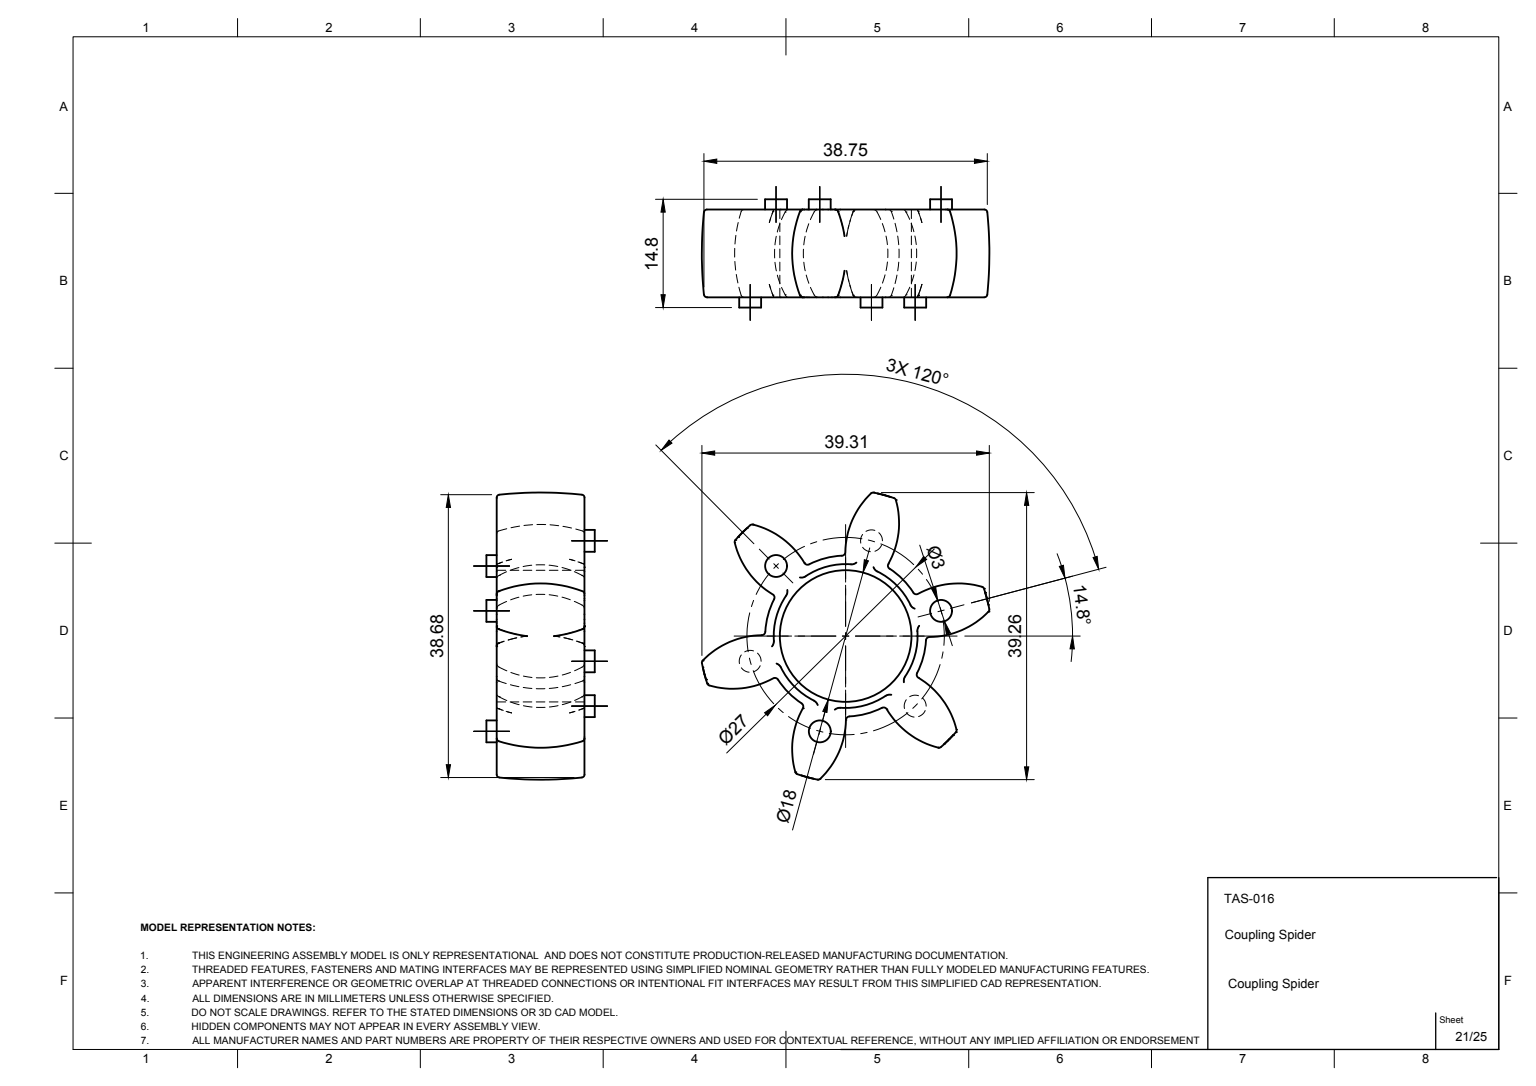
ISO-10303-21;
HEADER;
/* Generated by software containing ST-Developer
 * from STEP Tools, Inc. (www.steptools.com) 
 */

FILE_DESCRIPTION(
/* description */ ('STEP AP214'),
/* implementation_level */ '2;1');

FILE_NAME(
/* name */ 'Coupling Spider.step',
/* time_stamp */ '2026-11-15T14:55:55-08:00',
/* author */ (''),
/* organization */ (''),
/* preprocessor_version */ 'ST-DEVELOPER v20.2',
/* originating_system */ 'Autodesk Translation Framework v15.17.0.0',
/* authorisation */ '');

FILE_SCHEMA (('AUTOMOTIVE_DESIGN { 1 0 10303 214 3 1 1 }'));
ENDSEC;

DATA;
#10=MECHANICAL_DESIGN_GEOMETRIC_PRESENTATION_REPRESENTATION('',(#939),#57079);
#36=B_SPLINE_SURFACE_WITH_KNOTS('',3,3,((#37392,#37393,#37394,#37395,#37396),
(#37397,#37398,#37399,#37400,#37401),(#37402,#37403,#37404,#37405,#37406),
(#37407,#37408,#37409,#37410,#37411),(#37412,#37413,#37414,#37415,#37416),
(#37417,#37418,#37419,#37420,#37421),(#37422,#37423,#37424,#37425,#37426)),
 .UNSPECIFIED.,.F.,.F.,.F.,(4,1,1,1,4),(4,1,4),(0.002628442342492,0.25,
0.5,0.75,0.9693574094799),(0.1621510896547,6.217857289747,12.27407139219),
 .UNSPECIFIED.);
#37=B_SPLINE_SURFACE_WITH_KNOTS('',3,3,((#38122,#38123,#38124,#38125,#38126),
(#38127,#38128,#38129,#38130,#38131),(#38132,#38133,#38134,#38135,#38136),
(#38137,#38138,#38139,#38140,#38141)),.UNSPECIFIED.,.F.,.F.,.F.,(4,4),(4,
1,4),(-0.024990257354348,0.982485330053312),(0.334063910607008,6.217857289747,
12.1016506682418),.UNSPECIFIED.);
#38=B_SPLINE_SURFACE_WITH_KNOTS('',3,3,((#38952,#38953,#38954,#38955,#38956),
(#38957,#38958,#38959,#38960,#38961),(#38962,#38963,#38964,#38965,#38966),
(#38967,#38968,#38969,#38970,#38971),(#38972,#38973,#38974,#38975,#38976),
(#38977,#38978,#38979,#38980,#38981),(#38982,#38983,#38984,#38985,#38986)),
 .UNSPECIFIED.,.F.,.F.,.F.,(4,1,1,1,4),(4,1,4),(0.0306420330999,0.25,0.5,
0.75,0.9973715693979),(0.1621509986241,6.217857289747,12.27408153313),
 .UNSPECIFIED.);
#39=B_SPLINE_SURFACE_WITH_KNOTS('',3,3,((#39922,#39923,#39924,#39925,#39926),
(#39927,#39928,#39929,#39930,#39931),(#39932,#39933,#39934,#39935,#39936),
(#39937,#39938,#39939,#39940,#39941),(#39942,#39943,#39944,#39945,#39946),
(#39947,#39948,#39949,#39950,#39951),(#39952,#39953,#39954,#39955,#39956)),
 .UNSPECIFIED.,.F.,.F.,.F.,(4,1,1,1,4),(4,1,4),(0.002628433572892,0.25,
0.5,0.75,0.9693578567347),(0.1621510896604,6.217857289747,12.27407139218),
 .UNSPECIFIED.);
#40=B_SPLINE_SURFACE_WITH_KNOTS('',3,3,((#40661,#40662,#40663,#40664,#40665),
(#40666,#40667,#40668,#40669,#40670),(#40671,#40672,#40673,#40674,#40675),
(#40676,#40677,#40678,#40679,#40680)),.UNSPECIFIED.,.F.,.F.,.F.,(4,4),(4,
1,4),(-0.0250566951233491,0.98252386483041),(0.33399816619982,6.217857289747,
12.1017164126489),.UNSPECIFIED.);
#41=B_SPLINE_SURFACE_WITH_KNOTS('',3,3,((#41491,#41492,#41493,#41494,#41495),
(#41496,#41497,#41498,#41499,#41500),(#41501,#41502,#41503,#41504,#41505),
(#41506,#41507,#41508,#41509,#41510),(#41511,#41512,#41513,#41514,#41515),
(#41516,#41517,#41518,#41519,#41520),(#41521,#41522,#41523,#41524,#41525)),
 .UNSPECIFIED.,.F.,.F.,.F.,(4,1,1,1,4),(4,1,4),(0.03064262133498,0.25,0.5,
0.75,0.9973715578641),(0.1621509986155,6.217857289747,12.27408153314),
 .UNSPECIFIED.);
#42=B_SPLINE_SURFACE_WITH_KNOTS('',3,3,((#42483,#42484,#42485,#42486,#42487),
(#42488,#42489,#42490,#42491,#42492),(#42493,#42494,#42495,#42496,#42497),
(#42498,#42499,#42500,#42501,#42502),(#42503,#42504,#42505,#42506,#42507),
(#42508,#42509,#42510,#42511,#42512),(#42513,#42514,#42515,#42516,#42517)),
 .UNSPECIFIED.,.F.,.F.,.F.,(4,1,1,1,4),(4,1,4),(0.002628427667201,0.25,
0.5,0.75,0.9693581579284),(0.1621510896466,6.217857289747,12.2740713922),
 .UNSPECIFIED.);
#43=B_SPLINE_SURFACE_WITH_KNOTS('',3,3,((#43199,#43200,#43201,#43202,#43203),
(#43204,#43205,#43206,#43207,#43208),(#43209,#43210,#43211,#43212,#43213),
(#43214,#43215,#43216,#43217,#43218)),.UNSPECIFIED.,.F.,.F.,.F.,(4,4),(4,
1,4),(-0.025111513161759,0.982555658087823),(0.333943919417255,6.217857289747,
12.1017706594305),.UNSPECIFIED.);
#44=B_SPLINE_SURFACE_WITH_KNOTS('',3,3,((#44029,#44030,#44031,#44032,#44033),
(#44034,#44035,#44036,#44037,#44038),(#44039,#44040,#44041,#44042,#44043),
(#44044,#44045,#44046,#44047,#44048),(#44049,#44050,#44051,#44052,#44053),
(#44054,#44055,#44056,#44057,#44058),(#44059,#44060,#44061,#44062,#44063)),
 .UNSPECIFIED.,.F.,.F.,.F.,(4,1,1,1,4),(4,1,4),(0.0306416740573,0.25,0.5,
0.75,0.9973715764379),(0.1621509986173,6.217857289747,12.27408153313),
 .UNSPECIFIED.);
#45=B_SPLINE_SURFACE_WITH_KNOTS('',3,3,((#45013,#45014,#45015,#45016,#45017),
(#45018,#45019,#45020,#45021,#45022),(#45023,#45024,#45025,#45026,#45027),
(#45028,#45029,#45030,#45031,#45032),(#45033,#45034,#45035,#45036,#45037),
(#45038,#45039,#45040,#45041,#45042),(#45043,#45044,#45045,#45046,#45047)),
 .UNSPECIFIED.,.F.,.F.,.F.,(4,1,1,1,4),(4,1,4),(0.002628398063673,0.25,
0.5,0.75,0.9693596677257),(0.1621510897017,6.217857289747,12.27407139231),
 .UNSPECIFIED.);
#46=B_SPLINE_SURFACE_WITH_KNOTS('',3,3,((#45733,#45734,#45735,#45736,#45737),
(#45738,#45739,#45740,#45741,#45742),(#45743,#45744,#45745,#45746,#45747),
(#45748,#45749,#45750,#45751,#45752)),.UNSPECIFIED.,.F.,.F.,.F.,(4,4),(4,
1,4),(-0.0251115131966662,0.982555658077179),(0.3339439193833,6.217857289747,
12.1017706594645),.UNSPECIFIED.);
#47=B_SPLINE_SURFACE_WITH_KNOTS('',3,3,((#46556,#46557,#46558,#46559,#46560),
(#46561,#46562,#46563,#46564,#46565),(#46566,#46567,#46568,#46569,#46570),
(#46571,#46572,#46573,#46574,#46575),(#46576,#46577,#46578,#46579,#46580),
(#46581,#46582,#46583,#46584,#46585),(#46586,#46587,#46588,#46589,#46590)),
 .UNSPECIFIED.,.F.,.F.,.F.,(4,1,1,1,4),(4,1,4),(0.03064220512297,0.25,0.5,
0.75,0.997371566025),(0.1621509986341,6.217857289747,12.27408153327),
 .UNSPECIFIED.);
#48=B_SPLINE_SURFACE_WITH_KNOTS('',3,3,((#47286,#47287,#47288,#47289,#47290),
(#47291,#47292,#47293,#47294,#47295),(#47296,#47297,#47298,#47299,#47300),
(#47301,#47302,#47303,#47304,#47305),(#47306,#47307,#47308,#47309,#47310),
(#47311,#47312,#47313,#47314,#47315),(#47316,#47317,#47318,#47319,#47320)),
 .UNSPECIFIED.,.F.,.F.,.F.,(4,1,1,1,4),(4,1,4),(0.002628430752027,0.25,
0.5,0.75,0.9693580006005),(0.1621510896555,6.217857289747,12.27407139218),
 .UNSPECIFIED.);
#49=B_SPLINE_SURFACE_WITH_KNOTS('',3,3,((#48651,#48652,#48653,#48654,#48655),
(#48656,#48657,#48658,#48659,#48660),(#48661,#48662,#48663,#48664,#48665),
(#48666,#48667,#48668,#48669,#48670),(#48671,#48672,#48673,#48674,#48675),
(#48676,#48677,#48678,#48679,#48680),(#48681,#48682,#48683,#48684,#48685)),
 .UNSPECIFIED.,.F.,.F.,.F.,(4,1,1,1,4),(4,1,4),(0.002629007110398,0.25,
0.5,0.75,0.9693286059854),(0.162151089685,6.217857289747,12.27407139234),
 .UNSPECIFIED.);
#50=B_SPLINE_SURFACE_WITH_KNOTS('',3,3,((#49402,#49403,#49404,#49405,#49406),
(#49407,#49408,#49409,#49410,#49411),(#49412,#49413,#49414,#49415,#49416),
(#49417,#49418,#49419,#49420,#49421)),.UNSPECIFIED.,.F.,.F.,.F.,(4,4),(4,
1,4),(-0.025177674866951,0.982594028216162),(0.333878446168046,6.217857289747,
12.1018361326796),.UNSPECIFIED.);
#51=B_SPLINE_SURFACE_WITH_KNOTS('',3,3,((#50226,#50227,#50228,#50229,#50230),
(#50231,#50232,#50233,#50234,#50235),(#50236,#50237,#50238,#50239,#50240),
(#50241,#50242,#50243,#50244,#50245),(#50246,#50247,#50248,#50249,#50250),
(#50251,#50252,#50253,#50254,#50255),(#50256,#50257,#50258,#50259,#50260)),
 .UNSPECIFIED.,.F.,.F.,.F.,(4,1,1,1,4),(4,1,4),(0.03067153885244,0.25,0.5,
0.75,0.9973709908605),(0.1621509986464,6.217857289747,12.27408153326),
 .UNSPECIFIED.);
#52=B_SPLINE_SURFACE_WITH_KNOTS('',3,3,((#50705,#50706,#50707,#50708,#50709),
(#50710,#50711,#50712,#50713,#50714),(#50715,#50716,#50717,#50718,#50719),
(#50720,#50721,#50722,#50723,#50724)),.UNSPECIFIED.,.F.,.F.,.F.,(4,4),(4,
1,4),(-0.0249902573400751,0.982485330102956),(0.334063910620545,6.217857289747,
12.1016506682281),.UNSPECIFIED.);
#53=B_SPLINE_SURFACE_WITH_KNOTS('',3,3,((#51211,#51212,#51213,#51214,#51215),
(#51216,#51217,#51218,#51219,#51220),(#51221,#51222,#51223,#51224,#51225),
(#51226,#51227,#51228,#51229,#51230),(#51231,#51232,#51233,#51234,#51235),
(#51236,#51237,#51238,#51239,#51240),(#51241,#51242,#51243,#51244,#51245)),
 .UNSPECIFIED.,.F.,.F.,.F.,(4,1,1,1,4),(4,1,4),(0.03064179013217,0.25,0.5,
0.75,0.997371574162),(0.1621509986021,6.217857289747,12.27408153315),
 .UNSPECIFIED.);
#54=ELLIPSE('',#25490,14.1459545202442,4.90175276915756);
#55=ELLIPSE('',#25504,38.974702057433,37.2141854840257);
#56=ELLIPSE('',#25512,14.1454026092901,4.90137019917901);
#57=ELLIPSE('',#25526,38.9778279365771,37.2201555784017);
#58=ELLIPSE('',#25534,14.1449420010391,4.90105113596068);
#59=ELLIPSE('',#25548,38.975599782719,37.215899615947);
#60=ELLIPSE('',#25556,14.1449570638359,4.90106151145033);
#61=ELLIPSE('',#25570,38.9740482939914,37.2129370257381);
#62=ELLIPSE('',#25579,14.14611930392,4.90186695347628);
#63=ELLIPSE('',#25593,14.1445653378396,4.90078996091196);
#64=ELLIPSE('',#25607,38.9767662731696,37.2181280215083);
#65=ELLIPSE('',#25633,38.97568443858,37.2160612851944);
#162=(
BOUNDED_SURFACE()
B_SPLINE_SURFACE(3,3,((#36423,#36424,#36425,#36426,#36427,#36428,#36429,
#36430,#36431,#36432),(#36433,#36434,#36435,#36436,#36437,#36438,#36439,
#36440,#36441,#36442),(#36443,#36444,#36445,#36446,#36447,#36448,#36449,
#36450,#36451,#36452),(#36453,#36454,#36455,#36456,#36457,#36458,#36459,
#36460,#36461,#36462)),.UNSPECIFIED.,.F.,.F.,.F.)
B_SPLINE_SURFACE_WITH_KNOTS((4,4),(4,1,1,1,1,1,1,4),(0.0902477597713112,
0.904395368827396),(0.02358777781772,0.1427066556452,0.2856868894759,0.4285070295258,
0.571316470583,0.7141880571253,0.8571205016359,0.9886565450754),
 .UNSPECIFIED.)
GEOMETRIC_REPRESENTATION_ITEM()
RATIONAL_B_SPLINE_SURFACE(((1.11546174586943,1.11546174586943,1.11546174586943,
1.11546174586943,1.11546174586943,1.11546174586943,1.11546174586943,1.11546174586943,
1.11546174586943,1.11546174586943),(0.962519072862034,0.962519072862034,
0.962519072862034,0.962519072862034,0.962519072862034,0.962519072862034,
0.962519072862034,0.962519072862034,0.962519072862034,0.962519072862034),
(0.96151932941876,0.96151932941876,0.96151932941876,0.96151932941876,0.96151932941876,
0.96151932941876,0.96151932941876,0.96151932941876,0.96151932941876,0.96151932941876),
(1.1124625155396,1.1124625155396,1.1124625155396,1.1124625155396,1.1124625155396,
1.1124625155396,1.1124625155396,1.1124625155396,1.1124625155396,1.1124625155396)))
REPRESENTATION_ITEM('')
SURFACE()
);
#163=(
BOUNDED_SURFACE()
B_SPLINE_SURFACE(3,3,((#36555,#36556,#36557,#36558,#36559,#36560,#36561,
#36562,#36563),(#36564,#36565,#36566,#36567,#36568,#36569,#36570,#36571,
#36572),(#36573,#36574,#36575,#36576,#36577,#36578,#36579,#36580,#36581),
(#36582,#36583,#36584,#36585,#36586,#36587,#36588,#36589,#36590)),
 .UNSPECIFIED.,.F.,.F.,.F.)
B_SPLINE_SURFACE_WITH_KNOTS((4,4),(4,1,1,1,1,1,4),(0.0546212561079652,0.945380228523745),
(0.228750194394892,0.3042889925712,0.4133392424319,0.5264696341084,0.6424947869233,
0.7601009691825,0.774320140471063),.UNSPECIFIED.)
GEOMETRIC_REPRESENTATION_ITEM()
RATIONAL_B_SPLINE_SURFACE(((1.19596662858113,1.19596662858113,1.19596662858113,
1.19596662858113,1.19596662858113,1.19596662858113,1.19596662858113,1.19596662858113,
1.19596662858113),(0.934677354980995,0.934677354980995,0.934677354980995,
0.934677354980995,0.934677354980995,0.934677354980995,0.934677354980995,
0.934677354980995,0.934677354980995),(0.934677790473648,0.934677790473648,
0.934677790473648,0.934677790473648,0.934677790473648,0.934677790473648,
0.934677790473648,0.934677790473648,0.934677790473648),(1.19596793505909,
1.19596793505909,1.19596793505909,1.19596793505909,1.19596793505909,1.19596793505909,
1.19596793505909,1.19596793505909,1.19596793505909)))
REPRESENTATION_ITEM('')
SURFACE()
);
#164=(
BOUNDED_SURFACE()
B_SPLINE_SURFACE(3,3,((#36641,#36642,#36643,#36644,#36645,#36646,#36647,
#36648,#36649),(#36650,#36651,#36652,#36653,#36654,#36655,#36656,#36657,
#36658),(#36659,#36660,#36661,#36662,#36663,#36664,#36665,#36666,#36667),
(#36668,#36669,#36670,#36671,#36672,#36673,#36674,#36675,#36676)),
 .UNSPECIFIED.,.F.,.F.,.F.)
B_SPLINE_SURFACE_WITH_KNOTS((4,4),(4,1,1,1,1,1,4),(0.0545959214790058,0.945405071292651),
(0.226579922118566,0.3006458185639,0.4098657082077,0.5233967602133,0.640305105005,
0.7591301880899,0.772969164981535),.UNSPECIFIED.)
GEOMETRIC_REPRESENTATION_ITEM()
RATIONAL_B_SPLINE_SURFACE(((1.19598782351354,1.19598782351354,1.19598782351354,
1.19598782351354,1.19598782351354,1.19598782351354,1.19598782351354,1.19598782351354,
1.19598782351354),(0.934670434267463,0.934670434267463,0.934670434267463,
0.934670434267463,0.934670434267463,0.934670434267463,0.934670434267463,
0.934670434267463,0.934670434267463),(0.93467072549571,0.93467072549571,
0.93467072549571,0.93467072549571,0.93467072549571,0.93467072549571,0.93467072549571,
0.93467072549571,0.93467072549571),(1.19598869719828,1.19598869719828,1.19598869719828,
1.19598869719828,1.19598869719828,1.19598869719828,1.19598869719828,1.19598869719828,
1.19598869719828)))
REPRESENTATION_ITEM('')
SURFACE()
);
#165=(
BOUNDED_SURFACE()
B_SPLINE_SURFACE(3,3,((#36787,#36788,#36789,#36790,#36791,#36792,#36793,
#36794,#36795,#36796,#36797),(#36798,#36799,#36800,#36801,#36802,#36803,
#36804,#36805,#36806,#36807,#36808),(#36809,#36810,#36811,#36812,#36813,
#36814,#36815,#36816,#36817,#36818,#36819),(#36820,#36821,#36822,#36823,
#36824,#36825,#36826,#36827,#36828,#36829,#36830)),.UNSPECIFIED.,.F.,.F.,
 .F.)
B_SPLINE_SURFACE_WITH_KNOTS((4,4),(4,1,1,1,1,1,1,1,4),(0.0753633924341077,
0.903558847349357),(-0.009670337421386,0.,0.1430991485311,0.2858285059199,
0.4284781713031,0.5715215149008,0.7145472299923,0.8573672624017,0.9759160460961),
 .UNSPECIFIED.)
GEOMETRIC_REPRESENTATION_ITEM()
RATIONAL_B_SPLINE_SURFACE(((1.12354604895393,1.12354604895393,1.12354604895393,
1.12354604895393,1.12354604895393,1.12354604895393,1.12354604895393,1.12354604895393,
1.12354604895393,1.12354604895393,1.12354604895393),(0.962906301315212,
0.962906301315212,0.962906301315212,0.962906301315212,0.962906301315212,
0.962906301315212,0.962906301315212,0.962906301315212,0.962906301315212,
0.962906301315212,0.962906301315212),(0.958919449944363,0.958919449944363,
0.958919449944363,0.958919449944363,0.958919449944363,0.958919449944363,
0.958919449944363,0.958919449944363,0.958919449944363,0.958919449944363,
0.958919449944363),(1.11158549484138,1.11158549484138,1.11158549484138,
1.11158549484138,1.11158549484138,1.11158549484138,1.11158549484138,1.11158549484138,
1.11158549484138,1.11158549484138,1.11158549484138)))
REPRESENTATION_ITEM('')
SURFACE()
);
#166=(
BOUNDED_SURFACE()
B_SPLINE_SURFACE(3,3,((#36947,#36948,#36949,#36950),(#36951,#36952,#36953,
#36954),(#36955,#36956,#36957,#36958),(#36959,#36960,#36961,#36962)),
 .UNSPECIFIED.,.F.,.F.,.F.)
B_SPLINE_SURFACE_WITH_KNOTS((4,4),(4,4),(0.0986320320063612,0.901362552769513),
(-0.975145040413366,-0.0991746183846591),.UNSPECIFIED.)
GEOMETRIC_REPRESENTATION_ITEM()
RATIONAL_B_SPLINE_SURFACE(((1.17563600435392,1.17563600435392,1.17563600435392,
1.17563600435392),(0.941456244993259,0.941456244993259,0.941456244993259,
0.941456244993259),(0.941454665226083,0.941454665226083,0.941454665226083,
0.941454665226083),(1.17563126505239,1.17563126505239,1.17563126505239,
1.17563126505239)))
REPRESENTATION_ITEM('')
SURFACE()
);
#167=(
BOUNDED_SURFACE()
B_SPLINE_SURFACE(3,3,((#36981,#36982,#36983,#36984,#36985,#36986,#36987,
#36988,#36989,#36990,#36991,#36992,#36993,#36994,#36995,#36996,#36997,#36998,
#36999,#37000,#37001,#37002,#37003,#37004,#37005,#37006,#37007,#37008,#37009,
#37010,#37011,#37012,#37013),(#37014,#37015,#37016,#37017,#37018,#37019,
#37020,#37021,#37022,#37023,#37024,#37025,#37026,#37027,#37028,#37029,#37030,
#37031,#37032,#37033,#37034,#37035,#37036,#37037,#37038,#37039,#37040,#37041,
#37042,#37043,#37044,#37045,#37046),(#37047,#37048,#37049,#37050,#37051,
#37052,#37053,#37054,#37055,#37056,#37057,#37058,#37059,#37060,#37061,#37062,
#37063,#37064,#37065,#37066,#37067,#37068,#37069,#37070,#37071,#37072,#37073,
#37074,#37075,#37076,#37077,#37078,#37079),(#37080,#37081,#37082,#37083,
#37084,#37085,#37086,#37087,#37088,#37089,#37090,#37091,#37092,#37093,#37094,
#37095,#37096,#37097,#37098,#37099,#37100,#37101,#37102,#37103,#37104,#37105,
#37106,#37107,#37108,#37109,#37110,#37111,#37112)),.UNSPECIFIED.,.F.,.F.,
 .F.)
B_SPLINE_SURFACE_WITH_KNOTS((4,4),(4,1,1,1,1,1,1,1,1,1,1,1,1,1,1,1,1,1,
1,1,1,1,1,1,1,1,1,1,1,1,4),(0.10838765227344,0.903585982727356),(-0.009736901738826,
0.,0.02218340749156,0.04656850383685,0.07320121634793,0.1023238311649,0.1343066238742,
0.1695984990871,0.2086121558937,0.2515303853623,0.2985746389689,0.3503366286804,
0.4076785718738,0.4682255700465,0.5282360307704,0.5849839255388,0.6367806003914,
0.6825368401892,0.7235074075059,0.7605068126506,0.7940285468273,0.8241776680761,
0.851065051828,0.8750212083666,0.8964625051056,0.9157946807006,0.9333731860455,
0.9493575699015,0.9638584550806,0.977054470158,0.9857155005173),
 .UNSPECIFIED.)
GEOMETRIC_REPRESENTATION_ITEM()
RATIONAL_B_SPLINE_SURFACE(((1.07414161106601,1.07414161106601,1.07414161106601,
1.07414161106601,1.07414161106601,1.07414161106601,1.07414161106601,1.07414161106601,
1.07414161106601,1.07414161106601,1.07414161106601,1.07414161106601,1.07414161106601,
1.07414161106601,1.07414161106601,1.07414161106601,1.07414161106601,1.07414161106601,
1.07414161106601,1.07414161106601,1.07414161106601,1.07414161106601,1.07414161106601,
1.07414161106601,1.07414161106601,1.07414161106601,1.07414161106601,1.07414161106601,
1.07414161106601,1.07414161106601,1.07414161106601,1.07414161106601,1.07414161106601),
(0.973774865432272,0.973774865432272,0.973774865432272,0.973774865432272,
0.973774865432272,0.973774865432272,0.973774865432272,0.973774865432272,
0.973774865432272,0.973774865432272,0.973774865432272,0.973774865432272,
0.973774865432272,0.973774865432272,0.973774865432272,0.973774865432272,
0.973774865432272,0.973774865432272,0.973774865432272,0.973774865432272,
0.973774865432272,0.973774865432272,0.973774865432272,0.973774865432272,
0.973774865432272,0.973774865432272,0.973774865432272,0.973774865432272,
0.973774865432272,0.973774865432272,0.973774865432272,0.973774865432272,
0.973774865432272),(0.975309233264917,0.975309233264917,0.975309233264917,
0.975309233264917,0.975309233264917,0.975309233264917,0.975309233264917,
0.975309233264917,0.975309233264917,0.975309233264917,0.975309233264917,
0.975309233264917,0.975309233264917,0.975309233264917,0.975309233264917,
0.975309233264917,0.975309233264917,0.975309233264917,0.975309233264917,
0.975309233264917,0.975309233264917,0.975309233264917,0.975309233264917,
0.975309233264917,0.975309233264917,0.975309233264917,0.975309233264917,
0.975309233264917,0.975309233264917,0.975309233264917,0.975309233264917,
0.975309233264917,0.975309233264917),(1.07874471456394,1.07874471456394,
1.07874471456394,1.07874471456394,1.07874471456394,1.07874471456394,1.07874471456394,
1.07874471456394,1.07874471456394,1.07874471456394,1.07874471456394,1.07874471456394,
1.07874471456394,1.07874471456394,1.07874471456394,1.07874471456394,1.07874471456394,
1.07874471456394,1.07874471456394,1.07874471456394,1.07874471456394,1.07874471456394,
1.07874471456394,1.07874471456394,1.07874471456394,1.07874471456394,1.07874471456394,
1.07874471456394,1.07874471456394,1.07874471456394,1.07874471456394,1.07874471456394,
1.07874471456394)))
REPRESENTATION_ITEM('')
SURFACE()
);
#168=(
BOUNDED_SURFACE()
B_SPLINE_SURFACE(3,3,((#37499,#37500,#37501,#37502,#37503,#37504,#37505,
#37506,#37507,#37508),(#37509,#37510,#37511,#37512,#37513,#37514,#37515,
#37516,#37517,#37518),(#37519,#37520,#37521,#37522,#37523,#37524,#37525,
#37526,#37527,#37528),(#37529,#37530,#37531,#37532,#37533,#37534,#37535,
#37536,#37537,#37538)),.UNSPECIFIED.,.F.,.F.,.F.)
B_SPLINE_SURFACE_WITH_KNOTS((4,4),(4,1,1,1,1,1,1,4),(0.0573940888734465,
0.942594572239928),(0.2949017622243,0.3477745082592,0.410039088065,0.4702670303195,
0.5296668592001,0.589892029113,0.6521532381952,0.7051388515263),
 .UNSPECIFIED.)
GEOMETRIC_REPRESENTATION_ITEM()
RATIONAL_B_SPLINE_SURFACE(((1.19352947582456,1.19352947582456,1.19352947582456,
1.19352947582456,1.19352947582456,1.19352947582456,1.19352947582456,1.19352947582456,
1.19352947582456,1.19352947582456),(0.935493480011236,0.935493480011236,
0.935493480011236,0.935493480011236,0.935493480011236,0.935493480011236,
0.935493480011236,0.935493480011236,0.935493480011236,0.935493480011236),
(0.935490174767419,0.935490174767419,0.935490174767419,0.935490174767419,
0.935490174767419,0.935490174767419,0.935490174767419,0.935490174767419,
0.935490174767419,0.935490174767419),(1.19351956009311,1.19351956009311,
1.19351956009311,1.19351956009311,1.19351956009311,1.19351956009311,1.19351956009311,
1.19351956009311,1.19351956009311,1.19351956009311)))
REPRESENTATION_ITEM('')
SURFACE()
);
#169=(
BOUNDED_SURFACE()
B_SPLINE_SURFACE(3,3,((#37638,#37639,#37640,#37641,#37642,#37643,#37644,
#37645,#37646),(#37647,#37648,#37649,#37650,#37651,#37652,#37653,#37654,
#37655),(#37656,#37657,#37658,#37659,#37660,#37661,#37662,#37663,#37664),
(#37665,#37666,#37667,#37668,#37669,#37670,#37671,#37672,#37673)),
 .UNSPECIFIED.,.F.,.F.,.F.)
B_SPLINE_SURFACE_WITH_KNOTS((4,4),(4,1,1,1,1,1,4),(0.0546805339304302,0.945320968231971),
(0.225741042054691,0.2411747389776,0.3599582619163,0.4768206617319,0.5903023688695,
0.6994747309877,0.773101800008629),.UNSPECIFIED.)
GEOMETRIC_REPRESENTATION_ITEM()
RATIONAL_B_SPLINE_SURFACE(((1.19591424064832,1.19591424064832,1.19591424064832,
1.19591424064832,1.19591424064832,1.19591424064832,1.19591424064832,1.19591424064832,
1.19591424064832),(0.934694812542253,0.934694812542253,0.934694812542253,
0.934694812542253,0.934694812542253,0.934694812542253,0.934694812542253,
0.934694812542253,0.934694812542253),(0.934695253118102,0.934695253118102,
0.934695253118102,0.934695253118102,0.934695253118102,0.934695253118102,
0.934695253118102,0.934695253118102,0.934695253118102),(1.19591556237587,
1.19591556237587,1.19591556237587,1.19591556237587,1.19591556237587,1.19591556237587,
1.19591556237587,1.19591556237587,1.19591556237587)))
REPRESENTATION_ITEM('')
SURFACE()
);
#170=(
BOUNDED_SURFACE()
B_SPLINE_SURFACE(3,3,((#37790,#37791,#37792,#37793,#37794,#37795,#37796,
#37797,#37798,#37799),(#37800,#37801,#37802,#37803,#37804,#37805,#37806,
#37807,#37808,#37809),(#37810,#37811,#37812,#37813,#37814,#37815,#37816,
#37817,#37818,#37819),(#37820,#37821,#37822,#37823,#37824,#37825,#37826,
#37827,#37828,#37829)),.UNSPECIFIED.,.F.,.F.,.F.)
B_SPLINE_SURFACE_WITH_KNOTS((4,4),(4,1,1,1,1,1,1,4),(0.0902148383069544,
0.903852967096121),(0.01134228752749,0.1428795013597,0.2858119516079,0.4286835332756,
0.5714929665995,0.7143131101565,0.8572933444563,0.9764111906646),
 .UNSPECIFIED.)
GEOMETRIC_REPRESENTATION_ITEM()
RATIONAL_B_SPLINE_SURFACE(((1.11548029903383,1.11548029903383,1.11548029903383,
1.11548029903383,1.11548029903383,1.11548029903383,1.11548029903383,1.11548029903383,
1.11548029903383,1.11548029903383),(0.962621056026685,0.962621056026685,
0.962621056026685,0.962621056026685,0.962621056026685,0.962621056026685,
0.962621056026685,0.962621056026685,0.962621056026685,0.962621056026685),
(0.961514633856943,0.961514633856943,0.961514633856943,0.961514633856943,
0.961514633856943,0.961514633856943,0.961514633856943,0.961514633856943,
0.961514633856943,0.961514633856943),(1.1121610325246,1.1121610325246,1.1121610325246,
1.1121610325246,1.1121610325246,1.1121610325246,1.1121610325246,1.1121610325246,
1.1121610325246,1.1121610325246)))
REPRESENTATION_ITEM('')
SURFACE()
);
#171=(
BOUNDED_SURFACE()
B_SPLINE_SURFACE(3,3,((#37856,#37857,#37858,#37859,#37860,#37861,#37862,
#37863,#37864),(#37865,#37866,#37867,#37868,#37869,#37870,#37871,#37872,
#37873),(#37874,#37875,#37876,#37877,#37878,#37879,#37880,#37881,#37882),
(#37883,#37884,#37885,#37886,#37887,#37888,#37889,#37890,#37891)),
 .UNSPECIFIED.,.F.,.F.,.F.)
B_SPLINE_SURFACE_WITH_KNOTS((4,4),(4,1,1,1,1,1,4),(0.0546950340476835,0.945306466434247),
(0.226871363787984,0.3005222549961,0.4096933649143,0.5231718563143,0.6400288266084,
0.7588043312261,0.774243594722914),.UNSPECIFIED.)
GEOMETRIC_REPRESENTATION_ITEM()
RATIONAL_B_SPLINE_SURFACE(((1.19590147953157,1.19590147953157,1.19590147953157,
1.19590147953157,1.19590147953157,1.19590147953157,1.19590147953157,1.19590147953157,
1.19590147953157),(0.934699066754979,0.934699066754979,0.934699066754979,
0.934699066754979,0.934699066754979,0.934699066754979,0.934699066754979,
0.934699066754979,0.934699066754979),(0.934699506823618,0.934699506823618,
0.934699506823618,0.934699506823618,0.934699506823618,0.934699506823618,
0.934699506823618,0.934699506823618,0.934699506823618),(1.19590279973749,
1.19590279973749,1.19590279973749,1.19590279973749,1.19590279973749,1.19590279973749,
1.19590279973749,1.19590279973749,1.19590279973749)))
REPRESENTATION_ITEM('')
SURFACE()
);
#172=(
BOUNDED_SURFACE()
B_SPLINE_SURFACE(3,3,((#38005,#38006,#38007,#38008,#38009,#38010,#38011,
#38012,#38013,#38014),(#38015,#38016,#38017,#38018,#38019,#38020,#38021,
#38022,#38023,#38024),(#38025,#38026,#38027,#38028,#38029,#38030,#38031,
#38032,#38033,#38034),(#38035,#38036,#38037,#38038,#38039,#38040,#38041,
#38042,#38043,#38044)),.UNSPECIFIED.,.F.,.F.,.F.)
B_SPLINE_SURFACE_WITH_KNOTS((4,4),(4,1,1,1,1,1,1,4),(0.0902464241409013,
0.90385943340213),(0.02358777781733,0.1427066555246,0.2856868899129,0.4285070341315,
0.5713164659964,0.7141880467444,0.8571204980751,0.9886565450756),
 .UNSPECIFIED.)
GEOMETRIC_REPRESENTATION_ITEM()
RATIONAL_B_SPLINE_SURFACE(((1.115462498594,1.115462498594,1.115462498594,
1.115462498594,1.115462498594,1.115462498594,1.115462498594,1.115462498594,
1.115462498594,1.115462498594),(0.962619755259846,0.962619755259846,0.962619755259846,
0.962619755259846,0.962619755259846,0.962619755259846,0.962619755259846,
0.962619755259846,0.962619755259846,0.962619755259846),(0.961520464178815,
0.961520464178815,0.961520464178815,0.961520464178815,0.961520464178815,
0.961520464178815,0.961520464178815,0.961520464178815,0.961520464178815,
0.961520464178815),(1.11216462535091,1.11216462535091,1.11216462535091,
1.11216462535091,1.11216462535091,1.11216462535091,1.11216462535091,1.11216462535091,
1.11216462535091,1.11216462535091)))
REPRESENTATION_ITEM('')
SURFACE()
);
#173=(
BOUNDED_SURFACE()
B_SPLINE_SURFACE(3,3,((#38084,#38085,#38086,#38087,#38088,#38089),(#38090,
#38091,#38092,#38093,#38094,#38095),(#38096,#38097,#38098,#38099,#38100,
#38101),(#38102,#38103,#38104,#38105,#38106,#38107)),.UNSPECIFIED.,.F.,
 .F.,.F.)
B_SPLINE_SURFACE_WITH_KNOTS((4,4),(4,1,1,4),(0.098634219138839,0.901369959992847),
(0.317543733196422,0.3333147448851,0.6666852551146,0.682456266811579),
 .UNSPECIFIED.)
GEOMETRIC_REPRESENTATION_ITEM()
RATIONAL_B_SPLINE_SURFACE(((1.17563408853202,1.17563408853202,1.17563408853202,
1.17563408853202,1.17563408853202,1.17563408853202),(0.941454084655573,
0.941454084655573,0.941454084655573,0.941454084655573,0.941454084655573,
0.941454084655573),(0.941455303829106,0.941455303829106,0.941455303829106,
0.941455303829106,0.941455303829106,0.941455303829106),(1.17563774605262,
1.17563774605262,1.17563774605262,1.17563774605262,1.17563774605262,1.17563774605262)))
REPRESENTATION_ITEM('')
SURFACE()
);
#174=(
BOUNDED_SURFACE()
B_SPLINE_SURFACE(3,3,((#38347,#38348,#38349,#38350,#38351,#38352,#38353,
#38354,#38355,#38356,#38357,#38358,#38359,#38360,#38361,#38362,#38363,#38364,
#38365,#38366,#38367,#38368,#38369,#38370,#38371,#38372,#38373,#38374,#38375,
#38376,#38377,#38378,#38379,#38380,#38381,#38382,#38383,#38384,#38385,#38386),
(#38387,#38388,#38389,#38390,#38391,#38392,#38393,#38394,#38395,#38396,
#38397,#38398,#38399,#38400,#38401,#38402,#38403,#38404,#38405,#38406,#38407,
#38408,#38409,#38410,#38411,#38412,#38413,#38414,#38415,#38416,#38417,#38418,
#38419,#38420,#38421,#38422,#38423,#38424,#38425,#38426),(#38427,#38428,
#38429,#38430,#38431,#38432,#38433,#38434,#38435,#38436,#38437,#38438,#38439,
#38440,#38441,#38442,#38443,#38444,#38445,#38446,#38447,#38448,#38449,#38450,
#38451,#38452,#38453,#38454,#38455,#38456,#38457,#38458,#38459,#38460,#38461,
#38462,#38463,#38464,#38465,#38466),(#38467,#38468,#38469,#38470,#38471,
#38472,#38473,#38474,#38475,#38476,#38477,#38478,#38479,#38480,#38481,#38482,
#38483,#38484,#38485,#38486,#38487,#38488,#38489,#38490,#38491,#38492,#38493,
#38494,#38495,#38496,#38497,#38498,#38499,#38500,#38501,#38502,#38503,#38504,
#38505,#38506)),.UNSPECIFIED.,.F.,.F.,.F.)
B_SPLINE_SURFACE_WITH_KNOTS((4,4),(4,1,1,1,1,1,1,1,1,1,1,1,1,1,1,1,1,1,
1,1,1,1,1,1,1,1,1,1,1,1,1,1,1,1,1,1,1,4),(0.109557825387019,0.885251264327289),
(-0.009601789265351,0.,0.02232759876063,0.04690438428766,0.07379256313496,
0.1032821525101,0.1358145488914,0.1719130282251,0.2120212567552,0.2562571680377,
0.3048298949267,0.3584023231075,0.4161460884584,0.4734208057337,0.5265860543835,
0.5739192804757,0.6155188222739,0.652989783064,0.6871354795262,0.7180181889022,
0.7460302867732,0.7715243416789,0.7947371788944,0.8158355553748,0.8349846338442,
0.8523571535156,0.8681359777146,0.8825006466305,0.8956281837459,0.9076945427556,
0.918845104806,0.9291452127897,0.9386434680723,0.9473863882152,0.9554261628486,
0.9628162067307,0.9696068473728,0.972066289545),.UNSPECIFIED.)
GEOMETRIC_REPRESENTATION_ITEM()
RATIONAL_B_SPLINE_SURFACE(((1.07369782396742,1.07369782396742,1.07369782396742,
1.07369782396742,1.07369782396742,1.07369782396742,1.07369782396742,1.07369782396742,
1.07369782396742,1.07369782396742,1.07369782396742,1.07369782396742,1.07369782396742,
1.07369782396742,1.07369782396742,1.07369782396742,1.07369782396742,1.07369782396742,
1.07369782396742,1.07369782396742,1.07369782396742,1.07369782396742,1.07369782396742,
1.07369782396742,1.07369782396742,1.07369782396742,1.07369782396742,1.07369782396742,
1.07369782396742,1.07369782396742,1.07369782396742,1.07369782396742,1.07369782396742,
1.07369782396742,1.07369782396742,1.07369782396742,1.07369782396742,1.07369782396742,
1.07369782396742,1.07369782396742),(0.976087264738623,0.976087264738623,
0.976087264738623,0.976087264738623,0.976087264738623,0.976087264738623,
0.976087264738623,0.976087264738623,0.976087264738623,0.976087264738623,
0.976087264738623,0.976087264738623,0.976087264738623,0.976087264738623,
0.976087264738623,0.976087264738623,0.976087264738623,0.976087264738623,
0.976087264738623,0.976087264738623,0.976087264738623,0.976087264738623,
0.976087264738623,0.976087264738623,0.976087264738623,0.976087264738623,
0.976087264738623,0.976087264738623,0.976087264738623,0.976087264738623,
0.976087264738623,0.976087264738623,0.976087264738623,0.976087264738623,
0.976087264738623,0.976087264738623,0.976087264738623,0.976087264738623,
0.976087264738623,0.976087264738623),(0.975438400849373,0.975438400849373,
0.975438400849373,0.975438400849373,0.975438400849373,0.975438400849373,
0.975438400849373,0.975438400849373,0.975438400849373,0.975438400849373,
0.975438400849373,0.975438400849373,0.975438400849373,0.975438400849373,
0.975438400849373,0.975438400849373,0.975438400849373,0.975438400849373,
0.975438400849373,0.975438400849373,0.975438400849373,0.975438400849373,
0.975438400849373,0.975438400849373,0.975438400849373,0.975438400849373,
0.975438400849373,0.975438400849373,0.975438400849373,0.975438400849373,
0.975438400849373,0.975438400849373,0.975438400849373,0.975438400849373,
0.975438400849373,0.975438400849373,0.975438400849373,0.975438400849373,
0.975438400849373,0.975438400849373),(1.07175123229967,1.07175123229967,
1.07175123229967,1.07175123229967,1.07175123229967,1.07175123229967,1.07175123229967,
1.07175123229967,1.07175123229967,1.07175123229967,1.07175123229967,1.07175123229967,
1.07175123229967,1.07175123229967,1.07175123229967,1.07175123229967,1.07175123229967,
1.07175123229967,1.07175123229967,1.07175123229967,1.07175123229967,1.07175123229967,
1.07175123229967,1.07175123229967,1.07175123229967,1.07175123229967,1.07175123229967,
1.07175123229967,1.07175123229967,1.07175123229967,1.07175123229967,1.07175123229967,
1.07175123229967,1.07175123229967,1.07175123229967,1.07175123229967,1.07175123229967,
1.07175123229967,1.07175123229967,1.07175123229967)))
REPRESENTATION_ITEM('')
SURFACE()
);
#175=(
BOUNDED_SURFACE()
B_SPLINE_SURFACE(3,3,((#38632,#38633,#38634,#38635,#38636,#38637,#38638,
#38639,#38640),(#38641,#38642,#38643,#38644,#38645,#38646,#38647,#38648,
#38649),(#38650,#38651,#38652,#38653,#38654,#38655,#38656,#38657,#38658),
(#38659,#38660,#38661,#38662,#38663,#38664,#38665,#38666,#38667)),
 .UNSPECIFIED.,.F.,.F.,.F.)
B_SPLINE_SURFACE_WITH_KNOTS((4,4),(4,1,1,1,1,1,4),(0.0545575351232763,0.945444284135705),
(0.226990618484223,0.2408830109944,0.3597029788422,0.4766081773209,0.5901375306023,
0.6993568121791,0.773423227451189),.UNSPECIFIED.)
GEOMETRIC_REPRESENTATION_ITEM()
RATIONAL_B_SPLINE_SURFACE(((1.1960229215533,1.1960229215533,1.1960229215533,
1.1960229215533,1.1960229215533,1.1960229215533,1.1960229215533,1.1960229215533,
1.1960229215533),(0.934658492422782,0.934658492422782,0.934658492422782,
0.934658492422782,0.934658492422782,0.934658492422782,0.934658492422782,
0.934658492422782,0.934658492422782),(0.934659026150056,0.934659026150056,
0.934659026150056,0.934659026150056,0.934659026150056,0.934659026150056,
0.934659026150056,0.934659026150056,0.934659026150056),(1.19602452273512,
1.19602452273512,1.19602452273512,1.19602452273512,1.19602452273512,1.19602452273512,
1.19602452273512,1.19602452273512,1.19602452273512)))
REPRESENTATION_ITEM('')
SURFACE()
);
#176=(
BOUNDED_SURFACE()
B_SPLINE_SURFACE(3,3,((#38790,#38791,#38792,#38793,#38794,#38795,#38796,
#38797,#38798,#38799),(#38800,#38801,#38802,#38803,#38804,#38805,#38806,
#38807,#38808,#38809),(#38810,#38811,#38812,#38813,#38814,#38815,#38816,
#38817,#38818,#38819),(#38820,#38821,#38822,#38823,#38824,#38825,#38826,
#38827,#38828,#38829)),.UNSPECIFIED.,.F.,.F.,.F.)
B_SPLINE_SURFACE_WITH_KNOTS((4,4),(4,1,1,1,1,1,1,4),(0.089702696705292,
0.903562227825136),(0.02295305876099,0.1427319370604,0.2857219203474,0.4285792797614,
0.5713515650105,0.7142098207389,0.8572808214069,0.9622634165798),
 .UNSPECIFIED.)
GEOMETRIC_REPRESENTATION_ITEM()
RATIONAL_B_SPLINE_SURFACE(((1.11534309462385,1.11534309462385,1.11534309462385,
1.11534309462385,1.11534309462385,1.11534309462385,1.11534309462385,1.11534309462385,
1.11534309462385,1.11534309462385),(0.96281454820187,0.96281454820187,0.96281454820187,
0.96281454820187,0.96281454820187,0.96281454820187,0.96281454820187,0.96281454820187,
0.96281454820187,0.96281454820187),(0.961562661748843,0.961562661748843,
0.961562661748843,0.961562661748843,0.961562661748843,0.961562661748843,
0.961562661748843,0.961562661748843,0.961562661748843,0.961562661748843),
(1.11158743526477,1.11158743526477,1.11158743526477,1.11158743526477,1.11158743526477,
1.11158743526477,1.11158743526477,1.11158743526477,1.11158743526477,1.11158743526477)))
REPRESENTATION_ITEM('')
SURFACE()
);
#177=(
BOUNDED_SURFACE()
B_SPLINE_SURFACE(3,3,((#39048,#39049,#39050,#39051,#39052,#39053,#39054,
#39055,#39056,#39057),(#39058,#39059,#39060,#39061,#39062,#39063,#39064,
#39065,#39066,#39067),(#39068,#39069,#39070,#39071,#39072,#39073,#39074,
#39075,#39076,#39077),(#39078,#39079,#39080,#39081,#39082,#39083,#39084,
#39085,#39086,#39087)),.UNSPECIFIED.,.F.,.F.,.F.)
B_SPLINE_SURFACE_WITH_KNOTS((4,4),(4,1,1,1,1,1,1,4),(0.057320173478123,
0.942665361817278),(0.2948675792044,0.3465037559324,0.4092144664244,0.4700480650883,
0.529946403199,0.5907794942564,0.6534941325732,0.7051005237738),
 .UNSPECIFIED.)
GEOMETRIC_REPRESENTATION_ITEM()
RATIONAL_B_SPLINE_SURFACE(((1.19359440570704,1.19359440570704,1.19359440570704,
1.19359440570704,1.19359440570704,1.19359440570704,1.19359440570704,1.19359440570704,
1.19359440570704,1.19359440570704),(0.935472748603642,0.935472748603642,
0.935472748603642,0.935472748603642,0.935472748603642,0.935472748603642,
0.935472748603642,0.935472748603642,0.935472748603642,0.935472748603642),
(0.935468531499884,0.935468531499884,0.935468531499884,0.935468531499884,
0.935468531499884,0.935468531499884,0.935468531499884,0.935468531499884,
0.935468531499884,0.935468531499884),(1.19358175439577,1.19358175439577,
1.19358175439577,1.19358175439577,1.19358175439577,1.19358175439577,1.19358175439577,
1.19358175439577,1.19358175439577,1.19358175439577)))
REPRESENTATION_ITEM('')
SURFACE()
);
#178=(
BOUNDED_SURFACE()
B_SPLINE_SURFACE(3,3,((#39173,#39174,#39175,#39176,#39177,#39178,#39179,
#39180,#39181),(#39182,#39183,#39184,#39185,#39186,#39187,#39188,#39189,
#39190),(#39191,#39192,#39193,#39194,#39195,#39196,#39197,#39198,#39199),
(#39200,#39201,#39202,#39203,#39204,#39205,#39206,#39207,#39208)),
 .UNSPECIFIED.,.F.,.F.,.F.)
B_SPLINE_SURFACE_WITH_KNOTS((4,4),(4,1,1,1,1,1,4),(0.0545718989489667,0.945429093825032),
(0.226579922118891,0.300645818564,0.4098657082078,0.5233967602134,0.6403051050052,
0.7591301880902,0.77299234439195),.UNSPECIFIED.)
GEOMETRIC_REPRESENTATION_ITEM()
RATIONAL_B_SPLINE_SURFACE(((1.19600896499511,1.19600896499511,1.19600896499511,
1.19600896499511,1.19600896499511,1.19600896499511,1.19600896499511,1.19600896499511,
1.19600896499511),(0.934663387090781,0.934663387090781,0.934663387090781,
0.934663387090781,0.934663387090781,0.934663387090781,0.934663387090781,
0.934663387090781,0.934663387090781),(0.934663678335422,0.934663678335422,
0.934663678335422,0.934663678335422,0.934663678335422,0.934663678335422,
0.934663678335422,0.934663678335422,0.934663678335422),(1.19600983872903,
1.19600983872903,1.19600983872903,1.19600983872903,1.19600983872903,1.19600983872903,
1.19600983872903,1.19600983872903,1.19600983872903)))
REPRESENTATION_ITEM('')
SURFACE()
);
#179=(
BOUNDED_SURFACE()
B_SPLINE_SURFACE(3,3,((#39319,#39320,#39321,#39322,#39323,#39324,#39325,
#39326,#39327,#39328,#39329),(#39330,#39331,#39332,#39333,#39334,#39335,
#39336,#39337,#39338,#39339,#39340),(#39341,#39342,#39343,#39344,#39345,
#39346,#39347,#39348,#39349,#39350,#39351),(#39352,#39353,#39354,#39355,
#39356,#39357,#39358,#39359,#39360,#39361,#39362)),.UNSPECIFIED.,.F.,.F.,
 .F.)
B_SPLINE_SURFACE_WITH_KNOTS((4,4),(4,1,1,1,1,1,1,1,4),(0.0753633923116561,
0.903558734772718),(-0.009670337421385,0.,0.1430991485311,0.2858285059199,
0.4284781713031,0.5715215149008,0.7145472299923,0.8573672624017,0.9759160460961),
 .UNSPECIFIED.)
GEOMETRIC_REPRESENTATION_ITEM()
RATIONAL_B_SPLINE_SURFACE(((1.12354604900567,1.12354604900567,1.12354604900567,
1.12354604900567,1.12354604900567,1.12354604900567,1.12354604900567,1.12354604900567,
1.12354604900567,1.12354604900567,1.12354604900567),(0.962906323157822,
0.962906323157822,0.962906323157822,0.962906323157822,0.962906323157822,
0.962906323157822,0.962906323157822,0.962906323157822,0.962906323157822,
0.962906323157822,0.962906323157822),(0.958919451011949,0.958919451011949,
0.958919451011949,0.958919451011949,0.958919451011949,0.958919451011949,
0.958919451011949,0.958919451011949,0.958919451011949,0.958919451011949,
0.958919451011949),(1.11158543256805,1.11158543256805,1.11158543256805,
1.11158543256805,1.11158543256805,1.11158543256805,1.11158543256805,1.11158543256805,
1.11158543256805,1.11158543256805,1.11158543256805)))
REPRESENTATION_ITEM('')
SURFACE()
);
#180=(
BOUNDED_SURFACE()
B_SPLINE_SURFACE(3,3,((#39479,#39480,#39481,#39482),(#39483,#39484,#39485,
#39486),(#39487,#39488,#39489,#39490),(#39491,#39492,#39493,#39494)),
 .UNSPECIFIED.,.F.,.F.,.F.)
B_SPLINE_SURFACE_WITH_KNOTS((4,4),(4,4),(0.0986320319987802,0.901362552767005),
(-0.975145040400083,-0.0991746183717141),.UNSPECIFIED.)
GEOMETRIC_REPRESENTATION_ITEM()
RATIONAL_B_SPLINE_SURFACE(((1.17563600436181,1.17563600436181,1.17563600436181,
1.17563600436181),(0.94145624499344,0.94145624499344,0.94145624499344,0.94145624499344),
(0.94145466522332,0.941454665223321,0.941454665223321,0.941454665223321),
(1.17563126505145,1.17563126505145,1.17563126505145,1.17563126505145)))
REPRESENTATION_ITEM('')
SURFACE()
);
#181=(
BOUNDED_SURFACE()
B_SPLINE_SURFACE(3,3,((#39513,#39514,#39515,#39516,#39517,#39518,#39519,
#39520,#39521,#39522,#39523,#39524,#39525,#39526,#39527,#39528,#39529,#39530,
#39531,#39532,#39533,#39534,#39535,#39536,#39537,#39538,#39539,#39540,#39541,
#39542,#39543,#39544,#39545),(#39546,#39547,#39548,#39549,#39550,#39551,
#39552,#39553,#39554,#39555,#39556,#39557,#39558,#39559,#39560,#39561,#39562,
#39563,#39564,#39565,#39566,#39567,#39568,#39569,#39570,#39571,#39572,#39573,
#39574,#39575,#39576,#39577,#39578),(#39579,#39580,#39581,#39582,#39583,
#39584,#39585,#39586,#39587,#39588,#39589,#39590,#39591,#39592,#39593,#39594,
#39595,#39596,#39597,#39598,#39599,#39600,#39601,#39602,#39603,#39604,#39605,
#39606,#39607,#39608,#39609,#39610,#39611),(#39612,#39613,#39614,#39615,
#39616,#39617,#39618,#39619,#39620,#39621,#39622,#39623,#39624,#39625,#39626,
#39627,#39628,#39629,#39630,#39631,#39632,#39633,#39634,#39635,#39636,#39637,
#39638,#39639,#39640,#39641,#39642,#39643,#39644)),.UNSPECIFIED.,.F.,.F.,
 .F.)
B_SPLINE_SURFACE_WITH_KNOTS((4,4),(4,1,1,1,1,1,1,1,1,1,1,1,1,1,1,1,1,1,
1,1,1,1,1,1,1,1,1,1,1,1,4),(0.108382715709703,0.903586121555296),(-0.009736901741271,
0.,0.02218380445754,0.04656911069387,0.07320179425856,0.1023242565949,0.134306834044,
0.1695984355629,0.2086117112192,0.2515292087379,0.2985721062314,0.3503319196398,
0.4076720811719,0.4682188084844,0.5282303398,0.5849800412443,0.6367784970474,
0.6825358730223,0.7235071660675,0.760507022248,0.7940289957981,0.8241782115926,
0.8510656102853,0.8750217369476,0.8964629740695,0.915795075343,0.9333734980491,
0.949357773524,0.9638585157197,0.9770543997027,0.9857155005215),
 .UNSPECIFIED.)
GEOMETRIC_REPRESENTATION_ITEM()
RATIONAL_B_SPLINE_SURFACE(((1.07414347861564,1.07414347861564,1.07414347861564,
1.07414347861564,1.07414347861564,1.07414347861564,1.07414347861564,1.07414347861564,
1.07414347861564,1.07414347861564,1.07414347861564,1.07414347861564,1.07414347861564,
1.07414347861564,1.07414347861564,1.07414347861564,1.07414347861564,1.07414347861564,
1.07414347861564,1.07414347861564,1.07414347861564,1.07414347861564,1.07414347861564,
1.07414347861564,1.07414347861564,1.07414347861564,1.07414347861564,1.07414347861564,
1.07414347861564,1.07414347861564,1.07414347861564,1.07414347861564,1.07414347861564),
(0.973774829458314,0.973774829458314,0.973774829458314,0.973774829458314,
0.973774829458314,0.973774829458314,0.973774829458314,0.973774829458314,
0.973774829458314,0.973774829458314,0.973774829458314,0.973774829458314,
0.973774829458314,0.973774829458314,0.973774829458314,0.973774829458314,
0.973774829458314,0.973774829458314,0.973774829458314,0.973774829458314,
0.973774829458314,0.973774829458314,0.973774829458314,0.973774829458314,
0.973774829458314,0.973774829458314,0.973774829458314,0.973774829458314,
0.973774829458314,0.973774829458314,0.973774829458314,0.973774829458314,
0.973774829458314),(0.975308592237003,0.975308592237003,0.975308592237003,
0.975308592237003,0.975308592237003,0.975308592237003,0.975308592237003,
0.975308592237003,0.975308592237003,0.975308592237003,0.975308592237003,
0.975308592237003,0.975308592237003,0.975308592237003,0.975308592237003,
0.975308592237003,0.975308592237003,0.975308592237003,0.975308592237003,
0.975308592237003,0.975308592237003,0.975308592237003,0.975308592237003,
0.975308592237003,0.975308592237003,0.975308592237003,0.975308592237003,
0.975308592237003,0.975308592237003,0.975308592237003,0.975308592237003,
0.975308592237003,0.975308592237003),(1.07874476695171,1.07874476695171,
1.07874476695171,1.07874476695171,1.07874476695171,1.07874476695171,1.07874476695171,
1.07874476695171,1.07874476695171,1.07874476695171,1.07874476695171,1.07874476695171,
1.07874476695171,1.07874476695171,1.07874476695171,1.07874476695171,1.07874476695171,
1.07874476695171,1.07874476695171,1.07874476695171,1.07874476695171,1.07874476695171,
1.07874476695171,1.07874476695171,1.07874476695171,1.07874476695171,1.07874476695171,
1.07874476695171,1.07874476695171,1.07874476695171,1.07874476695171,1.07874476695171,
1.07874476695171)))
REPRESENTATION_ITEM('')
SURFACE()
);
#182=(
BOUNDED_SURFACE()
B_SPLINE_SURFACE(3,3,((#40029,#40030,#40031,#40032,#40033,#40034,#40035,
#40036,#40037,#40038),(#40039,#40040,#40041,#40042,#40043,#40044,#40045,
#40046,#40047,#40048),(#40049,#40050,#40051,#40052,#40053,#40054,#40055,
#40056,#40057,#40058),(#40059,#40060,#40061,#40062,#40063,#40064,#40065,
#40066,#40067,#40068)),.UNSPECIFIED.,.F.,.F.,.F.)
B_SPLINE_SURFACE_WITH_KNOTS((4,4),(4,1,1,1,1,1,1,4),(0.0573683470670303,
0.942619239203189),(0.2949033483364,0.3467756743286,0.4093838918203,0.4700724725555,
0.5298509963668,0.5905363232075,0.6531416885286,0.7051372589503),
 .UNSPECIFIED.)
GEOMETRIC_REPRESENTATION_ITEM()
RATIONAL_B_SPLINE_SURFACE(((1.19355202165888,1.19355202165888,1.19355202165888,
1.19355202165888,1.19355202165888,1.19355202165888,1.19355202165888,1.19355202165888,
1.19355202165888,1.19355202165888),(0.935486278261233,0.935486278261233,
0.935486278261233,0.935486278261233,0.935486278261233,0.935486278261233,
0.935486278261233,0.935486278261233,0.935486278261233,0.935486278261233),
(0.935482659497885,0.935482659497885,0.935482659497885,0.935482659497885,
0.935482659497885,0.935482659497885,0.935482659497885,0.935482659497885,
0.935482659497885,0.935482659497885),(1.19354116536884,1.19354116536884,
1.19354116536884,1.19354116536884,1.19354116536884,1.19354116536884,1.19354116536884,
1.19354116536884,1.19354116536884,1.19354116536884)))
REPRESENTATION_ITEM('')
SURFACE()
);
#183=(
BOUNDED_SURFACE()
B_SPLINE_SURFACE(3,3,((#40177,#40178,#40179,#40180,#40181,#40182,#40183,
#40184,#40185),(#40186,#40187,#40188,#40189,#40190,#40191,#40192,#40193,
#40194),(#40195,#40196,#40197,#40198,#40199,#40200,#40201,#40202,#40203),
(#40204,#40205,#40206,#40207,#40208,#40209,#40210,#40211,#40212)),
 .UNSPECIFIED.,.F.,.F.,.F.)
B_SPLINE_SURFACE_WITH_KNOTS((4,4),(4,1,1,1,1,1,4),(0.054657385317252,0.945344116841943),
(0.225718740397496,0.2411747389778,0.3599582619165,0.4768206617321,0.5903023688696,
0.6994747309877,0.773103852050118),.UNSPECIFIED.)
GEOMETRIC_REPRESENTATION_ITEM()
RATIONAL_B_SPLINE_SURFACE(((1.19593460922364,1.19593460922364,1.19593460922364,
1.19593460922364,1.19593460922364,1.19593460922364,1.19593460922364,1.19593460922364,
1.19593460922364),(0.934688022994918,0.934688022994918,0.934688022994918,
0.934688022994918,0.934688022994918,0.934688022994918,0.934688022994918,
0.934688022994918,0.934688022994918),(0.934688463592728,0.934688463592728,
0.934688463592728,0.934688463592728,0.934688463592728,0.934688463592728,
0.934688463592728,0.934688463592728,0.934688463592728),(1.19593593101708,
1.19593593101708,1.19593593101708,1.19593593101708,1.19593593101708,1.19593593101708,
1.19593593101708,1.19593593101708,1.19593593101708)))
REPRESENTATION_ITEM('')
SURFACE()
);
#184=(
BOUNDED_SURFACE()
B_SPLINE_SURFACE(3,3,((#40329,#40330,#40331,#40332,#40333,#40334,#40335,
#40336,#40337,#40338),(#40339,#40340,#40341,#40342,#40343,#40344,#40345,
#40346,#40347,#40348),(#40349,#40350,#40351,#40352,#40353,#40354,#40355,
#40356,#40357,#40358),(#40359,#40360,#40361,#40362,#40363,#40364,#40365,
#40366,#40367,#40368)),.UNSPECIFIED.,.F.,.F.,.F.)
B_SPLINE_SURFACE_WITH_KNOTS((4,4),(4,1,1,1,1,1,1,4),(0.090214820579119,
0.903852852741469),(0.0113422875274,0.1428795028973,0.2858119560905,0.4286835352561,
0.5714929646109,0.7143131099677,0.8572933445083,0.9764111906646),
 .UNSPECIFIED.)
GEOMETRIC_REPRESENTATION_ITEM()
RATIONAL_B_SPLINE_SURFACE(((1.11548030902687,1.11548030902687,1.11548030902687,
1.11548030902687,1.11548030902687,1.11548030902687,1.11548030902687,1.11548030902687,
1.11548030902687,1.11548030902687),(0.962621077558573,0.962621077558573,
0.962621077558573,0.962621077558573,0.962621077558573,0.962621077558573,
0.962621077558573,0.962621077558573,0.962621077558573,0.962621077558573),
(0.961514630885325,0.961514630885325,0.961514630885325,0.961514630885325,
0.961514630885325,0.961514630885325,0.961514630885325,0.961514630885325,
0.961514630885325,0.961514630885325),(1.11216096900712,1.11216096900712,
1.11216096900712,1.11216096900712,1.11216096900712,1.11216096900712,1.11216096900712,
1.11216096900712,1.11216096900712,1.11216096900712)))
REPRESENTATION_ITEM('')
SURFACE()
);
#185=(
BOUNDED_SURFACE()
B_SPLINE_SURFACE(3,3,((#40395,#40396,#40397,#40398,#40399,#40400,#40401,
#40402,#40403),(#40404,#40405,#40406,#40407,#40408,#40409,#40410,#40411,
#40412),(#40413,#40414,#40415,#40416,#40417,#40418,#40419,#40420,#40421),
(#40422,#40423,#40424,#40425,#40426,#40427,#40428,#40429,#40430)),
 .UNSPECIFIED.,.F.,.F.,.F.)
B_SPLINE_SURFACE_WITH_KNOTS((4,4),(4,1,1,1,1,1,4),(0.054728297573913,0.945273202908356),
(0.226874247895751,0.300522254996,0.4096933649142,0.5231718563142,0.6400288266082,
0.7588043312258,0.774211492154076),.UNSPECIFIED.)
GEOMETRIC_REPRESENTATION_ITEM()
RATIONAL_B_SPLINE_SURFACE(((1.19587221360212,1.19587221360212,1.19587221360212,
1.19587221360212,1.19587221360212,1.19587221360212,1.19587221360212,1.19587221360212,
1.19587221360212),(0.934708822097536,0.934708822097536,0.934708822097536,
0.934708822097536,0.934708822097536,0.934708822097536,0.934708822097536,
0.934708822097536,0.934708822097536),(0.934709262133402,0.934709262133402,
0.934709262133402,0.934709262133402,0.934709262133402,0.934709262133402,
0.934709262133402,0.934709262133402,0.934709262133402),(1.19587353370972,
1.19587353370972,1.19587353370972,1.19587353370972,1.19587353370972,1.19587353370972,
1.19587353370972,1.19587353370972,1.19587353370972)))
REPRESENTATION_ITEM('')
SURFACE()
);
#186=(
BOUNDED_SURFACE()
B_SPLINE_SURFACE(3,3,((#40544,#40545,#40546,#40547,#40548,#40549,#40550,
#40551,#40552,#40553),(#40554,#40555,#40556,#40557,#40558,#40559,#40560,
#40561,#40562,#40563),(#40564,#40565,#40566,#40567,#40568,#40569,#40570,
#40571,#40572,#40573),(#40574,#40575,#40576,#40577,#40578,#40579,#40580,
#40581,#40582,#40583)),.UNSPECIFIED.,.F.,.F.,.F.)
B_SPLINE_SURFACE_WITH_KNOTS((4,4),(4,1,1,1,1,1,1,4),(0.0902463740384735,
0.903859594390682),(0.02358777781734,0.1427066554906,0.2856868900361,0.4285070354297,
0.5713164647035,0.7141880438182,0.8571204970713,0.9886565450757),
 .UNSPECIFIED.)
GEOMETRIC_REPRESENTATION_ITEM()
RATIONAL_B_SPLINE_SURFACE(((1.11546252682894,1.11546252682894,1.11546252682894,
1.11546252682894,1.11546252682894,1.11546252682894,1.11546252682894,1.11546252682894,
1.11546252682894,1.11546252682894),(0.962619725152993,0.962619725152993,
0.962619725152993,0.962619725152993,0.962619725152993,0.962619725152993,
0.962619725152993,0.962619725152993,0.962619725152993,0.962619725152993),
(0.961520454467663,0.961520454467663,0.961520454467663,0.961520454467663,
0.961520454467663,0.961520454467663,0.961520454467663,0.961520454467663,
0.961520454467663,0.961520454467663),(1.11216471477295,1.11216471477295,
1.11216471477295,1.11216471477295,1.11216471477295,1.11216471477295,1.11216471477295,
1.11216471477295,1.11216471477295,1.11216471477295)))
REPRESENTATION_ITEM('')
SURFACE()
);
#187=(
BOUNDED_SURFACE()
B_SPLINE_SURFACE(3,3,((#40623,#40624,#40625,#40626,#40627,#40628),(#40629,
#40630,#40631,#40632,#40633,#40634),(#40635,#40636,#40637,#40638,#40639,
#40640),(#40641,#40642,#40643,#40644,#40645,#40646)),.UNSPECIFIED.,.F.,
 .F.,.F.)
B_SPLINE_SURFACE_WITH_KNOTS((4,4),(4,1,1,4),(0.0986342191388958,0.901369959996773),
(0.317543733191685,0.3333147448852,0.6666852551147,0.682456266808859),
 .UNSPECIFIED.)
GEOMETRIC_REPRESENTATION_ITEM()
RATIONAL_B_SPLINE_SURFACE(((1.17563408853197,1.17563408853197,1.17563408853197,
1.17563408853197,1.17563408853197,1.17563408853197),(0.941454084654427,
0.941454084654427,0.941454084654428,0.941454084654428,0.941454084654428,
0.941454084654428),(0.941455303829123,0.941455303829123,0.941455303829123,
0.941455303829123,0.941455303829123,0.941455303829123),(1.17563774605606,
1.17563774605606,1.17563774605606,1.17563774605606,1.17563774605606,1.17563774605606)))
REPRESENTATION_ITEM('')
SURFACE()
);
#188=(
BOUNDED_SURFACE()
B_SPLINE_SURFACE(3,3,((#40886,#40887,#40888,#40889,#40890,#40891,#40892,
#40893,#40894,#40895,#40896,#40897,#40898,#40899,#40900,#40901,#40902,#40903,
#40904,#40905,#40906,#40907,#40908,#40909,#40910,#40911,#40912,#40913,#40914,
#40915,#40916,#40917,#40918,#40919,#40920,#40921,#40922,#40923,#40924,#40925),
(#40926,#40927,#40928,#40929,#40930,#40931,#40932,#40933,#40934,#40935,
#40936,#40937,#40938,#40939,#40940,#40941,#40942,#40943,#40944,#40945,#40946,
#40947,#40948,#40949,#40950,#40951,#40952,#40953,#40954,#40955,#40956,#40957,
#40958,#40959,#40960,#40961,#40962,#40963,#40964,#40965),(#40966,#40967,
#40968,#40969,#40970,#40971,#40972,#40973,#40974,#40975,#40976,#40977,#40978,
#40979,#40980,#40981,#40982,#40983,#40984,#40985,#40986,#40987,#40988,#40989,
#40990,#40991,#40992,#40993,#40994,#40995,#40996,#40997,#40998,#40999,#41000,
#41001,#41002,#41003,#41004,#41005),(#41006,#41007,#41008,#41009,#41010,
#41011,#41012,#41013,#41014,#41015,#41016,#41017,#41018,#41019,#41020,#41021,
#41022,#41023,#41024,#41025,#41026,#41027,#41028,#41029,#41030,#41031,#41032,
#41033,#41034,#41035,#41036,#41037,#41038,#41039,#41040,#41041,#41042,#41043,
#41044,#41045)),.UNSPECIFIED.,.F.,.F.,.F.)
B_SPLINE_SURFACE_WITH_KNOTS((4,4),(4,1,1,1,1,1,1,1,1,1,1,1,1,1,1,1,1,1,
1,1,1,1,1,1,1,1,1,1,1,1,1,1,1,1,1,1,1,4),(0.109557713609705,0.885247213323687),
(-0.009601789269793,0.,0.02232800254047,0.04690499692097,0.07379314494475,
0.1032825879248,0.1358147775015,0.1719129911135,0.2120208291974,0.2562559556703,
0.3048272129563,0.3583973876345,0.4161404010308,0.4734162974592,0.526583520073,
0.5739184110835,0.6155189332402,0.6529905554197,0.6871367384821,0.7180197388927,
0.7460319790749,0.7715260585384,0.7947388244259,0.8158370649057,0.8349859745155,
0.852358315218,0.8681369543747,0.882501434184,0.895628780335,0.9076949488169,
0.9188453219145,0.9291452487614,0.9386433394322,0.9473861202751,0.9554257888082,
0.9628157674929,0.9696063892784,0.9720662895839),.UNSPECIFIED.)
GEOMETRIC_REPRESENTATION_ITEM()
RATIONAL_B_SPLINE_SURFACE(((1.07369786616139,1.07369786616139,1.07369786616139,
1.07369786616139,1.07369786616139,1.07369786616139,1.07369786616139,1.07369786616139,
1.07369786616139,1.07369786616139,1.07369786616139,1.07369786616139,1.07369786616139,
1.07369786616139,1.07369786616139,1.07369786616139,1.07369786616139,1.07369786616139,
1.07369786616139,1.07369786616139,1.07369786616139,1.07369786616139,1.07369786616139,
1.07369786616139,1.07369786616139,1.07369786616139,1.07369786616139,1.07369786616139,
1.07369786616139,1.07369786616139,1.07369786616139,1.07369786616139,1.07369786616139,
1.07369786616139,1.07369786616139,1.07369786616139,1.07369786616139,1.07369786616139,
1.07369786616139,1.07369786616139),(0.976087774690969,0.976087774690969,
0.976087774690969,0.976087774690969,0.976087774690969,0.976087774690969,
0.976087774690969,0.976087774690969,0.976087774690969,0.976087774690969,
0.976087774690969,0.976087774690969,0.976087774690969,0.976087774690969,
0.976087774690969,0.976087774690969,0.976087774690969,0.976087774690969,
0.976087774690969,0.976087774690969,0.976087774690969,0.976087774690969,
0.976087774690969,0.976087774690969,0.976087774690969,0.976087774690969,
0.976087774690969,0.976087774690969,0.976087774690969,0.976087774690969,
0.976087774690969,0.976087774690969,0.976087774690969,0.976087774690969,
0.976087774690969,0.976087774690969,0.976087774690969,0.976087774690969,
0.976087774690969,0.976087774690969),(0.975438393751835,0.975438393751835,
0.975438393751835,0.975438393751835,0.975438393751835,0.975438393751835,
0.975438393751835,0.975438393751835,0.975438393751835,0.975438393751835,
0.975438393751835,0.975438393751835,0.975438393751835,0.975438393751835,
0.975438393751835,0.975438393751835,0.975438393751835,0.975438393751835,
0.975438393751835,0.975438393751835,0.975438393751835,0.975438393751835,
0.975438393751835,0.975438393751835,0.975438393751835,0.975438393751835,
0.975438393751835,0.975438393751835,0.975438393751835,0.975438393751835,
0.975438393751835,0.975438393751835,0.975438393751835,0.975438393751835,
0.975438393751835,0.975438393751835,0.975438393751835,0.975438393751835,
0.975438393751835,0.975438393751835),(1.07174972334399,1.07174972334399,
1.07174972334399,1.07174972334399,1.07174972334399,1.07174972334399,1.07174972334399,
1.07174972334399,1.07174972334399,1.07174972334399,1.07174972334399,1.07174972334399,
1.07174972334399,1.07174972334399,1.07174972334399,1.07174972334399,1.07174972334399,
1.07174972334399,1.07174972334399,1.07174972334399,1.07174972334399,1.07174972334399,
1.07174972334399,1.07174972334399,1.07174972334399,1.07174972334399,1.07174972334399,
1.07174972334399,1.07174972334399,1.07174972334399,1.07174972334399,1.07174972334399,
1.07174972334399,1.07174972334399,1.07174972334399,1.07174972334399,1.07174972334399,
1.07174972334399,1.07174972334399,1.07174972334399)))
REPRESENTATION_ITEM('')
SURFACE()
);
#189=(
BOUNDED_SURFACE()
B_SPLINE_SURFACE(3,3,((#41171,#41172,#41173,#41174,#41175,#41176,#41177,
#41178,#41179),(#41180,#41181,#41182,#41183,#41184,#41185,#41186,#41187,
#41188),(#41189,#41190,#41191,#41192,#41193,#41194,#41195,#41196,#41197),
(#41198,#41199,#41200,#41201,#41202,#41203,#41204,#41205,#41206)),
 .UNSPECIFIED.,.F.,.F.,.F.)
B_SPLINE_SURFACE_WITH_KNOTS((4,4),(4,1,1,1,1,1,4),(0.0545876560709944,0.945414163178399),
(0.227019637278718,0.2408830109945,0.3597029788423,0.4766081773209,0.5901375306023,
0.6993568121791,0.77342322572),.UNSPECIFIED.)
GEOMETRIC_REPRESENTATION_ITEM()
RATIONAL_B_SPLINE_SURFACE(((1.19599641219284,1.19599641219284,1.19599641219284,
1.19599641219284,1.19599641219284,1.19599641219284,1.19599641219284,1.19599641219284,
1.19599641219284),(0.934667328915005,0.934667328915005,0.934667328915005,
0.934667328915005,0.934667328915005,0.934667328915005,0.934667328915005,
0.934667328915005,0.934667328915006),(0.934667862603376,0.934667862603376,
0.934667862603376,0.934667862603376,0.934667862603376,0.934667862603376,
0.934667862603376,0.934667862603376,0.934667862603376),(1.19599801325795,
1.19599801325795,1.19599801325795,1.19599801325795,1.19599801325795,1.19599801325795,
1.19599801325795,1.19599801325795,1.19599801325795)))
REPRESENTATION_ITEM('')
SURFACE()
);
#190=(
BOUNDED_SURFACE()
B_SPLINE_SURFACE(3,3,((#41329,#41330,#41331,#41332,#41333,#41334,#41335,
#41336,#41337,#41338),(#41339,#41340,#41341,#41342,#41343,#41344,#41345,
#41346,#41347,#41348),(#41349,#41350,#41351,#41352,#41353,#41354,#41355,
#41356,#41357,#41358),(#41359,#41360,#41361,#41362,#41363,#41364,#41365,
#41366,#41367,#41368)),.UNSPECIFIED.,.F.,.F.,.F.)
B_SPLINE_SURFACE_WITH_KNOTS((4,4),(4,1,1,1,1,1,1,4),(0.0897026986543284,
0.903562378195111),(0.02295305876099,0.1427319370604,0.2857219203474,0.4285792797614,
0.5713515650105,0.7142098207389,0.8572808214069,0.9622634165798),
 .UNSPECIFIED.)
GEOMETRIC_REPRESENTATION_ITEM()
RATIONAL_B_SPLINE_SURFACE(((1.11534309355231,1.11534309355231,1.11534309355231,
1.11534309355231,1.11534309355231,1.11534309355231,1.11534309355231,1.11534309355231,
1.11534309355231,1.11534309355231),(0.962814520006825,0.962814520006825,
0.962814520006825,0.962814520006825,0.962814520006825,0.962814520006825,
0.962814520006825,0.962814520006825,0.962814520006825,0.962814520006825),
(0.961562661637633,0.961562661637633,0.961562661637633,0.961562661637633,
0.961562661637633,0.961562661637633,0.961562661637633,0.961562661637633,
0.961562661637633,0.961562661637633),(1.11158751844473,1.11158751844473,
1.11158751844473,1.11158751844473,1.11158751844473,1.11158751844473,1.11158751844473,
1.11158751844473,1.11158751844473,1.11158751844473)))
REPRESENTATION_ITEM('')
SURFACE()
);
#191=(
BOUNDED_SURFACE()
B_SPLINE_SURFACE(3,3,((#41587,#41588,#41589,#41590,#41591,#41592,#41593,
#41594,#41595,#41596),(#41597,#41598,#41599,#41600,#41601,#41602,#41603,
#41604,#41605,#41606),(#41607,#41608,#41609,#41610,#41611,#41612,#41613,
#41614,#41615,#41616),(#41617,#41618,#41619,#41620,#41621,#41622,#41623,
#41624,#41625,#41626)),.UNSPECIFIED.,.F.,.F.,.F.)
B_SPLINE_SURFACE_WITH_KNOTS((4,4),(4,1,1,1,1,1,1,4),(0.0573528854689029,
0.942634096168851),(0.2948654053633,0.3479036645395,0.4101463286025,0.4703448613228,
0.5297234926217,0.5899248652657,0.6521709850243,0.7051026564205),
 .UNSPECIFIED.)
GEOMETRIC_REPRESENTATION_ITEM()
RATIONAL_B_SPLINE_SURFACE(((1.19356575363168,1.19356575363168,1.19356575363168,
1.19356575363168,1.19356575363168,1.19356575363168,1.19356575363168,1.19356575363168,
1.19356575363168,1.19356575363168),(0.935481877334427,0.935481877334427,
0.935481877334427,0.935481877334427,0.935481877334427,0.935481877334427,
0.935481877334427,0.935481877334427,0.935481877334427,0.935481877334427),
(0.935478082178781,0.935478082178781,0.935478082178781,0.935478082178781,
0.935478082178781,0.935478082178781,0.935478082178781,0.935478082178781,
0.935478082178781,0.935478082178781),(1.19355436816475,1.19355436816475,
1.19355436816475,1.19355436816475,1.19355436816475,1.19355436816475,1.19355436816475,
1.19355436816475,1.19355436816475,1.19355436816475)))
REPRESENTATION_ITEM('')
SURFACE()
);
#192=(
BOUNDED_SURFACE()
B_SPLINE_SURFACE(3,3,((#41733,#41734,#41735,#41736,#41737,#41738,#41739,
#41740,#41741),(#41742,#41743,#41744,#41745,#41746,#41747,#41748,#41749,
#41750),(#41751,#41752,#41753,#41754,#41755,#41756,#41757,#41758,#41759),
(#41760,#41761,#41762,#41763,#41764,#41765,#41766,#41767,#41768)),
 .UNSPECIFIED.,.F.,.F.,.F.)
B_SPLINE_SURFACE_WITH_KNOTS((4,4),(4,1,1,1,1,1,4),(0.0545525345384962,0.945448460040463),
(0.226579630138955,0.3004022999601,0.4096207676398,0.5231927024745,0.6401765809238,
0.7590171413674,0.773021471035039),.UNSPECIFIED.)
GEOMETRIC_REPRESENTATION_ITEM()
RATIONAL_B_SPLINE_SURFACE(((1.19602600408056,1.19602600408056,1.19602600408056,
1.19602600408056,1.19602600408056,1.19602600408056,1.19602600408056,1.19602600408056,
1.19602600408056),(0.934657706853242,0.934657706853242,0.934657706853242,
0.934657706853242,0.934657706853242,0.934657706853242,0.934657706853242,
0.934657706853242,0.934657706853242),(0.934657998640073,0.934657998640073,
0.934657998640073,0.934657998640073,0.934657998640073,0.934657998640073,
0.934657998640073,0.934657998640073,0.934657998640073),(1.19602687944105,
1.19602687944105,1.19602687944105,1.19602687944105,1.19602687944105,1.19602687944105,
1.19602687944105,1.19602687944105,1.19602687944105)))
REPRESENTATION_ITEM('')
SURFACE()
);
#193=(
BOUNDED_SURFACE()
B_SPLINE_SURFACE(3,3,((#41879,#41880,#41881,#41882,#41883,#41884,#41885,
#41886,#41887,#41888,#41889),(#41890,#41891,#41892,#41893,#41894,#41895,
#41896,#41897,#41898,#41899,#41900),(#41901,#41902,#41903,#41904,#41905,
#41906,#41907,#41908,#41909,#41910,#41911),(#41912,#41913,#41914,#41915,
#41916,#41917,#41918,#41919,#41920,#41921,#41922)),.UNSPECIFIED.,.F.,.F.,
 .F.)
B_SPLINE_SURFACE_WITH_KNOTS((4,4),(4,1,1,1,1,1,1,1,4),(0.0753633925526522,
0.903551965100841),(-0.009670337421388,0.,0.1430991485311,0.2858285059199,
0.4284781713031,0.5715215149008,0.7145472299923,0.8573672624017,0.9759160460961),
 .UNSPECIFIED.)
GEOMETRIC_REPRESENTATION_ITEM()
RATIONAL_B_SPLINE_SURFACE(((1.12354604891087,1.12354604891087,1.12354604891087,
1.12354604891087,1.12354604891087,1.12354604891087,1.12354604891087,1.12354604891087,
1.12354604891087,1.12354604891087,1.12354604891087),(0.962907636211588,
0.962907636211588,0.962907636211588,0.962907636211588,0.962907636211588,
0.962907636211588,0.962907636211588,0.962907636211588,0.962907636211588,
0.962907636211588,0.962907636211588),(0.958919516229146,0.958919516229146,
0.958919516229146,0.958919516229146,0.958919516229146,0.958919516229146,
0.958919516229146,0.958919516229146,0.958919516229146,0.958919516229146,
0.958919516229146),(1.11158168896355,1.11158168896355,1.11158168896355,
1.11158168896355,1.11158168896355,1.11158168896355,1.11158168896355,1.11158168896355,
1.11158168896355,1.11158168896355,1.11158168896355)))
REPRESENTATION_ITEM('')
SURFACE()
);
#194=(
BOUNDED_SURFACE()
B_SPLINE_SURFACE(3,3,((#42039,#42040,#42041,#42042),(#42043,#42044,#42045,
#42046),(#42047,#42048,#42049,#42050),(#42051,#42052,#42053,#42054)),
 .UNSPECIFIED.,.F.,.F.,.F.)
B_SPLINE_SURFACE_WITH_KNOTS((4,4),(4,4),(0.0986320320018917,0.901362552765544),
(-0.975145040392605,-0.0991746183702489),.UNSPECIFIED.)
GEOMETRIC_REPRESENTATION_ITEM()
RATIONAL_B_SPLINE_SURFACE(((1.17563600436037,1.17563600436037,1.17563600436037,
1.17563600436037),(0.941456244993406,0.941456244993406,0.941456244993406,
0.941456244993406),(0.941454665223768,0.941454665223768,0.941454665223768,
0.941454665223768),(1.17563126505145,1.17563126505145,1.17563126505145,
1.17563126505145)))
REPRESENTATION_ITEM('')
SURFACE()
);
#195=(
BOUNDED_SURFACE()
B_SPLINE_SURFACE(3,3,((#42073,#42074,#42075,#42076,#42077,#42078,#42079,
#42080,#42081,#42082,#42083,#42084,#42085,#42086,#42087,#42088,#42089,#42090,
#42091,#42092,#42093,#42094,#42095,#42096,#42097,#42098,#42099,#42100,#42101,
#42102,#42103,#42104,#42105),(#42106,#42107,#42108,#42109,#42110,#42111,
#42112,#42113,#42114,#42115,#42116,#42117,#42118,#42119,#42120,#42121,#42122,
#42123,#42124,#42125,#42126,#42127,#42128,#42129,#42130,#42131,#42132,#42133,
#42134,#42135,#42136,#42137,#42138),(#42139,#42140,#42141,#42142,#42143,
#42144,#42145,#42146,#42147,#42148,#42149,#42150,#42151,#42152,#42153,#42154,
#42155,#42156,#42157,#42158,#42159,#42160,#42161,#42162,#42163,#42164,#42165,
#42166,#42167,#42168,#42169,#42170,#42171),(#42172,#42173,#42174,#42175,
#42176,#42177,#42178,#42179,#42180,#42181,#42182,#42183,#42184,#42185,#42186,
#42187,#42188,#42189,#42190,#42191,#42192,#42193,#42194,#42195,#42196,#42197,
#42198,#42199,#42200,#42201,#42202,#42203,#42204)),.UNSPECIFIED.,.F.,.F.,
 .F.)
B_SPLINE_SURFACE_WITH_KNOTS((4,4),(4,1,1,1,1,1,1,1,1,1,1,1,1,1,1,1,1,1,
1,1,1,1,1,1,1,1,1,1,1,1,4),(0.108378650171574,0.903586235863032),(-0.009736901743296,
0.,0.02218413179576,0.04656961109638,0.07320227077888,0.1023246073713,0.1343070073107,
0.1695983831343,0.2086113444874,0.2515282384527,0.2985700177486,0.350328036692,
0.4076667288658,0.4682132326039,0.528225646619,0.5849768379219,0.6367767624475,
0.6825350754174,0.7235069669497,0.7605071950811,0.7940293660298,0.8241786597893,
0.8510660708028,0.8750221728291,0.8964633607905,0.9157954007781,0.9333737553394,
0.9493579414419,0.963858565732,0.9770543416123,0.985715500525),
 .UNSPECIFIED.)
GEOMETRIC_REPRESENTATION_ITEM()
RATIONAL_B_SPLINE_SURFACE(((1.07414501665385,1.07414501665385,1.07414501665385,
1.07414501665385,1.07414501665385,1.07414501665385,1.07414501665385,1.07414501665385,
1.07414501665385,1.07414501665385,1.07414501665385,1.07414501665385,1.07414501665385,
1.07414501665385,1.07414501665385,1.07414501665385,1.07414501665385,1.07414501665385,
1.07414501665385,1.07414501665385,1.07414501665385,1.07414501665385,1.07414501665385,
1.07414501665385,1.07414501665385,1.07414501665385,1.07414501665385,1.07414501665385,
1.07414501665385,1.07414501665385,1.07414501665385,1.07414501665385,1.07414501665385),
(0.973774799844115,0.973774799844115,0.973774799844115,0.973774799844115,
0.973774799844115,0.973774799844115,0.973774799844115,0.973774799844115,
0.973774799844115,0.973774799844115,0.973774799844115,0.973774799844115,
0.973774799844115,0.973774799844115,0.973774799844115,0.973774799844115,
0.973774799844115,0.973774799844115,0.973774799844115,0.973774799844115,
0.973774799844115,0.973774799844115,0.973774799844115,0.973774799844115,
0.973774799844115,0.973774799844115,0.973774799844115,0.973774799844115,
0.973774799844115,0.973774799844115,0.973774799844115,0.973774799844115,
0.973774799844115),(0.975308064317468,0.975308064317468,0.975308064317468,
0.975308064317468,0.975308064317468,0.975308064317468,0.975308064317468,
0.975308064317468,0.975308064317468,0.975308064317468,0.975308064317468,
0.975308064317468,0.975308064317468,0.975308064317468,0.975308064317468,
0.975308064317468,0.975308064317468,0.975308064317468,0.975308064317468,
0.975308064317468,0.975308064317468,0.975308064317468,0.975308064317468,
0.975308064317468,0.975308064317468,0.975308064317468,0.975308064317468,
0.975308064317468,0.975308064317468,0.975308064317468,0.975308064317468,
0.975308064317468,0.975308064317468),(1.07874481007391,1.07874481007391,
1.07874481007391,1.07874481007391,1.07874481007391,1.07874481007391,1.07874481007391,
1.07874481007391,1.07874481007391,1.07874481007391,1.07874481007391,1.07874481007391,
1.07874481007391,1.07874481007391,1.07874481007391,1.07874481007391,1.07874481007391,
1.07874481007391,1.07874481007391,1.07874481007391,1.07874481007391,1.07874481007391,
1.07874481007391,1.07874481007391,1.07874481007391,1.07874481007391,1.07874481007391,
1.07874481007391,1.07874481007391,1.07874481007391,1.07874481007391,1.07874481007391,
1.07874481007391)))
REPRESENTATION_ITEM('')
SURFACE()
);
#196=(
BOUNDED_SURFACE()
B_SPLINE_SURFACE(3,3,((#42590,#42591,#42592,#42593,#42594,#42595,#42596,
#42597,#42598,#42599,#42600),(#42601,#42602,#42603,#42604,#42605,#42606,
#42607,#42608,#42609,#42610,#42611),(#42612,#42613,#42614,#42615,#42616,
#42617,#42618,#42619,#42620,#42621,#42622),(#42623,#42624,#42625,#42626,
#42627,#42628,#42629,#42630,#42631,#42632,#42633)),.UNSPECIFIED.,.F.,.F.,
 .F.)
B_SPLINE_SURFACE_WITH_KNOTS((4,4),(4,1,1,1,1,1,1,1,4),(0.0573248939826349,
0.942652782085426),(0.294899609167,0.3228689298849,0.3831046509521,0.4422669195799,
0.4999589566113,0.5576491953134,0.6168076022616,0.6770470459264,0.7051410016013),
 .UNSPECIFIED.)
GEOMETRIC_REPRESENTATION_ITEM()
RATIONAL_B_SPLINE_SURFACE(((1.19358809665843,1.19358809665843,1.19358809665843,
1.19358809665843,1.19358809665843,1.19358809665843,1.19358809665843,1.19358809665843,
1.19358809665843,1.19358809665843,1.19358809665843),(0.935477142828405,
0.935477142828405,0.935477142828405,0.935477142828405,0.935477142828405,
0.935477142828405,0.935477142828405,0.935477142828405,0.935477142828405,
0.935477142828405,0.935477142828405),(0.935470634611331,0.935470634611331,
0.935470634611331,0.935470634611331,0.935470634611331,0.935470634611331,
0.935470634611331,0.935470634611331,0.935470634611331,0.935470634611331,
0.935470634611331),(1.19356857200721,1.19356857200721,1.19356857200721,
1.19356857200721,1.19356857200721,1.19356857200721,1.19356857200721,1.19356857200721,
1.19356857200721,1.19356857200721,1.19356857200721)))
REPRESENTATION_ITEM('')
SURFACE()
);
#197=(
BOUNDED_SURFACE()
B_SPLINE_SURFACE(3,3,((#42718,#42719,#42720,#42721,#42722,#42723,#42724,
#42725,#42726),(#42727,#42728,#42729,#42730,#42731,#42732,#42733,#42734,
#42735),(#42736,#42737,#42738,#42739,#42740,#42741,#42742,#42743,#42744),
(#42745,#42746,#42747,#42748,#42749,#42750,#42751,#42752,#42753)),
 .UNSPECIFIED.,.F.,.F.,.F.)
B_SPLINE_SURFACE_WITH_KNOTS((4,4),(4,1,1,1,1,1,4),(0.0546312169533823,0.945370286804514),
(0.225683109986944,0.2412765766488,0.3600743765287,0.4770048853175,0.5905230256156,
0.6996938806735,0.773232633815288),.UNSPECIFIED.)
GEOMETRIC_REPRESENTATION_ITEM()
RATIONAL_B_SPLINE_SURFACE(((1.19595763086821,1.19595763086821,1.19595763086821,
1.19595763086821,1.19595763086821,1.19595763086821,1.19595763086821,1.19595763086821,
1.19595763086821),(0.934680348618612,0.934680348618612,0.934680348618612,
0.934680348618612,0.934680348618612,0.934680348618612,0.934680348618612,
0.934680348618612,0.934680348618612),(0.934680789711243,0.934680789711243,
0.934680789711243,0.934680789711243,0.934680789711243,0.934680789711243,
0.934680789711243,0.934680789711243,0.934680789711243),(1.1959589541461,
1.1959589541461,1.1959589541461,1.1959589541461,1.1959589541461,1.1959589541461,
1.1959589541461,1.1959589541461,1.1959589541461)))
REPRESENTATION_ITEM('')
SURFACE()
);
#198=(
BOUNDED_SURFACE()
B_SPLINE_SURFACE(3,3,((#42867,#42868,#42869,#42870,#42871,#42872,#42873,
#42874,#42875,#42876),(#42877,#42878,#42879,#42880,#42881,#42882,#42883,
#42884,#42885,#42886),(#42887,#42888,#42889,#42890,#42891,#42892,#42893,
#42894,#42895,#42896),(#42897,#42898,#42899,#42900,#42901,#42902,#42903,
#42904,#42905,#42906)),.UNSPECIFIED.,.F.,.F.,.F.)
B_SPLINE_SURFACE_WITH_KNOTS((4,4),(4,1,1,1,1,1,1,4),(0.0902162146474901,
0.90384766932744),(0.01134228752741,0.1428795028254,0.2858119558808,0.4286835351635,
0.5714929647039,0.7143131099766,0.8572933445059,0.9764111906646),
 .UNSPECIFIED.)
GEOMETRIC_REPRESENTATION_ITEM()
RATIONAL_B_SPLINE_SURFACE(((1.11547952330921,1.11547952330921,1.11547952330921,
1.11547952330921,1.11547952330921,1.11547952330921,1.11547952330921,1.11547952330921,
1.11547952330921,1.11547952330921),(0.962622047579736,0.962622047579736,
0.962622047579736,0.962622047579736,0.962622047579736,0.962622047579736,
0.962622047579736,0.962622047579736,0.962622047579736,0.962622047579736),
(0.961514903100546,0.961514903100546,0.961514903100546,0.961514903100546,
0.961514903100546,0.961514903100546,0.961514903100546,0.961514903100546,
0.961514903100546,0.961514903100546),(1.11215808987164,1.11215808987164,
1.11215808987164,1.11215808987164,1.11215808987164,1.11215808987164,1.11215808987164,
1.11215808987164,1.11215808987164,1.11215808987164)))
REPRESENTATION_ITEM('')
SURFACE()
);
#199=(
BOUNDED_SURFACE()
B_SPLINE_SURFACE(3,3,((#42933,#42934,#42935,#42936,#42937,#42938,#42939,
#42940,#42941),(#42942,#42943,#42944,#42945,#42946,#42947,#42948,#42949,
#42950),(#42951,#42952,#42953,#42954,#42955,#42956,#42957,#42958,#42959),
(#42960,#42961,#42962,#42963,#42964,#42965,#42966,#42967,#42968)),
 .UNSPECIFIED.,.F.,.F.,.F.)
B_SPLINE_SURFACE_WITH_KNOTS((4,4),(4,1,1,1,1,1,4),(0.0547193706907307,0.94528212979141),
(0.226873519265384,0.300522254996,0.4096933649141,0.5231718563141,0.6400288266082,
0.7588043312258,0.774220135722599),.UNSPECIFIED.)
GEOMETRIC_REPRESENTATION_ITEM()
RATIONAL_B_SPLINE_SURFACE(((1.19588006744166,1.19588006744166,1.19588006744166,
1.19588006744166,1.19588006744166,1.19588006744166,1.19588006744166,1.19588006744166,
1.19588006744166),(0.934706204142303,0.934706204142303,0.934706204142303,
0.934706204142303,0.934706204142303,0.934706204142303,0.934706204142303,
0.934706204142303,0.934706204142303),(0.934706644186953,0.934706644186953,
0.934706644186953,0.934706644186953,0.934706644186953,0.934706644186953,
0.934706644186953,0.934706644186953,0.934706644186953),(1.19588138757561,
1.19588138757561,1.19588138757561,1.19588138757561,1.19588138757561,1.19588138757561,
1.19588138757561,1.19588138757561,1.19588138757561)))
REPRESENTATION_ITEM('')
SURFACE()
);
#200=(
BOUNDED_SURFACE()
B_SPLINE_SURFACE(3,3,((#43082,#43083,#43084,#43085,#43086,#43087,#43088,
#43089,#43090,#43091),(#43092,#43093,#43094,#43095,#43096,#43097,#43098,
#43099,#43100,#43101),(#43102,#43103,#43104,#43105,#43106,#43107,#43108,
#43109,#43110,#43111),(#43112,#43113,#43114,#43115,#43116,#43117,#43118,
#43119,#43120,#43121)),.UNSPECIFIED.,.F.,.F.,.F.)
B_SPLINE_SURFACE_WITH_KNOTS((4,4),(4,1,1,1,1,1,1,4),(0.0902477372797298,
0.903859553668012),(0.02358777781735,0.1427066554932,0.2856868900266,0.4285070353299,
0.5713164648028,0.714188044043,0.8571204971484,0.9886565450757),
 .UNSPECIFIED.)
GEOMETRIC_REPRESENTATION_ITEM()
RATIONAL_B_SPLINE_SURFACE(((1.11546175854762,1.11546175854762,1.11546175854762,
1.11546175854762,1.11546175854762,1.11546175854762,1.11546175854762,1.11546175854762,
1.11546175854762,1.11546175854762),(0.962619729119499,0.962619729119499,
0.962619729119499,0.962619729119499,0.962619729119499,0.962619729119499,
0.962619729119499,0.962619729119499,0.962619729119499,0.962619729119499),
(0.961520706987935,0.961520706987935,0.961520706987935,0.961520706987935,
0.961520706987935,0.961520706987935,0.961520706987935,0.961520706987935,
0.961520706987935,0.961520706987935),(1.11216469215293,1.11216469215293,
1.11216469215293,1.11216469215293,1.11216469215293,1.11216469215293,1.11216469215293,
1.11216469215293,1.11216469215293,1.11216469215293)))
REPRESENTATION_ITEM('')
SURFACE()
);
#201=(
BOUNDED_SURFACE()
B_SPLINE_SURFACE(3,3,((#43161,#43162,#43163,#43164,#43165,#43166),(#43167,
#43168,#43169,#43170,#43171,#43172),(#43173,#43174,#43175,#43176,#43177,
#43178),(#43179,#43180,#43181,#43182,#43183,#43184)),.UNSPECIFIED.,.F.,
 .F.,.F.)
B_SPLINE_SURFACE_WITH_KNOTS((4,4),(4,1,1,4),(0.0986342191388437,0.901369960096874),
(0.317543733191054,0.3333147448853,0.6666852551148,0.682456266810123),
 .UNSPECIFIED.)
GEOMETRIC_REPRESENTATION_ITEM()
RATIONAL_B_SPLINE_SURFACE(((1.17563408853202,1.17563408853202,1.17563408853202,
1.17563408853202,1.17563408853202,1.17563408853202),(0.941454084625226,
0.941454084625226,0.941454084625226,0.941454084625226,0.941454084625226,
0.941454084625226),(0.941455303829108,0.941455303829108,0.941455303829108,
0.941455303829108,0.941455303829108,0.941455303829108),(1.17563774614367,
1.17563774614367,1.17563774614367,1.17563774614367,1.17563774614367,1.17563774614367)))
REPRESENTATION_ITEM('')
SURFACE()
);
#202=(
BOUNDED_SURFACE()
B_SPLINE_SURFACE(3,3,((#43424,#43425,#43426,#43427,#43428,#43429,#43430,
#43431,#43432,#43433,#43434,#43435,#43436,#43437,#43438,#43439,#43440,#43441,
#43442,#43443,#43444,#43445,#43446,#43447,#43448,#43449,#43450,#43451,#43452,
#43453,#43454,#43455,#43456,#43457,#43458,#43459,#43460,#43461,#43462,#43463),
(#43464,#43465,#43466,#43467,#43468,#43469,#43470,#43471,#43472,#43473,
#43474,#43475,#43476,#43477,#43478,#43479,#43480,#43481,#43482,#43483,#43484,
#43485,#43486,#43487,#43488,#43489,#43490,#43491,#43492,#43493,#43494,#43495,
#43496,#43497,#43498,#43499,#43500,#43501,#43502,#43503),(#43504,#43505,
#43506,#43507,#43508,#43509,#43510,#43511,#43512,#43513,#43514,#43515,#43516,
#43517,#43518,#43519,#43520,#43521,#43522,#43523,#43524,#43525,#43526,#43527,
#43528,#43529,#43530,#43531,#43532,#43533,#43534,#43535,#43536,#43537,#43538,
#43539,#43540,#43541,#43542,#43543),(#43544,#43545,#43546,#43547,#43548,
#43549,#43550,#43551,#43552,#43553,#43554,#43555,#43556,#43557,#43558,#43559,
#43560,#43561,#43562,#43563,#43564,#43565,#43566,#43567,#43568,#43569,#43570,
#43571,#43572,#43573,#43574,#43575,#43576,#43577,#43578,#43579,#43580,#43581,
#43582,#43583)),.UNSPECIFIED.,.F.,.F.,.F.)
B_SPLINE_SURFACE_WITH_KNOTS((4,4),(4,1,1,1,1,1,1,1,1,1,1,1,1,1,1,1,1,1,
1,1,1,1,1,1,1,1,1,1,1,1,1,1,1,1,1,1,1,4),(0.109557623003378,0.885243870225913),
(-0.009601789273473,0.,0.02232833549656,0.04690550208439,0.07379362467687,
0.1032829469298,0.1358149659673,0.1719129604547,0.2120204765667,0.2562549558966,
0.3048250014041,0.3583933178769,0.4161357109095,0.4734125795377,0.5265814299997,
0.5739176940639,0.6155190247053,0.6529911923141,0.6871377766586,0.7180210170724,
0.7460333746103,0.7715274743231,0.7947401813888,0.8158383097167,0.8349870800806,
0.8523592732021,0.86813775977,0.8825020836395,0.8956292723195,0.9076952836912,
0.9188455009779,0.9291452784589,0.9386432333899,0.9473858993638,0.9554254804025,
0.9628154053197,0.9696060115487,0.972066289616),.UNSPECIFIED.)
GEOMETRIC_REPRESENTATION_ITEM()
RATIONAL_B_SPLINE_SURFACE(((1.07369790036373,1.07369790036373,1.07369790036373,
1.07369790036373,1.07369790036373,1.07369790036373,1.07369790036373,1.07369790036373,
1.07369790036373,1.07369790036373,1.07369790036373,1.07369790036373,1.07369790036373,
1.07369790036373,1.07369790036373,1.07369790036373,1.07369790036373,1.07369790036373,
1.07369790036373,1.07369790036373,1.07369790036373,1.07369790036373,1.07369790036373,
1.07369790036373,1.07369790036373,1.07369790036373,1.07369790036373,1.07369790036373,
1.07369790036373,1.07369790036373,1.07369790036373,1.07369790036373,1.07369790036373,
1.07369790036373,1.07369790036373,1.07369790036373,1.07369790036373,1.07369790036373,
1.07369790036373,1.07369790036373),(0.976088195527518,0.976088195527518,
0.976088195527518,0.976088195527518,0.976088195527518,0.976088195527518,
0.976088195527518,0.976088195527518,0.976088195527518,0.976088195527518,
0.976088195527518,0.976088195527518,0.976088195527518,0.976088195527518,
0.976088195527518,0.976088195527518,0.976088195527518,0.976088195527518,
0.976088195527518,0.976088195527518,0.976088195527518,0.976088195527518,
0.976088195527518,0.976088195527518,0.976088195527518,0.976088195527518,
0.976088195527518,0.976088195527518,0.976088195527518,0.976088195527518,
0.976088195527518,0.976088195527518,0.976088195527518,0.976088195527518,
0.976088195527518,0.976088195527518,0.976088195527518,0.976088195527518,
0.976088195527518,0.976088195527518),(0.97543838810218,0.97543838810218,
0.97543838810218,0.97543838810218,0.97543838810218,0.97543838810218,0.97543838810218,
0.97543838810218,0.97543838810218,0.97543838810218,0.97543838810218,0.97543838810218,
0.97543838810218,0.97543838810218,0.97543838810218,0.97543838810218,0.97543838810218,
0.97543838810218,0.97543838810218,0.97543838810218,0.97543838810218,0.97543838810218,
0.97543838810218,0.97543838810218,0.97543838810218,0.97543838810218,0.97543838810218,
0.97543838810218,0.97543838810218,0.97543838810218,0.97543838810218,0.97543838810218,
0.97543838810218,0.97543838810218,0.97543838810218,0.97543838810218,0.97543838810218,
0.97543838810218,0.97543838810218,0.97543838810218),(1.07174847808772,1.07174847808772,
1.07174847808772,1.07174847808772,1.07174847808772,1.07174847808772,1.07174847808772,
1.07174847808772,1.07174847808772,1.07174847808772,1.07174847808772,1.07174847808772,
1.07174847808772,1.07174847808772,1.07174847808772,1.07174847808772,1.07174847808772,
1.07174847808772,1.07174847808772,1.07174847808772,1.07174847808772,1.07174847808772,
1.07174847808772,1.07174847808772,1.07174847808772,1.07174847808772,1.07174847808772,
1.07174847808772,1.07174847808772,1.07174847808772,1.07174847808772,1.07174847808772,
1.07174847808772,1.07174847808772,1.07174847808772,1.07174847808772,1.07174847808772,
1.07174847808772,1.07174847808772,1.07174847808772)))
REPRESENTATION_ITEM('')
SURFACE()
);
#203=(
BOUNDED_SURFACE()
B_SPLINE_SURFACE(3,3,((#43709,#43710,#43711,#43712,#43713,#43714,#43715,
#43716,#43717),(#43718,#43719,#43720,#43721,#43722,#43723,#43724,#43725,
#43726),(#43727,#43728,#43729,#43730,#43731,#43732,#43733,#43734,#43735),
(#43736,#43737,#43738,#43739,#43740,#43741,#43742,#43743,#43744)),
 .UNSPECIFIED.,.F.,.F.,.F.)
B_SPLINE_SURFACE_WITH_KNOTS((4,4),(4,1,1,1,1,1,4),(0.0545793311456824,0.945422488105894),
(0.227011587403803,0.2408830109939,0.3597029788418,0.4766081773206,0.5901375306021,
0.6993568121789,0.773423223303175),.UNSPECIFIED.)
GEOMETRIC_REPRESENTATION_ITEM()
RATIONAL_B_SPLINE_SURFACE(((1.19600373875636,1.19600373875636,1.19600373875636,
1.19600373875636,1.19600373875636,1.19600373875636,1.19600373875636,1.19600373875636,
1.19600373875636),(0.934664886716483,0.934664886716483,0.934664886716483,
0.934664886716483,0.934664886716483,0.934664886716483,0.934664886716483,
0.934664886716483,0.934664886716483),(0.934665420415469,0.934665420415469,
0.934665420415469,0.934665420415469,0.934665420415469,0.934665420415469,
0.934665420415469,0.934665420415469,0.934665420415469),(1.19600533985332,
1.19600533985332,1.19600533985332,1.19600533985332,1.19600533985332,1.19600533985332,
1.19600533985332,1.19600533985332,1.19600533985332)))
REPRESENTATION_ITEM('')
SURFACE()
);
#204=(
BOUNDED_SURFACE()
B_SPLINE_SURFACE(3,3,((#43867,#43868,#43869,#43870,#43871,#43872,#43873,
#43874,#43875,#43876),(#43877,#43878,#43879,#43880,#43881,#43882,#43883,
#43884,#43885,#43886),(#43887,#43888,#43889,#43890,#43891,#43892,#43893,
#43894,#43895,#43896),(#43897,#43898,#43899,#43900,#43901,#43902,#43903,
#43904,#43905,#43906)),.UNSPECIFIED.,.F.,.F.,.F.)
B_SPLINE_SURFACE_WITH_KNOTS((4,4),(4,1,1,1,1,1,1,4),(0.0897026965389358,
0.903562338706292),(0.02295305876098,0.1427319370604,0.2857219203474,0.4285792797614,
0.5713515650105,0.7142098207389,0.8572808214069,0.9622634165798),
 .UNSPECIFIED.)
GEOMETRIC_REPRESENTATION_ITEM()
RATIONAL_B_SPLINE_SURFACE(((1.11534309473627,1.11534309473627,1.11534309473627,
1.11534309473627,1.11534309473627,1.11534309473627,1.11534309473627,1.11534309473627,
1.11534309473627,1.11534309473627),(0.962814527415761,0.962814527415761,
0.962814527415761,0.962814527415761,0.962814527415761,0.962814527415761,
0.962814527415761,0.962814527415761,0.962814527415761,0.962814527415761),
(0.961562661370903,0.961562661370903,0.961562661370903,0.961562661370903,
0.961562661370903,0.961562661370903,0.961562661370903,0.961562661370903,
0.961562661370903,0.961562661370903),(1.11158749660169,1.11158749660169,
1.11158749660169,1.11158749660169,1.11158749660169,1.11158749660169,1.11158749660169,
1.11158749660169,1.11158749660169,1.11158749660169)))
REPRESENTATION_ITEM('')
SURFACE()
);
#205=(
BOUNDED_SURFACE()
B_SPLINE_SURFACE(3,3,((#44125,#44126,#44127,#44128,#44129,#44130,#44131,
#44132,#44133,#44134),(#44135,#44136,#44137,#44138,#44139,#44140,#44141,
#44142,#44143,#44144),(#44145,#44146,#44147,#44148,#44149,#44150,#44151,
#44152,#44153,#44154),(#44155,#44156,#44157,#44158,#44159,#44160,#44161,
#44162,#44163,#44164)),.UNSPECIFIED.,.F.,.F.,.F.)
B_SPLINE_SURFACE_WITH_KNOTS((4,4),(4,1,1,1,1,1,1,4),(0.0573437802388626,
0.942642820662885),(0.2948660946595,0.3474071011045,0.4097589840936,0.4702619662571,
0.529805073191,0.590310974462,0.6526656534762,0.705101945972),
 .UNSPECIFIED.)
GEOMETRIC_REPRESENTATION_ITEM()
RATIONAL_B_SPLINE_SURFACE(((1.19357372994919,1.19357372994919,1.19357372994919,
1.19357372994919,1.19357372994919,1.19357372994919,1.19357372994919,1.19357372994919,
1.19357372994919,1.19357372994919),(0.935479329637411,0.935479329637411,
0.935479329637411,0.935479329637411,0.935479329637411,0.935479329637411,
0.935479329637411,0.935479329637411,0.935479329637411,0.935479329637411),
(0.935475423409424,0.935475423409424,0.935475423409424,0.935475423409424,
0.935475423409424,0.935475423409424,0.935475423409424,0.935475423409424,
0.935475423409424,0.935475423409424),(1.19356201126523,1.19356201126523,
1.19356201126523,1.19356201126523,1.19356201126523,1.19356201126523,1.19356201126523,
1.19356201126523,1.19356201126523,1.19356201126523)))
REPRESENTATION_ITEM('')
SURFACE()
);
#206=(
BOUNDED_SURFACE()
B_SPLINE_SURFACE(3,3,((#44259,#44260,#44261,#44262,#44263,#44264,#44265,
#44266,#44267),(#44268,#44269,#44270,#44271,#44272,#44273,#44274,#44275,
#44276),(#44277,#44278,#44279,#44280,#44281,#44282,#44283,#44284,#44285),
(#44286,#44287,#44288,#44289,#44290,#44291,#44292,#44293,#44294)),
 .UNSPECIFIED.,.F.,.F.,.F.)
B_SPLINE_SURFACE_WITH_KNOTS((4,4),(4,1,1,1,1,1,4),(0.0548579677244621,0.945143053644028),
(0.226589591927513,0.2992910874271,0.4098062007976,0.5242045106109,0.6406468664689,
0.7577450573157,0.772721238525241),.UNSPECIFIED.)
GEOMETRIC_REPRESENTATION_ITEM()
RATIONAL_B_SPLINE_SURFACE(((1.19575728709686,1.19575728709686,1.19575728709686,
1.19575728709686,1.19575728709686,1.19575728709686,1.19575728709686,1.19575728709686,
1.19575728709686),(0.934747271527121,0.934747271527121,0.934747271527121,
0.934747271527121,0.934747271527121,0.934747271527121,0.934747271527121,
0.934747271527121,0.934747271527121),(0.934747570967958,0.934747570967958,
0.934747570967958,0.934747570967958,0.934747570967958,0.934747570967958,
0.934747570967958,0.934747570967958,0.934747570967958),(1.19575818541937,
1.19575818541937,1.19575818541937,1.19575818541937,1.19575818541937,1.19575818541937,
1.19575818541937,1.19575818541937,1.19575818541937)))
REPRESENTATION_ITEM('')
SURFACE()
);
#207=(
BOUNDED_SURFACE()
B_SPLINE_SURFACE(3,3,((#44408,#44409,#44410,#44411,#44412,#44413,#44414,
#44415,#44416,#44417,#44418),(#44419,#44420,#44421,#44422,#44423,#44424,
#44425,#44426,#44427,#44428,#44429),(#44430,#44431,#44432,#44433,#44434,
#44435,#44436,#44437,#44438,#44439,#44440),(#44441,#44442,#44443,#44444,
#44445,#44446,#44447,#44448,#44449,#44450,#44451)),.UNSPECIFIED.,.F.,.F.,
 .F.)
B_SPLINE_SURFACE_WITH_KNOTS((4,4),(4,1,1,1,1,1,1,1,4),(0.075363327412368,
0.90576708085259),(-0.009670337409301,0.,0.1430996309434,0.2858291680282,
0.4284783625449,0.5715211775605,0.714546629698,0.8573667380228,0.9759160461734),
 .UNSPECIFIED.)
GEOMETRIC_REPRESENTATION_ITEM()
RATIONAL_B_SPLINE_SURFACE(((1.12354608676129,1.12354608676129,1.12354608676129,
1.12354608676129,1.12354608676129,1.12354608676129,1.12354608676129,1.12354608676129,
1.12354608676129,1.12354608676129,1.12354608676129),(0.962477985028778,
0.962477985028778,0.962477985028778,0.962477985028778,0.962477985028778,
0.962477985028778,0.962477985028778,0.962477985028778,0.962477985028778,
0.962477985028778,0.962477985028778),(0.958899291150656,0.958899291150656,
0.958899291150656,0.958899291150656,0.958899291150656,0.958899291150656,
0.958899291150656,0.958899291150656,0.958899291150656,0.958899291150656,
0.958899291150656),(1.11281000512692,1.11281000512692,1.11281000512692,
1.11281000512692,1.11281000512692,1.11281000512692,1.11281000512692,1.11281000512692,
1.11281000512692,1.11281000512692,1.11281000512692)))
REPRESENTATION_ITEM('')
SURFACE()
);
#208=(
BOUNDED_SURFACE()
B_SPLINE_SURFACE(3,3,((#44568,#44569,#44570,#44571),(#44572,#44573,#44574,
#44575),(#44576,#44577,#44578,#44579),(#44580,#44581,#44582,#44583)),
 .UNSPECIFIED.,.F.,.F.,.F.)
B_SPLINE_SURFACE_WITH_KNOTS((4,4),(4,4),(0.0986320319756791,0.901362552764652),
(-0.975145040412961,-0.0991746183684475),.UNSPECIFIED.)
GEOMETRIC_REPRESENTATION_ITEM()
RATIONAL_B_SPLINE_SURFACE(((1.17563600438331,1.17563600438331,1.17563600438331,
1.17563600438331),(0.941456244993666,0.941456244993666,0.941456244993666,
0.941456244993666),(0.941454665216122,0.941454665216122,0.941454665216122,
0.941454665216122),(1.17563126505067,1.17563126505067,1.17563126505067,
1.17563126505067)))
REPRESENTATION_ITEM('')
SURFACE()
);
#209=(
BOUNDED_SURFACE()
B_SPLINE_SURFACE(3,3,((#44602,#44603,#44604,#44605,#44606,#44607,#44608,
#44609,#44610,#44611,#44612,#44613,#44614,#44615,#44616,#44617,#44618,#44619,
#44620,#44621,#44622,#44623,#44624,#44625,#44626,#44627,#44628,#44629,#44630,
#44631,#44632,#44633,#44634),(#44635,#44636,#44637,#44638,#44639,#44640,
#44641,#44642,#44643,#44644,#44645,#44646,#44647,#44648,#44649,#44650,#44651,
#44652,#44653,#44654,#44655,#44656,#44657,#44658,#44659,#44660,#44661,#44662,
#44663,#44664,#44665,#44666,#44667),(#44668,#44669,#44670,#44671,#44672,
#44673,#44674,#44675,#44676,#44677,#44678,#44679,#44680,#44681,#44682,#44683,
#44684,#44685,#44686,#44687,#44688,#44689,#44690,#44691,#44692,#44693,#44694,
#44695,#44696,#44697,#44698,#44699,#44700),(#44701,#44702,#44703,#44704,
#44705,#44706,#44707,#44708,#44709,#44710,#44711,#44712,#44713,#44714,#44715,
#44716,#44717,#44718,#44719,#44720,#44721,#44722,#44723,#44724,#44725,#44726,
#44727,#44728,#44729,#44730,#44731,#44732,#44733)),.UNSPECIFIED.,.F.,.F.,
 .F.)
B_SPLINE_SURFACE_WITH_KNOTS((4,4),(4,1,1,1,1,1,1,1,1,1,1,1,1,1,1,1,1,1,
1,1,1,1,1,1,1,1,1,1,1,1,4),(0.108378650282158,0.90358623629129),(-0.009736901743293,
0.,0.02218413179616,0.04656961109721,0.07320227078019,0.1023246073732,0.1343070073132,
0.1695983831374,0.2086113444912,0.2515282384572,0.298570017754,0.3503280366984,
0.407666728873,0.4682132326112,0.5282256466259,0.5849768379281,0.6367767624527,
0.6825350754217,0.7235069669533,0.7605071950843,0.7940293660324,0.8241786597915,
0.8510660708046,0.8750221728306,0.8964633607917,0.915795400779,0.9333737553402,
0.9493579414425,0.9638585657324,0.9770543416126,0.985715500525),
 .UNSPECIFIED.)
GEOMETRIC_REPRESENTATION_ITEM()
RATIONAL_B_SPLINE_SURFACE(((1.07414501661197,1.07414501661197,1.07414501661197,
1.07414501661197,1.07414501661197,1.07414501661197,1.07414501661197,1.07414501661197,
1.07414501661197,1.07414501661197,1.07414501661197,1.07414501661197,1.07414501661197,
1.07414501661197,1.07414501661197,1.07414501661197,1.07414501661197,1.07414501661197,
1.07414501661197,1.07414501661197,1.07414501661197,1.07414501661197,1.07414501661197,
1.07414501661197,1.07414501661197,1.07414501661197,1.07414501661197,1.07414501661197,
1.07414501661197,1.07414501661197,1.07414501661197,1.07414501661197,1.07414501661197),
(0.973774799790487,0.973774799790487,0.973774799790487,0.973774799790487,
0.973774799790487,0.973774799790487,0.973774799790487,0.973774799790487,
0.973774799790487,0.973774799790487,0.973774799790487,0.973774799790487,
0.973774799790487,0.973774799790487,0.973774799790487,0.973774799790487,
0.973774799790487,0.973774799790487,0.973774799790487,0.973774799790487,
0.973774799790487,0.973774799790487,0.973774799790487,0.973774799790487,
0.973774799790487,0.973774799790487,0.973774799790487,0.973774799790487,
0.973774799790487,0.973774799790487,0.973774799790487,0.973774799790487,
0.973774799790487),(0.975308064333504,0.975308064333504,0.975308064333504,
0.975308064333504,0.975308064333504,0.975308064333504,0.975308064333504,
0.975308064333504,0.975308064333504,0.975308064333504,0.975308064333504,
0.975308064333504,0.975308064333504,0.975308064333504,0.975308064333504,
0.975308064333504,0.975308064333504,0.975308064333504,0.975308064333504,
0.975308064333504,0.975308064333504,0.975308064333504,0.975308064333504,
0.975308064333504,0.975308064333504,0.975308064333504,0.975308064333504,
0.975308064333504,0.975308064333504,0.975308064333504,0.975308064333504,
0.975308064333504,0.975308064333504),(1.07874481024102,1.07874481024102,
1.07874481024102,1.07874481024102,1.07874481024102,1.07874481024102,1.07874481024102,
1.07874481024102,1.07874481024102,1.07874481024102,1.07874481024102,1.07874481024102,
1.07874481024102,1.07874481024102,1.07874481024102,1.07874481024102,1.07874481024102,
1.07874481024102,1.07874481024102,1.07874481024102,1.07874481024102,1.07874481024102,
1.07874481024102,1.07874481024102,1.07874481024102,1.07874481024102,1.07874481024102,
1.07874481024102,1.07874481024102,1.07874481024102,1.07874481024102,1.07874481024102,
1.07874481024102)))
REPRESENTATION_ITEM('')
SURFACE()
);
#210=(
BOUNDED_SURFACE()
B_SPLINE_SURFACE(3,3,((#45120,#45121,#45122,#45123,#45124,#45125,#45126,
#45127,#45128,#45129),(#45130,#45131,#45132,#45133,#45134,#45135,#45136,
#45137,#45138,#45139),(#45140,#45141,#45142,#45143,#45144,#45145,#45146,
#45147,#45148,#45149),(#45150,#45151,#45152,#45153,#45154,#45155,#45156,
#45157,#45158,#45159)),.UNSPECIFIED.,.F.,.F.,.F.)
B_SPLINE_SURFACE_WITH_KNOTS((4,4),(4,1,1,1,1,1,1,4),(0.0576542468391072,
0.942338471723155),(0.2949063013325,0.3507658351833,0.4113946127403,0.470739629438,
0.5289312325493,0.5882633205163,0.6488928044224,0.7051344531532),
 .UNSPECIFIED.)
GEOMETRIC_REPRESENTATION_ITEM()
RATIONAL_B_SPLINE_SURFACE(((1.19330101599729,1.19330101599729,1.19330101599729,
1.19330101599729,1.19330101599729,1.19330101599729,1.19330101599729,1.19330101599729,
1.19330101599729,1.19330101599729),(0.935568449281609,0.935568449281609,
0.935568449281609,0.935568449281609,0.935568449281609,0.935568449281609,
0.935568449281609,0.935568449281609,0.935568449281609,0.935568449281609),
(0.935566328018295,0.935566328018295,0.935566328018295,0.935566328018295,
0.935566328018295,0.935566328018295,0.935566328018295,0.935566328018295,
0.935566328018295,0.935566328018295),(1.19329465220735,1.19329465220735,
1.19329465220735,1.19329465220735,1.19329465220735,1.19329465220735,1.19329465220735,
1.19329465220735,1.19329465220735,1.19329465220735)))
REPRESENTATION_ITEM('')
SURFACE()
);
#211=(
BOUNDED_SURFACE()
B_SPLINE_SURFACE(3,3,((#45250,#45251,#45252,#45253,#45254,#45255,#45256,
#45257,#45258),(#45259,#45260,#45261,#45262,#45263,#45264,#45265,#45266,
#45267),(#45268,#45269,#45270,#45271,#45272,#45273,#45274,#45275,#45276),
(#45277,#45278,#45279,#45280,#45281,#45282,#45283,#45284,#45285)),
 .UNSPECIFIED.,.F.,.F.,.F.)
B_SPLINE_SURFACE_WITH_KNOTS((4,4),(4,1,1,1,1,1,4),(0.0549539789496563,0.945047550786385),
(0.225999549185134,0.2426046586147,0.359632647929,0.4760208069216,0.5903747960474,
0.7008431878989,0.773895646058005),.UNSPECIFIED.)
GEOMETRIC_REPRESENTATION_ITEM()
RATIONAL_B_SPLINE_SURFACE(((1.19567368239687,1.19567368239687,1.19567368239687,
1.19567368239687,1.19567368239687,1.19567368239687,1.19567368239687,1.19567368239687,
1.19567368239687),(0.934774990814295,0.934774990814295,0.934774990814295,
0.934774990814295,0.934774990814295,0.934774990814295,0.934774990814295,
0.934774990814295,0.934774990814295),(0.93477543920178,0.93477543920178,
0.93477543920178,0.93477543920178,0.93477543920178,0.93477543920178,0.93477543920178,
0.93477543920178,0.93477543920178),(1.19567502755933,1.19567502755933,1.19567502755933,
1.19567502755933,1.19567502755933,1.19567502755933,1.19567502755933,1.19567502755933,
1.19567502755933)))
REPRESENTATION_ITEM('')
SURFACE()
);
#212=(
BOUNDED_SURFACE()
B_SPLINE_SURFACE(3,3,((#45402,#45403,#45404,#45405,#45406,#45407,#45408,
#45409,#45410,#45411),(#45412,#45413,#45414,#45415,#45416,#45417,#45418,
#45419,#45420,#45421),(#45422,#45423,#45424,#45425,#45426,#45427,#45428,
#45429,#45430,#45431),(#45432,#45433,#45434,#45435,#45436,#45437,#45438,
#45439,#45440,#45441)),.UNSPECIFIED.,.F.,.F.,.F.)
B_SPLINE_SURFACE_WITH_KNOTS((4,4),(4,1,1,1,1,1,1,4),(0.0902151502653892,
0.906139739364474),(0.0113422875341,0.1428793791643,0.2858116106518,0.4286834137584,
0.5714931631331,0.7143130817917,0.857293314129,0.9764111906614),
 .UNSPECIFIED.)
GEOMETRIC_REPRESENTATION_ITEM()
RATIONAL_B_SPLINE_SURFACE(((1.11548012320919,1.11548012320919,1.11548012320919,
1.11548012320919,1.11548012320919,1.11548012320919,1.11548012320919,1.11548012320919,
1.11548012320919,1.11548012320919),(0.962191436654982,0.962191436654982,
0.962191436654982,0.962191436654982,0.962191436654982,0.962191436654982,
0.962191436654982,0.962191436654982,0.962191436654982,0.962191436654982),
(0.961509671356259,0.961509671356259,0.961509671356259,0.961509671356259,
0.961509671356259,0.961509671356259,0.961509671356259,0.961509671356259,
0.961509671356259,0.961509671356259),(1.11343482731302,1.11343482731302,
1.11343482731302,1.11343482731302,1.11343482731302,1.11343482731302,1.11343482731302,
1.11343482731302,1.11343482731302,1.11343482731302)))
REPRESENTATION_ITEM('')
SURFACE()
);
#213=(
BOUNDED_SURFACE()
B_SPLINE_SURFACE(3,3,((#45468,#45469,#45470,#45471,#45472,#45473,#45474,
#45475),(#45476,#45477,#45478,#45479,#45480,#45481,#45482,#45483),(#45484,
#45485,#45486,#45487,#45488,#45489,#45490,#45491),(#45492,#45493,#45494,
#45495,#45496,#45497,#45498,#45499)),.UNSPECIFIED.,.F.,.F.,.F.)
B_SPLINE_SURFACE_WITH_KNOTS((4,4),(4,1,1,1,1,4),(0.0538108527545732,0.94619037239879),
(0.229096267158528,0.3087140271309,0.421124754351,0.5382875231502,0.659432849143,
0.77499777021192),.UNSPECIFIED.)
GEOMETRIC_REPRESENTATION_ITEM()
RATIONAL_B_SPLINE_SURFACE(((1.19668201979503,1.19668201979503,1.19668201979503,
1.19668201979503,1.19668201979503,1.19668201979503,1.19668201979503,1.19668201979503),
(0.934438966699946,0.934438966699946,0.934438966699946,0.934438966699946,
0.934438966699946,0.934438966699946,0.934438966699946,0.934438966699946),
(0.93443932673555,0.93443932673555,0.93443932673555,0.93443932673555,0.93443932673555,
0.93443932673555,0.93443932673555,0.93443932673555),(1.19668309990185,1.19668309990185,
1.19668309990185,1.19668309990185,1.19668309990185,1.19668309990185,1.19668309990185,
1.19668309990185)))
REPRESENTATION_ITEM('')
SURFACE()
);
#214=(
BOUNDED_SURFACE()
B_SPLINE_SURFACE(3,3,((#45616,#45617,#45618,#45619,#45620,#45621,#45622,
#45623,#45624,#45625),(#45626,#45627,#45628,#45629,#45630,#45631,#45632,
#45633,#45634,#45635),(#45636,#45637,#45638,#45639,#45640,#45641,#45642,
#45643,#45644,#45645),(#45646,#45647,#45648,#45649,#45650,#45651,#45652,
#45653,#45654,#45655)),.UNSPECIFIED.,.F.,.F.,.F.)
B_SPLINE_SURFACE_WITH_KNOTS((4,4),(4,1,1,1,1,1,1,4),(0.0902467380234992,
0.903452489290608),(0.02358777780153,0.1427066858466,0.2856869182934,0.4285068377462,
0.5713165853686,0.7141883873726,0.8571206201588,0.9886565450661),
 .UNSPECIFIED.)
GEOMETRIC_REPRESENTATION_ITEM()
RATIONAL_B_SPLINE_SURFACE(((1.11546232169106,1.11546232169106,1.11546232169106,
1.11546232169106,1.11546232169106,1.11546232169106,1.11546232169106,1.11546232169106,
1.11546232169106,1.11546232169106),(0.962696201577782,0.962696201577782,
0.962696201577782,0.962696201577782,0.962696201577782,0.962696201577782,
0.962696201577782,0.962696201577782,0.962696201577782,0.962696201577782),
(0.961521659864195,0.961521659864195,0.961521659864195,0.961521659864195,
0.961521659864195,0.961521659864195,0.961521659864195,0.961521659864195,
0.961521659864195,0.961521659864195),(1.1119386965503,1.1119386965503,1.1119386965503,
1.1119386965503,1.1119386965503,1.1119386965503,1.1119386965503,1.1119386965503,
1.1119386965503,1.1119386965503)))
REPRESENTATION_ITEM('')
SURFACE()
);
#215=(
BOUNDED_SURFACE()
B_SPLINE_SURFACE(3,3,((#45695,#45696,#45697,#45698,#45699,#45700),(#45701,
#45702,#45703,#45704,#45705,#45706),(#45707,#45708,#45709,#45710,#45711,
#45712),(#45713,#45714,#45715,#45716,#45717,#45718)),.UNSPECIFIED.,.F.,
 .F.,.F.)
B_SPLINE_SURFACE_WITH_KNOTS((4,4),(4,1,1,4),(0.0986342191388391,0.901369959991362),
(0.317543733196465,0.3333147448852,0.6666852551147,0.682456266811625),
 .UNSPECIFIED.)
GEOMETRIC_REPRESENTATION_ITEM()
RATIONAL_B_SPLINE_SURFACE(((1.17563408853202,1.17563408853202,1.17563408853202,
1.17563408853202,1.17563408853202,1.17563408853202),(0.941454084656006,
0.941454084656006,0.941454084656006,0.941454084656006,0.941454084656006,
0.941454084656006),(0.941455303829106,0.941455303829106,0.941455303829106,
0.941455303829106,0.941455303829106,0.941455303829106),(1.17563774605132,
1.17563774605132,1.17563774605132,1.17563774605132,1.17563774605132,1.17563774605132)))
REPRESENTATION_ITEM('')
SURFACE()
);
#216=(
BOUNDED_SURFACE()
B_SPLINE_SURFACE(3,3,((#45958,#45959,#45960,#45961,#45962,#45963,#45964,
#45965,#45966,#45967,#45968,#45969,#45970,#45971,#45972,#45973,#45974,#45975,
#45976,#45977,#45978,#45979,#45980,#45981,#45982,#45983,#45984,#45985,#45986,
#45987,#45988,#45989,#45990,#45991,#45992,#45993,#45994,#45995,#45996,#45997),
(#45998,#45999,#46000,#46001,#46002,#46003,#46004,#46005,#46006,#46007,
#46008,#46009,#46010,#46011,#46012,#46013,#46014,#46015,#46016,#46017,#46018,
#46019,#46020,#46021,#46022,#46023,#46024,#46025,#46026,#46027,#46028,#46029,
#46030,#46031,#46032,#46033,#46034,#46035,#46036,#46037),(#46038,#46039,
#46040,#46041,#46042,#46043,#46044,#46045,#46046,#46047,#46048,#46049,#46050,
#46051,#46052,#46053,#46054,#46055,#46056,#46057,#46058,#46059,#46060,#46061,
#46062,#46063,#46064,#46065,#46066,#46067,#46068,#46069,#46070,#46071,#46072,
#46073,#46074,#46075,#46076,#46077),(#46078,#46079,#46080,#46081,#46082,
#46083,#46084,#46085,#46086,#46087,#46088,#46089,#46090,#46091,#46092,#46093,
#46094,#46095,#46096,#46097,#46098,#46099,#46100,#46101,#46102,#46103,#46104,
#46105,#46106,#46107,#46108,#46109,#46110,#46111,#46112,#46113,#46114,#46115,
#46116,#46117)),.UNSPECIFIED.,.F.,.F.,.F.)
B_SPLINE_SURFACE_WITH_KNOTS((4,4),(4,1,1,1,1,1,1,1,1,1,1,1,1,1,1,1,1,1,
1,1,1,1,1,1,1,1,1,1,1,1,1,1,1,1,1,1,1,4),(0.109557621894297,0.885243870276793),
(-0.009601789273476,0.,0.02232833549642,0.04690550208409,0.0737936246764,
0.1032829469292,0.1358149659664,0.1719129604536,0.2120204765653,0.256254955895,
0.3048250014022,0.3583933178747,0.4161357109072,0.4734125795356,0.5265814299979,
0.5739176940624,0.615519024704,0.652991192313,0.6871377766576,0.7180210170715,
0.7460333746096,0.7715274743224,0.7947401813882,0.8158383097162,0.8349870800801,
0.8523592732018,0.8681377597697,0.8825020836392,0.8956292723193,0.907695283691,
0.9188455009777,0.9291452784588,0.9386432333898,0.9473858993637,0.9554254804025,
0.9628154053196,0.9696060115487,0.972066289616),.UNSPECIFIED.)
GEOMETRIC_REPRESENTATION_ITEM()
RATIONAL_B_SPLINE_SURFACE(((1.07369790078242,1.07369790078242,1.07369790078242,
1.07369790078242,1.07369790078242,1.07369790078242,1.07369790078242,1.07369790078242,
1.07369790078242,1.07369790078242,1.07369790078242,1.07369790078242,1.07369790078242,
1.07369790078242,1.07369790078242,1.07369790078242,1.07369790078242,1.07369790078242,
1.07369790078242,1.07369790078242,1.07369790078242,1.07369790078242,1.07369790078242,
1.07369790078242,1.07369790078242,1.07369790078242,1.07369790078242,1.07369790078242,
1.07369790078242,1.07369790078242,1.07369790078242,1.07369790078242,1.07369790078242,
1.07369790078242,1.07369790078242,1.07369790078242,1.07369790078242,1.07369790078242,
1.07369790078242,1.07369790078242),(0.976088195522974,0.976088195522974,
0.976088195522974,0.976088195522974,0.976088195522974,0.976088195522974,
0.976088195522974,0.976088195522974,0.976088195522974,0.976088195522974,
0.976088195522974,0.976088195522974,0.976088195522974,0.976088195522974,
0.976088195522974,0.976088195522974,0.976088195522974,0.976088195522974,
0.976088195522974,0.976088195522974,0.976088195522974,0.976088195522974,
0.976088195522974,0.976088195522974,0.976088195522974,0.976088195522974,
0.976088195522974,0.976088195522974,0.976088195522974,0.976088195522974,
0.976088195522974,0.976088195522974,0.976088195522974,0.976088195522974,
0.976088195522974,0.976088195522974,0.976088195522974,0.976088195522974,
0.976088195522974,0.976088195522974),(0.97543838796439,0.97543838796439,
0.97543838796439,0.97543838796439,0.97543838796439,0.97543838796439,0.97543838796439,
0.97543838796439,0.97543838796439,0.97543838796439,0.97543838796439,0.97543838796439,
0.97543838796439,0.97543838796439,0.97543838796439,0.97543838796439,0.97543838796439,
0.97543838796439,0.97543838796439,0.97543838796439,0.97543838796439,0.97543838796439,
0.97543838796439,0.97543838796439,0.97543838796439,0.97543838796439,0.97543838796439,
0.97543838796439,0.97543838796439,0.97543838796439,0.97543838796439,0.97543838796439,
0.97543838796439,0.97543838796439,0.97543838796439,0.97543838796439,0.97543838796439,
0.97543838796439,0.97543838796439,0.97543838796439),(1.07174847810667,1.07174847810667,
1.07174847810667,1.07174847810667,1.07174847810667,1.07174847810667,1.07174847810667,
1.07174847810667,1.07174847810667,1.07174847810667,1.07174847810667,1.07174847810667,
1.07174847810667,1.07174847810667,1.07174847810667,1.07174847810667,1.07174847810667,
1.07174847810667,1.07174847810667,1.07174847810667,1.07174847810667,1.07174847810667,
1.07174847810667,1.07174847810667,1.07174847810667,1.07174847810667,1.07174847810667,
1.07174847810667,1.07174847810667,1.07174847810667,1.07174847810667,1.07174847810667,
1.07174847810667,1.07174847810667,1.07174847810667,1.07174847810667,1.07174847810667,
1.07174847810667,1.07174847810667,1.07174847810667)))
REPRESENTATION_ITEM('')
SURFACE()
);
#217=(
BOUNDED_SURFACE()
B_SPLINE_SURFACE(3,3,((#46243,#46244,#46245,#46246,#46247,#46248,#46249,
#46250),(#46251,#46252,#46253,#46254,#46255,#46256,#46257,#46258),(#46259,
#46260,#46261,#46262,#46263,#46264,#46265,#46266),(#46267,#46268,#46269,
#46270,#46271,#46272,#46273,#46274)),.UNSPECIFIED.,.F.,.F.,.F.)
B_SPLINE_SURFACE_WITH_KNOTS((4,4),(4,1,1,1,1,4),(0.0538140162332302,0.946187598359706),
(0.226399629870169,0.3386790291836,0.4601779185567,0.5776891459497,0.6904350358172,
0.773432296606802),.UNSPECIFIED.)
GEOMETRIC_REPRESENTATION_ITEM()
RATIONAL_B_SPLINE_SURFACE(((1.19667979358655,1.19667979358655,1.19667979358655,
1.19667979358655,1.19667979358655,1.19667979358655,1.19667979358655,1.19667979358655),
(0.934439594326999,0.934439594326999,0.934439594326999,0.934439594326999,
0.934439594326999,0.934439594326999,0.934439594326999,0.934439594326999),
(0.934440068805344,0.934440068805343,0.934440068805343,0.934440068805343,
0.934440068805343,0.934440068805343,0.934440068805343,0.934440068805343),
(1.19668121702158,1.19668121702158,1.19668121702158,1.19668121702158,1.19668121702158,
1.19668121702158,1.19668121702158,1.19668121702158)))
REPRESENTATION_ITEM('')
SURFACE()
);
#218=(
BOUNDED_SURFACE()
B_SPLINE_SURFACE(3,3,((#46394,#46395,#46396,#46397,#46398,#46399,#46400,
#46401,#46402,#46403),(#46404,#46405,#46406,#46407,#46408,#46409,#46410,
#46411,#46412,#46413),(#46414,#46415,#46416,#46417,#46418,#46419,#46420,
#46421,#46422,#46423),(#46424,#46425,#46426,#46427,#46428,#46429,#46430,
#46431,#46432,#46433)),.UNSPECIFIED.,.F.,.F.,.F.)
B_SPLINE_SURFACE_WITH_KNOTS((4,4),(4,1,1,1,1,1,1,4),(0.0889032005159359,
0.902793520014641),(0.02295305876274,0.1427319133548,0.2857218418975,0.4285793286892,
0.5713517372348,0.7142096687795,0.8572807309771,0.9622634166072),
 .UNSPECIFIED.)
GEOMETRIC_REPRESENTATION_ITEM()
RATIONAL_B_SPLINE_SURFACE(((1.11579304262805,1.11579304262805,1.11579304262805,
1.11579304262805,1.11579304262805,1.11579304262805,1.11579304262805,1.11579304262805,
1.11579304262805,1.11579304262805),(0.962961500959473,0.962961500959473,
0.962961500959473,0.962961500959473,0.962961500959473,0.962961500959473,
0.962961500959473,0.962961500959473,0.962961500959473,0.962961500959473),
(0.961418065199563,0.961418065199563,0.961418065199563,0.961418065199563,
0.961418065199563,0.961418065199563,0.961418065199563,0.961418065199563,
0.961418065199563,0.961418065199563),(1.11116273534832,1.11116273534832,
1.11116273534832,1.11116273534832,1.11116273534832,1.11116273534832,1.11116273534832,
1.11116273534832,1.11116273534832,1.11116273534832)))
REPRESENTATION_ITEM('')
SURFACE()
);
#219=(
BOUNDED_SURFACE()
B_SPLINE_SURFACE(3,3,((#46652,#46653,#46654,#46655,#46656,#46657,#46658,
#46659,#46660,#46661),(#46662,#46663,#46664,#46665,#46666,#46667,#46668,
#46669,#46670,#46671),(#46672,#46673,#46674,#46675,#46676,#46677,#46678,
#46679,#46680,#46681),(#46682,#46683,#46684,#46685,#46686,#46687,#46688,
#46689,#46690,#46691)),.UNSPECIFIED.,.F.,.F.,.F.)
B_SPLINE_SURFACE_WITH_KNOTS((4,4),(4,1,1,1,1,1,1,4),(0.0566082084903071,
0.943377877952831),(0.294866436509,0.3476249436887,0.4099876923829,0.4703085802384,
0.5297603546224,0.5900842016518,0.6524504076229,0.7051016030693),
 .UNSPECIFIED.)
GEOMETRIC_REPRESENTATION_ITEM()
RATIONAL_B_SPLINE_SURFACE(((1.19421794191571,1.19421794191571,1.19421794191571,
1.19421794191571,1.19421794191571,1.19421794191571,1.19421794191571,1.19421794191571,
1.19421794191571,1.19421794191571),(0.935264749044728,0.935264749044728,
0.935264749044728,0.935264749044728,0.935264749044728,0.935264749044728,
0.935264749044728,0.935264749044728,0.935264749044728,0.935264749044728),
(0.935260686091779,0.935260686091779,0.935260686091779,0.935260686091779,
0.935260686091779,0.935260686091779,0.935260686091779,0.935260686091779,
0.935260686091779,0.935260686091779),(1.19420575305686,1.19420575305686,
1.19420575305686,1.19420575305686,1.19420575305686,1.19420575305686,1.19420575305686,
1.19420575305686,1.19420575305686,1.19420575305686)))
REPRESENTATION_ITEM('')
SURFACE()
);
#220=(
BOUNDED_SURFACE()
B_SPLINE_SURFACE(3,3,((#46787,#46788,#46789,#46790),(#46791,#46792,#46793,
#46794),(#46795,#46796,#46797,#46798),(#46799,#46800,#46801,#46802)),
 .UNSPECIFIED.,.F.,.F.,.F.)
B_SPLINE_SURFACE_WITH_KNOTS((4,4),(4,4),(0.0986320320012492,0.901362552769613),
(-0.975145040391543,-0.0991746183696281),.UNSPECIFIED.)
GEOMETRIC_REPRESENTATION_ITEM()
RATIONAL_B_SPLINE_SURFACE(((1.1756360043584,1.1756360043584,1.1756360043584,
1.1756360043584),(0.94145624499323,0.94145624499323,0.94145624499323,0.94145624499323),
(0.941454665224592,0.941454665224592,0.941454665224592,0.941454665224592),
(1.17563126505248,1.17563126505248,1.17563126505248,1.17563126505248)))
REPRESENTATION_ITEM('')
SURFACE()
);
#221=(
BOUNDED_SURFACE()
B_SPLINE_SURFACE(3,3,((#46821,#46822,#46823,#46824,#46825,#46826,#46827,
#46828,#46829,#46830,#46831),(#46832,#46833,#46834,#46835,#46836,#46837,
#46838,#46839,#46840,#46841,#46842),(#46843,#46844,#46845,#46846,#46847,
#46848,#46849,#46850,#46851,#46852,#46853),(#46854,#46855,#46856,#46857,
#46858,#46859,#46860,#46861,#46862,#46863,#46864)),.UNSPECIFIED.,.F.,.F.,
 .F.)
B_SPLINE_SURFACE_WITH_KNOTS((4,4),(4,1,1,1,1,1,1,1,4),(0.0753633925353489,
0.90355881590316),(-0.009670337421385,0.,0.1430991485311,0.2858285059199,
0.4284781713031,0.5715215149008,0.7145472299923,0.8573672624017,0.9759160460961),
 .UNSPECIFIED.)
GEOMETRIC_REPRESENTATION_ITEM()
RATIONAL_B_SPLINE_SURFACE(((1.12354604889356,1.12354604889356,1.12354604889356,
1.12354604889356,1.12354604889356,1.12354604889356,1.12354604889356,1.12354604889356,
1.12354604889356,1.12354604889356,1.12354604889356),(0.962906307414026,
0.962906307414026,0.962906307414026,0.962906307414026,0.962906307414026,
0.962906307414026,0.962906307414026,0.962906307414026,0.962906307414026,
0.962906307414026,0.962906307414026),(0.958919450266201,0.958919450266201,
0.958919450266201,0.958919450266201,0.958919450266201,0.958919450266201,
0.958919450266201,0.958919450266201,0.958919450266201,0.958919450266201,
0.958919450266201),(1.11158547745009,1.11158547745009,1.11158547745009,
1.11158547745009,1.11158547745009,1.11158547745009,1.11158547745009,1.11158547745009,
1.11158547745009,1.11158547745009,1.11158547745009)))
REPRESENTATION_ITEM('')
SURFACE()
);
#222=(
BOUNDED_SURFACE()
B_SPLINE_SURFACE(3,3,((#47032,#47033,#47034,#47035,#47036,#47037,#47038,
#47039,#47040),(#47041,#47042,#47043,#47044,#47045,#47046,#47047,#47048,
#47049),(#47050,#47051,#47052,#47053,#47054,#47055,#47056,#47057,#47058),
(#47059,#47060,#47061,#47062,#47063,#47064,#47065,#47066,#47067)),
 .UNSPECIFIED.,.F.,.F.,.F.)
B_SPLINE_SURFACE_WITH_KNOTS((4,4),(4,1,1,1,1,1,4),(0.0545899833427553,0.945411009430165),
(0.226573738413812,0.3006458185641,0.409865708208,0.5233967602136,0.6403051050053,
0.7591301880906,0.77297490226788),.UNSPECIFIED.)
GEOMETRIC_REPRESENTATION_ITEM()
RATIONAL_B_SPLINE_SURFACE(((1.19599304937649,1.19599304937649,1.19599304937649,
1.19599304937649,1.19599304937649,1.19599304937649,1.19599304937649,1.19599304937649,
1.19599304937649),(0.934668692308928,0.934668692308928,0.934668692308928,
0.934668692308928,0.934668692308928,0.934668692308928,0.934668692308928,
0.934668692308928,0.934668692308928),(0.934668983541427,0.934668983541427,
0.934668983541427,0.934668983541427,0.934668983541427,0.934668983541427,
0.934668983541427,0.934668983541427,0.934668983541427),(1.19599392307399,
1.19599392307399,1.19599392307399,1.19599392307399,1.19599392307399,1.19599392307399,
1.19599392307399,1.19599392307399,1.19599392307399)))
REPRESENTATION_ITEM('')
SURFACE()
);
#223=(
BOUNDED_SURFACE()
B_SPLINE_SURFACE(3,3,((#47118,#47119,#47120,#47121,#47122,#47123,#47124,
#47125,#47126,#47127),(#47128,#47129,#47130,#47131,#47132,#47133,#47134,
#47135,#47136,#47137),(#47138,#47139,#47140,#47141,#47142,#47143,#47144,
#47145,#47146,#47147),(#47148,#47149,#47150,#47151,#47152,#47153,#47154,
#47155,#47156,#47157)),.UNSPECIFIED.,.F.,.F.,.F.)
B_SPLINE_SURFACE_WITH_KNOTS((4,4),(4,1,1,1,1,1,1,4),(0.0573875678003812,
0.942600786703194),(0.2949023604086,0.3473747858184,0.4097087132847,0.4701865626765,
0.5297465130048,0.5902215650413,0.6525525187134,0.7051382449586),
 .UNSPECIFIED.)
GEOMETRIC_REPRESENTATION_ITEM()
RATIONAL_B_SPLINE_SURFACE(((1.19353520188251,1.19353520188251,1.19353520188251,
1.19353520188251,1.19353520188251,1.19353520188251,1.19353520188251,1.19353520188251,
1.19353520188251,1.19353520188251),(0.935491660752717,0.935491660752717,
0.935491660752717,0.935491660752717,0.935491660752717,0.935491660752717,
0.935491660752717,0.935491660752717,0.935491660752717,0.935491660752717),
(0.935488266084021,0.935488266084021,0.935488266084021,0.935488266084021,
0.935488266084021,0.935488266084021,0.935488266084021,0.935488266084021,
0.935488266084021,0.935488266084021),(1.19352501787643,1.19352501787643,
1.19352501787643,1.19352501787643,1.19352501787643,1.19352501787643,1.19352501787643,
1.19352501787643,1.19352501787643,1.19352501787643)))
REPRESENTATION_ITEM('')
SURFACE()
);
#224=(
BOUNDED_SURFACE()
B_SPLINE_SURFACE(3,3,((#47465,#47466,#47467,#47468,#47469,#47470,#47471,
#47472,#47473,#47474,#47475,#47476,#47477,#47478,#47479,#47480,#47481,#47482,
#47483,#47484,#47485,#47486,#47487,#47488,#47489,#47490,#47491,#47492,#47493,
#47494,#47495,#47496,#47497),(#47498,#47499,#47500,#47501,#47502,#47503,
#47504,#47505,#47506,#47507,#47508,#47509,#47510,#47511,#47512,#47513,#47514,
#47515,#47516,#47517,#47518,#47519,#47520,#47521,#47522,#47523,#47524,#47525,
#47526,#47527,#47528,#47529,#47530),(#47531,#47532,#47533,#47534,#47535,
#47536,#47537,#47538,#47539,#47540,#47541,#47542,#47543,#47544,#47545,#47546,
#47547,#47548,#47549,#47550,#47551,#47552,#47553,#47554,#47555,#47556,#47557,
#47558,#47559,#47560,#47561,#47562,#47563),(#47564,#47565,#47566,#47567,
#47568,#47569,#47570,#47571,#47572,#47573,#47574,#47575,#47576,#47577,#47578,
#47579,#47580,#47581,#47582,#47583,#47584,#47585,#47586,#47587,#47588,#47589,
#47590,#47591,#47592,#47593,#47594,#47595,#47596)),.UNSPECIFIED.,.F.,.F.,
 .F.)
B_SPLINE_SURFACE_WITH_KNOTS((4,4),(4,1,1,1,1,1,1,1,1,1,1,1,1,1,1,1,1,1,
1,1,1,1,1,1,1,1,1,1,1,1,4),(0.108387652276654,0.903585982346435),(-0.00973690173883,
0.,0.02218340749114,0.04656850383599,0.0732012163466,0.102323831163,0.1343066238718,
0.1695984990841,0.2086121558901,0.2515303853581,0.298574638964,0.3503366286747,
0.4076785718675,0.4682255700403,0.5282360307647,0.5849839255341,0.6367806003876,
0.6825368401862,0.7235074075035,0.7605068126486,0.7940285468258,0.8241776680749,
0.8510650518271,0.8750212083659,0.8964625051051,0.9157946807002,0.9333731860453,
0.9493575699013,0.9638584550805,0.9770544701579,0.9857155005173),
 .UNSPECIFIED.)
GEOMETRIC_REPRESENTATION_ITEM()
RATIONAL_B_SPLINE_SURFACE(((1.07414161106479,1.07414161106479,1.07414161106479,
1.07414161106479,1.07414161106479,1.07414161106479,1.07414161106479,1.07414161106479,
1.07414161106479,1.07414161106479,1.07414161106479,1.07414161106479,1.07414161106479,
1.07414161106479,1.07414161106479,1.07414161106479,1.07414161106479,1.07414161106479,
1.07414161106479,1.07414161106479,1.07414161106479,1.07414161106479,1.07414161106479,
1.07414161106479,1.07414161106479,1.07414161106479,1.07414161106479,1.07414161106479,
1.07414161106479,1.07414161106479,1.07414161106479,1.07414161106479,1.07414161106479),
(0.973774865480363,0.973774865480363,0.973774865480363,0.973774865480363,
0.973774865480363,0.973774865480363,0.973774865480363,0.973774865480363,
0.973774865480363,0.973774865480363,0.973774865480363,0.973774865480363,
0.973774865480363,0.973774865480363,0.973774865480363,0.973774865480363,
0.973774865480363,0.973774865480363,0.973774865480363,0.973774865480363,
0.973774865480363,0.973774865480363,0.973774865480363,0.973774865480363,
0.973774865480363,0.973774865480363,0.973774865480363,0.973774865480363,
0.973774865480363,0.973774865480363,0.973774865480363,0.973774865480363,
0.973774865480363),(0.975309233263865,0.975309233263865,0.975309233263865,
0.975309233263865,0.975309233263865,0.975309233263865,0.975309233263865,
0.975309233263865,0.975309233263865,0.975309233263865,0.975309233263865,
0.975309233263865,0.975309233263865,0.975309233263865,0.975309233263865,
0.975309233263865,0.975309233263865,0.975309233263865,0.975309233263865,
0.975309233263865,0.975309233263865,0.975309233263865,0.975309233263865,
0.975309233263865,0.975309233263865,0.975309233263865,0.975309233263865,
0.975309233263865,0.975309233263865,0.975309233263865,0.975309233263865,
0.975309233263865,0.975309233263865),(1.0787447144153,1.0787447144153,1.0787447144153,
1.0787447144153,1.0787447144153,1.0787447144153,1.0787447144153,1.0787447144153,
1.0787447144153,1.0787447144153,1.0787447144153,1.0787447144153,1.0787447144153,
1.0787447144153,1.0787447144153,1.0787447144153,1.0787447144153,1.0787447144153,
1.0787447144153,1.0787447144153,1.0787447144153,1.0787447144153,1.0787447144153,
1.0787447144153,1.0787447144153,1.0787447144153,1.0787447144153,1.0787447144153,
1.0787447144153,1.0787447144153,1.0787447144153,1.0787447144153,1.0787447144153)))
REPRESENTATION_ITEM('')
SURFACE()
);
#225=(
BOUNDED_SURFACE()
B_SPLINE_SURFACE(3,3,((#47691,#47692,#47693,#47694,#47695,#47696,#47697,
#47698,#47699,#47700),(#47701,#47702,#47703,#47704,#47705,#47706,#47707,
#47708,#47709,#47710),(#47711,#47712,#47713,#47714,#47715,#47716,#47717,
#47718,#47719,#47720),(#47721,#47722,#47723,#47724,#47725,#47726,#47727,
#47728,#47729,#47730)),.UNSPECIFIED.,.F.,.F.,.F.)
B_SPLINE_SURFACE_WITH_KNOTS((4,4),(4,1,1,1,1,1,1,4),(0.0902161588351993,
0.903852934841359),(0.01134228752764,0.1428794983947,0.2858119429636,0.4286835294563,
0.5714929704347,0.7143131105204,0.8572933443558,0.9764111906647),
 .UNSPECIFIED.)
GEOMETRIC_REPRESENTATION_ITEM()
RATIONAL_B_SPLINE_SURFACE(((1.115479554767,1.115479554767,1.115479554767,
1.115479554767,1.115479554767,1.115479554767,1.115479554767,1.115479554767,
1.115479554767,1.115479554767),(0.96262105849538,0.96262105849538,0.96262105849538,
0.96262105849538,0.96262105849538,0.96262105849538,0.96262105849538,0.96262105849538,
0.96262105849538,0.96262105849538),(0.96151487844256,0.96151487844256,0.96151487844256,
0.96151487844256,0.96151487844256,0.96151487844256,0.96151487844256,0.96151487844256,
0.96151487844256,0.96151487844256),(1.11216101460854,1.11216101460854,1.11216101460854,
1.11216101460854,1.11216101460854,1.11216101460854,1.11216101460854,1.11216101460854,
1.11216101460854,1.11216101460854)))
REPRESENTATION_ITEM('')
SURFACE()
);
#226=(
BOUNDED_SURFACE()
B_SPLINE_SURFACE(3,3,((#47806,#47807,#47808,#47809,#47810,#47811,#47812,
#47813,#47814),(#47815,#47816,#47817,#47818,#47819,#47820,#47821,#47822,
#47823),(#47824,#47825,#47826,#47827,#47828,#47829,#47830,#47831,#47832),
(#47833,#47834,#47835,#47836,#47837,#47838,#47839,#47840,#47841)),
 .UNSPECIFIED.,.F.,.F.,.F.)
B_SPLINE_SURFACE_WITH_KNOTS((4,4),(4,1,1,1,1,1,4),(0.0546747561307775,0.945326746030744),
(0.22573546897307,0.241174738978,0.3599582619168,0.4768206617324,0.5903023688699,
0.699474730988,0.773102378452142),.UNSPECIFIED.)
GEOMETRIC_REPRESENTATION_ITEM()
RATIONAL_B_SPLINE_SURFACE(((1.19591932446267,1.19591932446267,1.19591932446267,
1.19591932446267,1.19591932446267,1.19591932446267,1.19591932446267,1.19591932446267,
1.19591932446267),(0.934693117931845,0.934693117931846,0.934693117931845,
0.934693117931845,0.934693117931845,0.934693117931845,0.934693117931845,
0.934693117931845,0.934693117931845),(0.934693558513152,0.934693558513152,
0.934693558513152,0.934693558513152,0.934693558513152,0.934693558513152,
0.934693558513152,0.934693558513152,0.934693558513152),(1.19592064620659,
1.19592064620659,1.19592064620659,1.19592064620659,1.19592064620659,1.19592064620659,
1.19592064620659,1.19592064620659,1.19592064620659)))
REPRESENTATION_ITEM('')
SURFACE()
);
#227=(
BOUNDED_SURFACE()
B_SPLINE_SURFACE(3,3,((#47899,#47900,#47901,#47902,#47903,#47904,#47905,
#47906,#47907),(#47908,#47909,#47910,#47911,#47912,#47913,#47914,#47915,
#47916),(#47917,#47918,#47919,#47920,#47921,#47922,#47923,#47924,#47925),
(#47926,#47927,#47928,#47929,#47930,#47931,#47932,#47933,#47934)),
 .UNSPECIFIED.,.F.,.F.,.F.)
B_SPLINE_SURFACE_WITH_KNOTS((4,4),(4,1,1,1,1,1,4),(0.0546340546499548,0.945366954784258),
(0.0404198562176404,0.1289115432366,0.2650470428868,0.4067050538029,0.552064790134,
0.7002092373436,0.711879622175772),.UNSPECIFIED.)
GEOMETRIC_REPRESENTATION_ITEM()
RATIONAL_B_SPLINE_SURFACE(((1.19595478336993,1.19595478336993,1.19595478336993,
1.19595478336993,1.19595478336993,1.19595478336993,1.19595478336993,1.19595478336993,
1.19595478336993),(0.934681442785239,0.934681442785239,0.934681442785239,
0.934681442785239,0.934681442785239,0.934681442785239,0.934681442785239,
0.934681442785239,0.934681442785239),(0.934681738876859,0.934681738876859,
0.93468173887686,0.934681738876859,0.934681738876859,0.934681738876859,
0.934681738876859,0.934681738876859,0.934681738876859),(1.19595567164479,
1.19595567164479,1.19595567164479,1.19595567164479,1.19595567164479,1.19595567164479,
1.19595567164479,1.19595567164479,1.19595567164479)))
REPRESENTATION_ITEM('')
SURFACE()
);
#228=(
BOUNDED_SURFACE()
B_SPLINE_SURFACE(3,3,((#48048,#48049,#48050,#48051,#48052,#48053,#48054,
#48055,#48056,#48057,#48058),(#48059,#48060,#48061,#48062,#48063,#48064,
#48065,#48066,#48067,#48068,#48069),(#48070,#48071,#48072,#48073,#48074,
#48075,#48076,#48077,#48078,#48079,#48080),(#48081,#48082,#48083,#48084,
#48085,#48086,#48087,#48088,#48089,#48090,#48091)),.UNSPECIFIED.,.F.,.F.,
 .F.)
B_SPLINE_SURFACE_WITH_KNOTS((4,4),(4,1,1,1,1,1,1,1,4),(0.075363327330941,
0.903974066580243),(-0.009670337409304,0.,0.1430996309434,0.2858291680282,
0.4284783625449,0.5715211775606,0.714546629698,0.8573667380228,0.9759160461734),
 .UNSPECIFIED.)
GEOMETRIC_REPRESENTATION_ITEM()
RATIONAL_B_SPLINE_SURFACE(((1.12354608686857,1.12354608686857,1.12354608686857,
1.12354608686857,1.12354608686857,1.12354608686857,1.12354608686857,1.12354608686857,
1.12354608686857,1.12354608686857,1.12354608686857),(0.962825764515366,
0.962825764515366,0.962825764515366,0.962825764515366,0.962825764515366,
0.962825764515366,0.962825764515366,0.962825764515366,0.962825764515366,
0.962825764515366,0.962825764515366),(0.958915479647154,0.958915479647154,
0.958915479647154,0.958915479647154,0.958915479647154,0.958915479647154,
0.958915479647154,0.958915479647154,0.958915479647154,0.958915479647154,
0.958915479647154),(1.11181523226393,1.11181523226393,1.11181523226393,
1.11181523226393,1.11181523226393,1.11181523226393,1.11181523226393,1.11181523226393,
1.11181523226393,1.11181523226393,1.11181523226393)))
REPRESENTATION_ITEM('')
SURFACE()
);
#229=(
BOUNDED_SURFACE()
B_SPLINE_SURFACE(3,3,((#48208,#48209,#48210,#48211),(#48212,#48213,#48214,
#48215),(#48216,#48217,#48218,#48219),(#48220,#48221,#48222,#48223)),
 .UNSPECIFIED.,.F.,.F.,.F.)
B_SPLINE_SURFACE_WITH_KNOTS((4,4),(4,4),(0.0986320319978618,0.901362552762759),
(-0.975145040400047,-0.0991746183719311),.UNSPECIFIED.)
GEOMETRIC_REPRESENTATION_ITEM()
RATIONAL_B_SPLINE_SURFACE(((1.17563600436588,1.17563600436588,1.17563600436588,
1.17563600436588),(0.941456244993756,0.941456244993756,0.941456244993756,
0.941456244993756),(0.941454665222131,0.941454665222131,0.941454665222131,
0.941454665222131),(1.175631265051,1.175631265051,1.175631265051,1.175631265051)))
REPRESENTATION_ITEM('')
SURFACE()
);
#230=(
BOUNDED_SURFACE()
B_SPLINE_SURFACE(3,3,((#48242,#48243,#48244,#48245,#48246,#48247,#48248,
#48249,#48250,#48251,#48252,#48253,#48254,#48255,#48256,#48257,#48258,#48259,
#48260,#48261,#48262,#48263,#48264,#48265,#48266,#48267,#48268,#48269,#48270,
#48271,#48272,#48273,#48274),(#48275,#48276,#48277,#48278,#48279,#48280,
#48281,#48282,#48283,#48284,#48285,#48286,#48287,#48288,#48289,#48290,#48291,
#48292,#48293,#48294,#48295,#48296,#48297,#48298,#48299,#48300,#48301,#48302,
#48303,#48304,#48305,#48306,#48307),(#48308,#48309,#48310,#48311,#48312,
#48313,#48314,#48315,#48316,#48317,#48318,#48319,#48320,#48321,#48322,#48323,
#48324,#48325,#48326,#48327,#48328,#48329,#48330,#48331,#48332,#48333,#48334,
#48335,#48336,#48337,#48338,#48339,#48340),(#48341,#48342,#48343,#48344,
#48345,#48346,#48347,#48348,#48349,#48350,#48351,#48352,#48353,#48354,#48355,
#48356,#48357,#48358,#48359,#48360,#48361,#48362,#48363,#48364,#48365,#48366,
#48367,#48368,#48369,#48370,#48371,#48372,#48373)),.UNSPECIFIED.,.F.,.F.,
 .F.)
B_SPLINE_SURFACE_WITH_KNOTS((4,4),(4,1,1,1,1,1,1,1,1,1,1,1,1,1,1,1,1,1,
1,1,1,1,1,1,1,1,1,1,1,1,4),(0.108373753360322,0.903586374444769),(-0.00973690174573,
0.,0.02218452663189,0.04657021466942,0.07320284553102,0.1023250304429,0.1343072162648,
0.1695983198482,0.2086109020835,0.2515270680609,0.2985674986552,0.3503233532582,
0.4076602728557,0.4682065066511,0.528219985243,0.5849729736978,0.6367746699729,
0.6825341132663,0.7235067267525,0.7605074035617,0.7940298126239,0.8241792004265,
0.851066626301,0.8750226986103,0.896463827273,0.9157957933363,0.9333740656998,
0.949358143999,0.9638586260694,0.9770542715531,0.9857155005292),
 .UNSPECIFIED.)
GEOMETRIC_REPRESENTATION_ITEM()
RATIONAL_B_SPLINE_SURFACE(((1.07414686918065,1.07414686918065,1.07414686918065,
1.07414686918065,1.07414686918065,1.07414686918065,1.07414686918065,1.07414686918065,
1.07414686918065,1.07414686918065,1.07414686918065,1.07414686918065,1.07414686918065,
1.07414686918065,1.07414686918065,1.07414686918065,1.07414686918065,1.07414686918065,
1.07414686918065,1.07414686918065,1.07414686918065,1.07414686918065,1.07414686918065,
1.07414686918065,1.07414686918065,1.07414686918065,1.07414686918065,1.07414686918065,
1.07414686918065,1.07414686918065,1.07414686918065,1.07414686918065,1.07414686918065),
(0.973774764072452,0.973774764072452,0.973774764072452,0.973774764072452,
0.973774764072452,0.973774764072452,0.973774764072452,0.973774764072452,
0.973774764072452,0.973774764072452,0.973774764072452,0.973774764072452,
0.973774764072452,0.973774764072452,0.973774764072452,0.973774764072452,
0.973774764072452,0.973774764072452,0.973774764072452,0.973774764072452,
0.973774764072452,0.973774764072452,0.973774764072452,0.973774764072452,
0.973774764072452,0.973774764072452,0.973774764072452,0.973774764072452,
0.973774764072452,0.973774764072452,0.973774764072452,0.973774764072452,
0.973774764072452),(0.975307428462876,0.975307428462876,0.975307428462876,
0.975307428462876,0.975307428462876,0.975307428462876,0.975307428462876,
0.975307428462876,0.975307428462876,0.975307428462876,0.975307428462876,
0.975307428462876,0.975307428462876,0.975307428462876,0.975307428462876,
0.975307428462876,0.975307428462876,0.975307428462876,0.975307428462876,
0.975307428462876,0.975307428462876,0.975307428462876,0.975307428462876,
0.975307428462876,0.975307428462876,0.975307428462876,0.975307428462876,
0.975307428462876,0.975307428462876,0.975307428462876,0.975307428462876,
0.975307428462876,0.975307428462876),(1.07874486235192,1.07874486235192,
1.07874486235192,1.07874486235192,1.07874486235192,1.07874486235192,1.07874486235192,
1.07874486235192,1.07874486235192,1.07874486235192,1.07874486235192,1.07874486235192,
1.07874486235192,1.07874486235192,1.07874486235192,1.07874486235192,1.07874486235192,
1.07874486235192,1.07874486235192,1.07874486235192,1.07874486235192,1.07874486235192,
1.07874486235192,1.07874486235192,1.07874486235192,1.07874486235192,1.07874486235192,
1.07874486235192,1.07874486235192,1.07874486235192,1.07874486235192,1.07874486235192,
1.07874486235192)))
REPRESENTATION_ITEM('')
SURFACE()
);
#231=(
BOUNDED_SURFACE()
B_SPLINE_SURFACE(3,3,((#48758,#48759,#48760,#48761,#48762,#48763,#48764,
#48765,#48766,#48767,#48768,#48769,#48770),(#48771,#48772,#48773,#48774,
#48775,#48776,#48777,#48778,#48779,#48780,#48781,#48782,#48783),(#48784,
#48785,#48786,#48787,#48788,#48789,#48790,#48791,#48792,#48793,#48794,#48795,
#48796),(#48797,#48798,#48799,#48800,#48801,#48802,#48803,#48804,#48805,
#48806,#48807,#48808,#48809)),.UNSPECIFIED.,.F.,.F.,.F.)
B_SPLINE_SURFACE_WITH_KNOTS((4,4),(4,1,1,1,1,1,1,1,1,1,4),(0.0574231646653068,
0.945306788892276),(0.1309905936005,0.1664977910666,0.2356164564824,0.3128428890291,
0.4007505433904,0.5000361747357,0.5993121726045,0.6872040763411,0.7644181606731,
0.8335262268397,0.8690088218608),.UNSPECIFIED.)
GEOMETRIC_REPRESENTATION_ITEM()
RATIONAL_B_SPLINE_SURFACE(((1.19350274020032,1.19350274020032,1.19350274020032,
1.19350274020032,1.19350274020032,1.19350274020032,1.19350274020032,1.19350274020032,
1.19350274020032,1.19350274020032,1.19350274020032,1.19350274020032,1.19350274020032),
(0.934703362630941,0.934703362630941,0.934703362630941,0.934703362630941,
0.934703362630941,0.934703362630941,0.934703362630941,0.934703362630941,
0.934703362630941,0.934703362630941,0.934703362630941,0.934703362630941,
0.934703362630941),(0.935501540738208,0.935501540738208,0.935501540738208,
0.935501540738208,0.935501540738208,0.935501540738208,0.935501540738208,
0.935501540738208,0.935501540738208,0.935501540738208,0.935501540738208,
0.935501540738208,0.935501540738208),(1.19589727452213,1.19589727452213,
1.19589727452213,1.19589727452213,1.19589727452213,1.19589727452213,1.19589727452213,
1.19589727452213,1.19589727452213,1.19589727452213,1.19589727452213,1.19589727452213,
1.19589727452213)))
REPRESENTATION_ITEM('')
SURFACE()
);
#232=(
BOUNDED_SURFACE()
B_SPLINE_SURFACE(3,3,((#48921,#48922,#48923,#48924,#48925,#48926,#48927,
#48928,#48929),(#48930,#48931,#48932,#48933,#48934,#48935,#48936,#48937,
#48938),(#48939,#48940,#48941,#48942,#48943,#48944,#48945,#48946,#48947),
(#48948,#48949,#48950,#48951,#48952,#48953,#48954,#48955,#48956)),
 .UNSPECIFIED.,.F.,.F.,.F.)
B_SPLINE_SURFACE_WITH_KNOTS((4,4),(4,1,1,1,1,1,4),(0.0546972932257005,0.945304219631693),
(0.286889171703242,0.3000858921602,0.4481462942066,0.5934294748234,0.7350160218511,
0.8711055251025,0.961148082229091),.UNSPECIFIED.)
GEOMETRIC_REPRESENTATION_ITEM()
RATIONAL_B_SPLINE_SURFACE(((1.19590004288633,1.19590004288633,1.19590004288633,
1.19590004288633,1.19590004288633,1.19590004288633,1.19590004288633,1.19590004288633,
1.19590004288633),(0.934699542008166,0.934699542008166,0.934699542008166,
0.934699542008166,0.934699542008166,0.934699542008166,0.934699542008166,
0.934699542008166,0.934699542008166),(0.934699985705345,0.934699985705345,
0.934699985705345,0.934699985705345,0.934699985705345,0.934699985705345,
0.934699985705345,0.934699985705345,0.934699985705345),(1.19590137397786,
1.19590137397786,1.19590137397786,1.19590137397786,1.19590137397786,1.19590137397786,
1.19590137397786,1.19590137397786,1.19590137397786)))
REPRESENTATION_ITEM('')
SURFACE()
);
#233=(
BOUNDED_SURFACE()
B_SPLINE_SURFACE(3,3,((#49070,#49071,#49072,#49073,#49074,#49075,#49076,
#49077,#49078,#49079),(#49080,#49081,#49082,#49083,#49084,#49085,#49086,
#49087,#49088,#49089),(#49090,#49091,#49092,#49093,#49094,#49095,#49096,
#49097,#49098,#49099),(#49100,#49101,#49102,#49103,#49104,#49105,#49106,
#49107,#49108,#49109)),.UNSPECIFIED.,.F.,.F.,.F.)
B_SPLINE_SURFACE_WITH_KNOTS((4,4),(4,1,1,1,1,1,1,4),(0.0902165725701947,
0.904252559393621),(0.0113422875341,0.1428793759885,0.285811601384,0.4286834096628,
0.5714931672581,0.7143130821911,0.8572933140146,0.9764111906785),
 .UNSPECIFIED.)
GEOMETRIC_REPRESENTATION_ITEM()
RATIONAL_B_SPLINE_SURFACE(((1.11547932157709,1.11547932157709,1.11547932157709,
1.11547932157709,1.11547932157709,1.11547932157709,1.11547932157709,1.11547932157709,
1.11547932157709,1.11547932157709),(0.962545979710326,0.962545979710326,
0.962545979710326,0.962545979710326,0.962545979710326,0.962545979710326,
0.962545979710326,0.962545979710326,0.962545979710326,0.962545979710326),
(0.961513905112406,0.961513905112406,0.961513905112406,0.961513905112406,
0.961513905112406,0.961513905112406,0.961513905112406,0.961513905112406,
0.961513905112406,0.961513905112406),(1.11238309778333,1.11238309778333,
1.11238309778333,1.11238309778333,1.11238309778333,1.11238309778333,1.11238309778333,
1.11238309778333,1.11238309778333,1.11238309778333)))
REPRESENTATION_ITEM('')
SURFACE()
);
#234=(
BOUNDED_SURFACE()
B_SPLINE_SURFACE(3,3,((#49136,#49137,#49138,#49139,#49140,#49141,#49142,
#49143,#49144),(#49145,#49146,#49147,#49148,#49149,#49150,#49151,#49152,
#49153),(#49154,#49155,#49156,#49157,#49158,#49159,#49160,#49161,#49162),
(#49163,#49164,#49165,#49166,#49167,#49168,#49169,#49170,#49171)),
 .UNSPECIFIED.,.F.,.F.,.F.)
B_SPLINE_SURFACE_WITH_KNOTS((4,4),(4,1,1,1,1,1,4),(0.0547421202676084,0.945259392236121),
(0.038975628375885,0.1288834130457,0.26496497341,0.4065466125696,0.5518231987718,
0.6998761197252,0.71318036205432),.UNSPECIFIED.)
GEOMETRIC_REPRESENTATION_ITEM()
RATIONAL_B_SPLINE_SURFACE(((1.19586062030508,1.19586062030508,1.19586062030508,
1.19586062030508,1.19586062030508,1.19586062030508,1.19586062030508,1.19586062030508,
1.19586062030508),(0.934712683016858,0.934712683016858,0.934712683016858,
0.934712683016858,0.934712683016858,0.934712683016858,0.934712683016858,
0.934712683016858,0.934712683016858),(0.934713126565695,0.934713126565695,
0.934713126565695,0.934713126565695,0.934713126565695,0.934713126565695,
0.934713126565695,0.934713126565695,0.934713126565695),(1.19586195095159,
1.19586195095159,1.19586195095159,1.19586195095159,1.19586195095159,1.19586195095159,
1.19586195095159,1.19586195095159,1.19586195095159)))
REPRESENTATION_ITEM('')
SURFACE()
);
#235=(
BOUNDED_SURFACE()
B_SPLINE_SURFACE(3,3,((#49285,#49286,#49287,#49288,#49289,#49290,#49291,
#49292,#49293,#49294),(#49295,#49296,#49297,#49298,#49299,#49300,#49301,
#49302,#49303,#49304),(#49305,#49306,#49307,#49308,#49309,#49310,#49311,
#49312,#49313,#49314),(#49315,#49316,#49317,#49318,#49319,#49320,#49321,
#49322,#49323,#49324)),.UNSPECIFIED.,.F.,.F.,.F.)
B_SPLINE_SURFACE_WITH_KNOTS((4,4),(4,1,1,1,1,1,1,4),(0.0902480906385812,
0.904266113670097),(0.02358777780563,0.1427066860199,0.2856869176887,0.4285068315006,
0.5713165915697,0.7141884014049,0.8571206249672,0.9886565450657),
 .UNSPECIFIED.)
GEOMETRIC_REPRESENTATION_ITEM()
RATIONAL_B_SPLINE_SURFACE(((1.11546155940106,1.11546155940106,1.11546155940106,
1.11546155940106,1.11546155940106,1.11546155940106,1.11546155940106,1.11546155940106,
1.11546155940106,1.11546155940106),(0.962543353412622,0.962543353412622,
0.962543353412622,0.962543353412622,0.962543353412622,0.962543353412622,
0.962543353412622,0.962543353412622,0.962543353412622,0.962543353412622),
(0.961519712013558,0.961519712013558,0.961519712013558,0.961519712013558,
0.961519712013558,0.961519712013558,0.961519712013558,0.961519712013558,
0.961519712013558,0.961519712013558),(1.11239063520387,1.11239063520387,
1.11239063520387,1.11239063520387,1.11239063520387,1.11239063520387,1.11239063520387,
1.11239063520387,1.11239063520387,1.11239063520387)))
REPRESENTATION_ITEM('')
SURFACE()
);
#236=(
BOUNDED_SURFACE()
B_SPLINE_SURFACE(3,3,((#49364,#49365,#49366,#49367,#49368,#49369),(#49370,
#49371,#49372,#49373,#49374,#49375),(#49376,#49377,#49378,#49379,#49380,
#49381),(#49382,#49383,#49384,#49385,#49386,#49387)),.UNSPECIFIED.,.F.,
 .F.,.F.)
B_SPLINE_SURFACE_WITH_KNOTS((4,4),(4,1,1,4),(0.0986342191388939,0.901369960074243),
(0.317543733191689,0.3333147448852,0.6666852551147,0.682456266808865),
 .UNSPECIFIED.)
GEOMETRIC_REPRESENTATION_ITEM()
RATIONAL_B_SPLINE_SURFACE(((1.17563408853197,1.17563408853197,1.17563408853197,
1.17563408853197,1.17563408853197,1.17563408853197),(0.941454084631828,
0.941454084631828,0.941454084631828,0.941454084631828,0.941454084631828,
0.941454084631828),(0.941455303829123,0.941455303829123,0.941455303829123,
0.941455303829123,0.941455303829123,0.941455303829123),(1.17563774612386,
1.17563774612386,1.17563774612386,1.17563774612386,1.17563774612386,1.17563774612386)))
REPRESENTATION_ITEM('')
SURFACE()
);
#237=(
BOUNDED_SURFACE()
B_SPLINE_SURFACE(3,3,((#49627,#49628,#49629,#49630,#49631,#49632,#49633,
#49634,#49635,#49636,#49637,#49638,#49639,#49640,#49641,#49642,#49643,#49644,
#49645,#49646,#49647,#49648,#49649,#49650,#49651,#49652,#49653,#49654,#49655,
#49656,#49657,#49658,#49659,#49660,#49661,#49662,#49663,#49664,#49665,#49666),
(#49667,#49668,#49669,#49670,#49671,#49672,#49673,#49674,#49675,#49676,
#49677,#49678,#49679,#49680,#49681,#49682,#49683,#49684,#49685,#49686,#49687,
#49688,#49689,#49690,#49691,#49692,#49693,#49694,#49695,#49696,#49697,#49698,
#49699,#49700,#49701,#49702,#49703,#49704,#49705,#49706),(#49707,#49708,
#49709,#49710,#49711,#49712,#49713,#49714,#49715,#49716,#49717,#49718,#49719,
#49720,#49721,#49722,#49723,#49724,#49725,#49726,#49727,#49728,#49729,#49730,
#49731,#49732,#49733,#49734,#49735,#49736,#49737,#49738,#49739,#49740,#49741,
#49742,#49743,#49744,#49745,#49746),(#49747,#49748,#49749,#49750,#49751,
#49752,#49753,#49754,#49755,#49756,#49757,#49758,#49759,#49760,#49761,#49762,
#49763,#49764,#49765,#49766,#49767,#49768,#49769,#49770,#49771,#49772,#49773,
#49774,#49775,#49776,#49777,#49778,#49779,#49780,#49781,#49782,#49783,#49784,
#49785,#49786)),.UNSPECIFIED.,.F.,.F.,.F.)
B_SPLINE_SURFACE_WITH_KNOTS((4,4),(4,1,1,1,1,1,1,1,1,1,1,1,1,1,1,1,1,1,
1,1,1,1,1,1,1,1,1,1,1,1,1,1,1,1,1,1,1,4),(0.109557513697332,0.88523983460631),
(-0.009601789277903,0.,0.02232873710628,0.04690611139379,0.07379420329328,
0.1032833799132,0.1358151932356,0.1719129234016,0.2120200511384,0.2562537498977,
0.3048223338256,0.3583884089718,0.4161300533589,0.4734080944977,0.5265789086099,
0.5739168290462,0.615519134979,0.652991960542,0.6871390289507,0.7180225588761,
0.7460350579758,0.7715291821123,0.7947418182217,0.8158398112656,0.8349884136664,
0.8523604287723,0.8681387312846,0.8825028670571,0.8956298657939,0.9076956876584,
0.9188457170059,0.9291453143216,0.9386431055222,0.9473856329388,0.9554251084374,
0.9628149684932,0.9696055559494,0.9720662896547),.UNSPECIFIED.)
GEOMETRIC_REPRESENTATION_ITEM()
RATIONAL_B_SPLINE_SURFACE(((1.0736979416248,1.0736979416248,1.0736979416248,
1.0736979416248,1.0736979416248,1.0736979416248,1.0736979416248,1.0736979416248,
1.0736979416248,1.0736979416248,1.0736979416248,1.0736979416248,1.0736979416248,
1.0736979416248,1.0736979416248,1.0736979416248,1.0736979416248,1.0736979416248,
1.0736979416248,1.0736979416248,1.0736979416248,1.0736979416248,1.0736979416248,
1.0736979416248,1.0736979416248,1.0736979416248,1.0736979416248,1.0736979416248,
1.0736979416248,1.0736979416248,1.0736979416248,1.0736979416248,1.0736979416248,
1.0736979416248,1.0736979416248,1.0736979416248,1.0736979416248,1.0736979416248,
1.0736979416248,1.0736979416248),(0.976088703540388,0.976088703540388,0.976088703540388,
0.976088703540388,0.976088703540388,0.976088703540388,0.976088703540388,
0.976088703540388,0.976088703540388,0.976088703540388,0.976088703540388,
0.976088703540388,0.976088703540388,0.976088703540388,0.976088703540388,
0.976088703540388,0.976088703540388,0.976088703540388,0.976088703540388,
0.976088703540388,0.976088703540388,0.976088703540388,0.976088703540388,
0.976088703540388,0.976088703540388,0.976088703540388,0.976088703540388,
0.976088703540388,0.976088703540388,0.976088703540388,0.976088703540388,
0.976088703540388,0.976088703540388,0.976088703540388,0.976088703540388,
0.976088703540388,0.976088703540388,0.976088703540388,0.976088703540388,
0.976088703540388),(0.975438381295863,0.975438381295863,0.975438381295863,
0.975438381295863,0.975438381295863,0.975438381295863,0.975438381295863,
0.975438381295863,0.975438381295863,0.975438381295863,0.975438381295863,
0.975438381295863,0.975438381295863,0.975438381295863,0.975438381295863,
0.975438381295863,0.975438381295863,0.975438381295863,0.975438381295863,
0.975438381295863,0.975438381295863,0.975438381295863,0.975438381295863,
0.975438381295863,0.975438381295863,0.975438381295863,0.975438381295863,
0.975438381295863,0.975438381295863,0.975438381295863,0.975438381295863,
0.975438381295863,0.975438381295863,0.975438381295863,0.975438381295863,
0.975438381295863,0.975438381295863,0.975438381295863,0.975438381295863,
0.975438381295863),(1.07174697489122,1.07174697489122,1.07174697489122,
1.07174697489122,1.07174697489122,1.07174697489122,1.07174697489122,1.07174697489122,
1.07174697489122,1.07174697489122,1.07174697489122,1.07174697489122,1.07174697489122,
1.07174697489122,1.07174697489122,1.07174697489122,1.07174697489122,1.07174697489122,
1.07174697489122,1.07174697489122,1.07174697489122,1.07174697489122,1.07174697489122,
1.07174697489122,1.07174697489122,1.07174697489122,1.07174697489122,1.07174697489122,
1.07174697489122,1.07174697489122,1.07174697489122,1.07174697489122,1.07174697489122,
1.07174697489122,1.07174697489122,1.07174697489122,1.07174697489122,1.07174697489122,
1.07174697489122,1.07174697489122)))
REPRESENTATION_ITEM('')
SURFACE()
);
#238=(
BOUNDED_SURFACE()
B_SPLINE_SURFACE(3,3,((#49912,#49913,#49914,#49915,#49916,#49917,#49918,
#49919,#49920),(#49921,#49922,#49923,#49924,#49925,#49926,#49927,#49928,
#49929),(#49930,#49931,#49932,#49933,#49934,#49935,#49936,#49937,#49938),
(#49939,#49940,#49941,#49942,#49943,#49944,#49945,#49946,#49947)),
 .UNSPECIFIED.,.F.,.F.,.F.)
B_SPLINE_SURFACE_WITH_KNOTS((4,4),(4,1,1,1,1,1,4),(0.0546349420399352,0.945366895174421),
(0.288003830103446,0.2998193985502,0.4479601517394,0.5933162069375,0.7349712858318,
0.871099664451,0.959211435602542),.UNSPECIFIED.)
GEOMETRIC_REPRESENTATION_ITEM()
RATIONAL_B_SPLINE_SURFACE(((1.19595529172475,1.19595529172475,1.19595529172475,
1.19595529172475,1.19595529172475,1.19595529172475,1.19595529172475,1.19595529172475,
1.19595529172475),(0.93468103052344,0.93468103052344,0.93468103052344,0.93468103052344,
0.93468103052344,0.93468103052344,0.93468103052344,0.93468103052344,0.93468103052344),
(0.934681569426094,0.934681569426094,0.934681569426094,0.934681569426094,
0.934681569426094,0.934681569426094,0.934681569426094,0.934681569426094,
0.934681569426094),(1.19595690843272,1.19595690843272,1.19595690843272,
1.19595690843272,1.19595690843272,1.19595690843272,1.19595690843272,1.19595690843272,
1.19595690843272)))
REPRESENTATION_ITEM('')
SURFACE()
);
#239=(
BOUNDED_SURFACE()
B_SPLINE_SURFACE(3,3,((#50064,#50065,#50066,#50067,#50068,#50069,#50070,
#50071,#50072,#50073),(#50074,#50075,#50076,#50077,#50078,#50079,#50080,
#50081,#50082,#50083),(#50084,#50085,#50086,#50087,#50088,#50089,#50090,
#50091,#50092,#50093),(#50094,#50095,#50096,#50097,#50098,#50099,#50100,
#50101,#50102,#50103)),.UNSPECIFIED.,.F.,.F.,.F.)
B_SPLINE_SURFACE_WITH_KNOTS((4,4),(4,1,1,1,1,1,1,4),(0.0897027042850842,
0.903974528617832),(0.02295305876273,0.1427319133548,0.2857218418975,0.4285793286892,
0.5713517372348,0.7142096687795,0.8572807309771,0.9622634166072),
 .UNSPECIFIED.)
GEOMETRIC_REPRESENTATION_ITEM()
RATIONAL_B_SPLINE_SURFACE(((1.11534309040735,1.11534309040735,1.11534309040735,
1.11534309040735,1.11534309040735,1.11534309040735,1.11534309040735,1.11534309040735,
1.11534309040735,1.11534309040735),(0.962737277287542,0.962737277287542,
0.962737277287542,0.962737277287542,0.962737277287542,0.962737277287542,
0.962737277287542,0.962737277287542,0.962737277287542,0.962737277287542),
(0.961561433546803,0.961561433546803,0.961561433546803,0.961561433546803,
0.961561433546803,0.961561433546803,0.961561433546803,0.961561433546803,
0.961561433546803,0.961561433546803),(1.11181555918513,1.11181555918513,
1.11181555918513,1.11181555918513,1.11181555918513,1.11181555918513,1.11181555918513,
1.11181555918513,1.11181555918513,1.11181555918513)))
REPRESENTATION_ITEM('')
SURFACE()
);
#240=(
BOUNDED_SURFACE()
B_SPLINE_SURFACE(3,3,((#50322,#50323,#50324,#50325,#50326,#50327,#50328,
#50329,#50330,#50331,#50332,#50333,#50334),(#50335,#50336,#50337,#50338,
#50339,#50340,#50341,#50342,#50343,#50344,#50345,#50346,#50347),(#50348,
#50349,#50350,#50351,#50352,#50353,#50354,#50355,#50356,#50357,#50358,#50359,
#50360),(#50361,#50362,#50363,#50364,#50365,#50366,#50367,#50368,#50369,
#50370,#50371,#50372,#50373)),.UNSPECIFIED.,.F.,.F.,.F.)
B_SPLINE_SURFACE_WITH_KNOTS((4,4),(4,1,1,1,1,1,1,1,1,1,4),(0.0573922460373052,
0.945244139733566),(0.1310483619551,0.1664290842009,0.2355281267714,0.3127253439453,
0.4006209236964,0.4999619679894,0.5993131607486,0.6872253246198,0.7644355181441,
0.8335456904892,0.8689506588994),.UNSPECIFIED.)
GEOMETRIC_REPRESENTATION_ITEM()
RATIONAL_B_SPLINE_SURFACE(((1.19353001815818,1.19353001815818,1.19353001815818,
1.19353001815818,1.19353001815818,1.19353001815818,1.19353001815818,1.19353001815818,
1.19353001815818,1.19353001815818,1.19353001815818,1.19353001815818,1.19353001815818),
(0.934721488377597,0.934721488377597,0.934721488377597,0.934721488377597,
0.934721488377597,0.934721488377597,0.934721488377597,0.934721488377597,
0.934721488377597,0.934721488377597,0.934721488377597,0.934721488377597,
0.934721488377597),(0.935492282742568,0.935492282742568,0.935492282742568,
0.935492282742568,0.935492282742568,0.935492282742568,0.935492282742568,
0.935492282742568,0.935492282742568,0.935492282742568,0.935492282742568,
0.935492282742568,0.935492282742568),(1.19584240125309,1.19584240125309,
1.19584240125309,1.19584240125309,1.19584240125309,1.19584240125309,1.19584240125309,
1.19584240125309,1.19584240125309,1.19584240125309,1.19584240125309,1.19584240125309,
1.19584240125309)))
REPRESENTATION_ITEM('')
SURFACE()
);
#241=(
BOUNDED_SURFACE()
B_SPLINE_SURFACE(2,2,((#50483,#50484,#50485),(#50486,#50487,#50488),(#50489,
#50490,#50491)),.UNSPECIFIED.,.F.,.F.,.F.)
B_SPLINE_SURFACE_WITH_KNOTS((3,3),(3,3),(-0.384396778003823,0.384396780054855),
(0.714171252135544,1.38022246560866),.UNSPECIFIED.)
GEOMETRIC_REPRESENTATION_ITEM()
RATIONAL_B_SPLINE_SURFACE(((1.,0.945057588082017,1.),(0.92702480918682,
0.876091830262289,0.92702480918682),(1.,0.945057588082017,1.)))
REPRESENTATION_ITEM('')
SURFACE()
);
#242=(
BOUNDED_SURFACE()
B_SPLINE_SURFACE(2,2,((#50597,#50598,#50599),(#50600,#50601,#50602),(#50603,
#50604,#50605)),.UNSPECIFIED.,.F.,.F.,.F.)
B_SPLINE_SURFACE_WITH_KNOTS((3,3),(3,3),(-0.384396778088211,0.384396780096543),
(1.76137009171851,2.42742001680813),.UNSPECIFIED.)
GEOMETRIC_REPRESENTATION_ITEM()
RATIONAL_B_SPLINE_SURFACE(((1.,0.945057798670611,1.),(0.927024809163182,
0.8760920254608,0.927024809163182),(1.,0.945057798670611,1.)))
REPRESENTATION_ITEM('')
SURFACE()
);
#243=(
BOUNDED_SURFACE()
B_SPLINE_SURFACE(2,2,((#50608,#50609,#50610),(#50611,#50612,#50613),(#50614,
#50615,#50616)),.UNSPECIFIED.,.F.,.F.,.F.)
B_SPLINE_SURFACE_WITH_KNOTS((3,3),(3,3),(-0.384396778254674,0.384396780219765),
(-0.333024963743409,0.33302496374341),.UNSPECIFIED.)
GEOMETRIC_REPRESENTATION_ITEM()
RATIONAL_B_SPLINE_SURFACE(((1.,0.945057798278785,1.),(0.927024809108865,
0.876092025046235,0.927024809108865),(1.,0.945057798278785,1.)))
REPRESENTATION_ITEM('')
SURFACE()
);
#244=(
BOUNDED_SURFACE()
B_SPLINE_SURFACE(2,2,((#50619,#50620,#50621),(#50622,#50623,#50624),(#50625,
#50626,#50627)),.UNSPECIFIED.,.F.,.F.,.F.)
B_SPLINE_SURFACE_WITH_KNOTS((3,3),(3,3),(-0.384396778076674,0.384396780107987),
(-2.42742011306213,-1.76137023584075),.UNSPECIFIED.)
GEOMETRIC_REPRESENTATION_ITEM()
RATIONAL_B_SPLINE_SURFACE(((1.,0.945057806494753,1.),(0.927024809163199,
0.87609203271399,0.927024809163199),(1.,0.945057806494753,1.)))
REPRESENTATION_ITEM('')
SURFACE()
);
#245=(
BOUNDED_SURFACE()
B_SPLINE_SURFACE(2,2,((#50630,#50631,#50632),(#50633,#50634,#50635),(#50636,
#50637,#50638)),.UNSPECIFIED.,.F.,.F.,.F.)
B_SPLINE_SURFACE_WITH_KNOTS((3,3),(3,3),(-0.384396775432716,0.384396776804917),
(-1.38022383251571,-0.714172862049472),.UNSPECIFIED.)
GEOMETRIC_REPRESENTATION_ITEM()
RATIONAL_B_SPLINE_SURFACE(((1.,0.945057627801957,1.),(0.927024810278266,
0.876091868115137,0.927024810278266),(1.,0.945057627801957,1.)))
REPRESENTATION_ITEM('')
SURFACE()
);
#246=(
BOUNDED_SURFACE()
B_SPLINE_SURFACE(2,2,((#50641,#50642,#50643),(#50644,#50645,#50646),(#50647,
#50648,#50649)),.UNSPECIFIED.,.F.,.F.,.F.)
B_SPLINE_SURFACE_WITH_KNOTS((3,3),(3,3),(-0.384396777981939,0.384396780078218),
(-0.333024791636522,0.333024914411102),.UNSPECIFIED.)
GEOMETRIC_REPRESENTATION_ITEM()
RATIONAL_B_SPLINE_SURFACE(((1.,0.945057834473379,1.),(0.927024809186542,
0.876092058672931,0.927024809186542),(1.,0.945057834473379,1.)))
REPRESENTATION_ITEM('')
SURFACE()
);
#247=(
BOUNDED_SURFACE()
B_SPLINE_SURFACE(3,3,((#50680,#50681,#50682,#50683,#50684,#50685),(#50686,
#50687,#50688,#50689,#50690,#50691),(#50692,#50693,#50694,#50695,#50696,
#50697),(#50698,#50699,#50700,#50701,#50702,#50703)),.UNSPECIFIED.,.F.,
 .F.,.F.)
B_SPLINE_SURFACE_WITH_KNOTS((4,4),(4,1,1,4),(0.0986342191388488,0.901369960096482),
(0.317543733191041,0.3333147448853,0.6666852551147,0.682456266810084),
 .UNSPECIFIED.)
GEOMETRIC_REPRESENTATION_ITEM()
RATIONAL_B_SPLINE_SURFACE(((1.17563408853201,1.17563408853201,1.17563408853201,
1.17563408853201,1.17563408853201,1.17563408853201),(0.94145408462534,0.94145408462534,
0.94145408462534,0.94145408462534,0.94145408462534,0.94145408462534),(0.941455303829109,
0.941455303829109,0.941455303829109,0.941455303829109,0.941455303829109,
0.941455303829109),(1.17563774614332,1.17563774614332,1.17563774614332,
1.17563774614332,1.17563774614332,1.17563774614332)))
REPRESENTATION_ITEM('')
SURFACE()
);
#248=(
BOUNDED_SURFACE()
B_SPLINE_SURFACE(3,3,((#50930,#50931,#50932,#50933,#50934,#50935,#50936,
#50937,#50938,#50939,#50940,#50941,#50942,#50943,#50944,#50945,#50946,#50947,
#50948,#50949,#50950,#50951,#50952,#50953,#50954,#50955,#50956,#50957,#50958,
#50959,#50960,#50961,#50962,#50963,#50964,#50965,#50966,#50967,#50968,#50969),
(#50970,#50971,#50972,#50973,#50974,#50975,#50976,#50977,#50978,#50979,
#50980,#50981,#50982,#50983,#50984,#50985,#50986,#50987,#50988,#50989,#50990,
#50991,#50992,#50993,#50994,#50995,#50996,#50997,#50998,#50999,#51000,#51001,
#51002,#51003,#51004,#51005,#51006,#51007,#51008,#51009),(#51010,#51011,
#51012,#51013,#51014,#51015,#51016,#51017,#51018,#51019,#51020,#51021,#51022,
#51023,#51024,#51025,#51026,#51027,#51028,#51029,#51030,#51031,#51032,#51033,
#51034,#51035,#51036,#51037,#51038,#51039,#51040,#51041,#51042,#51043,#51044,
#51045,#51046,#51047,#51048,#51049),(#51050,#51051,#51052,#51053,#51054,
#51055,#51056,#51057,#51058,#51059,#51060,#51061,#51062,#51063,#51064,#51065,
#51066,#51067,#51068,#51069,#51070,#51071,#51072,#51073,#51074,#51075,#51076,
#51077,#51078,#51079,#51080,#51081,#51082,#51083,#51084,#51085,#51086,#51087,
#51088,#51089)),.UNSPECIFIED.,.F.,.F.,.F.)
B_SPLINE_SURFACE_WITH_KNOTS((4,4),(4,1,1,1,1,1,1,1,1,1,1,1,1,1,1,1,1,1,
1,1,1,1,1,1,1,1,1,1,1,1,1,1,1,1,1,1,1,4),(0.109557826006967,0.885251264281302),
(-0.009601789265348,0.,0.02232759876008,0.04690438428648,0.07379256313311,
0.1032821525075,0.1358145488879,0.1719130282207,0.2120212567498,0.2562571680312,
0.304829894919,0.3584023230986,0.416146088449,0.4734208057249,0.5265860543759,
0.5739192804694,0.6155188222685,0.6529897830592,0.6871354795221,0.7180181888986,
0.7460302867701,0.7715243416762,0.7947371788921,0.8158355553727,0.8349846338425,
0.8523571535141,0.8681359777133,0.8825006466294,0.8956281837449,0.9076945427548,
0.9188451048053,0.9291452127891,0.9386434680718,0.9473863882147,0.9554261628483,
0.9628162067304,0.9696068473725,0.972066289545),.UNSPECIFIED.)
GEOMETRIC_REPRESENTATION_ITEM()
RATIONAL_B_SPLINE_SURFACE(((1.07369782373338,1.07369782373338,1.07369782373338,
1.07369782373338,1.07369782373338,1.07369782373338,1.07369782373338,1.07369782373338,
1.07369782373338,1.07369782373338,1.07369782373338,1.07369782373338,1.07369782373338,
1.07369782373338,1.07369782373338,1.07369782373338,1.07369782373338,1.07369782373338,
1.07369782373338,1.07369782373338,1.07369782373338,1.07369782373338,1.07369782373338,
1.07369782373338,1.07369782373338,1.07369782373338,1.07369782373338,1.07369782373338,
1.07369782373338,1.07369782373338,1.07369782373338,1.07369782373338,1.07369782373338,
1.07369782373338,1.07369782373338,1.07369782373338,1.07369782373338,1.07369782373338,
1.07369782373338,1.07369782373338),(0.976087264743372,0.976087264743372,
0.976087264743372,0.976087264743372,0.976087264743372,0.976087264743372,
0.976087264743372,0.976087264743372,0.976087264743372,0.976087264743372,
0.976087264743372,0.976087264743372,0.976087264743372,0.976087264743372,
0.976087264743372,0.976087264743372,0.976087264743372,0.976087264743372,
0.976087264743372,0.976087264743372,0.976087264743372,0.976087264743372,
0.976087264743372,0.976087264743372,0.976087264743372,0.976087264743372,
0.976087264743372,0.976087264743372,0.976087264743372,0.976087264743372,
0.976087264743372,0.976087264743372,0.976087264743372,0.976087264743372,
0.976087264743372,0.976087264743372,0.976087264743372,0.976087264743372,
0.976087264743372,0.976087264743372),(0.975438400926425,0.975438400926425,
0.975438400926425,0.975438400926425,0.975438400926425,0.975438400926425,
0.975438400926425,0.975438400926425,0.975438400926425,0.975438400926425,
0.975438400926425,0.975438400926425,0.975438400926425,0.975438400926425,
0.975438400926425,0.975438400926425,0.975438400926425,0.975438400926425,
0.975438400926425,0.975438400926425,0.975438400926425,0.975438400926425,
0.975438400926425,0.975438400926425,0.975438400926425,0.975438400926425,
0.975438400926425,0.975438400926425,0.975438400926425,0.975438400926425,
0.975438400926425,0.975438400926425,0.975438400926425,0.975438400926425,
0.975438400926425,0.975438400926425,0.975438400926425,0.975438400926425,
0.975438400926425,0.975438400926425),(1.07175123228254,1.07175123228254,
1.07175123228254,1.07175123228254,1.07175123228254,1.07175123228254,1.07175123228254,
1.07175123228254,1.07175123228254,1.07175123228254,1.07175123228254,1.07175123228254,
1.07175123228254,1.07175123228254,1.07175123228254,1.07175123228254,1.07175123228254,
1.07175123228254,1.07175123228254,1.07175123228254,1.07175123228254,1.07175123228254,
1.07175123228254,1.07175123228254,1.07175123228254,1.07175123228254,1.07175123228254,
1.07175123228254,1.07175123228254,1.07175123228254,1.07175123228254,1.07175123228254,
1.07175123228254,1.07175123228254,1.07175123228254,1.07175123228254,1.07175123228254,
1.07175123228254,1.07175123228254,1.07175123228254)))
REPRESENTATION_ITEM('')
SURFACE()
);
#249=(
BOUNDED_SURFACE()
B_SPLINE_SURFACE(3,3,((#51342,#51343,#51344,#51345,#51346,#51347,#51348,
#51349,#51350,#51351,#51352),(#51353,#51354,#51355,#51356,#51357,#51358,
#51359,#51360,#51361,#51362,#51363),(#51364,#51365,#51366,#51367,#51368,
#51369,#51370,#51371,#51372,#51373,#51374),(#51375,#51376,#51377,#51378,
#51379,#51380,#51381,#51382,#51383,#51384,#51385)),.UNSPECIFIED.,.F.,.F.,
 .F.)
B_SPLINE_SURFACE_WITH_KNOTS((4,4),(4,1,1,1,1,1,1,1,4),(0.0572583228212178,
0.942717312100056),(0.294864893273,0.3218289753162,0.3824545414156,0.4420617671716,
0.5001624934407,0.5582690238001,0.6178889113001,0.678495276987,0.7051030418064),
 .UNSPECIFIED.)
GEOMETRIC_REPRESENTATION_ITEM()
RATIONAL_B_SPLINE_SURFACE(((1.19364643609647,1.19364643609647,1.19364643609647,
1.19364643609647,1.19364643609647,1.19364643609647,1.19364643609647,1.19364643609647,
1.19364643609647,1.19364643609647,1.19364643609647),(0.93545829250305,0.93545829250305,
0.93545829250305,0.93545829250305,0.93545829250305,0.93545829250305,0.93545829250305,
0.93545829250305,0.93545829250305,0.93545829250305,0.93545829250305),(0.935451188163467,
0.935451188163467,0.935451188163467,0.935451188163467,0.935451188163467,
0.935451188163467,0.935451188163467,0.935451188163467,0.935451188163467,
0.935451188163467,0.935451188163467),(1.19362512307772,1.19362512307772,
1.19362512307772,1.19362512307772,1.19362512307772,1.19362512307772,1.19362512307772,
1.19362512307772,1.19362512307772,1.19362512307772,1.19362512307772)))
REPRESENTATION_ITEM('')
SURFACE()
);
#250=(
BOUNDED_SURFACE()
B_SPLINE_SURFACE(3,3,((#51387,#51388,#51389,#51390,#51391,#51392,#51393,
#51394,#51395),(#51396,#51397,#51398,#51399,#51400,#51401,#51402,#51403,
#51404),(#51405,#51406,#51407,#51408,#51409,#51410,#51411,#51412,#51413),
(#51414,#51415,#51416,#51417,#51418,#51419,#51420,#51421,#51422)),
 .UNSPECIFIED.,.F.,.F.,.F.)
B_SPLINE_SURFACE_WITH_KNOTS((4,4),(4,1,1,1,1,1,4),(0.0529020528542322,0.947099750452704),
(0.225333279461291,0.239572547302,0.3572550155842,0.4733386917216,0.5865153077446,
0.6955949780245,0.773470390427119),.UNSPECIFIED.)
GEOMETRIC_REPRESENTATION_ITEM()
RATIONAL_B_SPLINE_SURFACE(((1.19748288514912,1.19748288514912,1.19748288514912,
1.19748288514912,1.19748288514912,1.19748288514912,1.19748288514912,1.19748288514912,
1.19748288514912),(0.934171840603826,0.934171840603826,0.934171840603826,
0.934171840603826,0.934171840603826,0.934171840603826,0.934171840603826,
0.934171840603826,0.934171840603826),(0.934172371617932,0.934172371617932,
0.934172371617932,0.934172371617932,0.934172371617932,0.934172371617932,
0.934172371617932,0.934172371617932,0.934172371617932),(1.19748447819143,
1.19748447819143,1.19748447819143,1.19748447819143,1.19748447819143,1.19748447819143,
1.19748447819143,1.19748447819143,1.19748447819143)))
REPRESENTATION_ITEM('')
SURFACE()
);
#251=(
BOUNDED_SURFACE()
B_SPLINE_SURFACE(3,3,((#51525,#51526,#51527,#51528,#51529,#51530,#51531,
#51532,#51533,#51534),(#51535,#51536,#51537,#51538,#51539,#51540,#51541,
#51542,#51543,#51544),(#51545,#51546,#51547,#51548,#51549,#51550,#51551,
#51552,#51553,#51554),(#51555,#51556,#51557,#51558,#51559,#51560,#51561,
#51562,#51563,#51564)),.UNSPECIFIED.,.F.,.F.,.F.)
B_SPLINE_SURFACE_WITH_KNOTS((4,4),(4,1,1,1,1,1,1,4),(0.0889268305855224,
0.904017315502728),(0.02295305876099,0.1427319370604,0.2857219203474,0.4285792797614,
0.5713515650105,0.7142098207389,0.8572808214069,0.9622634165798),
 .UNSPECIFIED.)
GEOMETRIC_REPRESENTATION_ITEM()
RATIONAL_B_SPLINE_SURFACE(((1.11577973130528,1.11577973130528,1.11577973130528,
1.11577973130528,1.11577973130528,1.11577973130528,1.11577973130528,1.11577973130528,
1.11577973130528,1.11577973130528),(0.962731621536822,0.962731621536822,
0.962731621536822,0.962731621536822,0.962731621536822,0.962731621536822,
0.962731621536822,0.962731621536822,0.962731621536822,0.962731621536822),
(0.961418126538433,0.961418126538433,0.961418126538433,0.961418126538433,
0.961418126538433,0.961418126538433,0.961418126538433,0.961418126538433,
0.961418126538433,0.961418126538433),(1.11183924631011,1.11183924631011,
1.11183924631011,1.11183924631011,1.11183924631011,1.11183924631011,1.11183924631011,
1.11183924631011,1.11183924631011,1.11183924631011)))
REPRESENTATION_ITEM('')
SURFACE()
);
#254=SPHERICAL_SURFACE('',#25482,0.4000000000033);
#255=SPHERICAL_SURFACE('',#25492,0.4);
#256=SPHERICAL_SURFACE('',#25497,0.4000000000033);
#257=SPHERICAL_SURFACE('',#25501,0.4000000000033);
#258=SPHERICAL_SURFACE('',#25506,0.4000000000004);
#259=SPHERICAL_SURFACE('',#25514,0.4);
#260=SPHERICAL_SURFACE('',#25519,0.4000000000033);
#261=SPHERICAL_SURFACE('',#25523,0.4000000000033);
#262=SPHERICAL_SURFACE('',#25528,0.4000000000004);
#263=SPHERICAL_SURFACE('',#25536,0.4);
#264=SPHERICAL_SURFACE('',#25541,0.4000000000033);
#265=SPHERICAL_SURFACE('',#25545,0.4000000000033);
#266=SPHERICAL_SURFACE('',#25550,0.4000000000004);
#267=SPHERICAL_SURFACE('',#25558,0.4);
#268=SPHERICAL_SURFACE('',#25563,0.4000000000033);
#269=SPHERICAL_SURFACE('',#25567,0.4000000000033);
#270=SPHERICAL_SURFACE('',#25572,0.4000000000004);
#271=SPHERICAL_SURFACE('',#25575,0.4000000000003);
#272=SPHERICAL_SURFACE('',#25581,0.4);
#273=SPHERICAL_SURFACE('',#25587,0.4000000000033);
#274=SPHERICAL_SURFACE('',#25595,0.4);
#275=SPHERICAL_SURFACE('',#25600,0.4000000000033);
#276=SPHERICAL_SURFACE('',#25604,0.4000000000033);
#277=SPHERICAL_SURFACE('',#25609,0.4000000000004);
#664=B_SPLINE_CURVE_WITH_KNOTS('',3,(#36464,#36465,#36466,#36467,#36468,
#36469,#36470,#36471,#36472,#36473,#36474,#36475,#36476,#36477,#36478,#36479,
#36480,#36481,#36482,#36483,#36484,#36485),.UNSPECIFIED.,.F.,.F.,(4,3,3,
3,3,3,3,4),(0.,0.1428571428571,0.2857142857143,0.4285714285714,0.5714285714286,
0.7142857142857,0.8571428571429,0.999999898934281),.UNSPECIFIED.);
#665=B_SPLINE_CURVE_WITH_KNOTS('',3,(#36487,#36488,#36489,#36490,#36491,
#36492,#36493,#36494,#36495,#36496),.UNSPECIFIED.,.F.,.F.,(4,2,2,2,4),(0.,
0.25,0.5,0.75,0.999999977827856),.UNSPECIFIED.);
#666=B_SPLINE_CURVE_WITH_KNOTS('',3,(#36497,#36498,#36499,#36500,#36501,
#36502,#36503,#36504,#36505,#36506,#36507,#36508,#36509,#36510,#36511,#36512,
#36513,#36514,#36515,#36516,#36517,#36518,#36519,#36520,#36521,#36522,#36523,
#36524,#36525,#36526,#36527,#36528,#36529,#36530,#36531,#36532,#36533,#36534,
#36535,#36536,#36537,#36538,#36539,#36540,#36541,#36542,#36543,#36544,#36545,
#36546,#36547,#36548,#36549,#36550,#36551,#36552,#36553,#36554),
 .UNSPECIFIED.,.F.,.F.,(4,3,3,3,3,3,3,3,3,3,3,3,3,3,3,3,3,3,3,4),(0.,0.105002988004599,
0.155917176333588,0.250000000000014,0.344903197011831,0.374883793981179,
0.375000000000021,0.437500000000025,0.468750000000026,0.484375000000028,
0.49475363720318,0.50000000000003,0.589831227578696,0.605819254748115,0.693556036024795,
0.774340158848298,0.83459764802956,0.912184758108774,0.984866536115133,
1.),.UNSPECIFIED.);
#667=B_SPLINE_CURVE_WITH_KNOTS('',3,(#36594,#36595,#36596,#36597,#36598,
#36599,#36600),.UNSPECIFIED.,.F.,.F.,(4,3,4),(0.,0.5,1.),.UNSPECIFIED.);
#668=B_SPLINE_CURVE_WITH_KNOTS('',3,(#36601,#36602,#36603,#36604,#36605,
#36606,#36607,#36608,#36609,#36610,#36611,#36612,#36613,#36614,#36615,#36616,
#36617,#36618,#36619,#36620,#36621,#36622,#36623,#36624,#36625,#36626,#36627,
#36628,#36629,#36630,#36631,#36632,#36633,#36634,#36635,#36636,#36637,#36638,
#36639,#36640),.UNSPECIFIED.,.F.,.F.,(4,3,3,3,3,3,3,3,3,3,3,3,3,4),(0.,
0.0909082481788675,0.123952457010317,0.249999999999991,0.369498550498918,
0.437499999999988,0.466123466012437,0.495112348455061,0.499999999999986,
0.615780953250484,0.725499099793163,0.834738856311408,0.940690774028189,
0.999999999999981),.UNSPECIFIED.);
#669=B_SPLINE_CURVE_WITH_KNOTS('',3,(#36681,#36682,#36683,#36684,#36685,
#36686,#36687),.UNSPECIFIED.,.F.,.F.,(4,3,4),(0.,0.5,1.),.UNSPECIFIED.);
#670=B_SPLINE_CURVE_WITH_KNOTS('',3,(#36689,#36690,#36691,#36692,#36693,
#36694,#36695,#36696,#36697,#36698,#36699,#36700,#36701,#36702,#36703,#36704,
#36705,#36706,#36707,#36708,#36709,#36710,#36711,#36712,#36713,#36714,#36715,
#36716,#36717,#36718,#36719,#36720,#36721,#36722,#36723,#36724,#36725,#36726,
#36727,#36728),.UNSPECIFIED.,.F.,.F.,(4,3,3,3,3,3,3,3,3,3,3,3,3,4),(0.,
0.0902944655636358,0.118857317207941,0.249999999999996,0.363581344800914,
0.437499999999993,0.46615258320005,0.495170166317412,0.499999999999992,
0.615785321959331,0.718419711826768,0.827854048218974,0.933927706995318,
1.),.UNSPECIFIED.);
#671=B_SPLINE_CURVE_WITH_KNOTS('',3,(#36729,#36730,#36731,#36732,#36733,
#36734,#36735,#36736,#36737,#36738,#36739,#36740,#36741,#36742,#36743,#36744,
#36745,#36746,#36747,#36748,#36749,#36750,#36751,#36752,#36753,#36754,#36755,
#36756,#36757,#36758,#36759,#36760,#36761,#36762,#36763,#36764,#36765,#36766,
#36767,#36768,#36769,#36770,#36771,#36772,#36773,#36774,#36775,#36776,#36777,
#36778,#36779,#36780,#36781,#36782,#36783,#36784,#36785,#36786),
 .UNSPECIFIED.,.F.,.F.,(4,3,3,3,3,3,3,3,3,3,3,3,3,3,3,3,3,3,3,4),(0.,0.105552995127946,
0.150464219760517,0.249999999999963,0.345315720540772,0.371222911163473,
0.374999999999944,0.437499999999933,0.468749999999929,0.484374999999928,
0.494785177746841,0.499999999999927,0.589592294372024,0.602891943836453,
0.690489241102981,0.771089083019577,0.833649950322395,0.911000884560973,
0.983433730186261,1.),.UNSPECIFIED.);
#672=B_SPLINE_CURVE_WITH_KNOTS('',3,(#36832,#36833,#36834,#36835,#36836,
#36837,#36838,#36839,#36840,#36841,#36842,#36843,#36844,#36845,#36846,#36847,
#36848,#36849,#36850,#36851,#36852,#36853,#36854,#36855,#36856,#36857,#36858,
#36859,#36860,#36861,#36862,#36863,#36864,#36865,#36866,#36867,#36868,#36869,
#36870,#36871,#36872,#36873,#36874,#36875,#36876,#36877,#36878,#36879,#36880,
#36881,#36882,#36883,#36884,#36885,#36886,#36887,#36888,#36889,#36890,#36891,
#36892,#36893,#36894,#36895,#36896,#36897,#36898,#36899,#36900,#36901,#36902,
#36903,#36904),.UNSPECIFIED.,.F.,.F.,(4,3,3,3,3,3,3,3,3,3,3,3,3,3,3,3,3,
3,3,3,3,3,3,3,4),(0.,0.0458328892065342,0.0918178601818331,0.137727870818893,
0.1428571428571,0.14853659813261,0.203804992710247,0.259124754660749,0.2857142857143,
0.296137570174206,0.362354499372803,0.4285714285714,0.443717909280085,0.511006798168795,
0.5714285714286,0.591516277431312,0.658633939603418,0.7142857142857,0.739436741598557,
0.798289799370729,0.8571428571429,0.887213042156971,0.933524276500352,0.979590782779799,
1.),.UNSPECIFIED.);
#673=B_SPLINE_CURVE_WITH_KNOTS('',3,(#36907,#36908,#36909,#36910,#36911,
#36912,#36913,#36914,#36915,#36916,#36917,#36918,#36919,#36920,#36921,#36922,
#36923,#36924,#36925,#36926,#36927,#36928,#36929,#36930,#36931,#36932,#36933,
#36934,#36935,#36936,#36937,#36938,#36939,#36940,#36941,#36942,#36943,#36944,
#36945,#36946),.UNSPECIFIED.,.F.,.F.,(4,3,3,3,3,3,3,3,3,3,3,3,3,4),(0.,
0.13299060193257,0.15336958276858,0.288984804521056,0.306719318925449,0.443622689339626,
0.460361902078992,0.597256089920579,0.614811263003171,0.75,0.769627679195988,
0.90936404691236,0.924609578280667,0.999999999980555),.UNSPECIFIED.);
#674=B_SPLINE_CURVE_WITH_KNOTS('',3,(#36969,#36970,#36971,#36972,#36973,
#36974,#36975,#36976,#36977,#36978),.UNSPECIFIED.,.F.,.F.,(4,3,3,4),(0.,
0.3333333333333,0.6666666666667,1.),.UNSPECIFIED.);
#675=B_SPLINE_CURVE_WITH_KNOTS('',3,(#37114,#37115,#37116,#37117,#37118,
#37119,#37120,#37121,#37122,#37123,#37124,#37125,#37126,#37127,#37128,#37129,
#37130,#37131,#37132,#37133,#37134,#37135,#37136,#37137,#37138,#37139,#37140,
#37141,#37142,#37143,#37144,#37145,#37146,#37147,#37148,#37149,#37150,#37151,
#37152,#37153,#37154,#37155,#37156,#37157,#37158,#37159,#37160,#37161,#37162,
#37163,#37164,#37165,#37166,#37167,#37168,#37169,#37170,#37171,#37172,#37173,
#37174,#37175,#37176,#37177,#37178,#37179,#37180,#37181,#37182,#37183,#37184,
#37185,#37186,#37187,#37188,#37189,#37190,#37191,#37192,#37193,#37194,#37195,
#37196,#37197,#37198,#37199,#37200,#37201,#37202),.UNSPECIFIED.,.F.,.F.,
(4,2,2,1,2,2,2,2,1,1,2,2,2,2,1,1,1,2,2,2,2,2,2,2,2,2,1,2,2,2,1,1,2,2,2,
2,1,1,2,2,2,2,1,1,2,2,2,1,1,2,2,4),(0.,0.031249999999999,0.0468749999999985,
0.0546874999999983,0.0585937499999983,0.0624999999999984,0.0937499999999984,
0.109374999999998,0.117187499999999,0.121093749999999,0.123046874999999,
0.124999999999999,0.1875,0.21875,0.234375,0.2421875,0.24609375,0.248046875,
0.25,0.312500000000001,0.343750000000002,0.359375000000002,0.375000000000002,
0.437500000000003,0.468750000000003,0.484375000000004,0.492187500000004,
0.496093750000004,0.500000000000004,0.562500000000005,0.593750000000005,
0.609375000000006,0.617187500000006,0.625000000000006,0.687500000000006,
0.718750000000006,0.734375000000007,0.742187500000007,0.746093750000007,
0.750000000000007,0.812500000000008,0.843750000000008,0.859375000000009,
0.867187500000009,0.871093750000009,0.875000000000009,0.906250000000007,
0.921875000000006,0.929687500000006,0.933593750000006,0.937500000000006,
1.),.UNSPECIFIED.);
#676=B_SPLINE_CURVE_WITH_KNOTS('',3,(#37205,#37206,#37207,#37208,#37209,
#37210,#37211,#37212,#37213,#37214,#37215,#37216,#37217,#37218,#37219,#37220,
#37221,#37222,#37223,#37224,#37225,#37226,#37227,#37228,#37229,#37230,#37231,
#37232,#37233,#37234,#37235,#37236,#37237,#37238,#37239,#37240,#37241,#37242,
#37243,#37244,#37245,#37246,#37247,#37248,#37249,#37250,#37251,#37252,#37253,
#37254,#37255,#37256,#37257,#37258,#37259,#37260,#37261,#37262,#37263,#37264,
#37265,#37266,#37267,#37268,#37269,#37270,#37271,#37272,#37273,#37274,#37275,
#37276,#37277,#37278,#37279,#37280,#37281,#37282,#37283,#37284,#37285,#37286,
#37287,#37288,#37289,#37290,#37291,#37292,#37293,#37294,#37295,#37296,#37297,
#37298,#37299,#37300,#37301,#37302,#37303,#37304,#37305,#37306,#37307,#37308,
#37309,#37310,#37311,#37312,#37313,#37314,#37315,#37316,#37317,#37318,#37319,
#37320,#37321,#37322,#37323,#37324,#37325,#37326,#37327,#37328,#37329,#37330,
#37331,#37332,#37333,#37334,#37335,#37336,#37337,#37338,#37339,#37340,#37341,
#37342,#37343,#37344,#37345,#37346,#37347,#37348,#37349,#37350,#37351,#37352,
#37353,#37354,#37355,#37356,#37357,#37358,#37359,#37360,#37361,#37362,#37363,
#37364,#37365,#37366,#37367,#37368,#37369,#37370,#37371,#37372,#37373,#37374,
#37375,#37376,#37377,#37378,#37379,#37380,#37381,#37382,#37383,#37384,#37385,
#37386,#37387,#37388,#37389,#37390,#37391),.UNSPECIFIED.,.F.,.F.,(4,3,3,
3,3,3,3,3,3,3,3,3,3,3,3,3,3,3,3,3,3,3,3,3,3,3,3,3,3,3,3,3,3,3,3,3,3,3,3,
3,3,3,3,3,3,3,3,3,3,3,3,3,3,3,3,3,3,3,3,3,3,3,4),(7.50077097463719E-8,2.18347029427447E-7,
0.0229487856938132,0.0291139710122845,0.0509738189930032,0.0551840493051654,
0.0624999999999677,0.0795327477259671,0.100117077611303,0.102945273631019,
0.109374999999943,0.11718749999994,0.121093749999938,0.123046874999937,
0.124511718749936,0.124999999999936,0.126823302088405,0.154172312025519,
0.168540298053765,0.195094832668279,0.207814194056933,0.234374999999943,
0.243586029297769,0.245604724495927,0.249999999999944,0.286467474258032,
0.32318429611145,0.33538678826966,0.372228071632762,0.396071565286844,0.433033005791837,
0.468749999999958,0.471330308172129,0.484374999999959,0.49218749999996,
0.499325175973332,0.49999999999996,0.539362014881174,0.553208179067863,
0.592489117635982,0.619376295226936,0.658509964129895,0.6731316840546,0.711996821297296,
0.71672755379256,0.718749999999974,0.734374999999975,0.742187499999975,
0.746093749999976,0.749489018450129,0.749999999999976,0.753696520049675,
0.789783434716073,0.822480899844826,0.851890674726284,0.878120292282693,
0.901491656587809,0.922410562386568,0.941272552181438,0.958424197689089,
0.97402098939019,0.988170714014038,1.),.UNSPECIFIED.);
#677=B_SPLINE_CURVE_WITH_KNOTS('',3,(#37428,#37429,#37430,#37431,#37432,
#37433,#37434,#37435,#37436,#37437),.UNSPECIFIED.,.F.,.F.,(4,2,2,2,4),(2.21660088532052E-8,
0.25,0.5,0.75,1.),.UNSPECIFIED.);
#678=B_SPLINE_CURVE_WITH_KNOTS('',3,(#37438,#37439,#37440,#37441,#37442,
#37443,#37444,#37445,#37446,#37447,#37448,#37449,#37450,#37451,#37452,#37453,
#37454,#37455,#37456,#37457,#37458,#37459,#37460,#37461,#37462,#37463,#37464,
#37465,#37466,#37467,#37468,#37469,#37470,#37471,#37472,#37473,#37474,#37475,
#37476,#37477,#37478,#37479,#37480,#37481,#37482,#37483,#37484,#37485,#37486,
#37487,#37488,#37489,#37490,#37491,#37492,#37493,#37494,#37495,#37496,#37497,
#37498),.UNSPECIFIED.,.F.,.F.,(4,3,3,3,3,3,3,3,3,3,3,3,3,3,3,3,3,3,3,3,
4),(4.17868136098958E-11,0.100717583252596,0.175358791626298,0.238666052088337,
0.25,0.301434359568119,0.35111583137364,0.400012448249277,0.450006224124639,
0.497458126672331,0.5,0.500002161178376,0.547542422094837,0.598156816571128,
0.647554640521333,0.698777320260667,0.75,0.812847074588508,0.88799364390341,
0.987406860642747,0.999999999945156),.UNSPECIFIED.);
#679=B_SPLINE_CURVE_WITH_KNOTS('',3,(#37541,#37542,#37543,#37544,#37545,
#37546,#37547,#37548,#37549,#37550,#37551,#37552,#37553,#37554,#37555,#37556,
#37557,#37558,#37559,#37560,#37561,#37562,#37563,#37564,#37565,#37566,#37567,
#37568,#37569,#37570,#37571,#37572,#37573,#37574,#37575,#37576,#37577,#37578,
#37579,#37580,#37581,#37582,#37583,#37584,#37585,#37586,#37587,#37588,#37589,
#37590,#37591,#37592,#37593,#37594,#37595,#37596,#37597,#37598,#37599,#37600,
#37601,#37602,#37603,#37604,#37605,#37606,#37607,#37608,#37609,#37610,#37611,
#37612,#37613,#37614,#37615,#37616,#37617,#37618,#37619,#37620,#37621,#37622,
#37623,#37624,#37625,#37626,#37627,#37628,#37629,#37630,#37631,#37632,#37633,
#37634,#37635,#37636,#37637),.UNSPECIFIED.,.F.,.F.,(4,3,3,3,3,3,3,3,3,3,
3,3,3,3,3,3,3,3,3,3,3,3,3,3,3,3,3,3,3,3,3,3,4),(0.,0.0611399008016612,0.118912943243393,
0.122279801603322,0.125000000000001,0.18183766361929,0.187500000000002,
0.218750000000002,0.234375000000002,0.242187500000002,0.247821297884802,
0.250000000000002,0.273770686693072,0.341484900394223,0.40789775146333,
0.425473607482879,0.492297059906689,0.500000000000002,0.565514473352424,
0.574275766966002,0.625000000000002,0.687500000000002,0.718750000000001,
0.725971908159189,0.734375000000002,0.742187500000001,0.747865905418132,
0.750000000000001,0.805738424564014,0.862859242738749,0.877451482579203,
0.938725741289602,1.),.UNSPECIFIED.);
#680=B_SPLINE_CURVE_WITH_KNOTS('',3,(#37676,#37677,#37678,#37679,#37680,
#37681,#37682,#37683,#37684,#37685,#37686,#37687,#37688,#37689,#37690,#37691,
#37692,#37693,#37694,#37695,#37696,#37697,#37698,#37699,#37700,#37701,#37702,
#37703,#37704,#37705,#37706,#37707,#37708,#37709,#37710,#37711,#37712,#37713,
#37714,#37715,#37716,#37717,#37718,#37719,#37720,#37721,#37722,#37723,#37724),
 .UNSPECIFIED.,.F.,.F.,(4,3,3,3,3,3,3,3,3,3,3,3,3,3,3,3,4),(0.,0.0770829581399577,
0.115833104604136,0.19702880740101,0.250000000000003,0.333153117311277,
0.356333767066429,0.375000000000002,0.422947860378306,0.471329030291448,
0.500000000000002,0.606855024395177,0.708280894793895,0.713710048790352,
0.815228553321396,0.918005904150946,1.),.UNSPECIFIED.);
#681=B_SPLINE_CURVE_WITH_KNOTS('',3,(#37725,#37726,#37727,#37728,#37729,
#37730,#37731),.UNSPECIFIED.,.F.,.F.,(4,3,4),(0.,0.5,0.999999979800132),
 .UNSPECIFIED.);
#682=B_SPLINE_CURVE_WITH_KNOTS('',3,(#37732,#37733,#37734,#37735,#37736,
#37737,#37738,#37739,#37740,#37741,#37742,#37743,#37744,#37745,#37746,#37747,
#37748,#37749,#37750,#37751,#37752,#37753,#37754,#37755,#37756,#37757,#37758,
#37759,#37760,#37761,#37762,#37763,#37764,#37765,#37766,#37767,#37768,#37769,
#37770,#37771,#37772,#37773,#37774,#37775,#37776,#37777,#37778,#37779,#37780,
#37781,#37782,#37783,#37784,#37785,#37786,#37787,#37788,#37789),
 .UNSPECIFIED.,.F.,.F.,(4,3,3,3,3,3,3,3,3,3,3,3,3,3,3,3,3,3,3,4),(0.,0.0715674218076948,
0.147880597762145,0.168248115152606,0.25000000000001,0.335016575408999,
0.375000000000014,0.399721731097707,0.437500000000018,0.468750000000019,
0.48437500000002,0.49533836253787,0.50000000000002,0.59336847865171,0.631329959825261,
0.726440396785077,0.827653169575289,0.852289991333602,0.957929681900358,
1.),.UNSPECIFIED.);
#683=B_SPLINE_CURVE_WITH_KNOTS('',3,(#37832,#37833,#37834,#37835,#37836,
#37837,#37838,#37839,#37840,#37841,#37842,#37843,#37844,#37845,#37846,#37847,
#37848,#37849,#37850,#37851,#37852,#37853),.UNSPECIFIED.,.F.,.F.,(4,3,3,
3,3,3,3,4),(1.01036473954356E-7,0.1428571428571,0.2857142857143,0.4285714285714,
0.5714285714286,0.7142857142857,0.8571428571429,1.),.UNSPECIFIED.);
#684=B_SPLINE_CURVE_WITH_KNOTS('',3,(#37896,#37897,#37898,#37899,#37900,
#37901,#37902),.UNSPECIFIED.,.F.,.F.,(4,3,4),(2.15057445811703E-8,0.5,1.),
 .UNSPECIFIED.);
#685=B_SPLINE_CURVE_WITH_KNOTS('',3,(#37904,#37905,#37906,#37907,#37908,
#37909,#37910,#37911,#37912,#37913,#37914,#37915,#37916,#37917,#37918,#37919,
#37920,#37921,#37922,#37923,#37924,#37925,#37926,#37927,#37928,#37929,#37930,
#37931,#37932,#37933,#37934,#37935,#37936,#37937,#37938,#37939,#37940,#37941,
#37942,#37943,#37944,#37945,#37946),.UNSPECIFIED.,.F.,.F.,(4,3,3,3,3,3,
3,3,3,3,3,3,3,3,4),(0.,0.0900134680643692,0.1164031392641,0.243030188030943,
0.249999999999983,0.360148491907499,0.437499999999976,0.466161731423018,
0.495188458339603,0.499999999999975,0.615787821036494,0.712805741778485,
0.822400103490752,0.928574215008832,1.),.UNSPECIFIED.);
#686=B_SPLINE_CURVE_WITH_KNOTS('',3,(#37947,#37948,#37949,#37950,#37951,
#37952,#37953,#37954,#37955,#37956,#37957,#37958,#37959,#37960,#37961,#37962,
#37963,#37964,#37965,#37966,#37967,#37968,#37969,#37970,#37971,#37972,#37973,
#37974,#37975,#37976,#37977,#37978,#37979,#37980,#37981,#37982,#37983,#37984,
#37985,#37986,#37987,#37988,#37989,#37990,#37991,#37992,#37993,#37994,#37995,
#37996,#37997,#37998,#37999,#38000,#38001,#38002,#38003,#38004),
 .UNSPECIFIED.,.F.,.F.,(4,3,3,3,3,3,3,3,3,3,3,3,3,3,3,3,3,3,3,4),(0.,0.105620931649772,
0.147712761945928,0.249999999999997,0.345332751509973,0.368665278781871,
0.374999999999996,0.437499999999994,0.468749999999995,0.484374999999994,
0.494735172857366,0.499999999999994,0.589017276416335,0.600284492062021,
0.686110218149057,0.749999999999997,0.831760917477541,0.908457546686943,
0.980209191163759,1.),.UNSPECIFIED.);
#687=B_SPLINE_CURVE_WITH_KNOTS('',3,(#38046,#38047,#38048,#38049,#38050,
#38051,#38052,#38053,#38054,#38055,#38056,#38057,#38058,#38059,#38060,#38061,
#38062,#38063,#38064,#38065,#38066,#38067),.UNSPECIFIED.,.F.,.F.,(4,3,3,
3,3,3,3,4),(0.,0.1428571428571,0.2857142857143,0.4285714285714,0.5714285714286,
0.7142857142857,0.8571428571429,0.99999989893635),.UNSPECIFIED.);
#688=B_SPLINE_CURVE_WITH_KNOTS('',3,(#38070,#38071,#38072,#38073,#38074,
#38075,#38076,#38077,#38078,#38079),.UNSPECIFIED.,.F.,.F.,(4,2,2,2,4),(0.,
0.25,0.499999999999999,0.749999999999999,0.999999977827809),
 .UNSPECIFIED.);
#689=B_SPLINE_CURVE_WITH_KNOTS('',3,(#38109,#38110,#38111,#38112,#38113,
#38114,#38115,#38116,#38117,#38118,#38119,#38120,#38121),.UNSPECIFIED.,
 .F.,.F.,(4,3,3,3,4),(0.,0.0431918509065784,0.5,0.956806409099894,1.),
 .UNSPECIFIED.);
#690=B_SPLINE_CURVE_WITH_KNOTS('',3,(#38142,#38143,#38144,#38145,#38146,
#38147,#38148,#38149,#38150,#38151,#38152,#38153,#38154,#38155,#38156,#38157,
#38158,#38159,#38160,#38161,#38162,#38163,#38164,#38165,#38166,#38167,#38168,
#38169,#38170,#38171,#38172,#38173,#38174,#38175,#38176,#38177,#38178,#38179,
#38180,#38181,#38182,#38183,#38184,#38185,#38186,#38187,#38188,#38189,#38190,
#38191,#38192,#38193,#38194,#38195,#38196,#38197,#38198,#38199,#38200,#38201,
#38202,#38203,#38204,#38205,#38206,#38207,#38208,#38209,#38210,#38211,#38212,
#38213,#38214,#38215,#38216,#38217,#38218,#38219,#38220,#38221,#38222,#38223,
#38224,#38225,#38226,#38227,#38228,#38229,#38230,#38231,#38232,#38233,#38234,
#38235,#38236,#38237,#38238,#38239,#38240,#38241,#38242,#38243,#38244,#38245,
#38246,#38247,#38248,#38249,#38250,#38251,#38252,#38253,#38254,#38255,#38256,
#38257,#38258,#38259,#38260,#38261,#38262,#38263,#38264,#38265,#38266,#38267,
#38268,#38269,#38270,#38271,#38272,#38273,#38274,#38275,#38276,#38277,#38278,
#38279,#38280,#38281,#38282,#38283,#38284,#38285,#38286,#38287,#38288,#38289,
#38290,#38291,#38292,#38293,#38294,#38295,#38296,#38297,#38298,#38299,#38300,
#38301,#38302,#38303,#38304,#38305,#38306,#38307,#38308,#38309,#38310,#38311,
#38312,#38313,#38314,#38315,#38316,#38317,#38318,#38319,#38320,#38321,#38322,
#38323,#38324,#38325,#38326,#38327,#38328,#38329,#38330,#38331,#38332,#38333,
#38334,#38335,#38336,#38337,#38338,#38339,#38340,#38341,#38342,#38343,#38344,
#38345,#38346),.UNSPECIFIED.,.F.,.F.,(4,3,3,3,3,3,3,3,3,3,3,3,3,3,3,3,3,
3,3,3,3,3,3,3,3,3,3,3,3,3,3,3,3,3,3,3,3,3,3,3,3,3,3,3,3,3,3,3,3,3,3,3,3,
3,3,3,3,3,3,3,3,3,3,3,3,3,3,3,4),(0.,0.0249952040648666,0.0499029976050593,
0.0680454790691359,0.0924338447088906,0.107880913519564,0.131553995034703,
0.140984707740201,0.16395680048273,0.171035558612113,0.193345860441903,
0.199615480235769,0.218750000000002,0.227604280455894,0.234375000000003,
0.242187500000003,0.246093750000003,0.248046875000003,0.249023437500003,
0.250000000000003,0.254582622012608,0.280004563056784,0.307433325464391,
0.30946109206094,0.337151591946959,0.344194252878218,0.372025449866619,
0.384942334286463,0.412589612654437,0.429868562571756,0.457864931018828,
0.468749999999994,0.477270445734503,0.484374999999993,0.492187499999993,
0.496093749999992,0.498046874999992,0.499999999999992,0.531323458090248,
0.565671952103585,0.578524990186005,0.613136937556426,0.61640423603698,
0.648095328683626,0.674911251899195,0.697968240955163,0.718048375778514,
0.718749999999977,0.734374999999976,0.735668182771794,0.742187499999975,
0.746093749999975,0.748046874999975,0.749023437499975,0.749999999999975,
0.751820094958488,0.773837782688054,0.795119290834591,0.815755174137061,
0.835862819339601,0.855595765790536,0.874999999999987,0.875158502104443,
0.894772749621587,0.914585430706598,0.934770786003287,0.955587723025151,
0.977474708625959,0.999999988569583),.UNSPECIFIED.);
#691=B_SPLINE_CURVE_WITH_KNOTS('',3,(#38509,#38510,#38511,#38512,#38513,
#38514,#38515,#38516,#38517,#38518,#38519,#38520,#38521,#38522,#38523,#38524,
#38525,#38526,#38527,#38528,#38529,#38530,#38531,#38532,#38533,#38534,#38535,
#38536,#38537,#38538,#38539,#38540,#38541,#38542,#38543,#38544,#38545,#38546,
#38547,#38548,#38549,#38550,#38551,#38552,#38553,#38554,#38555,#38556,#38557,
#38558,#38559,#38560,#38561,#38562,#38563,#38564,#38565,#38566,#38567,#38568,
#38569,#38570,#38571,#38572,#38573,#38574,#38575,#38576,#38577,#38578,#38579,
#38580,#38581,#38582,#38583,#38584,#38585,#38586,#38587,#38588,#38589,#38590,
#38591,#38592,#38593,#38594,#38595,#38596,#38597,#38598,#38599,#38600,#38601,
#38602,#38603,#38604,#38605,#38606,#38607,#38608,#38609,#38610,#38611,#38612,
#38613,#38614,#38615,#38616,#38617,#38618,#38619,#38620,#38621,#38622,#38623,
#38624,#38625,#38626,#38627,#38628,#38629),.UNSPECIFIED.,.F.,.F.,(4,3,3,
3,3,3,3,3,3,3,3,3,3,3,3,3,3,3,3,3,3,3,3,3,3,3,3,3,3,3,3,3,3,3,3,3,3,3,3,
3,4),(7.98332897105801E-8,0.0312500598749729,0.0618422405072992,0.0934211202536609,
0.125000000000023,0.155569265149762,0.187159632574901,0.218750000000039,
0.234375000000042,0.242187500000044,0.246093750000044,0.248046875000045,
0.249023437500045,0.250000000000045,0.450377467746167,0.499981371599102,
0.500000000000075,0.625000000000089,0.687500000000097,0.718750000000101,
0.734375000000103,0.742187500000103,0.749511718750104,0.750000000000104,
0.765918986862788,0.781838152049637,0.79775750567844,0.813677171231473,
0.829597016624591,0.845517165313362,0.859375000000058,0.867187500000055,
0.871093750000053,0.873046875000052,0.874023437500052,0.875000000000052,
0.899836670682714,0.924877489292667,0.949727576111283,0.974863760616905,
0.999999945122527),.UNSPECIFIED.);
#692=B_SPLINE_CURVE_WITH_KNOTS('',3,(#38670,#38671,#38672,#38673,#38674,
#38675,#38676,#38677,#38678,#38679,#38680,#38681,#38682,#38683,#38684,#38685,
#38686,#38687,#38688,#38689,#38690,#38691,#38692,#38693,#38694,#38695,#38696,
#38697,#38698,#38699,#38700,#38701,#38702,#38703,#38704,#38705,#38706,#38707,
#38708,#38709,#38710,#38711,#38712,#38713,#38714,#38715,#38716,#38717,#38718),
 .UNSPECIFIED.,.F.,.F.,(4,3,3,3,3,3,3,3,3,3,3,3,3,3,3,3,4),(0.,0.0771288858376249,
0.118224466833141,0.199428832370291,0.25,0.333192391283466,0.35971949877537,
0.375000000000001,0.422997119033468,0.471428608082327,0.500000000000001,
0.602026122232166,0.703467968575276,0.719208889717013,0.820752755140426,
0.923561571449876,1.),.UNSPECIFIED.);
#693=B_SPLINE_CURVE_WITH_KNOTS('',3,(#38720,#38721,#38722,#38723,#38724,
#38725,#38726),.UNSPECIFIED.,.F.,.F.,(4,3,4),(0.,0.5,1.),.UNSPECIFIED.);
#694=B_SPLINE_CURVE_WITH_KNOTS('',3,(#38729,#38730,#38731,#38732,#38733,
#38734,#38735,#38736,#38737,#38738,#38739,#38740,#38741,#38742,#38743,#38744,
#38745,#38746,#38747,#38748,#38749,#38750,#38751,#38752,#38753,#38754,#38755,
#38756,#38757,#38758,#38759,#38760,#38761,#38762,#38763,#38764,#38765,#38766,
#38767,#38768,#38769,#38770,#38771,#38772,#38773,#38774,#38775,#38776,#38777,
#38778,#38779,#38780,#38781,#38782,#38783,#38784,#38785,#38786,#38787,#38788,
#38789),.UNSPECIFIED.,.F.,.F.,(4,3,3,3,3,3,3,3,3,3,3,3,3,3,3,3,3,3,3,3,
4),(0.,0.0723228733734608,0.149373740660938,0.166421151448187,0.245216396826458,
0.249999999999982,0.335716238671773,0.374999999999972,0.397180419852709,
0.437499999999968,0.468749999999969,0.48437499999997,0.495375830345444,
0.499999999999971,0.593362814881258,0.628795106216759,0.723805214627839,
0.824915510586949,0.849552874144399,0.955120141692627,1.),.UNSPECIFIED.);
#695=B_SPLINE_CURVE_WITH_KNOTS('',3,(#38830,#38831,#38832,#38833,#38834,
#38835,#38836,#38837,#38838,#38839,#38840,#38841,#38842,#38843,#38844,#38845,
#38846,#38847,#38848,#38849,#38850,#38851,#38852,#38853,#38854,#38855,#38856,
#38857,#38858,#38859,#38860,#38861,#38862,#38863,#38864,#38865,#38866,#38867,
#38868,#38869,#38870,#38871,#38872),.UNSPECIFIED.,.F.,.F.,(4,3,3,3,3,3,
3,3,3,3,3,3,3,3,4),(2.99705957294E-11,0.0832138091825946,0.218578168494638,
0.246109287965936,0.25,0.383459477745923,0.408370300217607,0.541180649747327,
0.570056216707183,0.702294204129991,0.731364949826117,0.75,0.881938317493617,
0.892442289989345,0.999999987394246),.UNSPECIFIED.);
#696=B_SPLINE_CURVE_WITH_KNOTS('',3,(#38873,#38874,#38875,#38876,#38877,
#38878,#38879,#38880,#38881,#38882,#38883,#38884,#38885,#38886,#38887,#38888,
#38889,#38890,#38891,#38892,#38893,#38894,#38895,#38896,#38897,#38898,#38899,
#38900,#38901,#38902,#38903,#38904,#38905,#38906,#38907,#38908,#38909,#38910,
#38911,#38912,#38913,#38914,#38915,#38916,#38917,#38918,#38919,#38920,#38921,
#38922,#38923,#38924,#38925,#38926,#38927,#38928,#38929,#38930,#38931,#38932,
#38933,#38934,#38935,#38936,#38937,#38938,#38939,#38940,#38941,#38942,#38943,
#38944,#38945,#38946,#38947,#38948,#38949,#38950,#38951),.UNSPECIFIED.,
 .F.,.F.,(4,3,3,3,3,3,3,3,3,3,3,3,3,3,3,3,3,3,3,3,3,3,3,3,3,3,4),(0.,0.0457810664062895,
0.0917889143914393,0.120317290917192,0.1428571428571,0.198222944257388,
0.253550325461388,0.275526256355529,0.2857142857143,0.349641048829855,0.41364518951731,
0.4285714285714,0.430597609456488,0.496176324090972,0.561795552687674,0.5714285714286,
0.585374526667744,0.649830120476722,0.7142857142857,0.740396273233819,0.795252877513523,
0.850177989920913,0.8571428571429,0.895765393026058,0.94186342671897,0.987754574481698,
0.999999797061768),.UNSPECIFIED.);
#697=B_SPLINE_CURVE_WITH_KNOTS('',3,(#38987,#38988,#38989,#38990,#38991,
#38992,#38993,#38994,#38995,#38996,#38997,#38998,#38999,#39000,#39001,#39002,
#39003,#39004,#39005,#39006,#39007,#39008,#39009,#39010,#39011,#39012,#39013,
#39014,#39015,#39016,#39017,#39018,#39019,#39020,#39021,#39022,#39023,#39024,
#39025,#39026,#39027,#39028,#39029,#39030,#39031,#39032,#39033,#39034,#39035,
#39036,#39037,#39038,#39039,#39040,#39041,#39042,#39043,#39044,#39045,#39046,
#39047),.UNSPECIFIED.,.F.,.F.,(4,3,3,3,3,3,3,3,3,3,3,3,3,3,3,3,3,3,3,3,
4),(5.6316964680001E-11,0.100718446959904,0.175359223479952,0.23866647207507,
0.25,0.301429678396237,0.351106896227335,0.399999481032942,0.449999740516471,
0.497447897994334,0.5,0.500001693682381,0.547538310465323,0.598153732848992,
0.647547504212216,0.698773752106108,0.75,0.812847820507721,0.887998910942513,
0.987406932145145,0.999999999944183),.UNSPECIFIED.);
#698=B_SPLINE_CURVE_WITH_KNOTS('',3,(#39088,#39089,#39090,#39091,#39092,
#39093,#39094,#39095,#39096,#39097,#39098,#39099,#39100,#39101,#39102,#39103,
#39104,#39105,#39106,#39107,#39108,#39109,#39110,#39111,#39112,#39113,#39114,
#39115,#39116,#39117,#39118,#39119,#39120,#39121,#39122,#39123,#39124,#39125,
#39126,#39127,#39128,#39129,#39130,#39131,#39132,#39133,#39134,#39135,#39136,
#39137,#39138,#39139,#39140,#39141,#39142,#39143,#39144,#39145,#39146,#39147,
#39148,#39149,#39150,#39151,#39152,#39153,#39154,#39155,#39156,#39157,#39158,
#39159,#39160,#39161,#39162,#39163,#39164,#39165,#39166,#39167,#39168,#39169,
#39170,#39171,#39172),.UNSPECIFIED.,.F.,.F.,(4,3,3,3,3,3,3,3,3,3,3,3,3,
3,3,3,3,3,3,3,3,3,3,3,3,3,3,3,4),(0.,0.0661535075836036,0.118578546619141,
0.125,0.187500000000001,0.218750000000001,0.234375000000001,0.243852058161108,
0.250000000000001,0.272481796236854,0.339700986415693,0.406654744578485,
0.424962283673657,0.491652042830103,0.500000000000001,0.565705494396537,
0.575150315587252,0.625000000000002,0.687500000000002,0.718750000000002,
0.727633374502205,0.734375000000002,0.743881940457977,0.750000000000002,
0.81217804106019,0.876338528453975,0.881522335850663,0.948429399218141,
1.),.UNSPECIFIED.);
#699=B_SPLINE_CURVE_WITH_KNOTS('',3,(#39213,#39214,#39215,#39216,#39217,
#39218,#39219),.UNSPECIFIED.,.F.,.F.,(4,3,4),(0.,0.5,0.999999999983266),
 .UNSPECIFIED.);
#700=B_SPLINE_CURVE_WITH_KNOTS('',3,(#39221,#39222,#39223,#39224,#39225,
#39226,#39227,#39228,#39229,#39230,#39231,#39232,#39233,#39234,#39235,#39236,
#39237,#39238,#39239,#39240,#39241,#39242,#39243,#39244,#39245,#39246,#39247,
#39248,#39249,#39250,#39251,#39252,#39253,#39254,#39255,#39256,#39257,#39258,
#39259,#39260),.UNSPECIFIED.,.F.,.F.,(4,3,3,3,3,3,3,3,3,3,3,3,3,4),(0.,
0.0902944655942792,0.118857317205525,0.250000000000005,0.363581344799241,
0.437500000000004,0.466152583196255,0.495170166310217,0.500000000000003,
0.615785321950757,0.718419711847765,0.827854048242836,0.933927707021626,
0.999999999999981),.UNSPECIFIED.);
#701=B_SPLINE_CURVE_WITH_KNOTS('',3,(#39261,#39262,#39263,#39264,#39265,
#39266,#39267,#39268,#39269,#39270,#39271,#39272,#39273,#39274,#39275,#39276,
#39277,#39278,#39279,#39280,#39281,#39282,#39283,#39284,#39285,#39286,#39287,
#39288,#39289,#39290,#39291,#39292,#39293,#39294,#39295,#39296,#39297,#39298,
#39299,#39300,#39301,#39302,#39303,#39304,#39305,#39306,#39307,#39308,#39309,
#39310,#39311,#39312,#39313,#39314,#39315,#39316,#39317,#39318),
 .UNSPECIFIED.,.F.,.F.,(4,3,3,3,3,3,3,3,3,3,3,3,3,3,3,3,3,3,3,4),(0.,0.105552984689735,
0.150464224794851,0.250000000000038,0.345315709929821,0.371222912678605,
0.375000000000057,0.437500000000066,0.468750000000071,0.484375000000072,
0.494785170063038,0.500000000000074,0.58959223919739,0.602892053414376,
0.690489305247616,0.771089123956182,0.833650045697548,0.911000967360328,
0.983433814593619,1.),.UNSPECIFIED.);
#702=B_SPLINE_CURVE_WITH_KNOTS('',3,(#39364,#39365,#39366,#39367,#39368,
#39369,#39370,#39371,#39372,#39373,#39374,#39375,#39376,#39377,#39378,#39379,
#39380,#39381,#39382,#39383,#39384,#39385,#39386,#39387,#39388,#39389,#39390,
#39391,#39392,#39393,#39394,#39395,#39396,#39397,#39398,#39399,#39400,#39401,
#39402,#39403,#39404,#39405,#39406,#39407,#39408,#39409,#39410,#39411,#39412,
#39413,#39414,#39415,#39416,#39417,#39418,#39419,#39420,#39421,#39422,#39423,
#39424,#39425,#39426,#39427,#39428,#39429,#39430,#39431,#39432,#39433,#39434,
#39435,#39436),.UNSPECIFIED.,.F.,.F.,(4,3,3,3,3,3,3,3,3,3,3,3,3,3,3,3,3,
3,3,3,3,3,3,3,4),(0.,0.0458328892178335,0.0918178602034833,0.137727870849418,
0.1428571428571,0.14853659813257,0.203804992723845,0.259124754689577,0.2857142857143,
0.296137570174493,0.362354499372946,0.4285714285714,0.443717909280358,0.511006798196711,
0.5714285714286,0.591516277431817,0.658633939614426,0.7142857142857,0.739436741598696,
0.798289799370798,0.8571428571429,0.887213042157008,0.9335242764972,0.979590782772933,
1.),.UNSPECIFIED.);
#703=B_SPLINE_CURVE_WITH_KNOTS('',3,(#39439,#39440,#39441,#39442,#39443,
#39444,#39445,#39446,#39447,#39448,#39449,#39450,#39451,#39452,#39453,#39454,
#39455,#39456,#39457,#39458,#39459,#39460,#39461,#39462,#39463,#39464,#39465,
#39466,#39467,#39468,#39469,#39470,#39471,#39472,#39473,#39474,#39475,#39476,
#39477,#39478),.UNSPECIFIED.,.F.,.F.,(4,3,3,3,3,3,3,3,3,3,3,3,3,4),(0.,
0.132990593054672,0.153369582492901,0.288984795668459,0.306719318472942,
0.443622679891926,0.460361901548923,0.597256080254731,0.614811262496377,
0.75,0.769627678792761,0.909364409081581,0.924609577548183,0.999999999966827),
 .UNSPECIFIED.);
#704=B_SPLINE_CURVE_WITH_KNOTS('',3,(#39501,#39502,#39503,#39504,#39505,
#39506,#39507,#39508,#39509,#39510),.UNSPECIFIED.,.F.,.F.,(4,3,3,4),(0.,
0.3333333333333,0.6666666666667,1.),.UNSPECIFIED.);
#705=B_SPLINE_CURVE_WITH_KNOTS('',3,(#39646,#39647,#39648,#39649,#39650,
#39651,#39652,#39653,#39654,#39655,#39656,#39657,#39658,#39659,#39660,#39661,
#39662,#39663,#39664,#39665,#39666,#39667,#39668,#39669,#39670,#39671,#39672,
#39673,#39674,#39675,#39676,#39677,#39678,#39679,#39680,#39681,#39682,#39683,
#39684,#39685,#39686,#39687,#39688,#39689,#39690,#39691,#39692,#39693,#39694,
#39695,#39696,#39697,#39698,#39699,#39700,#39701,#39702,#39703,#39704,#39705,
#39706,#39707,#39708,#39709,#39710,#39711,#39712,#39713,#39714,#39715,#39716,
#39717,#39718,#39719,#39720,#39721,#39722,#39723,#39724,#39725,#39726,#39727,
#39728,#39729,#39730,#39731,#39732),.UNSPECIFIED.,.F.,.F.,(4,2,2,1,2,2,
2,1,1,1,2,2,2,2,1,1,1,2,2,2,2,2,2,2,2,1,1,2,2,2,1,1,2,2,2,2,1,1,2,2,2,2,
1,1,2,2,2,1,1,2,2,4),(0.,0.0312500000000048,0.0468750000000071,0.0546875000000082,
0.0585937500000085,0.0625000000000087,0.0937500000000093,0.10937500000001,
0.11718750000001,0.12109375000001,0.12304687500001,0.12500000000001,0.187500000000013,
0.218750000000014,0.234375000000015,0.242187500000015,0.246093750000016,
0.248046875000016,0.250000000000016,0.312500000000016,0.343750000000015,
0.359375000000015,0.375000000000015,0.437500000000015,0.468750000000016,
0.484375000000016,0.492187500000016,0.496093750000016,0.500000000000016,
0.562500000000016,0.593750000000016,0.609375000000016,0.617187500000016,
0.625000000000016,0.687500000000016,0.718750000000016,0.734375000000016,
0.742187500000016,0.746093750000016,0.750000000000016,0.812500000000014,
0.843750000000013,0.859375000000013,0.867187500000013,0.871093750000012,
0.875000000000012,0.906250000000011,0.92187500000001,0.92968750000001,0.933593750000009,
0.937500000000009,1.),.UNSPECIFIED.);
#706=B_SPLINE_CURVE_WITH_KNOTS('',3,(#39735,#39736,#39737,#39738,#39739,
#39740,#39741,#39742,#39743,#39744,#39745,#39746,#39747,#39748,#39749,#39750,
#39751,#39752,#39753,#39754,#39755,#39756,#39757,#39758,#39759,#39760,#39761,
#39762,#39763,#39764,#39765,#39766,#39767,#39768,#39769,#39770,#39771,#39772,
#39773,#39774,#39775,#39776,#39777,#39778,#39779,#39780,#39781,#39782,#39783,
#39784,#39785,#39786,#39787,#39788,#39789,#39790,#39791,#39792,#39793,#39794,
#39795,#39796,#39797,#39798,#39799,#39800,#39801,#39802,#39803,#39804,#39805,
#39806,#39807,#39808,#39809,#39810,#39811,#39812,#39813,#39814,#39815,#39816,
#39817,#39818,#39819,#39820,#39821,#39822,#39823,#39824,#39825,#39826,#39827,
#39828,#39829,#39830,#39831,#39832,#39833,#39834,#39835,#39836,#39837,#39838,
#39839,#39840,#39841,#39842,#39843,#39844,#39845,#39846,#39847,#39848,#39849,
#39850,#39851,#39852,#39853,#39854,#39855,#39856,#39857,#39858,#39859,#39860,
#39861,#39862,#39863,#39864,#39865,#39866,#39867,#39868,#39869,#39870,#39871,
#39872,#39873,#39874,#39875,#39876,#39877,#39878,#39879,#39880,#39881,#39882,
#39883,#39884,#39885,#39886,#39887,#39888,#39889,#39890,#39891,#39892,#39893,
#39894,#39895,#39896,#39897,#39898,#39899,#39900,#39901,#39902,#39903,#39904,
#39905,#39906,#39907,#39908,#39909,#39910,#39911,#39912,#39913,#39914,#39915,
#39916,#39917,#39918,#39919,#39920,#39921),.UNSPECIFIED.,.F.,.F.,(4,3,3,
3,3,3,3,3,3,3,3,3,3,3,3,3,3,3,3,3,3,3,3,3,3,3,3,3,3,3,3,3,3,3,3,3,3,3,3,
3,3,3,3,3,3,3,3,3,3,3,3,3,3,3,3,3,3,3,3,3,3,3,4),(7.50078281829221E-8,2.18347309079937E-7,
0.0229487363769535,0.0291144599814069,0.0509742552696368,0.0551846684308731,
0.062499999999996,0.0795332519016023,0.100117540398566,0.102945588654808,
0.109374999999993,0.117187499999992,0.121093749999992,0.123046874999992,
0.124511718749992,0.124999999999992,0.126823526748048,0.154172375961179,
0.168540269274348,0.195094650684728,0.207813798624315,0.234374999999993,
0.243585986145407,0.245603686859174,0.249999999999993,0.28646503409748,
0.323181702761501,0.335381864186567,0.372223006657599,0.396063887874889,
0.433025218886611,0.468749999999996,0.471320710204426,0.484374999999996,
0.492187499999996,0.499324683781458,0.499999999999996,0.539362467141619,
0.553200429548843,0.592481915029558,0.619371300972094,0.65850546985717,
0.673128963060043,0.711994605162659,0.716726220534974,0.718749999999999,
0.734374999999999,0.742187499999999,0.746093749999999,0.749489064792616,
0.749999999999999,0.753696015195325,0.789783408896454,0.822481143086698,
0.851891042285857,0.878120703107442,0.901492063881429,0.9224109344836,0.941272872505627,
0.958424456266756,0.974021159408361,0.988170760125037,1.),.UNSPECIFIED.);
#707=B_SPLINE_CURVE_WITH_KNOTS('',3,(#39958,#39959,#39960,#39961,#39962,
#39963,#39964,#39965,#39966,#39967),.UNSPECIFIED.,.F.,.F.,(4,2,2,2,4),(2.21660101455866E-8,
0.25,0.5,0.75,1.),.UNSPECIFIED.);
#708=B_SPLINE_CURVE_WITH_KNOTS('',3,(#39968,#39969,#39970,#39971,#39972,
#39973,#39974,#39975,#39976,#39977,#39978,#39979,#39980,#39981,#39982,#39983,
#39984,#39985,#39986,#39987,#39988,#39989,#39990,#39991,#39992,#39993,#39994,
#39995,#39996,#39997,#39998,#39999,#40000,#40001,#40002,#40003,#40004,#40005,
#40006,#40007,#40008,#40009,#40010,#40011,#40012,#40013,#40014,#40015,#40016,
#40017,#40018,#40019,#40020,#40021,#40022,#40023,#40024,#40025,#40026,#40027,
#40028),.UNSPECIFIED.,.F.,.F.,(4,3,3,3,3,3,3,3,3,3,3,3,3,3,3,3,3,3,3,3,
4),(5.84282689630331E-11,0.10071860689625,0.175359303448125,0.238666822178488,
0.25,0.30143097883946,0.35110935564115,0.400003027959161,0.450001513979581,
0.497450659112773,0.5,0.500002157722716,0.547539602846247,0.598154702134685,
0.647549372595313,0.698774686297657,0.75,0.812847367231791,0.887996855249994,
0.987406130706481,0.99999999994403),.UNSPECIFIED.);
#709=B_SPLINE_CURVE_WITH_KNOTS('',3,(#40071,#40072,#40073,#40074,#40075,
#40076,#40077,#40078,#40079,#40080,#40081,#40082,#40083,#40084,#40085,#40086,
#40087,#40088,#40089,#40090,#40091,#40092,#40093,#40094,#40095,#40096,#40097,
#40098,#40099,#40100,#40101,#40102,#40103,#40104,#40105,#40106,#40107,#40108,
#40109,#40110,#40111,#40112,#40113,#40114,#40115,#40116,#40117,#40118,#40119,
#40120,#40121,#40122,#40123,#40124,#40125,#40126,#40127,#40128,#40129,#40130,
#40131,#40132,#40133,#40134,#40135,#40136,#40137,#40138,#40139,#40140,#40141,
#40142,#40143,#40144,#40145,#40146,#40147,#40148,#40149,#40150,#40151,#40152,
#40153,#40154,#40155,#40156,#40157,#40158,#40159,#40160,#40161,#40162,#40163,
#40164,#40165,#40166,#40167,#40168,#40169,#40170,#40171,#40172,#40173,#40174,
#40175,#40176),.UNSPECIFIED.,.F.,.F.,(4,3,3,3,3,3,3,3,3,3,3,3,3,3,3,3,3,
3,3,3,3,3,3,3,3,3,3,3,3,3,3,3,3,3,3,4),(0.,0.0534073021192575,0.105850843534235,
0.121448216935405,0.124999999999998,0.17639020141179,0.187499999999997,
0.218749999999996,0.234374999999996,0.242187499999996,0.246093749999996,
0.249763585925269,0.249999999999996,0.272897684871302,0.338775824548075,
0.402712273103291,0.425593601158696,0.490426704513184,0.499999999999998,
0.564257404599829,0.574134006701701,0.624999999999999,0.6875,0.71875,0.726818737615628,
0.734375,0.7421875,0.74609375,0.749803046606295,0.75,0.80028432490764,0.851651062187545,
0.878254012626795,0.931592833707594,0.986051689536171,1.),.UNSPECIFIED.);
#710=B_SPLINE_CURVE_WITH_KNOTS('',3,(#40215,#40216,#40217,#40218,#40219,
#40220,#40221,#40222,#40223,#40224,#40225,#40226,#40227,#40228,#40229,#40230,
#40231,#40232,#40233,#40234,#40235,#40236,#40237,#40238,#40239,#40240,#40241,
#40242,#40243,#40244,#40245,#40246,#40247,#40248,#40249,#40250,#40251,#40252,
#40253,#40254,#40255,#40256,#40257,#40258,#40259,#40260,#40261,#40262,#40263),
 .UNSPECIFIED.,.F.,.F.,(4,3,3,3,3,3,3,3,3,3,3,3,3,3,3,3,4),(0.,0.0770829582185647,
0.115833104658598,0.197028807512659,0.249999999999993,0.333153117361608,
0.356333767149255,0.374999999999989,0.422947860085873,0.471329029702914,
0.499999999999989,0.606855024408351,0.708280894829689,0.713710048816712,
0.815228553348316,0.918005904185723,1.),.UNSPECIFIED.);
#711=B_SPLINE_CURVE_WITH_KNOTS('',3,(#40264,#40265,#40266,#40267,#40268,
#40269,#40270),.UNSPECIFIED.,.F.,.F.,(4,3,4),(2.44821180092488E-11,0.5,
0.999999979802023),.UNSPECIFIED.);
#712=B_SPLINE_CURVE_WITH_KNOTS('',3,(#40271,#40272,#40273,#40274,#40275,
#40276,#40277,#40278,#40279,#40280,#40281,#40282,#40283,#40284,#40285,#40286,
#40287,#40288,#40289,#40290,#40291,#40292,#40293,#40294,#40295,#40296,#40297,
#40298,#40299,#40300,#40301,#40302,#40303,#40304,#40305,#40306,#40307,#40308,
#40309,#40310,#40311,#40312,#40313,#40314,#40315,#40316,#40317,#40318,#40319,
#40320,#40321,#40322,#40323,#40324,#40325,#40326,#40327,#40328),
 .UNSPECIFIED.,.F.,.F.,(4,3,3,3,3,3,3,3,3,3,3,3,3,3,3,3,3,3,3,4),(0.,0.0715675761621514,
0.147880847450542,0.168247999802698,0.250000000000023,0.335016489680616,
0.375000000000033,0.399721616125445,0.437500000000038,0.468750000000039,
0.48437500000004,0.49533835708464,0.500000000000041,0.593368467641783,0.631329958382462,
0.726440385039814,0.827653147299548,0.852289986581864,0.957929667074719,
1.),.UNSPECIFIED.);
#713=B_SPLINE_CURVE_WITH_KNOTS('',3,(#40371,#40372,#40373,#40374,#40375,
#40376,#40377,#40378,#40379,#40380,#40381,#40382,#40383,#40384,#40385,#40386,
#40387,#40388,#40389,#40390,#40391,#40392),.UNSPECIFIED.,.F.,.F.,(4,3,3,
3,3,3,3,4),(1.01036450470102E-7,0.1428571428571,0.2857142857143,0.4285714285714,
0.5714285714286,0.7142857142857,0.8571428571429,1.),.UNSPECIFIED.);
#714=B_SPLINE_CURVE_WITH_KNOTS('',3,(#40435,#40436,#40437,#40438,#40439,
#40440,#40441),.UNSPECIFIED.,.F.,.F.,(4,3,4),(2.1506060516552E-8,0.5,0.99999999998187),
 .UNSPECIFIED.);
#715=B_SPLINE_CURVE_WITH_KNOTS('',3,(#40443,#40444,#40445,#40446,#40447,
#40448,#40449,#40450,#40451,#40452,#40453,#40454,#40455,#40456,#40457,#40458,
#40459,#40460,#40461,#40462,#40463,#40464,#40465,#40466,#40467,#40468,#40469,
#40470,#40471,#40472,#40473,#40474,#40475,#40476,#40477,#40478,#40479,#40480,
#40481,#40482,#40483,#40484,#40485),.UNSPECIFIED.,.F.,.F.,(4,3,3,3,3,3,
3,3,3,3,3,3,3,3,4),(0.,0.0900137143300672,0.116403415329186,0.243030893620983,
0.25,0.360149316915376,0.4375,0.466162190612914,0.495189352431254,0.5,0.615787612830892,
0.712806427318202,0.822400533667193,0.928574394609824,1.),.UNSPECIFIED.);
#716=B_SPLINE_CURVE_WITH_KNOTS('',3,(#40486,#40487,#40488,#40489,#40490,
#40491,#40492,#40493,#40494,#40495,#40496,#40497,#40498,#40499,#40500,#40501,
#40502,#40503,#40504,#40505,#40506,#40507,#40508,#40509,#40510,#40511,#40512,
#40513,#40514,#40515,#40516,#40517,#40518,#40519,#40520,#40521,#40522,#40523,
#40524,#40525,#40526,#40527,#40528,#40529,#40530,#40531,#40532,#40533,#40534,
#40535,#40536,#40537,#40538,#40539,#40540,#40541,#40542,#40543),
 .UNSPECIFIED.,.F.,.F.,(4,3,3,3,3,3,3,3,3,3,3,3,3,3,3,3,3,3,3,4),(0.,0.105620946107267,
0.147712755041571,0.250000000000056,0.345332766185357,0.368665276576495,
0.375000000000084,0.437500000000099,0.468750000000106,0.484375000000107,
0.494735183221286,0.500000000000108,0.589017398444796,0.600284329803979,
0.686110181738736,0.750000000000054,0.831760754742984,0.908457269195526,
0.980208706438598,1.),.UNSPECIFIED.);
#717=B_SPLINE_CURVE_WITH_KNOTS('',3,(#40585,#40586,#40587,#40588,#40589,
#40590,#40591,#40592,#40593,#40594,#40595,#40596,#40597,#40598,#40599,#40600,
#40601,#40602,#40603,#40604,#40605,#40606),.UNSPECIFIED.,.F.,.F.,(4,3,3,
3,3,3,3,4),(0.,0.1428571428571,0.2857142857143,0.4285714285714,0.5714285714286,
0.7142857142857,0.8571428571429,0.999999898936422),.UNSPECIFIED.);
#718=B_SPLINE_CURVE_WITH_KNOTS('',3,(#40609,#40610,#40611,#40612,#40613,
#40614,#40615,#40616,#40617,#40618),.UNSPECIFIED.,.F.,.F.,(4,2,2,2,4),(0.,
0.25,0.5,0.75,0.999999977827818),.UNSPECIFIED.);
#719=B_SPLINE_CURVE_WITH_KNOTS('',3,(#40648,#40649,#40650,#40651,#40652,
#40653,#40654,#40655,#40656,#40657,#40658,#40659,#40660),.UNSPECIFIED.,
 .F.,.F.,(4,3,3,3,4),(0.,0.0431918509093698,0.5,0.956806409091625,1.),
 .UNSPECIFIED.);
#720=B_SPLINE_CURVE_WITH_KNOTS('',3,(#40681,#40682,#40683,#40684,#40685,
#40686,#40687,#40688,#40689,#40690,#40691,#40692,#40693,#40694,#40695,#40696,
#40697,#40698,#40699,#40700,#40701,#40702,#40703,#40704,#40705,#40706,#40707,
#40708,#40709,#40710,#40711,#40712,#40713,#40714,#40715,#40716,#40717,#40718,
#40719,#40720,#40721,#40722,#40723,#40724,#40725,#40726,#40727,#40728,#40729,
#40730,#40731,#40732,#40733,#40734,#40735,#40736,#40737,#40738,#40739,#40740,
#40741,#40742,#40743,#40744,#40745,#40746,#40747,#40748,#40749,#40750,#40751,
#40752,#40753,#40754,#40755,#40756,#40757,#40758,#40759,#40760,#40761,#40762,
#40763,#40764,#40765,#40766,#40767,#40768,#40769,#40770,#40771,#40772,#40773,
#40774,#40775,#40776,#40777,#40778,#40779,#40780,#40781,#40782,#40783,#40784,
#40785,#40786,#40787,#40788,#40789,#40790,#40791,#40792,#40793,#40794,#40795,
#40796,#40797,#40798,#40799,#40800,#40801,#40802,#40803,#40804,#40805,#40806,
#40807,#40808,#40809,#40810,#40811,#40812,#40813,#40814,#40815,#40816,#40817,
#40818,#40819,#40820,#40821,#40822,#40823,#40824,#40825,#40826,#40827,#40828,
#40829,#40830,#40831,#40832,#40833,#40834,#40835,#40836,#40837,#40838,#40839,
#40840,#40841,#40842,#40843,#40844,#40845,#40846,#40847,#40848,#40849,#40850,
#40851,#40852,#40853,#40854,#40855,#40856,#40857,#40858,#40859,#40860,#40861,
#40862,#40863,#40864,#40865,#40866,#40867,#40868,#40869,#40870,#40871,#40872,
#40873,#40874,#40875,#40876,#40877,#40878,#40879,#40880,#40881,#40882,#40883,
#40884,#40885),.UNSPECIFIED.,.F.,.F.,(4,3,3,3,3,3,3,3,3,3,3,3,3,3,3,3,3,
3,3,3,3,3,3,3,3,3,3,3,3,3,3,3,3,3,3,3,3,3,3,3,3,3,3,3,3,3,3,3,3,3,3,3,3,
3,3,3,3,3,3,3,3,3,3,3,3,3,3,3,4),(0.,0.0249899757898509,0.0498925985927389,
0.0680547145672805,0.0924380116089264,0.107884502821677,0.131552669723352,
0.140982390017907,0.163949714740866,0.171027459458805,0.19333313068864,
0.199601692626754,0.218749999999987,0.227584804003973,0.234374999999986,
0.242187499999986,0.246093749999986,0.248046874999986,0.249023437499986,
0.249999999999986,0.254563033347897,0.279986528061362,0.307418668000935,
0.309444125572636,0.337138172534275,0.344177504666389,0.372012337381321,
0.384925968447627,0.41257692077012,0.429852529706512,0.457852628540933,
0.468749999999996,0.477253131218569,0.484374999999997,0.492187499999998,
0.496093749999998,0.498046874999998,0.499999999999998,0.531304980715094,
0.565655536933447,0.578514455459115,0.613128561202045,0.616399033761582,
0.648094081067902,0.674913002638068,0.697972341505022,0.718054360421838,
0.718750000000008,0.734375000000008,0.735675698049429,0.742187500000009,
0.746093750000009,0.748046875000009,0.749023437500009,0.750000000000009,
0.75183323557947,0.773849534001207,0.795129686077898,0.815764243845486,
0.835870588208117,0.855602251914255,0.875000000000005,0.875163715889217,
0.894776692921227,0.914588112884019,0.93477223603792,0.955588003084658,
0.977473939702512,0.999999988549721),.UNSPECIFIED.);
#721=B_SPLINE_CURVE_WITH_KNOTS('',3,(#41048,#41049,#41050,#41051,#41052,
#41053,#41054,#41055,#41056,#41057,#41058,#41059,#41060,#41061,#41062,#41063,
#41064,#41065,#41066,#41067,#41068,#41069,#41070,#41071,#41072,#41073,#41074,
#41075,#41076,#41077,#41078,#41079,#41080,#41081,#41082,#41083,#41084,#41085,
#41086,#41087,#41088,#41089,#41090,#41091,#41092,#41093,#41094,#41095,#41096,
#41097,#41098,#41099,#41100,#41101,#41102,#41103,#41104,#41105,#41106,#41107,
#41108,#41109,#41110,#41111,#41112,#41113,#41114,#41115,#41116,#41117,#41118,
#41119,#41120,#41121,#41122,#41123,#41124,#41125,#41126,#41127,#41128,#41129,
#41130,#41131,#41132,#41133,#41134,#41135,#41136,#41137,#41138,#41139,#41140,
#41141,#41142,#41143,#41144,#41145,#41146,#41147,#41148,#41149,#41150,#41151,
#41152,#41153,#41154,#41155,#41156,#41157,#41158,#41159,#41160,#41161,#41162,
#41163,#41164,#41165,#41166,#41167,#41168),.UNSPECIFIED.,.F.,.F.,(4,3,3,
3,3,3,3,3,3,3,3,3,3,3,3,3,3,3,3,3,3,3,3,3,3,3,3,3,3,3,3,3,3,3,3,3,3,3,3,
3,4),(7.98332591227906E-8,0.0312500598749484,0.0618422377334466,0.0934211188667314,
0.125000000000016,0.155569262381823,0.187159631190926,0.218750000000029,
0.234375000000031,0.242187500000032,0.246093750000032,0.248046875000032,
0.249023437500033,0.250000000000033,0.450348688189998,0.499981342333456,
0.500000000000063,0.625000000000078,0.687500000000086,0.71875000000009,
0.734375000000092,0.742187500000092,0.749511718750093,0.750000000000093,
0.76591902426714,0.781838226860177,0.797757617896502,0.813677320857265,
0.829597203658077,0.845517389752812,0.859375000000061,0.867187500000059,
0.871093750000058,0.873046875000057,0.874023437500057,0.875000000000056,
0.899836748384693,0.924877547569079,0.949727712244665,0.974863828683451,
0.999999945122236),.UNSPECIFIED.);
#722=B_SPLINE_CURVE_WITH_KNOTS('',3,(#41209,#41210,#41211,#41212,#41213,
#41214,#41215,#41216,#41217,#41218,#41219,#41220,#41221,#41222,#41223,#41224,
#41225,#41226,#41227,#41228,#41229,#41230,#41231,#41232,#41233,#41234,#41235,
#41236,#41237,#41238,#41239,#41240,#41241,#41242,#41243,#41244,#41245,#41246,
#41247,#41248,#41249,#41250,#41251,#41252,#41253,#41254,#41255,#41256,#41257),
 .UNSPECIFIED.,.F.,.F.,(4,3,3,3,3,3,3,3,3,3,3,3,3,3,3,3,4),(0.,0.0771290273449875,
0.118224704472258,0.199429219826042,0.250000000000003,0.333192555504809,
0.359720294597202,0.375000000000003,0.422998467267463,0.471431284351993,
0.500000000000003,0.602025867947538,0.703467460959905,0.719209589455199,
0.820753199246495,0.923561758329389,1.),.UNSPECIFIED.);
#723=B_SPLINE_CURVE_WITH_KNOTS('',3,(#41259,#41260,#41261,#41262,#41263,
#41264,#41265),.UNSPECIFIED.,.F.,.F.,(4,3,4),(2.58811215489952E-11,0.5,
1.),.UNSPECIFIED.);
#724=B_SPLINE_CURVE_WITH_KNOTS('',3,(#41268,#41269,#41270,#41271,#41272,
#41273,#41274,#41275,#41276,#41277,#41278,#41279,#41280,#41281,#41282,#41283,
#41284,#41285,#41286,#41287,#41288,#41289,#41290,#41291,#41292,#41293,#41294,
#41295,#41296,#41297,#41298,#41299,#41300,#41301,#41302,#41303,#41304,#41305,
#41306,#41307,#41308,#41309,#41310,#41311,#41312,#41313,#41314,#41315,#41316,
#41317,#41318,#41319,#41320,#41321,#41322,#41323,#41324,#41325,#41326,#41327,
#41328),.UNSPECIFIED.,.F.,.F.,(4,3,3,3,3,3,3,3,3,3,3,3,3,3,3,3,3,3,3,3,
4),(0.,0.0723226571286148,0.149373391393564,0.166421306541277,0.245216470047908,
0.249999999999981,0.335716357982209,0.374999999999975,0.397180576939525,
0.437499999999972,0.468749999999974,0.484374999999974,0.495375838037244,
0.499999999999974,0.593362829860859,0.628795108092315,0.723805230530685,
0.824915540841586,0.849552880666,0.955120161906881,1.),.UNSPECIFIED.);
#725=B_SPLINE_CURVE_WITH_KNOTS('',3,(#41369,#41370,#41371,#41372,#41373,
#41374,#41375,#41376,#41377,#41378,#41379,#41380,#41381,#41382,#41383,#41384,
#41385,#41386,#41387,#41388,#41389,#41390,#41391,#41392,#41393,#41394,#41395,
#41396,#41397,#41398,#41399,#41400,#41401,#41402,#41403,#41404,#41405,#41406,
#41407,#41408,#41409,#41410,#41411),.UNSPECIFIED.,.F.,.F.,(4,3,3,3,3,3,
3,3,3,3,3,3,3,3,4),(1.98991421892558E-11,0.0832138081695056,0.218577781387173,
0.246109287404286,0.25,0.383459488805014,0.408370299490802,0.541180660031661,
0.570056215972447,0.702294214224038,0.731364949239141,0.75,0.881938328104128,
0.892442289703727,0.999999987394212),.UNSPECIFIED.);
#726=B_SPLINE_CURVE_WITH_KNOTS('',3,(#41412,#41413,#41414,#41415,#41416,
#41417,#41418,#41419,#41420,#41421,#41422,#41423,#41424,#41425,#41426,#41427,
#41428,#41429,#41430,#41431,#41432,#41433,#41434,#41435,#41436,#41437,#41438,
#41439,#41440,#41441,#41442,#41443,#41444,#41445,#41446,#41447,#41448,#41449,
#41450,#41451,#41452,#41453,#41454,#41455,#41456,#41457,#41458,#41459,#41460,
#41461,#41462,#41463,#41464,#41465,#41466,#41467,#41468,#41469,#41470,#41471,
#41472,#41473,#41474,#41475,#41476,#41477,#41478,#41479,#41480,#41481,#41482,
#41483,#41484,#41485,#41486,#41487,#41488,#41489,#41490),.UNSPECIFIED.,
 .F.,.F.,(4,3,3,3,3,3,3,3,3,3,3,3,3,3,3,3,3,3,3,3,3,3,3,3,3,3,4),(0.,0.0457810663886033,
0.0917889143557284,0.120317290916942,0.1428571428571,0.198222944263035,
0.253550325472813,0.275526256355525,0.2857142857143,0.349641048844645,0.413645189546886,
0.4285714285714,0.43059760945638,0.496176324094908,0.561795552695129,0.5714285714286,
0.585374526667842,0.649830120476771,0.7142857142857,0.740396273234167,0.795252877507973,
0.850177989909437,0.8571428571429,0.895765393025868,0.941863426735384,0.987754574515315,
0.999999797061845),.UNSPECIFIED.);
#727=B_SPLINE_CURVE_WITH_KNOTS('',3,(#41526,#41527,#41528,#41529,#41530,
#41531,#41532,#41533,#41534,#41535,#41536,#41537,#41538,#41539,#41540,#41541,
#41542,#41543,#41544,#41545,#41546,#41547,#41548,#41549,#41550,#41551,#41552,
#41553,#41554,#41555,#41556,#41557,#41558,#41559,#41560,#41561,#41562,#41563,
#41564,#41565,#41566,#41567,#41568,#41569,#41570,#41571,#41572,#41573,#41574,
#41575,#41576,#41577,#41578,#41579,#41580,#41581,#41582,#41583,#41584,#41585,
#41586),.UNSPECIFIED.,.F.,.F.,(4,3,3,3,3,3,3,3,3,3,3,3,3,3,3,3,3,3,3,3,
4),(5.47317109184868E-11,0.100716841584173,0.175358420792086,0.238665162138364,
0.25,0.301434484455404,0.351116096330567,0.400012858909411,0.450006429454706,
0.497458494136093,0.5,0.500001657323632,0.547542156254057,0.598156617190543,
0.647554747965031,0.698777373982516,0.75,0.812847460886534,0.887994716881443,
0.987407949822264,0.999999999957208),.UNSPECIFIED.);
#728=B_SPLINE_CURVE_WITH_KNOTS('',3,(#41627,#41628,#41629,#41630,#41631,
#41632,#41633,#41634,#41635,#41636,#41637,#41638,#41639,#41640,#41641,#41642,
#41643,#41644,#41645,#41646,#41647,#41648,#41649,#41650,#41651,#41652,#41653,
#41654,#41655,#41656,#41657,#41658,#41659,#41660,#41661,#41662,#41663,#41664,
#41665,#41666,#41667,#41668,#41669,#41670,#41671,#41672,#41673,#41674,#41675,
#41676,#41677,#41678,#41679,#41680,#41681,#41682,#41683,#41684,#41685,#41686,
#41687,#41688,#41689,#41690,#41691,#41692,#41693,#41694,#41695,#41696,#41697,
#41698,#41699,#41700,#41701,#41702,#41703,#41704,#41705,#41706,#41707,#41708,
#41709,#41710,#41711,#41712,#41713,#41714,#41715,#41716,#41717,#41718,#41719,
#41720,#41721,#41722,#41723,#41724,#41725,#41726,#41727,#41728,#41729,#41730,
#41731,#41732),.UNSPECIFIED.,.F.,.F.,(4,3,3,3,3,3,3,3,3,3,3,3,3,3,3,3,3,
3,3,3,3,3,3,3,3,3,3,3,3,3,3,3,3,3,3,4),(0.,0.053257050465951,0.105540886337049,
0.12396561413214,0.124999999999997,0.176282843367685,0.187499999999996,
0.218749999999995,0.234374999999995,0.242187499999994,0.246093749999994,
0.249704840463526,0.249999999999994,0.274255888483978,0.340144308274661,
0.404109232423276,0.426142645440888,0.490995077175135,0.499999999999994,
0.564437556258508,0.574120495681384,0.624999999999994,0.687499999999994,
0.718749999999994,0.726015446468681,0.734374999999994,0.742187499999994,
0.746093749999994,0.749746192108767,0.749999999999994,0.800189142872996,
0.851447051024866,0.876295161158848,0.929482782934934,0.983795496276306,
1.),.UNSPECIFIED.);
#729=B_SPLINE_CURVE_WITH_KNOTS('',3,(#41773,#41774,#41775,#41776,#41777,
#41778,#41779),.UNSPECIFIED.,.F.,.F.,(4,3,4),(0.,0.5,1.),.UNSPECIFIED.);
#730=B_SPLINE_CURVE_WITH_KNOTS('',3,(#41781,#41782,#41783,#41784,#41785,
#41786,#41787,#41788,#41789,#41790,#41791,#41792,#41793,#41794,#41795,#41796,
#41797,#41798,#41799,#41800,#41801,#41802,#41803,#41804,#41805,#41806,#41807,
#41808,#41809,#41810,#41811,#41812,#41813,#41814,#41815,#41816,#41817,#41818,
#41819,#41820),.UNSPECIFIED.,.F.,.F.,(4,3,3,3,3,3,3,3,3,3,3,3,3,4),(0.,
0.0902369168203611,0.118370167438031,0.25,0.36295411350154,0.4375,0.466154710754423,
0.495174404959947,0.499999999999999,0.615785132678318,0.717634497424337,
0.827090029722756,0.933176968893971,1.),.UNSPECIFIED.);
#731=B_SPLINE_CURVE_WITH_KNOTS('',3,(#41821,#41822,#41823,#41824,#41825,
#41826,#41827,#41828,#41829,#41830,#41831,#41832,#41833,#41834,#41835,#41836,
#41837,#41838,#41839,#41840,#41841,#41842,#41843,#41844,#41845,#41846,#41847,
#41848,#41849,#41850,#41851,#41852,#41853,#41854,#41855,#41856,#41857,#41858,
#41859,#41860,#41861,#41862,#41863,#41864,#41865,#41866,#41867,#41868,#41869,
#41870,#41871,#41872,#41873,#41874,#41875,#41876,#41877,#41878),
 .UNSPECIFIED.,.F.,.F.,(4,3,3,3,3,3,3,3,3,3,3,3,3,3,3,3,3,3,3,4),(0.,0.105589045184164,
0.149929520074555,0.249999999999981,0.345340162396845,0.370793467763536,
0.374999999999975,0.437499999999971,0.46874999999997,0.484374999999968,
0.494783657022549,0.499999999999967,0.589543647990068,0.60253603942224,
0.690095556674877,0.770652073013828,0.833509297677349,0.91080736609718,
0.983185422022552,1.),.UNSPECIFIED.);
#732=B_SPLINE_CURVE_WITH_KNOTS('',3,(#41924,#41925,#41926,#41927,#41928,
#41929,#41930,#41931,#41932,#41933,#41934,#41935,#41936,#41937,#41938,#41939,
#41940,#41941,#41942,#41943,#41944,#41945,#41946,#41947,#41948,#41949,#41950,
#41951,#41952,#41953,#41954,#41955,#41956,#41957,#41958,#41959,#41960,#41961,
#41962,#41963,#41964,#41965,#41966,#41967,#41968,#41969,#41970,#41971,#41972,
#41973,#41974,#41975,#41976,#41977,#41978,#41979,#41980,#41981,#41982,#41983,
#41984,#41985,#41986,#41987,#41988,#41989,#41990,#41991,#41992,#41993,#41994,
#41995,#41996),.UNSPECIFIED.,.F.,.F.,(4,3,3,3,3,3,3,3,3,3,3,3,3,3,3,3,3,
3,3,3,3,3,3,3,4),(0.,0.0458328892255905,0.0918178602187016,0.137727870872198,
0.1428571428571,0.148536598132459,0.203804992720327,0.259124754682715,0.2857142857143,
0.296137570174044,0.362354499372722,0.4285714285714,0.443717909280033,0.511006798196311,
0.5714285714286,0.591516277431717,0.658633939622798,0.7142857142857,0.739436741599132,
0.798289799371016,0.8571428571429,0.88721304215739,0.933524276536456,0.979590782851303,
1.),.UNSPECIFIED.);
#733=B_SPLINE_CURVE_WITH_KNOTS('',3,(#41999,#42000,#42001,#42002,#42003,
#42004,#42005,#42006,#42007,#42008,#42009,#42010,#42011,#42012,#42013,#42014,
#42015,#42016,#42017,#42018,#42019,#42020,#42021,#42022,#42023,#42024,#42025,
#42026,#42027,#42028,#42029,#42030,#42031,#42032,#42033,#42034,#42035,#42036,
#42037,#42038),.UNSPECIFIED.,.F.,.F.,(4,3,3,3,3,3,3,3,3,3,3,3,3,4),(0.,
0.132990604309484,0.153369582850421,0.28898480733553,0.306719319059886,
0.443622692112419,0.460361902236848,0.597256092732825,0.614811263154823,
0.75,0.769627679030996,0.909368696860574,0.924609571052109,0.999999999960875),
 .UNSPECIFIED.);
#734=B_SPLINE_CURVE_WITH_KNOTS('',3,(#42061,#42062,#42063,#42064,#42065,
#42066,#42067,#42068,#42069,#42070),.UNSPECIFIED.,.F.,.F.,(4,3,3,4),(0.,
0.3333333333333,0.6666666666667,1.),.UNSPECIFIED.);
#735=B_SPLINE_CURVE_WITH_KNOTS('',3,(#42206,#42207,#42208,#42209,#42210,
#42211,#42212,#42213,#42214,#42215,#42216,#42217,#42218,#42219,#42220,#42221,
#42222,#42223,#42224,#42225,#42226,#42227,#42228,#42229,#42230,#42231,#42232,
#42233,#42234,#42235,#42236,#42237,#42238,#42239,#42240,#42241,#42242,#42243,
#42244,#42245,#42246,#42247,#42248,#42249,#42250,#42251,#42252,#42253,#42254,
#42255,#42256,#42257,#42258,#42259,#42260,#42261,#42262,#42263,#42264,#42265,
#42266,#42267,#42268,#42269,#42270,#42271,#42272,#42273,#42274,#42275,#42276,
#42277,#42278,#42279,#42280,#42281,#42282,#42283,#42284,#42285,#42286,#42287,
#42288,#42289,#42290,#42291,#42292,#42293),.UNSPECIFIED.,.F.,.F.,(4,2,2,
1,2,2,2,1,1,1,2,2,2,2,1,1,1,2,2,2,2,2,2,2,2,2,1,2,2,2,1,1,2,2,2,2,1,1,2,
2,2,2,1,1,2,2,2,1,1,2,2,4),(0.,0.03125,0.046875,0.0546874999999999,0.0585937499999999,
0.0624999999999999,0.0937499999999991,0.109374999999999,0.117187499999998,
0.121093749999998,0.123046874999998,0.124999999999998,0.187499999999997,
0.218749999999997,0.234374999999997,0.242187499999997,0.246093749999997,
0.248046874999997,0.249999999999997,0.312500000000001,0.343750000000002,
0.359375000000003,0.375000000000004,0.437500000000007,0.468750000000008,
0.484375000000009,0.49218750000001,0.49609375000001,0.50000000000001,0.562500000000013,
0.593750000000014,0.609375000000015,0.617187500000016,0.625000000000016,
0.687500000000019,0.71875000000002,0.734375000000021,0.742187500000021,
0.746093750000021,0.750000000000021,0.812500000000022,0.843750000000022,
0.859375000000022,0.867187500000022,0.871093750000022,0.875000000000021,
0.906250000000017,0.921875000000014,0.929687500000013,0.933593750000012,
0.937500000000011,1.),.UNSPECIFIED.);
#736=B_SPLINE_CURVE_WITH_KNOTS('',3,(#42296,#42297,#42298,#42299,#42300,
#42301,#42302,#42303,#42304,#42305,#42306,#42307,#42308,#42309,#42310,#42311,
#42312,#42313,#42314,#42315,#42316,#42317,#42318,#42319,#42320,#42321,#42322,
#42323,#42324,#42325,#42326,#42327,#42328,#42329,#42330,#42331,#42332,#42333,
#42334,#42335,#42336,#42337,#42338,#42339,#42340,#42341,#42342,#42343,#42344,
#42345,#42346,#42347,#42348,#42349,#42350,#42351,#42352,#42353,#42354,#42355,
#42356,#42357,#42358,#42359,#42360,#42361,#42362,#42363,#42364,#42365,#42366,
#42367,#42368,#42369,#42370,#42371,#42372,#42373,#42374,#42375,#42376,#42377,
#42378,#42379,#42380,#42381,#42382,#42383,#42384,#42385,#42386,#42387,#42388,
#42389,#42390,#42391,#42392,#42393,#42394,#42395,#42396,#42397,#42398,#42399,
#42400,#42401,#42402,#42403,#42404,#42405,#42406,#42407,#42408,#42409,#42410,
#42411,#42412,#42413,#42414,#42415,#42416,#42417,#42418,#42419,#42420,#42421,
#42422,#42423,#42424,#42425,#42426,#42427,#42428,#42429,#42430,#42431,#42432,
#42433,#42434,#42435,#42436,#42437,#42438,#42439,#42440,#42441,#42442,#42443,
#42444,#42445,#42446,#42447,#42448,#42449,#42450,#42451,#42452,#42453,#42454,
#42455,#42456,#42457,#42458,#42459,#42460,#42461,#42462,#42463,#42464,#42465,
#42466,#42467,#42468,#42469,#42470,#42471,#42472,#42473,#42474,#42475,#42476,
#42477,#42478,#42479,#42480,#42481,#42482),.UNSPECIFIED.,.F.,.F.,(4,3,3,
3,3,3,3,3,3,3,3,3,3,3,3,3,3,3,3,3,3,3,3,3,3,3,3,3,3,3,3,3,3,3,3,3,3,3,3,
3,3,3,3,3,3,3,3,3,3,3,3,3,3,3,3,3,3,3,3,3,3,3,4),(7.50080231389504E-8,2.18347877829989E-7,
0.0229487004070204,0.0291148588785608,0.0509746146692638,0.0551851739629441,
0.0625000000000166,0.0795336635547587,0.100117921827564,0.102945846128966,
0.109375000000029,0.117187500000031,0.121093750000032,0.123046875000033,
0.124511718750033,0.125000000000033,0.126823712684557,0.154172414242767,
0.168540255145738,0.195094495105245,0.207813480733301,0.234375000000029,
0.243585926132158,0.24560283163885,0.250000000000028,0.286463023045781,
0.323179567483026,0.335377806100086,0.372218834583004,0.396057559740644,
0.433018802754509,0.46875000000002,0.47131279681658,0.484375000000019,0.492187500000019,
0.499324279379621,0.500000000000018,0.539362840686631,0.553194038309196,
0.592475975376577,0.619367181733849,0.658501763493894,0.673126718677383,
0.711992777641369,0.716725120819943,0.718750000000009,0.734375000000009,
0.742187500000009,0.746093750000008,0.749489103071601,0.750000000000008,
0.753695598866092,0.789783387614058,0.822481343688618,0.851891345405229,
0.87812104190446,0.901492399765885,0.922411241342964,0.941273136670307,
0.958424669511547,0.974021299622459,0.988170798160383,1.),.UNSPECIFIED.);
#737=B_SPLINE_CURVE_WITH_KNOTS('',3,(#42519,#42520,#42521,#42522,#42523,
#42524,#42525,#42526,#42527,#42528),.UNSPECIFIED.,.F.,.F.,(4,2,2,2,4),(2.2166076873242E-8,
0.25,0.5,0.75,1.),.UNSPECIFIED.);
#738=B_SPLINE_CURVE_WITH_KNOTS('',3,(#42529,#42530,#42531,#42532,#42533,
#42534,#42535,#42536,#42537,#42538,#42539,#42540,#42541,#42542,#42543,#42544,
#42545,#42546,#42547,#42548,#42549,#42550,#42551,#42552,#42553,#42554,#42555,
#42556,#42557,#42558,#42559,#42560,#42561,#42562,#42563,#42564,#42565,#42566,
#42567,#42568,#42569,#42570,#42571,#42572,#42573,#42574,#42575,#42576,#42577,
#42578,#42579,#42580,#42581,#42582,#42583,#42584,#42585,#42586,#42587,#42588,
#42589),.UNSPECIFIED.,.F.,.F.,(4,3,3,3,3,3,3,3,3,3,3,3,3,3,3,3,3,3,3,3,
4),(7.25467506948197E-11,0.100714571809277,0.175357285904639,0.238677150602764,
0.25,0.301434921986588,0.351121064526266,0.400024066781372,0.450012033390686,
0.497473671964868,0.5,0.500002027333907,0.547551851798238,0.598163888848679,
0.647567147211436,0.698783573605718,0.75,0.812861036075596,0.888030478108711,
0.987429614109391,0.999999999930326),.UNSPECIFIED.);
#739=B_SPLINE_CURVE_WITH_KNOTS('',3,(#42636,#42637,#42638,#42639,#42640,
#42641,#42642,#42643,#42644,#42645,#42646,#42647,#42648,#42649,#42650,#42651,
#42652,#42653,#42654,#42655,#42656,#42657,#42658,#42659,#42660,#42661,#42662,
#42663,#42664,#42665,#42666,#42667,#42668,#42669,#42670,#42671,#42672,#42673,
#42674,#42675,#42676,#42677,#42678,#42679,#42680,#42681,#42682,#42683,#42684,
#42685,#42686,#42687,#42688,#42689,#42690,#42691,#42692,#42693,#42694,#42695,
#42696,#42697,#42698,#42699,#42700,#42701,#42702,#42703,#42704,#42705,#42706,
#42707,#42708,#42709,#42710,#42711,#42712,#42713,#42714,#42715,#42716,#42717),
 .UNSPECIFIED.,.F.,.F.,(4,3,3,3,3,3,3,3,3,3,3,3,3,3,3,3,3,3,3,3,3,3,3,3,
3,3,3,4),(0.,0.0598753172964264,0.125,0.1875,0.208388761471869,0.21875,
0.234375,0.244077550301959,0.25,0.317441934267976,0.355226492165471,0.421839748974101,
0.488155247822196,0.499851881816781,0.499999999999999,0.564309740464253,
0.624999999999999,0.644482028662084,0.687499999999999,0.718749999999999,
0.734374999999999,0.744118095785684,0.749999999999999,0.791308742059749,
0.855329516807886,0.921469561084981,0.939826496901372,0.999999999999963),
 .UNSPECIFIED.);
#740=B_SPLINE_CURVE_WITH_KNOTS('',3,(#42756,#42757,#42758,#42759,#42760,
#42761,#42762,#42763,#42764,#42765,#42766,#42767,#42768,#42769,#42770,#42771,
#42772,#42773,#42774,#42775,#42776,#42777,#42778,#42779,#42780,#42781,#42782,
#42783,#42784,#42785,#42786,#42787,#42788,#42789,#42790,#42791,#42792,#42793,
#42794,#42795,#42796,#42797,#42798,#42799,#42800,#42801),.UNSPECIFIED.,
 .F.,.F.,(4,3,3,3,3,3,3,3,3,3,3,3,3,3,3,4),(0.,0.0770736690795171,0.11540458327814,
0.19659836676276,0.249999999999999,0.333146148439707,0.355774863218928,
0.374999999999999,0.422940018737277,0.471313219975339,0.499999999999999,
0.606506586343226,0.713013172686453,0.814528961412497,0.917302819950146,
1.),.UNSPECIFIED.);
#741=B_SPLINE_CURVE_WITH_KNOTS('',3,(#42802,#42803,#42804,#42805,#42806,
#42807,#42808),.UNSPECIFIED.,.F.,.F.,(4,3,4),(0.,0.5,0.999999975355396),
 .UNSPECIFIED.);
#742=B_SPLINE_CURVE_WITH_KNOTS('',3,(#42809,#42810,#42811,#42812,#42813,
#42814,#42815,#42816,#42817,#42818,#42819,#42820,#42821,#42822,#42823,#42824,
#42825,#42826,#42827,#42828,#42829,#42830,#42831,#42832,#42833,#42834,#42835,
#42836,#42837,#42838,#42839,#42840,#42841,#42842,#42843,#42844,#42845,#42846,
#42847,#42848,#42849,#42850,#42851,#42852,#42853,#42854,#42855,#42856,#42857,
#42858,#42859,#42860,#42861,#42862,#42863,#42864,#42865,#42866),
 .UNSPECIFIED.,.F.,.F.,(4,3,3,3,3,3,3,3,3,3,3,3,3,3,3,3,3,3,3,4),(0.,0.0715177076076025,
0.147781603164113,0.168373690108482,0.25000000000002,0.334962898290653,
0.375000000000031,0.400046415107386,0.437500000000033,0.468750000000035,
0.484375000000036,0.495337496274554,0.500000000000038,0.593386942558541,
0.631716791369734,0.726860228272911,0.828107710230089,0.852770844187471,
0.958441713256798,1.),.UNSPECIFIED.);
#743=B_SPLINE_CURVE_WITH_KNOTS('',3,(#42909,#42910,#42911,#42912,#42913,
#42914,#42915,#42916,#42917,#42918,#42919,#42920,#42921,#42922,#42923,#42924,
#42925,#42926,#42927,#42928,#42929,#42930),.UNSPECIFIED.,.F.,.F.,(4,3,3,
3,3,3,3,4),(1.01038589610438E-7,0.1428571428571,0.2857142857143,0.4285714285714,
0.5714285714286,0.7142857142857,0.8571428571429,1.),.UNSPECIFIED.);
#744=B_SPLINE_CURVE_WITH_KNOTS('',3,(#42973,#42974,#42975,#42976,#42977,
#42978,#42979),.UNSPECIFIED.,.F.,.F.,(4,3,4),(2.15062665969218E-8,0.5,0.999999999974515),
 .UNSPECIFIED.);
#745=B_SPLINE_CURVE_WITH_KNOTS('',3,(#42981,#42982,#42983,#42984,#42985,
#42986,#42987,#42988,#42989,#42990,#42991,#42992,#42993,#42994,#42995,#42996,
#42997,#42998,#42999,#43000,#43001,#43002,#43003,#43004,#43005,#43006,#43007,
#43008,#43009,#43010,#43011,#43012,#43013,#43014,#43015,#43016,#43017,#43018,
#43019,#43020,#43021,#43022,#43023),.UNSPECIFIED.,.F.,.F.,(4,3,3,3,3,3,
3,3,3,3,3,3,3,3,4),(0.,0.0900140533241843,0.116403794824626,0.243031863324909,
0.250000000000001,0.360150451046764,0.437499999999997,0.466162821938923,
0.495190581692203,0.499999999999996,0.615787326593693,0.712807369725428,
0.822401125042849,0.928574641518961,1.),.UNSPECIFIED.);
#746=B_SPLINE_CURVE_WITH_KNOTS('',3,(#43024,#43025,#43026,#43027,#43028,
#43029,#43030,#43031,#43032,#43033,#43034,#43035,#43036,#43037,#43038,#43039,
#43040,#43041,#43042,#43043,#43044,#43045,#43046,#43047,#43048,#43049,#43050,
#43051,#43052,#43053,#43054,#43055,#43056,#43057,#43058,#43059,#43060,#43061,
#43062,#43063,#43064,#43065,#43066,#43067,#43068,#43069,#43070,#43071,#43072,
#43073,#43074,#43075,#43076,#43077,#43078,#43079,#43080,#43081),
 .UNSPECIFIED.,.F.,.F.,(4,3,3,3,3,3,3,3,3,3,3,3,3,3,3,3,3,3,3,4),(0.,0.105620942331472,
0.147712756907025,0.250000000000027,0.345332762315205,0.368665277226416,
0.375000000000042,0.437500000000047,0.468750000000048,0.484375000000051,
0.49473518058623,0.500000000000054,0.589017367505976,0.600284370952884,
0.686110190968832,0.750000000000027,0.831760796016761,0.908457339360646,
0.980208828865569,1.),.UNSPECIFIED.);
#747=B_SPLINE_CURVE_WITH_KNOTS('',3,(#43123,#43124,#43125,#43126,#43127,
#43128,#43129,#43130,#43131,#43132,#43133,#43134,#43135,#43136,#43137,#43138,
#43139,#43140,#43141,#43142,#43143,#43144),.UNSPECIFIED.,.F.,.F.,(4,3,3,
3,3,3,3,4),(0.,0.1428571428571,0.2857142857143,0.4285714285714,0.5714285714286,
0.7142857142857,0.8571428571429,0.99999989893428),.UNSPECIFIED.);
#748=B_SPLINE_CURVE_WITH_KNOTS('',3,(#43147,#43148,#43149,#43150,#43151,
#43152,#43153,#43154,#43155,#43156),.UNSPECIFIED.,.F.,.F.,(4,2,2,2,4),(0.,
0.25,0.5,0.75,0.999999977827856),.UNSPECIFIED.);
#749=B_SPLINE_CURVE_WITH_KNOTS('',3,(#43186,#43187,#43188,#43189,#43190,
#43191,#43192,#43193,#43194,#43195,#43196,#43197,#43198),.UNSPECIFIED.,
 .F.,.F.,(4,3,3,3,4),(0.,0.0431918505797328,0.5,0.956806409420606,1.),
 .UNSPECIFIED.);
#750=B_SPLINE_CURVE_WITH_KNOTS('',3,(#43219,#43220,#43221,#43222,#43223,
#43224,#43225,#43226,#43227,#43228,#43229,#43230,#43231,#43232,#43233,#43234,
#43235,#43236,#43237,#43238,#43239,#43240,#43241,#43242,#43243,#43244,#43245,
#43246,#43247,#43248,#43249,#43250,#43251,#43252,#43253,#43254,#43255,#43256,
#43257,#43258,#43259,#43260,#43261,#43262,#43263,#43264,#43265,#43266,#43267,
#43268,#43269,#43270,#43271,#43272,#43273,#43274,#43275,#43276,#43277,#43278,
#43279,#43280,#43281,#43282,#43283,#43284,#43285,#43286,#43287,#43288,#43289,
#43290,#43291,#43292,#43293,#43294,#43295,#43296,#43297,#43298,#43299,#43300,
#43301,#43302,#43303,#43304,#43305,#43306,#43307,#43308,#43309,#43310,#43311,
#43312,#43313,#43314,#43315,#43316,#43317,#43318,#43319,#43320,#43321,#43322,
#43323,#43324,#43325,#43326,#43327,#43328,#43329,#43330,#43331,#43332,#43333,
#43334,#43335,#43336,#43337,#43338,#43339,#43340,#43341,#43342,#43343,#43344,
#43345,#43346,#43347,#43348,#43349,#43350,#43351,#43352,#43353,#43354,#43355,
#43356,#43357,#43358,#43359,#43360,#43361,#43362,#43363,#43364,#43365,#43366,
#43367,#43368,#43369,#43370,#43371,#43372,#43373,#43374,#43375,#43376,#43377,
#43378,#43379,#43380,#43381,#43382,#43383,#43384,#43385,#43386,#43387,#43388,
#43389,#43390,#43391,#43392,#43393,#43394,#43395,#43396,#43397,#43398,#43399,
#43400,#43401,#43402,#43403,#43404,#43405,#43406,#43407,#43408,#43409,#43410,
#43411,#43412,#43413,#43414,#43415,#43416,#43417,#43418,#43419,#43420,#43421,
#43422,#43423),.UNSPECIFIED.,.F.,.F.,(4,3,3,3,3,3,3,3,3,3,3,3,3,3,3,3,3,
3,3,3,3,3,3,3,3,3,3,3,3,3,3,3,3,3,3,3,3,3,3,3,3,3,3,3,3,3,3,3,3,3,3,3,3,
3,3,3,3,3,3,3,3,3,3,3,3,3,3,3,4),(0.,0.02498566546768,0.049884025399438,
0.0680623311189957,0.0924414494617866,0.107887461956563,0.131551576955674,
0.140980478002927,0.163943871857324,0.171020780322756,0.193322633875285,
0.199590323256334,0.218750000000002,0.227568744214109,0.234375000000002,
0.242187500000002,0.246093750000002,0.248046875000002,0.249023437500002,
0.250000000000002,0.254546871473152,0.279971649656408,0.307406578415395,
0.309430130689131,0.337127106350482,0.344163692255729,0.37200152680762,
0.384912473573474,0.412566459342994,0.429839311238586,0.457842489942603,
0.46874999999999,0.477238857091961,0.484374999999989,0.492187499999988,
0.496093749999988,0.498046874999988,0.499999999999988,0.531289746912242,
0.56564199746469,0.578505777121612,0.613121656810267,0.616394754523827,
0.648093063112125,0.674914456580065,0.697975732163873,0.718059303584619,
0.718749999999981,0.73437499999998,0.735681902185849,0.74218749999998,0.74609374999998,
0.748046874999979,0.749023437499979,0.749999999999979,0.751844076693351,
0.773859225168292,0.79513825511006,0.815771716334843,0.835876984948117,
0.855607588286063,0.87499999999999,0.875168000986653,0.894779928887882,
0.914590308239194,0.934773415781677,0.955588220120383,0.977473296500908,
0.999999988534214),.UNSPECIFIED.);
#751=B_SPLINE_CURVE_WITH_KNOTS('',3,(#43586,#43587,#43588,#43589,#43590,
#43591,#43592,#43593,#43594,#43595,#43596,#43597,#43598,#43599,#43600,#43601,
#43602,#43603,#43604,#43605,#43606,#43607,#43608,#43609,#43610,#43611,#43612,
#43613,#43614,#43615,#43616,#43617,#43618,#43619,#43620,#43621,#43622,#43623,
#43624,#43625,#43626,#43627,#43628,#43629,#43630,#43631,#43632,#43633,#43634,
#43635,#43636,#43637,#43638,#43639,#43640,#43641,#43642,#43643,#43644,#43645,
#43646,#43647,#43648,#43649,#43650,#43651,#43652,#43653,#43654,#43655,#43656,
#43657,#43658,#43659,#43660,#43661,#43662,#43663,#43664,#43665,#43666,#43667,
#43668,#43669,#43670,#43671,#43672,#43673,#43674,#43675,#43676,#43677,#43678,
#43679,#43680,#43681,#43682,#43683,#43684,#43685,#43686,#43687,#43688,#43689,
#43690,#43691,#43692,#43693,#43694,#43695,#43696,#43697,#43698,#43699,#43700,
#43701,#43702,#43703,#43704,#43705,#43706),.UNSPECIFIED.,.F.,.F.,(4,3,3,
3,3,3,3,3,3,3,3,3,3,3,3,3,3,3,3,3,3,3,3,3,3,3,3,3,3,3,3,3,3,3,3,3,3,3,3,
3,4),(7.98332310068083E-8,0.0312500598749252,0.0618422367860364,0.0934211183930221,
0.125000000000008,0.155569261434962,0.187159630717487,0.218750000000013,
0.234375000000014,0.242187500000015,0.246093750000015,0.248046875000015,
0.249023437500015,0.250000000000015,0.450324982651065,0.49998131820124,
0.500000000000021,0.625000000000023,0.687500000000025,0.718750000000025,
0.734375000000026,0.742187500000026,0.749511718750026,0.750000000000026,
0.765919055600215,0.781838289527891,0.797757711899691,0.813677446196644,
0.829597360333286,0.845517577762525,0.859375000000007,0.867187500000006,
0.871093750000005,0.873046875000005,0.874023437500005,0.875000000000005,
0.899836811730506,0.924877595078578,0.949727823226582,0.974863884174689,
0.999999945122795),.UNSPECIFIED.);
#752=B_SPLINE_CURVE_WITH_KNOTS('',3,(#43747,#43748,#43749,#43750,#43751,
#43752,#43753,#43754,#43755,#43756,#43757,#43758,#43759,#43760,#43761,#43762,
#43763,#43764,#43765,#43766,#43767,#43768,#43769,#43770,#43771,#43772,#43773,
#43774,#43775,#43776,#43777,#43778,#43779,#43780,#43781,#43782,#43783,#43784,
#43785,#43786,#43787,#43788,#43789,#43790,#43791,#43792,#43793,#43794,#43795),
 .UNSPECIFIED.,.F.,.F.,(4,3,3,3,3,3,3,3,3,3,3,3,3,3,3,3,4),(0.,0.077129221718004,
0.118225031062465,0.199429752236532,0.249999999999997,0.333192781133113,
0.359721388485999,0.374999999999996,0.423000321495183,0.471434965050803,
0.499999999999995,0.602025518392161,0.703466763159088,0.719210551366323,
0.820753809715136,0.923562015178621,1.),.UNSPECIFIED.);
#753=B_SPLINE_CURVE_WITH_KNOTS('',3,(#43797,#43798,#43799,#43800,#43801,
#43802,#43803),.UNSPECIFIED.,.F.,.F.,(4,3,4),(0.,0.5,1.),.UNSPECIFIED.);
#754=B_SPLINE_CURVE_WITH_KNOTS('',3,(#43806,#43807,#43808,#43809,#43810,
#43811,#43812,#43813,#43814,#43815,#43816,#43817,#43818,#43819,#43820,#43821,
#43822,#43823,#43824,#43825,#43826,#43827,#43828,#43829,#43830,#43831,#43832,
#43833,#43834,#43835,#43836,#43837,#43838,#43839,#43840,#43841,#43842,#43843,
#43844,#43845,#43846,#43847,#43848,#43849,#43850,#43851,#43852,#43853,#43854,
#43855,#43856,#43857,#43858,#43859,#43860,#43861,#43862,#43863,#43864,#43865,
#43866),.UNSPECIFIED.,.F.,.F.,(4,3,3,3,3,3,3,3,3,3,3,3,3,3,3,3,3,3,3,3,
4),(0.,0.0723227135726931,0.149373482450991,0.166421265554989,0.245216450281879,
0.24999999999999,0.335716326463502,0.374999999999983,0.397180535434601,
0.437499999999978,0.468749999999973,0.484374999999972,0.495375835992438,
0.499999999999971,0.593362825587567,0.628795107419847,0.723805225870199,
0.824915532107725,0.849552878717866,0.955120156071517,1.),.UNSPECIFIED.);
#755=B_SPLINE_CURVE_WITH_KNOTS('',3,(#43907,#43908,#43909,#43910,#43911,
#43912,#43913,#43914,#43915,#43916,#43917,#43918,#43919,#43920,#43921,#43922,
#43923,#43924,#43925,#43926,#43927,#43928,#43929,#43930,#43931,#43932,#43933,
#43934,#43935,#43936,#43937,#43938,#43939,#43940,#43941,#43942,#43943,#43944,
#43945,#43946,#43947,#43948,#43949),.UNSPECIFIED.,.F.,.F.,(4,3,3,3,3,3,
3,3,3,3,3,3,3,3,4),(2.99160140262836E-11,0.0832138083944097,0.218577885005784,
0.246109287452998,0.25,0.383459487824275,0.408370299553468,0.541180659138591,
0.570056216035696,0.702294213347345,0.731364949289518,0.75,0.881938327221045,
0.892442289727949,0.999999987394256),.UNSPECIFIED.);
#756=B_SPLINE_CURVE_WITH_KNOTS('',3,(#43950,#43951,#43952,#43953,#43954,
#43955,#43956,#43957,#43958,#43959,#43960,#43961,#43962,#43963,#43964,#43965,
#43966,#43967,#43968,#43969,#43970,#43971,#43972,#43973,#43974,#43975,#43976,
#43977,#43978,#43979,#43980,#43981,#43982,#43983,#43984,#43985,#43986,#43987,
#43988,#43989,#43990,#43991,#43992,#43993,#43994,#43995,#43996,#43997,#43998,
#43999,#44000,#44001,#44002,#44003,#44004,#44005,#44006,#44007,#44008,#44009,
#44010,#44011,#44012,#44013,#44014,#44015,#44016,#44017,#44018,#44019,#44020,
#44021,#44022,#44023,#44024,#44025,#44026,#44027,#44028),.UNSPECIFIED.,
 .F.,.F.,(4,3,3,3,3,3,3,3,3,3,3,3,3,3,3,3,3,3,3,3,3,3,3,3,3,3,4),(0.,0.0457810663232214,
0.0917889142262468,0.120317290917319,0.1428571428571,0.198222944211764,
0.253550325370331,0.275526256355539,0.2857142857143,0.349641048789147,0.413645189435696,
0.4285714285714,0.430597609456793,0.49617632407596,0.561795552657668,0.5714285714286,
0.585374526668123,0.649830120476911,0.7142857142857,0.7403962732342,0.795252877501319,
0.850177989897438,0.8571428571429,0.895765393025997,0.941863426709497,0.987754574459855,
0.999999797061878),.UNSPECIFIED.);
#757=B_SPLINE_CURVE_WITH_KNOTS('',3,(#44064,#44065,#44066,#44067,#44068,
#44069,#44070,#44071,#44072,#44073,#44074,#44075,#44076,#44077,#44078,#44079,
#44080,#44081,#44082,#44083,#44084,#44085,#44086,#44087,#44088,#44089,#44090,
#44091,#44092,#44093,#44094,#44095,#44096,#44097,#44098,#44099,#44100,#44101,
#44102,#44103,#44104,#44105,#44106,#44107,#44108,#44109,#44110,#44111,#44112,
#44113,#44114,#44115,#44116,#44117,#44118,#44119,#44120,#44121,#44122,#44123,
#44124),.UNSPECIFIED.,.F.,.F.,(4,3,3,3,3,3,3,3,3,3,3,3,3,3,3,3,3,3,3,3,
4),(5.51331975023469E-11,0.100729568242541,0.175364784121271,0.238681770721503,
0.25,0.301425913559992,0.351100073817221,0.399989929903429,0.449994964951714,
0.497440910286256,0.5,0.500001662220487,0.54753591343043,0.598151935072823,
0.647542568098908,0.698771284049454,0.75,0.812858492196759,0.888031547366612,
0.98742976017277,0.99999999994457),.UNSPECIFIED.);
#758=B_SPLINE_CURVE_WITH_KNOTS('',3,(#44165,#44166,#44167,#44168,#44169,
#44170,#44171,#44172,#44173,#44174,#44175,#44176,#44177,#44178,#44179,#44180,
#44181,#44182,#44183,#44184,#44185,#44186,#44187,#44188,#44189,#44190,#44191,
#44192,#44193,#44194,#44195,#44196,#44197,#44198,#44199,#44200,#44201,#44202,
#44203,#44204,#44205,#44206,#44207,#44208,#44209,#44210,#44211,#44212,#44213,
#44214,#44215,#44216,#44217,#44218,#44219,#44220,#44221,#44222,#44223,#44224,
#44225,#44226,#44227,#44228,#44229,#44230,#44231,#44232,#44233,#44234,#44235,
#44236,#44237,#44238,#44239,#44240,#44241,#44242,#44243,#44244,#44245,#44246,
#44247,#44248,#44249,#44250,#44251,#44252,#44253,#44254,#44255,#44256,#44257,
#44258),.UNSPECIFIED.,.F.,.F.,(4,3,3,3,3,3,3,3,3,3,3,3,3,3,3,3,3,3,3,3,
3,3,3,3,3,3,3,3,3,3,3,4),(0.,0.0608427785031114,0.121685557006223,0.125000000000001,
0.182031019624917,0.187500000000002,0.218750000000002,0.234375000000003,
0.242187500000002,0.247942132015918,0.250000000000002,0.273617827471563,
0.341050580590077,0.407249199298602,0.425682324109709,0.492217475541122,
0.500000000000002,0.565400091710283,0.574576838490885,0.625000000000001,
0.687500000000001,0.718750000000001,0.726647659500348,0.734375000000001,
0.742187500000001,0.747984593859013,0.750000000000001,0.805925774071174,
0.863236880411379,0.878574885619189,0.939287442809595,1.),.UNSPECIFIED.);
#759=B_SPLINE_CURVE_WITH_KNOTS('',3,(#44299,#44300,#44301,#44302,#44303,
#44304,#44305),.UNSPECIFIED.,.F.,.F.,(4,3,4),(0.,0.5,0.999999999992773),
 .UNSPECIFIED.);
#760=B_SPLINE_CURVE_WITH_KNOTS('',3,(#44307,#44308,#44309,#44310,#44311,
#44312,#44313,#44314,#44315,#44316,#44317,#44318,#44319,#44320,#44321,#44322,
#44323,#44324,#44325,#44326,#44327,#44328,#44329,#44330,#44331,#44332,#44333,
#44334,#44335,#44336,#44337,#44338,#44339,#44340,#44341,#44342,#44343,#44344,
#44345,#44346,#44347,#44348,#44349),.UNSPECIFIED.,.F.,.F.,(4,3,3,3,3,3,
3,3,3,3,3,3,3,3,4),(0.,0.0899680658841344,0.116138968898349,0.242390930404426,
0.25000000000001,0.363401837080852,0.437500000000014,0.466169905219584,
0.495204599768524,0.500000000000013,0.615774222962765,0.721520585496806,
0.830869548090939,0.936889486863146,1.),.UNSPECIFIED.);
#761=B_SPLINE_CURVE_WITH_KNOTS('',3,(#44350,#44351,#44352,#44353,#44354,
#44355,#44356,#44357,#44358,#44359,#44360,#44361,#44362,#44363,#44364,#44365,
#44366,#44367,#44368,#44369,#44370,#44371,#44372,#44373,#44374,#44375,#44376,
#44377,#44378,#44379,#44380,#44381,#44382,#44383,#44384,#44385,#44386,#44387,
#44388,#44389,#44390,#44391,#44392,#44393,#44394,#44395,#44396,#44397,#44398,
#44399,#44400,#44401,#44402,#44403,#44404,#44405,#44406,#44407),
 .UNSPECIFIED.,.F.,.F.,(4,3,3,3,3,3,3,3,3,3,3,3,3,3,3,3,3,3,3,4),(0.,0.104831354904759,
0.146359487096874,0.25000000000003,0.344476853378971,0.368351209780046,
0.375000000000043,0.43750000000005,0.468750000000052,0.484375000000053,
0.49465917516026,0.500000000000053,0.58999972691812,0.600572762837569,0.688690709817914,
0.769751602688375,0.832826399321062,0.910573005906539,0.983365812451633,
1.),.UNSPECIFIED.);
#762=B_SPLINE_CURVE_WITH_KNOTS('',3,(#44453,#44454,#44455,#44456,#44457,
#44458,#44459,#44460,#44461,#44462,#44463,#44464,#44465,#44466,#44467,#44468,
#44469,#44470,#44471,#44472,#44473,#44474,#44475,#44476,#44477,#44478,#44479,
#44480,#44481,#44482,#44483,#44484,#44485,#44486,#44487,#44488,#44489,#44490,
#44491,#44492,#44493,#44494,#44495,#44496,#44497,#44498,#44499,#44500,#44501,
#44502,#44503,#44504,#44505,#44506,#44507,#44508,#44509,#44510,#44511,#44512,
#44513,#44514,#44515,#44516,#44517,#44518,#44519,#44520,#44521,#44522,#44523,
#44524,#44525),.UNSPECIFIED.,.F.,.F.,(4,3,3,3,3,3,3,3,3,3,3,3,3,3,3,3,3,
3,3,3,3,3,3,3,4),(0.,0.0458328812420613,0.0918178429902138,0.137727842668992,
0.1428571428571,0.148537109984561,0.203805441054238,0.259125141492703,0.2857142857143,
0.296138265592348,0.362354847081874,0.4285714285714,0.443718112661787,0.511007039375829,
0.5714285714286,0.591515929737013,0.658633627441551,0.7142857142857,0.739436118157717,
0.798289487650309,0.8571428571429,0.887212493478405,0.933523714257452,0.979590210065679,
1.),.UNSPECIFIED.);
#763=B_SPLINE_CURVE_WITH_KNOTS('',3,(#44528,#44529,#44530,#44531,#44532,
#44533,#44534,#44535,#44536,#44537,#44538,#44539,#44540,#44541,#44542,#44543,
#44544,#44545,#44546,#44547,#44548,#44549,#44550,#44551,#44552,#44553,#44554,
#44555,#44556,#44557,#44558,#44559,#44560,#44561,#44562,#44563,#44564,#44565,
#44566,#44567),.UNSPECIFIED.,.F.,.F.,(4,3,3,3,3,3,3,3,3,3,3,3,3,4),(0.,
0.132990593304601,0.153370100778055,0.288985327651276,0.306720031714283,
0.443623442712682,0.460362108909032,0.597256308685064,0.614810898821594,
0.75,0.769627028952669,0.909362273050122,0.924609010238514,0.999999999982405),
 .UNSPECIFIED.);
#764=B_SPLINE_CURVE_WITH_KNOTS('',3,(#44590,#44591,#44592,#44593,#44594,
#44595,#44596,#44597,#44598,#44599),.UNSPECIFIED.,.F.,.F.,(4,3,3,4),(0.,
0.3333333333333,0.6666666666667,1.),.UNSPECIFIED.);
#765=B_SPLINE_CURVE_WITH_KNOTS('',3,(#44735,#44736,#44737,#44738,#44739,
#44740,#44741,#44742,#44743,#44744,#44745,#44746,#44747,#44748,#44749,#44750,
#44751,#44752,#44753,#44754,#44755,#44756,#44757,#44758,#44759,#44760,#44761,
#44762,#44763,#44764,#44765,#44766,#44767,#44768,#44769,#44770,#44771,#44772,
#44773,#44774,#44775,#44776,#44777,#44778,#44779,#44780,#44781,#44782,#44783,
#44784,#44785,#44786,#44787,#44788,#44789,#44790,#44791,#44792,#44793,#44794,
#44795,#44796,#44797,#44798,#44799,#44800,#44801,#44802,#44803,#44804,#44805,
#44806,#44807,#44808,#44809,#44810,#44811,#44812,#44813,#44814,#44815,#44816,
#44817,#44818,#44819,#44820,#44821,#44822,#44823),.UNSPECIFIED.,.F.,.F.,
(4,2,2,1,2,2,2,2,1,1,2,2,2,2,1,1,1,2,2,2,2,2,2,2,2,2,1,2,2,2,1,1,2,2,2,
2,1,1,2,2,2,2,1,1,2,2,2,1,1,2,2,4),(0.,0.0312499999999994,0.046874999999999,
0.0546874999999987,0.0585937499999986,0.0624999999999985,0.0937499999999971,
0.109374999999996,0.117187499999996,0.121093749999996,0.123046874999996,
0.124999999999996,0.187499999999999,0.21875,0.234375000000001,0.242187500000001,
0.246093750000002,0.248046875000002,0.250000000000002,0.312500000000002,
0.343750000000003,0.359375000000003,0.375000000000003,0.437500000000004,
0.468750000000004,0.484375000000004,0.492187500000004,0.496093750000004,
0.500000000000004,0.562500000000005,0.593750000000005,0.609375000000005,
0.617187500000005,0.625000000000005,0.687500000000005,0.718750000000005,
0.734375000000005,0.742187500000005,0.746093750000005,0.750000000000005,
0.812500000000005,0.843750000000006,0.859375000000005,0.867187500000005,
0.871093750000005,0.875000000000005,0.906250000000004,0.921875000000003,
0.929687500000003,0.933593750000003,0.937500000000003,1.),.UNSPECIFIED.);
#766=B_SPLINE_CURVE_WITH_KNOTS('',3,(#44826,#44827,#44828,#44829,#44830,
#44831,#44832,#44833,#44834,#44835,#44836,#44837,#44838,#44839,#44840,#44841,
#44842,#44843,#44844,#44845,#44846,#44847,#44848,#44849,#44850,#44851,#44852,
#44853,#44854,#44855,#44856,#44857,#44858,#44859,#44860,#44861,#44862,#44863,
#44864,#44865,#44866,#44867,#44868,#44869,#44870,#44871,#44872,#44873,#44874,
#44875,#44876,#44877,#44878,#44879,#44880,#44881,#44882,#44883,#44884,#44885,
#44886,#44887,#44888,#44889,#44890,#44891,#44892,#44893,#44894,#44895,#44896,
#44897,#44898,#44899,#44900,#44901,#44902,#44903,#44904,#44905,#44906,#44907,
#44908,#44909,#44910,#44911,#44912,#44913,#44914,#44915,#44916,#44917,#44918,
#44919,#44920,#44921,#44922,#44923,#44924,#44925,#44926,#44927,#44928,#44929,
#44930,#44931,#44932,#44933,#44934,#44935,#44936,#44937,#44938,#44939,#44940,
#44941,#44942,#44943,#44944,#44945,#44946,#44947,#44948,#44949,#44950,#44951,
#44952,#44953,#44954,#44955,#44956,#44957,#44958,#44959,#44960,#44961,#44962,
#44963,#44964,#44965,#44966,#44967,#44968,#44969,#44970,#44971,#44972,#44973,
#44974,#44975,#44976,#44977,#44978,#44979,#44980,#44981,#44982,#44983,#44984,
#44985,#44986,#44987,#44988,#44989,#44990,#44991,#44992,#44993,#44994,#44995,
#44996,#44997,#44998,#44999,#45000,#45001,#45002,#45003,#45004,#45005,#45006,
#45007,#45008,#45009,#45010,#45011,#45012),.UNSPECIFIED.,.F.,.F.,(4,3,3,
3,3,3,3,3,3,3,3,3,3,3,3,3,3,3,3,3,3,3,3,3,3,3,3,3,3,3,3,3,3,3,3,3,3,3,3,
3,3,3,3,3,3,3,3,3,3,3,3,3,3,3,3,3,3,3,3,3,3,3,4),(7.50077744408458E-8,2.18347065731793E-7,
0.0229486992448132,0.0291148599209922,0.0509746147885199,0.0551851751703622,
0.0624999999999753,0.0795336645402833,0.100117921833713,0.102945846679325,
0.109374999999957,0.117187499999954,0.121093749999952,0.123046874999952,
0.124511718749951,0.124999999999951,0.126823713026409,0.154172407482107,
0.168540259620717,0.195094492624172,0.207813484550183,0.234374999999958,
0.243585913496471,0.245602831811104,0.249999999999959,0.286463024092484,
0.32317957057371,0.335377808175913,0.372218838783674,0.396057562301687,
0.433018807503827,0.468749999999972,0.471312798122102,0.484374999999973,
0.492187499999974,0.499324281709741,0.499999999999974,0.539362839729169,
0.553194039019897,0.592475975164342,0.619367182653107,0.65850176352843,
0.673126719387982,0.711992777523277,0.716725121178675,0.718749999999988,
0.734374999999989,0.742187499999989,0.746093749999989,0.749489102970321,
0.74999999999999,0.753695598868588,0.789783387615562,0.822481343689209,
0.851891345405311,0.878121041904186,0.90149239976546,0.922411241342462,
0.941273136669776,0.958424669511218,0.974021299622255,0.988170798160314,
1.),.UNSPECIFIED.);
#767=B_SPLINE_CURVE_WITH_KNOTS('',3,(#45049,#45050,#45051,#45052,#45053,
#45054,#45055,#45056,#45057,#45058),.UNSPECIFIED.,.F.,.F.,(4,2,2,2,4),(2.21660018633822E-8,
0.25,0.5,0.75,1.),.UNSPECIFIED.);
#768=B_SPLINE_CURVE_WITH_KNOTS('',3,(#45059,#45060,#45061,#45062,#45063,
#45064,#45065,#45066,#45067,#45068,#45069,#45070,#45071,#45072,#45073,#45074,
#45075,#45076,#45077,#45078,#45079,#45080,#45081,#45082,#45083,#45084,#45085,
#45086,#45087,#45088,#45089,#45090,#45091,#45092,#45093,#45094,#45095,#45096,
#45097,#45098,#45099,#45100,#45101,#45102,#45103,#45104,#45105,#45106,#45107,
#45108,#45109,#45110,#45111,#45112,#45113,#45114,#45115,#45116,#45117,#45118,
#45119),.UNSPECIFIED.,.F.,.F.,(4,3,3,3,3,3,3,3,3,3,3,3,3,3,3,3,3,3,3,3,
4),(3.71092975531932E-11,0.10075796569964,0.17537898284982,0.238719107558443,
0.25,0.301412310165757,0.351074976513478,0.399954340676608,0.449977170338304,
0.497414131176893,0.5,0.50000257236142,0.547527734549922,0.598145800912442,
0.647524947458811,0.698762473729406,0.75,0.812880663949358,0.888102663575457,
0.987477736473804,0.99999999995342),.UNSPECIFIED.);
#769=B_SPLINE_CURVE_WITH_KNOTS('',3,(#45162,#45163,#45164,#45165,#45166,
#45167,#45168,#45169,#45170,#45171,#45172,#45173,#45174,#45175,#45176,#45177,
#45178,#45179,#45180,#45181,#45182,#45183,#45184,#45185,#45186,#45187,#45188,
#45189,#45190,#45191,#45192,#45193,#45194,#45195,#45196,#45197,#45198,#45199,
#45200,#45201,#45202,#45203,#45204,#45205,#45206,#45207,#45208,#45209,#45210,
#45211,#45212,#45213,#45214,#45215,#45216,#45217,#45218,#45219,#45220,#45221,
#45222,#45223,#45224,#45225,#45226,#45227,#45228,#45229,#45230,#45231,#45232,
#45233,#45234,#45235,#45236,#45237,#45238,#45239,#45240,#45241,#45242,#45243,
#45244,#45245,#45246,#45247,#45248,#45249),.UNSPECIFIED.,.F.,.F.,(4,3,3,
3,3,3,3,3,3,3,3,3,3,3,3,3,3,3,3,3,3,3,3,3,3,3,3,3,3,4),(0.,0.0590919852588188,
0.11700786268473,0.124999999999999,0.131471991461492,0.187499999999999,
0.218749999999999,0.234374999999998,0.243548805830801,0.249999999999998,
0.280266149608354,0.347497113067735,0.413420413834471,0.427679421923862,
0.494017799351283,0.499999999999998,0.564689257159006,0.571457994333151,
0.624999999999998,0.687499999999998,0.718749999999998,0.718850415436541,
0.734374999999998,0.743575440506396,0.749999999999998,0.808807839857273,
0.867615679714548,0.926690041742276,0.987210740295307,1.),.UNSPECIFIED.);
#770=B_SPLINE_CURVE_WITH_KNOTS('',3,(#45288,#45289,#45290,#45291,#45292,
#45293,#45294,#45295,#45296,#45297,#45298,#45299,#45300,#45301,#45302,#45303,
#45304,#45305,#45306,#45307,#45308,#45309,#45310,#45311,#45312,#45313,#45314,
#45315,#45316,#45317,#45318,#45319,#45320,#45321,#45322,#45323,#45324,#45325,
#45326,#45327,#45328,#45329,#45330,#45331,#45332,#45333,#45334,#45335,#45336),
 .UNSPECIFIED.,.F.,.F.,(4,3,3,3,3,3,3,3,3,3,3,3,3,3,3,3,4),(0.,0.0770534094112941,
0.113178684151245,0.194390251507181,0.250000000000004,0.333175386735155,
0.356184877277791,0.375000000000004,0.422808196248102,0.471047643121825,
0.500000000000004,0.602035527258785,0.703481183539205,0.716723706355646,
0.818257118256476,0.921054244078466,1.),.UNSPECIFIED.);
#771=B_SPLINE_CURVE_WITH_KNOTS('',3,(#45337,#45338,#45339,#45340,#45341,
#45342,#45343),.UNSPECIFIED.,.F.,.F.,(4,3,4),(0.,0.5,1.),.UNSPECIFIED.);
#772=B_SPLINE_CURVE_WITH_KNOTS('',3,(#45344,#45345,#45346,#45347,#45348,
#45349,#45350,#45351,#45352,#45353,#45354,#45355,#45356,#45357,#45358,#45359,
#45360,#45361,#45362,#45363,#45364,#45365,#45366,#45367,#45368,#45369,#45370,
#45371,#45372,#45373,#45374,#45375,#45376,#45377,#45378,#45379,#45380,#45381,
#45382,#45383,#45384,#45385,#45386,#45387,#45388,#45389,#45390,#45391,#45392,
#45393,#45394,#45395,#45396,#45397,#45398,#45399,#45400,#45401),
 .UNSPECIFIED.,.F.,.F.,(4,3,3,3,3,3,3,3,3,3,3,3,3,3,3,3,3,3,3,4),(0.,0.0719184804286781,
0.148618114776114,0.169128486210845,0.249999999999983,0.335388721840469,
0.374999999999972,0.402161385818952,0.437499999999966,0.468749999999962,
0.484374999999962,0.495231216441581,0.499999999999961,0.592539932569911,
0.634235212438464,0.728584906446939,0.829025201759185,0.856412790238199,
0.961308327777253,1.),.UNSPECIFIED.);
#773=B_SPLINE_CURVE_WITH_KNOTS('',3,(#45444,#45445,#45446,#45447,#45448,
#45449,#45450,#45451,#45452,#45453,#45454,#45455,#45456,#45457,#45458,#45459,
#45460,#45461,#45462,#45463,#45464,#45465),.UNSPECIFIED.,.F.,.F.,(4,3,3,
3,3,3,3,4),(1.01036188073728E-7,0.1428571428571,0.2857142857143,0.4285714285714,
0.5714285714286,0.7142857142857,0.8571428571429,1.),.UNSPECIFIED.);
#774=B_SPLINE_CURVE_WITH_KNOTS('',3,(#45504,#45505,#45506,#45507,#45508,
#45509,#45510,#45511,#45512,#45513,#45514,#45515,#45516,#45517,#45518,#45519),
 .UNSPECIFIED.,.F.,.F.,(4,3,3,3,3,4),(0.,0.269796418766363,0.446837155942232,
0.5,0.767870847367721,0.999999999967383),.UNSPECIFIED.);
#775=B_SPLINE_CURVE_WITH_KNOTS('',3,(#45521,#45522,#45523,#45524,#45525,
#45526,#45527,#45528,#45529,#45530,#45531,#45532,#45533,#45534,#45535,#45536,
#45537,#45538,#45539,#45540,#45541,#45542,#45543,#45544,#45545,#45546,#45547,
#45548,#45549,#45550,#45551,#45552,#45553,#45554,#45555,#45556,#45557,#45558,
#45559,#45560,#45561,#45562,#45563),.UNSPECIFIED.,.F.,.F.,(4,3,3,3,3,3,
3,3,3,3,3,3,3,3,4),(0.,0.0918948483207178,0.132863053438045,0.249999999999997,
0.389695921194281,0.437499999999998,0.466122318206124,0.495108641874883,
0.499999999999999,0.616165726887126,0.729387146575313,0.772201865170694,
0.880137531088479,0.985278722839219,1.),.UNSPECIFIED.);
#776=B_SPLINE_CURVE_WITH_KNOTS('',3,(#45564,#45565,#45566,#45567,#45568,
#45569,#45570,#45571,#45572,#45573,#45574,#45575,#45576,#45577,#45578,#45579,
#45580,#45581,#45582,#45583,#45584,#45585,#45586,#45587,#45588,#45589,#45590,
#45591,#45592,#45593,#45594,#45595,#45596,#45597,#45598,#45599,#45600,#45601,
#45602,#45603,#45604,#45605,#45606,#45607,#45608,#45609,#45610,#45611,#45612,
#45613,#45614,#45615),.UNSPECIFIED.,.F.,.F.,(4,3,3,3,3,3,3,3,3,3,3,3,3,
3,3,3,3,4),(0.,0.105512176586077,0.166506332434029,0.249999999999994,0.346021730220121,
0.37499999999999,0.391545484010592,0.437499999999987,0.468749999999988,
0.484391044121635,0.499999999999989,0.595751032836016,0.626515006508435,
0.720124709531476,0.807105535962062,0.857083639881126,0.93982049409868,
1.),.UNSPECIFIED.);
#777=B_SPLINE_CURVE_WITH_KNOTS('',3,(#45657,#45658,#45659,#45660,#45661,
#45662,#45663,#45664,#45665,#45666,#45667,#45668,#45669,#45670,#45671,#45672,
#45673,#45674,#45675,#45676,#45677,#45678),.UNSPECIFIED.,.F.,.F.,(4,3,3,
3,3,3,3,4),(0.,0.1428571428571,0.2857142857143,0.4285714285714,0.5714285714286,
0.7142857142857,0.8571428571429,0.999999898936753),.UNSPECIFIED.);
#778=B_SPLINE_CURVE_WITH_KNOTS('',3,(#45681,#45682,#45683,#45684,#45685,
#45686,#45687,#45688,#45689,#45690),.UNSPECIFIED.,.F.,.F.,(4,2,2,2,4),(0.,
0.25,0.5,0.75,0.999999977827887),.UNSPECIFIED.);
#779=B_SPLINE_CURVE_WITH_KNOTS('',3,(#45720,#45721,#45722,#45723,#45724,
#45725,#45726,#45727,#45728,#45729,#45730,#45731,#45732),.UNSPECIFIED.,
 .F.,.F.,(4,3,3,3,4),(0.,0.0431918509658033,0.5,0.956806409055318,1.),
 .UNSPECIFIED.);
#780=B_SPLINE_CURVE_WITH_KNOTS('',3,(#45753,#45754,#45755,#45756,#45757,
#45758,#45759,#45760,#45761,#45762,#45763,#45764,#45765,#45766,#45767,#45768,
#45769,#45770,#45771,#45772,#45773,#45774,#45775,#45776,#45777,#45778,#45779,
#45780,#45781,#45782,#45783,#45784,#45785,#45786,#45787,#45788,#45789,#45790,
#45791,#45792,#45793,#45794,#45795,#45796,#45797,#45798,#45799,#45800,#45801,
#45802,#45803,#45804,#45805,#45806,#45807,#45808,#45809,#45810,#45811,#45812,
#45813,#45814,#45815,#45816,#45817,#45818,#45819,#45820,#45821,#45822,#45823,
#45824,#45825,#45826,#45827,#45828,#45829,#45830,#45831,#45832,#45833,#45834,
#45835,#45836,#45837,#45838,#45839,#45840,#45841,#45842,#45843,#45844,#45845,
#45846,#45847,#45848,#45849,#45850,#45851,#45852,#45853,#45854,#45855,#45856,
#45857,#45858,#45859,#45860,#45861,#45862,#45863,#45864,#45865,#45866,#45867,
#45868,#45869,#45870,#45871,#45872,#45873,#45874,#45875,#45876,#45877,#45878,
#45879,#45880,#45881,#45882,#45883,#45884,#45885,#45886,#45887,#45888,#45889,
#45890,#45891,#45892,#45893,#45894,#45895,#45896,#45897,#45898,#45899,#45900,
#45901,#45902,#45903,#45904,#45905,#45906,#45907,#45908,#45909,#45910,#45911,
#45912,#45913,#45914,#45915,#45916,#45917,#45918,#45919,#45920,#45921,#45922,
#45923,#45924,#45925,#45926,#45927,#45928,#45929,#45930,#45931,#45932,#45933,
#45934,#45935,#45936,#45937,#45938,#45939,#45940,#45941,#45942,#45943,#45944,
#45945,#45946,#45947,#45948,#45949,#45950,#45951,#45952,#45953,#45954,#45955,
#45956,#45957),.UNSPECIFIED.,.F.,.F.,(4,3,3,3,3,3,3,3,3,3,3,3,3,3,3,3,3,
3,3,3,3,3,3,3,3,3,3,3,3,3,3,3,3,3,3,3,3,3,3,3,3,3,3,3,3,3,3,3,3,3,3,3,3,
3,3,3,3,3,3,3,3,3,3,3,3,3,3,3,4),(0.,0.0249856653057896,0.0498840250895596,
0.0680623319906546,0.0924414501656426,0.107887462717563,0.131551577536791,
0.140980478615626,0.163943872360021,0.171020780779603,0.193322634140233,
0.19959032355363,0.218750000000014,0.22756874434828,0.234375000000015,0.242187500000016,
0.246093750000016,0.248046875000016,0.249023437500016,0.250000000000016,
0.254546871436753,0.279971649431658,0.307406577861317,0.309430130279663,
0.337127105577854,0.344163691684047,0.372001525912439,0.384912472908073,
0.412566458291854,0.429839310630959,0.457842489000878,0.468750000000014,
0.477238856805736,0.484375000000014,0.492187500000014,0.496093750000014,
0.498046875000014,0.500000000000014,0.531289744877457,0.565641998369439,
0.578505773627244,0.613121656100364,0.616394750861499,0.648093059813583,
0.674914453874227,0.697975730141801,0.718059302271027,0.718750000000014,
0.734375000000014,0.735681901570784,0.742187500000014,0.746093750000014,
0.748046875000014,0.749023437500014,0.750000000000014,0.75184407675242,
0.773859225905082,0.795138256456607,0.815771718220529,0.8358769872991,0.855607591022799,
0.875000000000007,0.875168004019054,0.89477993210703,0.914590311502922,
0.934773418892348,0.955588222783837,0.977473298233141,0.999999988534264),
 .UNSPECIFIED.);
#781=B_SPLINE_CURVE_WITH_KNOTS('',3,(#46120,#46121,#46122,#46123,#46124,
#46125,#46126,#46127,#46128,#46129,#46130,#46131,#46132,#46133,#46134,#46135,
#46136,#46137,#46138,#46139,#46140,#46141,#46142,#46143,#46144,#46145,#46146,
#46147,#46148,#46149,#46150,#46151,#46152,#46153,#46154,#46155,#46156,#46157,
#46158,#46159,#46160,#46161,#46162,#46163,#46164,#46165,#46166,#46167,#46168,
#46169,#46170,#46171,#46172,#46173,#46174,#46175,#46176,#46177,#46178,#46179,
#46180,#46181,#46182,#46183,#46184,#46185,#46186,#46187,#46188,#46189,#46190,
#46191,#46192,#46193,#46194,#46195,#46196,#46197,#46198,#46199,#46200,#46201,
#46202,#46203,#46204,#46205,#46206,#46207,#46208,#46209,#46210,#46211,#46212,
#46213,#46214,#46215,#46216,#46217,#46218,#46219,#46220,#46221,#46222,#46223,
#46224,#46225,#46226,#46227,#46228,#46229,#46230,#46231,#46232,#46233,#46234,
#46235,#46236,#46237,#46238,#46239,#46240),.UNSPECIFIED.,.F.,.F.,(4,3,3,
3,3,3,3,3,3,3,3,3,3,3,3,3,3,3,3,3,3,3,3,3,3,3,3,3,3,3,3,3,3,3,3,3,3,3,3,
3,4),(7.98330076221588E-8,0.031250059874758,0.0618422366267454,0.0934211183133773,
0.125000000000009,0.155569261276705,0.187159630638361,0.218750000000016,
0.234375000000017,0.242187500000018,0.246093750000018,0.248046875000018,
0.249023437500018,0.250000000000018,0.450324981199179,0.499981318201029,
0.500000000000023,0.625000000000025,0.687500000000026,0.718750000000026,
0.734375000000026,0.742187500000027,0.749511718750026,0.750000000000026,
0.765919054620212,0.781838287567876,0.797757708959856,0.81367744227693,
0.829597355433741,0.845517571883335,0.859375000000014,0.867187500000013,
0.871093750000013,0.873046875000013,0.874023437500013,0.875000000000013,
0.899836813687984,0.924877596546642,0.949727826656971,0.974863885889794,
0.999999945122618),.UNSPECIFIED.);
#782=B_SPLINE_CURVE_WITH_KNOTS('',3,(#46277,#46278,#46279,#46280,#46281,
#46282,#46283,#46284,#46285,#46286,#46287,#46288,#46289,#46290,#46291,#46292,
#46293,#46294,#46295,#46296,#46297,#46298,#46299,#46300,#46301,#46302,#46303,
#46304,#46305,#46306,#46307,#46308,#46309,#46310,#46311,#46312,#46313,#46314,
#46315,#46316,#46317,#46318,#46319,#46320,#46321,#46322,#46323,#46324,#46325),
 .UNSPECIFIED.,.F.,.F.,(4,3,3,3,3,3,3,3,3,3,3,3,3,3,3,3,4),(0.,0.077478098023877,
0.135874094516151,0.217128639935507,0.25,0.33343704912886,0.374999999999998,
0.392068058960876,0.440389336306725,0.489414520804398,0.499999999999996,
0.601853270166522,0.703313489677787,0.783418260834186,0.885329497471594,
0.988564571994781,0.999999999998388),.UNSPECIFIED.);
#783=B_SPLINE_CURVE_WITH_KNOTS('',3,(#46327,#46328,#46329,#46330,#46331,
#46332,#46333,#46334,#46335,#46336,#46337,#46338,#46339,#46340,#46341,#46342),
 .UNSPECIFIED.,.F.,.F.,(4,3,3,3,3,4),(0.,0.267749500822812,0.5,0.532448232691873,
0.802237959956232,1.),.UNSPECIFIED.);
#784=B_SPLINE_CURVE_WITH_KNOTS('',3,(#46345,#46346,#46347,#46348,#46349,
#46350,#46351,#46352,#46353,#46354,#46355,#46356,#46357,#46358,#46359,#46360,
#46361,#46362,#46363,#46364,#46365,#46366,#46367,#46368,#46369,#46370,#46371,
#46372,#46373,#46374,#46375,#46376,#46377,#46378,#46379,#46380,#46381,#46382,
#46383,#46384,#46385,#46386,#46387,#46388,#46389,#46390,#46391,#46392,#46393),
 .UNSPECIFIED.,.F.,.F.,(4,3,3,3,3,3,3,3,3,3,3,3,3,3,3,3,4),(0.,0.0744713783998642,
0.150804301319361,0.230306545116836,0.250000000000007,0.336435447589264,
0.375000000000008,0.437500000000008,0.468750000000007,0.485132844005362,
0.500000000000006,0.5872348585764,0.676833467819857,0.770825792057067,0.867637831307337,
0.969202827667639,1.),.UNSPECIFIED.);
#785=B_SPLINE_CURVE_WITH_KNOTS('',3,(#46434,#46435,#46436,#46437,#46438,
#46439,#46440,#46441,#46442,#46443,#46444,#46445,#46446,#46447,#46448,#46449,
#46450,#46451,#46452,#46453,#46454,#46455,#46456,#46457,#46458,#46459,#46460,
#46461,#46462,#46463,#46464,#46465,#46466,#46467,#46468,#46469,#46470,#46471,
#46472,#46473,#46474,#46475,#46476),.UNSPECIFIED.,.F.,.F.,(4,3,3,3,3,3,
3,3,3,3,3,3,3,3,4),(4.64734132034318E-12,0.083213773511874,0.218574767489085,
0.246109194308012,0.25,0.383459560668354,0.408370349991552,0.541180765413226,
0.570056405676159,0.702294512896255,0.731364773860962,0.75,0.881938378821876,
0.892442186051743,0.999999987394215),.UNSPECIFIED.);
#786=B_SPLINE_CURVE_WITH_KNOTS('',3,(#46477,#46478,#46479,#46480,#46481,
#46482,#46483,#46484,#46485,#46486,#46487,#46488,#46489,#46490,#46491,#46492,
#46493,#46494,#46495,#46496,#46497,#46498,#46499,#46500,#46501,#46502,#46503,
#46504,#46505,#46506,#46507,#46508,#46509,#46510,#46511,#46512,#46513,#46514,
#46515,#46516,#46517,#46518,#46519,#46520,#46521,#46522,#46523,#46524,#46525,
#46526,#46527,#46528,#46529,#46530,#46531,#46532,#46533,#46534,#46535,#46536,
#46537,#46538,#46539,#46540,#46541,#46542,#46543,#46544,#46545,#46546,#46547,
#46548,#46549,#46550,#46551,#46552,#46553,#46554,#46555),.UNSPECIFIED.,
 .F.,.F.,(4,3,3,3,3,3,3,3,3,3,3,3,3,3,3,3,3,3,3,3,3,3,3,3,3,3,4),(0.,0.0457027398302697,
0.0916124646568031,0.120396457889583,0.1428571428571,0.197268351864743,
0.251639643768668,0.275598313608457,0.2857142857143,0.349088877065947,0.412548015414617,
0.4285714285714,0.430653820896832,0.496062938448994,0.561513727370746,0.5714285714286,
0.585415481341103,0.649850597813402,0.7142857142857,0.740421636160008,0.795269302788479,
0.850185494204953,0.8571428571429,0.895775578845262,0.941868729299644,0.987754979081763,
0.999999797081979),.UNSPECIFIED.);
#787=B_SPLINE_CURVE_WITH_KNOTS('',3,(#46591,#46592,#46593,#46594,#46595,
#46596,#46597,#46598,#46599,#46600,#46601,#46602,#46603,#46604,#46605,#46606,
#46607,#46608,#46609,#46610,#46611,#46612,#46613,#46614,#46615,#46616,#46617,
#46618,#46619,#46620,#46621,#46622,#46623,#46624,#46625,#46626,#46627,#46628,
#46629,#46630,#46631,#46632,#46633,#46634,#46635,#46636,#46637,#46638,#46639,
#46640,#46641,#46642,#46643,#46644,#46645,#46646,#46647,#46648,#46649,#46650,
#46651),.UNSPECIFIED.,.F.,.F.,(4,3,3,3,3,3,3,3,3,3,3,3,3,3,3,3,3,3,3,3,
4),(8.7034819132607E-11,0.100686132890676,0.175343066445338,0.23862704943103,
0.25,0.301428394363909,0.351104884437592,0.39999698373092,0.44999849186546,
0.497446586143753,0.5,0.500001665638562,0.547538082380572,0.598153561785429,
0.647546551590073,0.698773275795036,0.75,0.812823294069069,0.887911054136799,
0.987361330124032,0.999999999998726),.UNSPECIFIED.);
#788=B_SPLINE_CURVE_WITH_KNOTS('',3,(#46692,#46693,#46694,#46695,#46696,
#46697,#46698,#46699,#46700,#46701,#46702,#46703,#46704,#46705,#46706,#46707,
#46708,#46709,#46710,#46711,#46712,#46713,#46714,#46715,#46716,#46717,#46718,
#46719,#46720,#46721,#46722,#46723,#46724,#46725,#46726,#46727,#46728,#46729,
#46730,#46731,#46732,#46733,#46734,#46735,#46736,#46737,#46738,#46739,#46740,
#46741,#46742,#46743,#46744,#46745,#46746,#46747,#46748,#46749,#46750,#46751,
#46752,#46753,#46754,#46755,#46756,#46757,#46758,#46759,#46760,#46761,#46762,
#46763,#46764,#46765,#46766,#46767,#46768,#46769,#46770,#46771,#46772,#46773,
#46774,#46775,#46776,#46777,#46778,#46779),.UNSPECIFIED.,.F.,.F.,(4,3,3,
3,3,3,3,3,3,3,3,3,3,3,3,3,3,3,3,3,3,3,3,3,3,3,3,3,3,4),(0.,0.0669970386142676,
0.120382710412332,0.125000000000001,0.187500000000001,0.218750000000001,
0.234375000000001,0.242187500000001,0.248477936970486,0.250000000000001,
0.272887810025426,0.34017169545409,0.407404427623042,0.425042432395696,
0.491875641585318,0.500000000000001,0.566167202439539,0.575220629187228,
0.625000000000001,0.687500000000002,0.718750000000001,0.727380078328301,
0.734375000000001,0.742187500000001,0.74851347129672,0.750000000000001,
0.814942759651571,0.87988551930314,0.947512676699537,1.),.UNSPECIFIED.);
#789=B_SPLINE_CURVE_WITH_KNOTS('',3,(#46807,#46808,#46809,#46810,#46811,
#46812,#46813,#46814,#46815,#46816),.UNSPECIFIED.,.F.,.F.,(4,3,3,4),(0.,
0.3333333333333,0.6666666666667,1.),.UNSPECIFIED.);
#790=B_SPLINE_CURVE_WITH_KNOTS('',3,(#46866,#46867,#46868,#46869,#46870,
#46871,#46872,#46873,#46874,#46875,#46876,#46877,#46878,#46879,#46880,#46881,
#46882,#46883,#46884,#46885,#46886,#46887,#46888,#46889,#46890,#46891,#46892,
#46893,#46894,#46895,#46896,#46897,#46898,#46899,#46900,#46901,#46902,#46903,
#46904,#46905,#46906,#46907,#46908,#46909,#46910,#46911,#46912,#46913,#46914,
#46915,#46916,#46917,#46918,#46919,#46920,#46921,#46922,#46923,#46924,#46925,
#46926,#46927,#46928,#46929,#46930,#46931,#46932,#46933,#46934,#46935,#46936,
#46937,#46938),.UNSPECIFIED.,.F.,.F.,(4,3,3,3,3,3,3,3,3,3,3,3,3,3,3,3,3,
3,3,3,3,3,3,3,4),(0.,0.0458328892270865,0.0918178602216913,0.137727870876666,
0.1428571428571,0.148536598132325,0.203804992721712,0.259124754685508,0.2857142857143,
0.296137570173946,0.362354499372673,0.4285714285714,0.443717909279761,0.51100679814713,
0.5714285714286,0.591516277430998,0.658633939571757,0.7142857142857,0.739436741598742,
0.798289799370821,0.8571428571429,0.887213042157107,0.933524276499682,0.979590782777999,
1.),.UNSPECIFIED.);
#791=B_SPLINE_CURVE_WITH_KNOTS('',3,(#46940,#46941,#46942,#46943,#46944,
#46945,#46946,#46947,#46948,#46949,#46950,#46951,#46952,#46953,#46954,#46955,
#46956,#46957,#46958,#46959,#46960,#46961,#46962,#46963,#46964,#46965,#46966,
#46967,#46968,#46969,#46970,#46971,#46972,#46973,#46974,#46975,#46976,#46977,
#46978,#46979),.UNSPECIFIED.,.F.,.F.,(4,3,3,3,3,3,3,3,3,3,3,3,3,4),(0.,
0.132990595149974,0.153369582561691,0.288984797962432,0.306719318585581,
0.443622682221199,0.460361901680837,0.597256082674871,0.614811262622601,
0.75,0.769627678904013,0.909364143399665,0.92460957800544,1.),
 .UNSPECIFIED.);
#792=B_SPLINE_CURVE_WITH_KNOTS('',3,(#46980,#46981,#46982,#46983,#46984,
#46985,#46986,#46987,#46988,#46989,#46990,#46991,#46992,#46993,#46994,#46995,
#46996,#46997,#46998,#46999,#47000,#47001,#47002,#47003,#47004,#47005,#47006,
#47007,#47008,#47009,#47010,#47011,#47012,#47013,#47014,#47015,#47016,#47017,
#47018,#47019,#47020,#47021,#47022,#47023,#47024,#47025,#47026,#47027,#47028,
#47029,#47030,#47031),.UNSPECIFIED.,.F.,.F.,(4,3,3,3,3,3,3,3,3,3,3,3,3,
3,3,3,3,4),(0.,0.0996458179615122,0.194999931615914,0.249999999999888,0.342098757858286,
0.374999999999833,0.437499999999808,0.468749999999796,0.484374999999795,
0.494788821211196,0.499999999999793,0.582568432156327,0.661614822642106,
0.737537010890375,0.809528033495748,0.879516105785263,0.946950744268271,
1.),.UNSPECIFIED.);
#793=B_SPLINE_CURVE_WITH_KNOTS('',3,(#47071,#47072,#47073,#47074,#47075,
#47076,#47077),.UNSPECIFIED.,.F.,.F.,(4,3,4),(0.,0.5,0.999999999974384),
 .UNSPECIFIED.);
#794=B_SPLINE_CURVE_WITH_KNOTS('',3,(#47078,#47079,#47080,#47081,#47082,
#47083,#47084,#47085,#47086,#47087,#47088,#47089,#47090,#47091,#47092,#47093,
#47094,#47095,#47096,#47097,#47098,#47099,#47100,#47101,#47102,#47103,#47104,
#47105,#47106,#47107,#47108,#47109,#47110,#47111,#47112,#47113,#47114,#47115,
#47116,#47117),.UNSPECIFIED.,.F.,.F.,(4,3,3,3,3,3,3,3,3,3,3,3,3,4),(0.,
0.0902944655579604,0.118857317209722,0.250000000000003,0.363581344801778,
0.437500000000005,0.466152583203494,0.495170166324027,0.500000000000006,
0.615785321962388,0.718419711808763,0.827854048198698,0.933927706970455,
1.),.UNSPECIFIED.);
#795=B_SPLINE_CURVE_WITH_KNOTS('',3,(#47161,#47162,#47163,#47164,#47165,
#47166,#47167,#47168,#47169,#47170,#47171,#47172,#47173,#47174,#47175,#47176,
#47177,#47178,#47179,#47180,#47181,#47182,#47183,#47184,#47185,#47186,#47187,
#47188,#47189,#47190,#47191,#47192,#47193,#47194,#47195,#47196,#47197,#47198,
#47199,#47200,#47201,#47202,#47203,#47204,#47205,#47206,#47207,#47208,#47209,
#47210,#47211,#47212,#47213,#47214,#47215,#47216,#47217,#47218,#47219,#47220,
#47221,#47222,#47223,#47224,#47225,#47226,#47227,#47228,#47229,#47230,#47231,
#47232,#47233,#47234,#47235,#47236,#47237,#47238,#47239,#47240,#47241,#47242),
 .UNSPECIFIED.,.F.,.F.,(4,3,3,3,3,3,3,3,3,3,3,3,3,3,3,3,3,3,3,3,3,3,3,3,
3,3,3,4),(0.,0.0670666130844619,0.12030178167153,0.125,0.1875,0.21875,0.234375,
0.243836099690824,0.25,0.273217637634883,0.340387408247809,0.407458049097731,
0.42502958529848,0.491732958316918,0.5,0.56585106029968,0.574716454972842,
0.625,0.6875,0.71875,0.726524647119784,0.734375,0.743877173835152,0.75,
0.814715983346842,0.879431966693684,0.947069143523809,1.),.UNSPECIFIED.);
#796=B_SPLINE_CURVE_WITH_KNOTS('',3,(#47243,#47244,#47245,#47246,#47247,
#47248,#47249,#47250,#47251,#47252,#47253,#47254,#47255,#47256,#47257,#47258,
#47259,#47260,#47261,#47262,#47263,#47264,#47265,#47266,#47267,#47268,#47269,
#47270,#47271,#47272,#47273,#47274,#47275,#47276,#47277,#47278,#47279,#47280,
#47281,#47282,#47283,#47284,#47285),.UNSPECIFIED.,.F.,.F.,(4,3,3,3,3,3,
3,3,3,3,3,3,3,3,4),(0.,0.120531524854355,0.242397124478255,0.25,0.27549375772157,
0.398768379129118,0.425841349187489,0.549212605428686,0.573906646855301,
0.697195745258833,0.724246467936576,0.75,0.871872563813813,0.879199606827093,
0.99999999999059),.UNSPECIFIED.);
#797=B_SPLINE_CURVE_WITH_KNOTS('',3,(#47322,#47323,#47324,#47325,#47326,
#47327,#47328,#47329,#47330,#47331,#47332,#47333,#47334,#47335,#47336,#47337,
#47338,#47339,#47340,#47341,#47342,#47343,#47344,#47345,#47346,#47347,#47348,
#47349,#47350,#47351,#47352,#47353,#47354,#47355,#47356,#47357,#47358,#47359,
#47360,#47361,#47362,#47363,#47364,#47365,#47366,#47367,#47368,#47369,#47370,
#47371,#47372,#47373,#47374,#47375,#47376,#47377,#47378,#47379,#47380,#47381,
#47382,#47383,#47384,#47385,#47386,#47387,#47388,#47389,#47390,#47391,#47392,
#47393,#47394,#47395,#47396,#47397,#47398,#47399,#47400,#47401,#47402,#47403,
#47404,#47405,#47406,#47407,#47408,#47409,#47410,#47411,#47412,#47413,#47414,
#47415,#47416,#47417,#47418,#47419,#47420,#47421,#47422,#47423,#47424,#47425,
#47426,#47427,#47428,#47429,#47430,#47431,#47432,#47433,#47434,#47435,#47436,
#47437,#47438,#47439,#47440,#47441,#47442,#47443,#47444,#47445,#47446,#47447,
#47448,#47449,#47450,#47451,#47452,#47453,#47454),.UNSPECIFIED.,.F.,.F.,
(4,3,3,3,3,3,3,3,3,3,3,3,3,3,3,3,3,3,3,3,3,3,3,3,3,3,3,3,3,3,3,3,3,3,3,
3,3,3,3,3,3,3,3,3,4),(7.5007832586842E-8,0.0217670658682142,0.0431895788594497,
0.0625000000000103,0.0832736756201858,0.0937500000000153,0.109375000000018,
0.117187500000019,0.12109375000002,0.12304687500002,0.12451171875002,0.12500000000002,
0.152494864340801,0.179650433481905,0.187500000000019,0.214360095933258,
0.218750000000018,0.234375000000018,0.24351577464818,0.250000000000018,
0.312500000000017,0.365427443838984,0.375000000000015,0.416806169790061,
0.437500000000014,0.468750000000014,0.484375000000013,0.492187500000013,
0.499677511217752,0.500000000000013,0.544190340299808,0.589518547111297,
0.625000000000011,0.684246463305914,0.687500000000009,0.718750000000009,
0.734375000000008,0.742187500000008,0.746093750000008,0.749474899577793,
0.750000000000008,0.815485730321359,0.881497052371249,0.948535357396417,
1.),.UNSPECIFIED.);
#798=B_SPLINE_CURVE_WITH_KNOTS('',3,(#47455,#47456,#47457,#47458,#47459,
#47460,#47461,#47462,#47463,#47464),.UNSPECIFIED.,.F.,.F.,(4,2,2,2,4),(2.21660080701014E-8,
0.25,0.5,0.75,1.),.UNSPECIFIED.);
#799=B_SPLINE_CURVE_WITH_KNOTS('',3,(#47598,#47599,#47600,#47601,#47602,
#47603,#47604,#47605,#47606,#47607,#47608,#47609,#47610,#47611,#47612,#47613,
#47614,#47615,#47616,#47617,#47618,#47619,#47620,#47621,#47622,#47623,#47624,
#47625,#47626,#47627,#47628,#47629,#47630,#47631,#47632,#47633,#47634,#47635,
#47636,#47637,#47638,#47639,#47640,#47641,#47642,#47643,#47644,#47645,#47646,
#47647,#47648,#47649,#47650,#47651,#47652,#47653,#47654,#47655,#47656,#47657,
#47658,#47659,#47660,#47661,#47662,#47663,#47664,#47665,#47666,#47667,#47668,
#47669,#47670,#47671,#47672,#47673,#47674,#47675,#47676,#47677,#47678,#47679,
#47680,#47681,#47682,#47683,#47684,#47685),.UNSPECIFIED.,.F.,.F.,(4,2,2,
1,2,2,2,1,1,1,2,2,2,2,1,1,1,2,2,2,2,2,2,2,2,2,1,2,2,2,1,1,2,2,2,2,1,1,2,
2,2,2,1,1,2,2,2,1,1,2,2,4),(0.,0.0312500000000003,0.0468750000000006,0.0546875000000004,
0.0585937500000001,0.0624999999999998,0.0937499999999988,0.109374999999998,
0.117187499999998,0.121093749999998,0.123046874999998,0.124999999999998,
0.187499999999995,0.218749999999994,0.234374999999994,0.242187499999994,
0.246093749999994,0.248046874999994,0.249999999999994,0.312499999999996,
0.343749999999997,0.359374999999998,0.374999999999998,0.4375,0.468750000000001,
0.484375000000002,0.492187500000002,0.496093750000002,0.500000000000003,
0.562500000000005,0.593750000000006,0.609375000000007,0.617187500000007,
0.625000000000007,0.687500000000008,0.718750000000009,0.734375000000009,
0.742187500000009,0.746093750000009,0.750000000000009,0.812500000000006,
0.843750000000005,0.859375000000004,0.867187500000004,0.871093750000004,
0.875000000000004,0.906250000000002,0.921875000000002,0.929687500000001,
0.933593750000001,0.937500000000001,1.),.UNSPECIFIED.);
#800=B_SPLINE_CURVE_WITH_KNOTS('',3,(#47732,#47733,#47734,#47735,#47736,
#47737,#47738,#47739,#47740,#47741,#47742,#47743,#47744,#47745,#47746,#47747,
#47748,#47749,#47750,#47751,#47752,#47753),.UNSPECIFIED.,.F.,.F.,(4,3,3,
3,3,3,3,4),(1.01038572354475E-7,0.1428571428571,0.2857142857143,0.4285714285714,
0.5714285714286,0.7142857142857,0.8571428571429,1.),.UNSPECIFIED.);
#801=B_SPLINE_CURVE_WITH_KNOTS('',3,(#47754,#47755,#47756,#47757,#47758,
#47759,#47760,#47761,#47762,#47763,#47764,#47765,#47766,#47767,#47768,#47769,
#47770,#47771,#47772,#47773,#47774,#47775,#47776,#47777,#47778,#47779,#47780,
#47781,#47782,#47783,#47784,#47785,#47786,#47787,#47788,#47789,#47790,#47791,
#47792,#47793,#47794,#47795,#47796,#47797,#47798,#47799,#47800,#47801,#47802,
#47803,#47804,#47805),.UNSPECIFIED.,.F.,.F.,(4,3,3,3,3,3,3,3,3,3,3,3,3,
3,3,3,3,4),(0.,0.065830358537903,0.133277278734282,0.203793753321675,0.25000000000003,
0.328519758658406,0.375000000000045,0.437500000000051,0.468750000000049,
0.48437500000005,0.495342149468993,0.50000000000005,0.586653387589681,0.675658006518003,
0.76905306807574,0.865255834852487,0.966232492263845,1.),.UNSPECIFIED.);
#802=B_SPLINE_CURVE_WITH_KNOTS('',3,(#47843,#47844,#47845,#47846,#47847,
#47848,#47849,#47850,#47851,#47852,#47853,#47854,#47855,#47856,#47857,#47858,
#47859,#47860,#47861,#47862,#47863,#47864,#47865,#47866,#47867,#47868,#47869,
#47870,#47871,#47872,#47873,#47874,#47875,#47876,#47877,#47878,#47879,#47880,
#47881,#47882,#47883,#47884,#47885,#47886,#47887,#47888,#47889,#47890,#47891),
 .UNSPECIFIED.,.F.,.F.,(4,3,3,3,3,3,3,3,3,3,3,3,3,3,3,3,4),(0.,0.0770829581291472,
0.115833104594291,0.197028807380885,0.250000000000002,0.333153117301368,
0.356333767049974,0.375000000000002,0.422947860458973,0.471329030452833,
0.500000000000003,0.606855024376987,0.708280894756902,0.713710048753971,
0.815228553265648,0.918005904080637,1.),.UNSPECIFIED.);
#803=B_SPLINE_CURVE_WITH_KNOTS('',3,(#47892,#47893,#47894,#47895,#47896,
#47897,#47898),.UNSPECIFIED.,.F.,.F.,(4,3,4),(1.79043455598195E-11,0.5,
0.999999979798419),.UNSPECIFIED.);
#804=B_SPLINE_CURVE_WITH_KNOTS('',3,(#47939,#47940,#47941,#47942,#47943,
#47944,#47945),.UNSPECIFIED.,.F.,.F.,(4,3,4),(0.,0.5,1.),.UNSPECIFIED.);
#805=B_SPLINE_CURVE_WITH_KNOTS('',3,(#47947,#47948,#47949,#47950,#47951,
#47952,#47953,#47954,#47955,#47956,#47957,#47958,#47959,#47960,#47961,#47962,
#47963,#47964,#47965,#47966,#47967,#47968,#47969,#47970,#47971,#47972,#47973,
#47974,#47975,#47976,#47977,#47978,#47979,#47980,#47981,#47982,#47983,#47984,
#47985,#47986,#47987,#47988,#47989),.UNSPECIFIED.,.F.,.F.,(4,3,3,3,3,3,
3,3,3,3,3,3,3,3,4),(0.,0.0912182191841853,0.112406184524464,0.234107463982405,
0.249999999999994,0.356823512053016,0.437499999999994,0.466379266642358,
0.495620975073898,0.499999999999994,0.61567283621949,0.711311199443657,
0.820914964356108,0.927083278900066,1.),.UNSPECIFIED.);
#806=B_SPLINE_CURVE_WITH_KNOTS('',3,(#47990,#47991,#47992,#47993,#47994,
#47995,#47996,#47997,#47998,#47999,#48000,#48001,#48002,#48003,#48004,#48005,
#48006,#48007,#48008,#48009,#48010,#48011,#48012,#48013,#48014,#48015,#48016,
#48017,#48018,#48019,#48020,#48021,#48022,#48023,#48024,#48025,#48026,#48027,
#48028,#48029,#48030,#48031,#48032,#48033,#48034,#48035,#48036,#48037,#48038,
#48039,#48040,#48041,#48042,#48043,#48044,#48045,#48046,#48047),
 .UNSPECIFIED.,.F.,.F.,(4,3,3,3,3,3,3,3,3,3,3,3,3,3,3,3,3,3,3,4),(0.,0.103649568295827,
0.142660071316879,0.249999999999991,0.34718853504273,0.365815758592943,
0.374999999999986,0.437499999999983,0.468749999999981,0.48437499999998,
0.494825109892429,0.49999999999998,0.589167146235496,0.599109405757341,
0.685328701907224,0.74999999999999,0.831438322732351,0.908502174159926,
0.980614281843201,1.),.UNSPECIFIED.);
#807=B_SPLINE_CURVE_WITH_KNOTS('',3,(#48093,#48094,#48095,#48096,#48097,
#48098,#48099,#48100,#48101,#48102,#48103,#48104,#48105,#48106,#48107,#48108,
#48109,#48110,#48111,#48112,#48113,#48114,#48115,#48116,#48117,#48118,#48119,
#48120,#48121,#48122,#48123,#48124,#48125,#48126,#48127,#48128,#48129,#48130,
#48131,#48132,#48133,#48134,#48135,#48136,#48137,#48138,#48139,#48140,#48141,
#48142,#48143,#48144,#48145,#48146,#48147,#48148,#48149,#48150,#48151,#48152,
#48153,#48154,#48155,#48156,#48157,#48158,#48159,#48160,#48161,#48162,#48163,
#48164,#48165),.UNSPECIFIED.,.F.,.F.,(4,3,3,3,3,3,3,3,3,3,3,3,3,3,3,3,3,
3,3,3,3,3,3,3,4),(0.,0.045832881241204,0.0918178429888426,0.137727842667475,
0.1428571428571,0.148537109981302,0.203805441048692,0.259125141483677,0.2857142857143,
0.296138265585979,0.362354847078689,0.4285714285714,0.443718112652216,0.511007039282419,
0.5714285714286,0.591515929724954,0.658633627239864,0.7142857142857,0.739436118141299,
0.7982894876421,0.8571428571429,0.887212493461699,0.933523713871146,0.979590209317017,
1.),.UNSPECIFIED.);
#808=B_SPLINE_CURVE_WITH_KNOTS('',3,(#48168,#48169,#48170,#48171,#48172,
#48173,#48174,#48175,#48176,#48177,#48178,#48179,#48180,#48181,#48182,#48183,
#48184,#48185,#48186,#48187,#48188,#48189,#48190,#48191,#48192,#48193,#48194,
#48195,#48196,#48197,#48198,#48199,#48200,#48201,#48202,#48203,#48204,#48205,
#48206,#48207),.UNSPECIFIED.,.F.,.F.,(4,3,3,3,3,3,3,3,3,3,3,3,3,4),(0.,
0.132990611297914,0.153370101342381,0.288985346045089,0.306720032640923,
0.443623462076149,0.460362109994673,0.597256328470644,0.614810899859838,
0.75,0.769627029706129,0.909362740892189,0.924609009850741,0.999999999982011),
 .UNSPECIFIED.);
#809=B_SPLINE_CURVE_WITH_KNOTS('',3,(#48230,#48231,#48232,#48233,#48234,
#48235,#48236,#48237,#48238,#48239),.UNSPECIFIED.,.F.,.F.,(4,3,3,4),(0.,
0.3333333333333,0.6666666666667,1.),.UNSPECIFIED.);
#810=B_SPLINE_CURVE_WITH_KNOTS('',3,(#48375,#48376,#48377,#48378,#48379,
#48380,#48381,#48382,#48383,#48384,#48385,#48386,#48387,#48388,#48389,#48390,
#48391,#48392,#48393,#48394,#48395,#48396,#48397,#48398,#48399,#48400,#48401,
#48402,#48403,#48404,#48405,#48406,#48407,#48408,#48409,#48410,#48411,#48412,
#48413,#48414,#48415,#48416,#48417,#48418,#48419,#48420,#48421,#48422,#48423,
#48424,#48425,#48426,#48427,#48428,#48429,#48430,#48431,#48432,#48433,#48434,
#48435,#48436,#48437,#48438,#48439,#48440,#48441,#48442,#48443,#48444,#48445,
#48446,#48447,#48448,#48449,#48450,#48451,#48452,#48453,#48454,#48455,#48456,
#48457,#48458,#48459,#48460,#48461),.UNSPECIFIED.,.F.,.F.,(4,2,2,1,2,2,
2,1,1,1,2,2,2,2,1,1,1,2,2,2,2,2,2,2,2,1,1,2,2,2,1,1,2,2,2,2,1,1,2,2,2,2,
1,1,2,2,2,1,1,2,2,4),(0.,0.0312499999999956,0.0468749999999935,0.0546874999999927,
0.0585937499999926,0.0624999999999925,0.0937499999999921,0.109374999999992,
0.117187499999992,0.121093749999992,0.123046874999992,0.124999999999992,
0.187499999999993,0.218749999999993,0.234374999999993,0.242187499999993,
0.246093749999993,0.248046874999993,0.249999999999993,0.312499999999994,
0.343749999999994,0.359374999999994,0.374999999999994,0.437499999999994,
0.468749999999994,0.484374999999994,0.492187499999994,0.496093749999994,
0.499999999999994,0.562499999999994,0.593749999999994,0.609374999999994,
0.617187499999994,0.624999999999994,0.687499999999994,0.718749999999995,
0.734374999999995,0.742187499999995,0.746093749999995,0.749999999999995,
0.812499999999997,0.843749999999998,0.859374999999998,0.867187499999998,
0.871093749999998,0.874999999999998,0.906249999999999,0.921874999999999,
0.9296875,0.93359375,0.9375,1.),.UNSPECIFIED.);
#811=B_SPLINE_CURVE_WITH_KNOTS('',3,(#48464,#48465,#48466,#48467,#48468,
#48469,#48470,#48471,#48472,#48473,#48474,#48475,#48476,#48477,#48478,#48479,
#48480,#48481,#48482,#48483,#48484,#48485,#48486,#48487,#48488,#48489,#48490,
#48491,#48492,#48493,#48494,#48495,#48496,#48497,#48498,#48499,#48500,#48501,
#48502,#48503,#48504,#48505,#48506,#48507,#48508,#48509,#48510,#48511,#48512,
#48513,#48514,#48515,#48516,#48517,#48518,#48519,#48520,#48521,#48522,#48523,
#48524,#48525,#48526,#48527,#48528,#48529,#48530,#48531,#48532,#48533,#48534,
#48535,#48536,#48537,#48538,#48539,#48540,#48541,#48542,#48543,#48544,#48545,
#48546,#48547,#48548,#48549,#48550,#48551,#48552,#48553,#48554,#48555,#48556,
#48557,#48558,#48559,#48560,#48561,#48562,#48563,#48564,#48565,#48566,#48567,
#48568,#48569,#48570,#48571,#48572,#48573,#48574,#48575,#48576,#48577,#48578,
#48579,#48580,#48581,#48582,#48583,#48584,#48585,#48586,#48587,#48588,#48589,
#48590,#48591,#48592,#48593,#48594,#48595,#48596,#48597,#48598,#48599,#48600,
#48601,#48602,#48603,#48604,#48605,#48606,#48607,#48608,#48609,#48610,#48611,
#48612,#48613,#48614,#48615,#48616,#48617,#48618,#48619,#48620,#48621,#48622,
#48623,#48624,#48625,#48626,#48627,#48628,#48629,#48630,#48631,#48632,#48633,
#48634,#48635,#48636,#48637,#48638,#48639,#48640,#48641,#48642,#48643,#48644,
#48645,#48646,#48647,#48648,#48649,#48650),.UNSPECIFIED.,.F.,.F.,(4,3,3,
3,3,3,3,3,3,3,3,3,3,3,3,3,3,3,3,3,3,3,3,3,3,3,3,3,3,3,3,3,3,3,3,3,3,3,3,
3,3,3,3,3,3,3,3,3,3,3,3,3,3,3,3,3,3,3,3,3,3,3,4),(7.50077796095116E-8,2.1834712232905E-7,
0.0229486522988532,0.029115344241334,0.0509750486302945,0.0551857885997794,
0.0625000000000054,0.0795341640465225,0.100118382040926,0.102946158886626,
0.109375000000009,0.11718750000001,0.12109375000001,0.123046875000011,0.124511718750011,
0.125000000000011,0.126823937250289,0.154172453479257,0.168540242544379,
0.195094304959414,0.207813101074959,0.23437500000001,0.243585841679061,
0.245601800237161,0.25000000000001,0.286460598154731,0.323176994279279,
0.335372913036784,0.372213805675533,0.396049928737796,0.433011067267819,
0.468750000000008,0.471303252420127,0.484375000000008,0.492187500000008,
0.499323792057643,0.500000000000007,0.539363292696495,0.553186327532695,
0.592468810689562,0.619362211295797,0.658497292358972,0.673124010224558,
0.711990573304192,0.716723793723807,0.718750000000005,0.734375000000005,
0.742187500000005,0.746093750000005,0.749489149398016,0.750000000000005,
0.75369509666723,0.78978336194932,0.822481585671004,0.85189171104547,0.878121450578709,
0.901492804926207,0.922411611492371,0.941273455320735,0.958424926741568,
0.974021468761295,0.988170844049958,1.),.UNSPECIFIED.);
#812=B_SPLINE_CURVE_WITH_KNOTS('',3,(#48687,#48688,#48689,#48690,#48691,
#48692,#48693,#48694,#48695,#48696),.UNSPECIFIED.,.F.,.F.,(4,2,2,2,4),(2.21659726367817E-8,
0.25,0.5,0.75,1.),.UNSPECIFIED.);
#813=B_SPLINE_CURVE_WITH_KNOTS('',3,(#48697,#48698,#48699,#48700,#48701,
#48702,#48703,#48704,#48705,#48706,#48707,#48708,#48709,#48710,#48711,#48712,
#48713,#48714,#48715,#48716,#48717,#48718,#48719,#48720,#48721,#48722,#48723,
#48724,#48725,#48726,#48727,#48728,#48729,#48730,#48731,#48732,#48733,#48734,
#48735,#48736,#48737,#48738,#48739,#48740,#48741,#48742,#48743,#48744,#48745,
#48746,#48747,#48748,#48749,#48750,#48751,#48752,#48753,#48754,#48755,#48756,
#48757),.UNSPECIFIED.,.F.,.F.,(4,3,3,3,3,3,3,3,3,3,3,3,3,3,3,3,3,3,3,3,
4),(3.81864810483332E-11,0.100941758984912,0.175470879492456,0.239253214458431,
0.25,0.301331982929159,0.350998987196869,0.399809398891569,0.449904699445784,
0.497278586630275,0.5,0.500002028503135,0.54746307741508,0.595562936975098,
0.644828923272954,0.697414461636477,0.75,0.813347304646379,0.889651753803061,
0.988069371159003,0.999999999951421),.UNSPECIFIED.);
#814=B_SPLINE_CURVE_WITH_KNOTS('',3,(#48812,#48813,#48814,#48815,#48816,
#48817,#48818,#48819,#48820,#48821,#48822,#48823,#48824,#48825,#48826,#48827,
#48828,#48829,#48830,#48831,#48832,#48833,#48834,#48835,#48836,#48837,#48838,
#48839,#48840,#48841,#48842,#48843,#48844,#48845,#48846,#48847,#48848,#48849,
#48850,#48851,#48852,#48853,#48854,#48855,#48856,#48857,#48858,#48859,#48860,
#48861,#48862,#48863,#48864,#48865,#48866,#48867,#48868,#48869,#48870,#48871,
#48872,#48873,#48874,#48875,#48876,#48877,#48878,#48879,#48880,#48881,#48882,
#48883,#48884,#48885,#48886,#48887,#48888,#48889,#48890,#48891,#48892,#48893,
#48894,#48895,#48896,#48897,#48898,#48899,#48900,#48901,#48902,#48903,#48904,
#48905,#48906,#48907,#48908,#48909,#48910,#48911,#48912,#48913,#48914,#48915,
#48916,#48917,#48918,#48919,#48920),.UNSPECIFIED.,.F.,.F.,(4,3,3,3,3,3,
3,3,3,3,3,3,3,3,3,3,3,3,3,3,3,3,3,3,3,3,3,3,3,3,3,3,3,3,3,3,4),(0.,0.0469750755483397,
0.107013261195238,0.125000000000003,0.158323162137369,0.187500000000005,
0.218750000000006,0.234375000000006,0.242187500000006,0.246093750000006,
0.248046875000006,0.250000000000006,0.272270513448122,0.328769794302826,
0.380131831410091,0.436169931231429,0.490512436112259,0.500000000000005,
0.500020141526524,0.552994048955501,0.607576031489257,0.619923874724667,
0.625000000000005,0.682586167998106,0.687500000000005,0.718750000000005,
0.727765077201715,0.734375000000005,0.742187500000005,0.746093750000005,
0.748046875000005,0.750000000000005,0.808692100492686,0.841709576216595,
0.902639581263564,0.953058336704736,0.999999999999993),.UNSPECIFIED.);
#815=B_SPLINE_CURVE_WITH_KNOTS('',3,(#48959,#48960,#48961,#48962,#48963,
#48964,#48965,#48966,#48967,#48968,#48969,#48970,#48971,#48972,#48973,#48974,
#48975,#48976,#48977,#48978,#48979,#48980,#48981,#48982,#48983,#48984,#48985,
#48986,#48987,#48988,#48989,#48990,#48991,#48992,#48993,#48994,#48995,#48996,
#48997,#48998,#48999,#49000,#49001,#49002,#49003,#49004),.UNSPECIFIED.,
 .F.,.F.,(4,3,3,3,3,3,3,3,3,3,3,3,3,3,3,4),(0.,0.0782430522660074,0.11197985752849,
0.1933350730998,0.249999999999997,0.333365304872076,0.352554727932383,0.374999999999995,
0.421439760445618,0.468291981355138,0.499999999999995,0.60472551068549,
0.709451021370985,0.81095438778007,0.913715460883307,1.),.UNSPECIFIED.);
#816=B_SPLINE_CURVE_WITH_KNOTS('',3,(#49005,#49006,#49007,#49008,#49009,
#49010,#49011),.UNSPECIFIED.,.F.,.F.,(4,3,4),(0.,0.5,1.),.UNSPECIFIED.);
#817=B_SPLINE_CURVE_WITH_KNOTS('',3,(#49012,#49013,#49014,#49015,#49016,
#49017,#49018,#49019,#49020,#49021,#49022,#49023,#49024,#49025,#49026,#49027,
#49028,#49029,#49030,#49031,#49032,#49033,#49034,#49035,#49036,#49037,#49038,
#49039,#49040,#49041,#49042,#49043,#49044,#49045,#49046,#49047,#49048,#49049,
#49050,#49051,#49052,#49053,#49054,#49055,#49056,#49057,#49058,#49059,#49060,
#49061,#49062,#49063,#49064,#49065,#49066,#49067,#49068,#49069),
 .UNSPECIFIED.,.F.,.F.,(4,3,3,3,3,3,3,3,3,3,3,3,3,3,3,3,3,3,3,4),(0.,0.0713925938266771,
0.147548684834906,0.169708372945268,0.249999999999987,0.33487881468383,
0.374999999999981,0.402047408896451,0.43749999999998,0.468749999999982,
0.484374999999984,0.49538572687912,0.499999999999986,0.594440192107133,
0.635063053479894,0.732129617709673,0.835445829871013,0.857807936589943,
0.961497480103932,1.),.UNSPECIFIED.);
#818=B_SPLINE_CURVE_WITH_KNOTS('',3,(#49112,#49113,#49114,#49115,#49116,
#49117,#49118,#49119,#49120,#49121,#49122,#49123,#49124,#49125,#49126,#49127,
#49128,#49129,#49130,#49131,#49132,#49133),.UNSPECIFIED.,.F.,.F.,(4,3,3,
3,3,3,3,4),(1.01038257746567E-7,0.1428571428571,0.2857142857143,0.4285714285714,
0.5714285714286,0.7142857142857,0.8571428571429,1.),.UNSPECIFIED.);
#819=B_SPLINE_CURVE_WITH_KNOTS('',3,(#49176,#49177,#49178,#49179,#49180,
#49181,#49182),.UNSPECIFIED.,.F.,.F.,(4,3,4),(0.,0.5,1.),.UNSPECIFIED.);
#820=B_SPLINE_CURVE_WITH_KNOTS('',3,(#49184,#49185,#49186,#49187,#49188,
#49189,#49190,#49191,#49192,#49193,#49194,#49195,#49196,#49197,#49198,#49199,
#49200,#49201,#49202,#49203,#49204,#49205,#49206,#49207,#49208,#49209,#49210,
#49211,#49212,#49213,#49214,#49215,#49216,#49217,#49218,#49219,#49220,#49221,
#49222,#49223,#49224,#49225,#49226),.UNSPECIFIED.,.F.,.F.,(4,3,3,3,3,3,
3,3,3,3,3,3,3,3,4),(0.,0.0911164890363828,0.111478099373908,0.233136812955381,
0.250000000000001,0.35510274217642,0.437500000000001,0.466389059279721,
0.495640200714861,0.500000000000002,0.615671350380528,0.707817213420784,
0.817519612891894,0.923748890587099,1.),.UNSPECIFIED.);
#821=B_SPLINE_CURVE_WITH_KNOTS('',3,(#49227,#49228,#49229,#49230,#49231,
#49232,#49233,#49234,#49235,#49236,#49237,#49238,#49239,#49240,#49241,#49242,
#49243,#49244,#49245,#49246,#49247,#49248,#49249,#49250,#49251,#49252,#49253,
#49254,#49255,#49256,#49257,#49258,#49259,#49260,#49261,#49262,#49263,#49264,
#49265,#49266,#49267,#49268,#49269,#49270,#49271,#49272,#49273,#49274,#49275,
#49276,#49277,#49278,#49279,#49280,#49281,#49282,#49283,#49284),
 .UNSPECIFIED.,.F.,.F.,(4,3,3,3,3,3,3,3,3,3,3,3,3,3,3,3,3,3,3,4),(0.,0.103631820601983,
0.141618933845124,0.249999999999985,0.347157432574721,0.364507186385042,
0.374999999999978,0.437499999999977,0.46874999999998,0.484374999999984,
0.494780989963732,0.499999999999987,0.588702567953257,0.597579109022073,
0.683307469833132,0.749999999999994,0.830117206554479,0.906641913854849,
0.978194795254131,1.),.UNSPECIFIED.);
#822=B_SPLINE_CURVE_WITH_KNOTS('',3,(#49326,#49327,#49328,#49329,#49330,
#49331,#49332,#49333,#49334,#49335,#49336,#49337,#49338,#49339,#49340,#49341,
#49342,#49343,#49344,#49345,#49346,#49347),.UNSPECIFIED.,.F.,.F.,(4,3,3,
3,3,3,3,4),(0.,0.1428571428571,0.2857142857143,0.4285714285714,0.5714285714286,
0.7142857142857,0.8571428571429,0.999999898934671),.UNSPECIFIED.);
#823=B_SPLINE_CURVE_WITH_KNOTS('',3,(#49350,#49351,#49352,#49353,#49354,
#49355,#49356,#49357,#49358,#49359),.UNSPECIFIED.,.F.,.F.,(4,2,2,2,4),(0.,
0.25,0.5,0.75,0.999999977827931),.UNSPECIFIED.);
#824=B_SPLINE_CURVE_WITH_KNOTS('',3,(#49389,#49390,#49391,#49392,#49393,
#49394,#49395,#49396,#49397,#49398,#49399,#49400,#49401),.UNSPECIFIED.,
 .F.,.F.,(4,3,3,3,4),(0.,0.0431918506380903,0.5,0.956806409374189,1.),
 .UNSPECIFIED.);
#825=B_SPLINE_CURVE_WITH_KNOTS('',3,(#49422,#49423,#49424,#49425,#49426,
#49427,#49428,#49429,#49430,#49431,#49432,#49433,#49434,#49435,#49436,#49437,
#49438,#49439,#49440,#49441,#49442,#49443,#49444,#49445,#49446,#49447,#49448,
#49449,#49450,#49451,#49452,#49453,#49454,#49455,#49456,#49457,#49458,#49459,
#49460,#49461,#49462,#49463,#49464,#49465,#49466,#49467,#49468,#49469,#49470,
#49471,#49472,#49473,#49474,#49475,#49476,#49477,#49478,#49479,#49480,#49481,
#49482,#49483,#49484,#49485,#49486,#49487,#49488,#49489,#49490,#49491,#49492,
#49493,#49494,#49495,#49496,#49497,#49498,#49499,#49500,#49501,#49502,#49503,
#49504,#49505,#49506,#49507,#49508,#49509,#49510,#49511,#49512,#49513,#49514,
#49515,#49516,#49517,#49518,#49519,#49520,#49521,#49522,#49523,#49524,#49525,
#49526,#49527,#49528,#49529,#49530,#49531,#49532,#49533,#49534,#49535,#49536,
#49537,#49538,#49539,#49540,#49541,#49542,#49543,#49544,#49545,#49546,#49547,
#49548,#49549,#49550,#49551,#49552,#49553,#49554,#49555,#49556,#49557,#49558,
#49559,#49560,#49561,#49562,#49563,#49564,#49565,#49566,#49567,#49568,#49569,
#49570,#49571,#49572,#49573,#49574,#49575,#49576,#49577,#49578,#49579,#49580,
#49581,#49582,#49583,#49584,#49585,#49586,#49587,#49588,#49589,#49590,#49591,
#49592,#49593,#49594,#49595,#49596,#49597,#49598,#49599,#49600,#49601,#49602,
#49603,#49604,#49605,#49606,#49607,#49608,#49609,#49610,#49611,#49612,#49613,
#49614,#49615,#49616,#49617,#49618,#49619,#49620,#49621,#49622,#49623,#49624,
#49625,#49626),.UNSPECIFIED.,.F.,.F.,(4,3,3,3,3,3,3,3,3,3,3,3,3,3,3,3,3,
3,3,3,3,3,3,3,3,3,3,3,3,3,3,3,3,3,3,3,3,3,3,3,3,3,3,3,3,3,3,3,3,3,3,3,3,
3,3,3,3,3,3,3,3,3,3,3,3,3,3,3,4),(0.,0.0249804636836571,0.0498736791136485,
0.0680715392667395,0.0924456145405575,0.107891047923709,0.13155027304587,
0.140978184745424,0.163936834710769,0.171012733705645,0.193309979955154,
0.19957661620216,0.218750000000013,0.227549376577307,0.234375000000014,
0.242187500000015,0.246093750000015,0.248046875000015,0.249023437500015,
0.250000000000015,0.254527365901607,0.279953693811535,0.307391988817704,
0.309413242316365,0.337113752967077,0.344147025953986,0.371988483723474,
0.384896192383363,0.412553839552332,0.429823366019842,0.457830262004141,
0.468750000000032,0.477221641980619,0.484375000000033,0.492187500000034,
0.496093750000034,0.498046875000034,0.500000000000034,0.531271360692087,
0.565625668115633,0.578495294938005,0.613113327045429,0.616389579700112,
0.648091824942008,0.674916203548571,0.697979818908304,0.718065266624333,
0.718750000000046,0.734375000000046,0.735689389724538,0.742187500000047,
0.746093750000047,0.748046875000047,0.749023437500047,0.750000000000047,
0.751857160445813,0.773870925559924,0.795148605277167,0.815780746718848,
0.835884720177279,0.855614046419167,0.875000000000023,0.875173192428097,
0.894783855532303,0.914592979453005,0.93477486045262,0.955588500169355,
0.977472532414895,0.999999988514636),.UNSPECIFIED.);
#826=B_SPLINE_CURVE_WITH_KNOTS('',3,(#49789,#49790,#49791,#49792,#49793,
#49794,#49795,#49796,#49797,#49798,#49799,#49800,#49801,#49802,#49803,#49804,
#49805,#49806,#49807,#49808,#49809,#49810,#49811,#49812,#49813,#49814,#49815,
#49816,#49817,#49818,#49819,#49820,#49821,#49822,#49823,#49824,#49825,#49826,
#49827,#49828,#49829,#49830,#49831,#49832,#49833,#49834,#49835,#49836,#49837,
#49838,#49839,#49840,#49841,#49842,#49843,#49844,#49845,#49846,#49847,#49848,
#49849,#49850,#49851,#49852,#49853,#49854,#49855,#49856,#49857,#49858,#49859,
#49860,#49861,#49862,#49863,#49864,#49865,#49866,#49867,#49868,#49869,#49870,
#49871,#49872,#49873,#49874,#49875,#49876,#49877,#49878,#49879,#49880,#49881,
#49882,#49883,#49884,#49885,#49886,#49887,#49888,#49889,#49890,#49891,#49892,
#49893,#49894,#49895,#49896,#49897,#49898,#49899,#49900,#49901,#49902,#49903,
#49904,#49905,#49906,#49907,#49908,#49909),.UNSPECIFIED.,.F.,.F.,(4,3,3,
3,3,3,3,3,3,3,3,3,3,3,3,3,3,3,3,3,3,3,3,3,3,3,3,3,3,3,3,3,3,3,3,3,3,3,3,
3,4),(7.98329640859155E-8,0.0312500598747272,0.0618422344833354,0.093421117241676,
0.125000000000017,0.155569259137103,0.187159629568566,0.218750000000029,
0.234375000000031,0.242187500000032,0.246093750000032,0.248046875000033,
0.249023437500033,0.250000000000033,0.450296396147656,0.499981289091065,
0.500000000000053,0.625000000000064,0.687500000000069,0.718750000000071,
0.734375000000072,0.742187500000073,0.749511718750074,0.750000000000074,
0.765919093593849,0.781838365516704,0.797757825884924,0.813677598178679,
0.829597550311721,0.845517805734134,0.859375000000023,0.86718750000002,
0.871093750000018,0.873046875000017,0.874023437500017,0.875000000000016,
0.899836887460964,0.924877651876229,0.949727955905382,0.974863950513704,
0.999999945122025),.UNSPECIFIED.);
#827=B_SPLINE_CURVE_WITH_KNOTS('',3,(#49950,#49951,#49952,#49953,#49954,
#49955,#49956,#49957,#49958,#49959,#49960,#49961,#49962,#49963,#49964,#49965,
#49966,#49967,#49968,#49969,#49970,#49971,#49972,#49973,#49974,#49975,#49976,
#49977,#49978,#49979,#49980,#49981,#49982,#49983,#49984,#49985,#49986,#49987,
#49988,#49989,#49990,#49991,#49992,#49993,#49994,#49995),.UNSPECIFIED.,
 .F.,.F.,(4,3,3,3,3,3,3,3,3,3,3,3,3,3,3,4),(0.,0.0782533266680479,0.111885264806691,
0.193250892056667,0.25,0.333382423143553,0.353144888706974,0.375000000000001,
0.421430089632216,0.468271936287447,0.500000000000001,0.605744038432394,
0.711488076864787,0.812997093824424,0.915766521323154,1.),.UNSPECIFIED.);
#828=B_SPLINE_CURVE_WITH_KNOTS('',3,(#49997,#49998,#49999,#50000,#50001,
#50002,#50003),.UNSPECIFIED.,.F.,.F.,(4,3,4),(0.,0.5,1.),.UNSPECIFIED.);
#829=B_SPLINE_CURVE_WITH_KNOTS('',3,(#50006,#50007,#50008,#50009,#50010,
#50011,#50012,#50013,#50014,#50015,#50016,#50017,#50018,#50019,#50020,#50021,
#50022,#50023,#50024,#50025,#50026,#50027,#50028,#50029,#50030,#50031,#50032,
#50033,#50034,#50035,#50036,#50037,#50038,#50039,#50040,#50041,#50042,#50043,
#50044,#50045,#50046,#50047,#50048,#50049,#50050,#50051,#50052,#50053,#50054,
#50055,#50056,#50057,#50058,#50059,#50060,#50061,#50062,#50063),
 .UNSPECIFIED.,.F.,.F.,(4,3,3,3,3,3,3,3,3,3,3,3,3,3,3,3,3,3,3,4),(0.,0.0718960185229564,
0.148549048540975,0.168812943342999,0.250000000000035,0.335330459216654,
0.375000000000054,0.401332658039912,0.437500000000066,0.468750000000068,
0.484375000000069,0.4954147011734,0.50000000000007,0.594522675873066,0.634654368293966,
0.731775982825236,0.835154805307982,0.857963598960442,0.961721678414487,
1.),.UNSPECIFIED.);
#830=B_SPLINE_CURVE_WITH_KNOTS('',3,(#50104,#50105,#50106,#50107,#50108,
#50109,#50110,#50111,#50112,#50113,#50114,#50115,#50116,#50117,#50118,#50119,
#50120,#50121,#50122,#50123,#50124,#50125,#50126,#50127,#50128,#50129,#50130,
#50131,#50132,#50133,#50134,#50135,#50136,#50137,#50138,#50139,#50140,#50141,
#50142,#50143,#50144,#50145,#50146),.UNSPECIFIED.,.F.,.F.,(4,3,3,3,3,3,
3,3,3,3,3,3,3,3,4),(2.75833894896721E-11,0.0832137801231444,0.218577222507133,
0.246109198300411,0.25,0.383459482332676,0.408370355156758,0.541180692332896,
0.57005641089706,0.702294441295682,0.731364778032269,0.75,0.881938303227582,
0.892442188083098,0.999999987394052),.UNSPECIFIED.);
#831=B_SPLINE_CURVE_WITH_KNOTS('',3,(#50147,#50148,#50149,#50150,#50151,
#50152,#50153,#50154,#50155,#50156,#50157,#50158,#50159,#50160,#50161,#50162,
#50163,#50164,#50165,#50166,#50167,#50168,#50169,#50170,#50171,#50172,#50173,
#50174,#50175,#50176,#50177,#50178,#50179,#50180,#50181,#50182,#50183,#50184,
#50185,#50186,#50187,#50188,#50189,#50190,#50191,#50192,#50193,#50194,#50195,
#50196,#50197,#50198,#50199,#50200,#50201,#50202,#50203,#50204,#50205,#50206,
#50207,#50208,#50209,#50210,#50211,#50212,#50213,#50214,#50215,#50216,#50217,
#50218,#50219,#50220,#50221,#50222,#50223,#50224,#50225),.UNSPECIFIED.,
 .F.,.F.,(4,3,3,3,3,3,3,3,3,3,3,3,3,3,3,3,3,3,3,3,3,3,3,3,3,3,4),(0.,0.0457810645246147,
0.0917889109041794,0.120317263742967,0.1428571428571,0.198222938253958,
0.253550313181452,0.275526169261383,0.2857142857143,0.349641017084231,0.413645125780723,
0.4285714285714,0.430597661234344,0.49617639314214,0.561795640410392,0.5714285714286,
0.585374712199986,0.649830213242843,0.7142857142857,0.740396105591031,0.795252697928882,
0.850177797878476,0.8571428571429,0.895765291931708,0.941863322899958,0.987754468934129,
0.999999797061789),.UNSPECIFIED.);
#832=B_SPLINE_CURVE_WITH_KNOTS('',3,(#50261,#50262,#50263,#50264,#50265,
#50266,#50267,#50268,#50269,#50270,#50271,#50272,#50273,#50274,#50275,#50276,
#50277,#50278,#50279,#50280,#50281,#50282,#50283,#50284,#50285,#50286,#50287,
#50288,#50289,#50290,#50291,#50292,#50293,#50294,#50295,#50296,#50297,#50298,
#50299,#50300,#50301,#50302,#50303,#50304,#50305,#50306,#50307,#50308,#50309,
#50310,#50311,#50312,#50313,#50314,#50315,#50316,#50317,#50318,#50319,#50320,
#50321),.UNSPECIFIED.,.F.,.F.,(4,3,3,3,3,3,3,3,3,3,3,3,3,3,3,3,3,3,3,3,
4),(4.8303250918634E-11,0.100941512885383,0.175470756442692,0.239253174153164,
0.25,0.301331842025548,0.350998881519161,0.399809175346533,0.449904587673267,
0.49727836962675,0.5,0.500001745528387,0.547462517145405,0.595562092315673,
0.644827784964439,0.69741389248222,0.75,0.813347997687032,0.88965388098933,
0.988070502192274,0.999999999949836),.UNSPECIFIED.);
#833=B_SPLINE_CURVE_WITH_KNOTS('',3,(#50374,#50375,#50376,#50377,#50378,
#50379,#50380,#50381,#50382,#50383,#50384,#50385,#50386,#50387,#50388,#50389,
#50390,#50391,#50392,#50393,#50394,#50395,#50396,#50397,#50398,#50399,#50400,
#50401,#50402,#50403,#50404,#50405,#50406,#50407,#50408,#50409,#50410,#50411,
#50412,#50413,#50414,#50415,#50416,#50417,#50418,#50419,#50420,#50421,#50422,
#50423,#50424,#50425,#50426,#50427,#50428,#50429,#50430,#50431,#50432,#50433,
#50434,#50435,#50436,#50437,#50438,#50439,#50440,#50441,#50442,#50443,#50444,
#50445,#50446,#50447,#50448,#50449,#50450,#50451,#50452,#50453,#50454,#50455,
#50456,#50457,#50458,#50459,#50460,#50461,#50462,#50463,#50464,#50465,#50466,
#50467,#50468,#50469,#50470,#50471,#50472,#50473,#50474,#50475,#50476,#50477,
#50478,#50479,#50480,#50481,#50482),.UNSPECIFIED.,.F.,.F.,(4,3,3,3,3,3,
3,3,3,3,3,3,3,3,3,3,3,3,3,3,3,3,3,3,3,3,3,3,3,3,3,3,3,3,3,3,4),(0.,0.0467928392075614,
0.106852595902104,0.12499999999999,0.158174590936753,0.187499999999985,
0.218749999999983,0.234374999999982,0.242187499999981,0.246093749999981,
0.248046874999981,0.249999999999981,0.272158913360276,0.328161519570208,
0.380022334667793,0.435536871025077,0.489384170464846,0.499978897694337,
0.499999999999984,0.552950484647908,0.607509892827094,0.619956343228664,
0.624999999999986,0.682568620262455,0.687499999999987,0.718749999999987,
0.727810778333793,0.734374999999988,0.742187499999988,0.746093749999988,
0.748046874999988,0.749999999999988,0.808696804403464,0.841783862121717,
0.90271961245407,0.953171011994076,1.),.UNSPECIFIED.);
#834=B_SPLINE_CURVE_WITH_KNOTS('',3,(#50494,#50495,#50496,#50497,#50498,
#50499,#50500),.UNSPECIFIED.,.F.,.F.,(4,3,4),(0.,0.5,1.),.UNSPECIFIED.);
#835=B_SPLINE_CURVE_WITH_KNOTS('',3,(#50503,#50504,#50505,#50506,#50507,
#50508,#50509,#50510,#50511,#50512,#50513,#50514,#50515,#50516,#50517,#50518,
#50519,#50520,#50521,#50522,#50523,#50524,#50525,#50526,#50527,#50528,#50529,
#50530,#50531,#50532,#50533,#50534,#50535,#50536,#50537,#50538,#50539,#50540,
#50541,#50542,#50543,#50544,#50545,#50546,#50547,#50548,#50549,#50550,#50551,
#50552,#50553,#50554,#50555,#50556,#50557,#50558,#50559,#50560,#50561,#50562,
#50563,#50564,#50565,#50566,#50567,#50568,#50569,#50570,#50571,#50572,#50573,
#50574,#50575,#50576,#50577,#50578,#50579,#50580,#50581,#50582,#50583,#50584,
#50585,#50586,#50587,#50588,#50589,#50590,#50591,#50592,#50593,#50594,#50595,
#50596),.UNSPECIFIED.,.F.,.F.,(4,3,3,3,3,3,3,3,3,3,3,3,3,3,3,3,3,3,3,3,
3,3,3,3,3,3,3,3,3,3,3,4),(0.,0.0582117372293125,0.11492486666494,0.125,
0.183308049049635,0.1875,0.207496971641933,0.21875,0.234375,0.2421875,0.24802262248796,
0.25,0.317558458591829,0.355181903648077,0.422153520719486,0.487812341416293,
0.500000000000002,0.500435668994842,0.564209449619831,0.625000000000003,
0.645724511137929,0.687500000000003,0.718750000000004,0.734375000000004,
0.742187500000004,0.748068593613938,0.750000000000004,0.793398748827164,
0.850370210729963,0.908819711975139,0.942690483272083,0.999999999999969),
 .UNSPECIFIED.);
#836=B_SPLINE_CURVE_WITH_KNOTS('',3,(#50667,#50668,#50669,#50670,#50671,
#50672,#50673,#50674,#50675,#50676,#50677,#50678,#50679),.UNSPECIFIED.,
 .F.,.F.,(4,3,3,3,4),(0.,0.0431918505795297,0.5,0.95680640941812,1.),
 .UNSPECIFIED.);
#837=B_SPLINE_CURVE_WITH_KNOTS('',3,(#50725,#50726,#50727,#50728,#50729,
#50730,#50731,#50732,#50733,#50734,#50735,#50736,#50737,#50738,#50739,#50740,
#50741,#50742,#50743,#50744,#50745,#50746,#50747,#50748,#50749,#50750,#50751,
#50752,#50753,#50754,#50755,#50756,#50757,#50758,#50759,#50760,#50761,#50762,
#50763,#50764,#50765,#50766,#50767,#50768,#50769,#50770,#50771,#50772,#50773,
#50774,#50775,#50776,#50777,#50778,#50779,#50780,#50781,#50782,#50783,#50784,
#50785,#50786,#50787,#50788,#50789,#50790,#50791,#50792,#50793,#50794,#50795,
#50796,#50797,#50798,#50799,#50800,#50801,#50802,#50803,#50804,#50805,#50806,
#50807,#50808,#50809,#50810,#50811,#50812,#50813,#50814,#50815,#50816,#50817,
#50818,#50819,#50820,#50821,#50822,#50823,#50824,#50825,#50826,#50827,#50828,
#50829,#50830,#50831,#50832,#50833,#50834,#50835,#50836,#50837,#50838,#50839,
#50840,#50841,#50842,#50843,#50844,#50845,#50846,#50847,#50848,#50849,#50850,
#50851,#50852,#50853,#50854,#50855,#50856,#50857,#50858,#50859,#50860,#50861,
#50862,#50863,#50864,#50865,#50866,#50867,#50868,#50869,#50870,#50871,#50872,
#50873,#50874,#50875,#50876,#50877,#50878,#50879,#50880,#50881,#50882,#50883,
#50884,#50885,#50886,#50887,#50888,#50889,#50890,#50891,#50892,#50893,#50894,
#50895,#50896,#50897,#50898,#50899,#50900,#50901,#50902,#50903,#50904,#50905,
#50906,#50907,#50908,#50909,#50910,#50911,#50912,#50913,#50914,#50915,#50916,
#50917,#50918,#50919,#50920,#50921,#50922,#50923,#50924,#50925,#50926,#50927,
#50928,#50929),.UNSPECIFIED.,.F.,.F.,(4,3,3,3,3,3,3,3,3,3,3,3,3,3,3,3,3,
3,3,3,3,3,3,3,3,3,3,3,3,3,3,3,3,3,3,3,3,3,3,3,3,3,3,3,3,3,3,3,3,3,3,3,3,
3,3,3,3,3,3,3,3,3,3,3,3,3,3,3,4),(0.,0.024995203988787,0.0499029973964458,
0.0680454794037188,0.0924338450081712,0.10788091381137,0.131553995326861,
0.140984707974704,0.163956800589375,0.171035558786358,0.193345860615578,
0.199615480348319,0.21875000000001,0.227604280505406,0.234375000000011,
0.242187500000011,0.246093750000011,0.248046875000011,0.249023437500011,
0.250000000000011,0.254582621996816,0.280004562969263,0.307433325257189,
0.309461091902956,0.337151591648368,0.344194252658166,0.372025449551419,
0.38494233403053,0.412589612231462,0.42986856233789,0.457864930665073,0.468750000000003,
0.477270445622972,0.484375000000002,0.492187500000002,0.496093750000002,
0.498046875000001,0.500000000000001,0.531323457773232,0.565671952248005,
0.578524989644827,0.613136937399731,0.616404235470285,0.648095328173456,
0.674911251480646,0.697968240642263,0.718048375575022,0.718749999999998,
0.734374999999997,0.735668182676169,0.742187499999997,0.746093749999997,
0.748046874999997,0.749023437499997,0.749999999999997,0.751820094994314,
0.773837783154619,0.79511929168836,0.815755175333351,0.83586282083153,0.855595767527349,
0.874999999999999,0.87515850402918,0.894772751664911,0.91458543277808,0.934770787977508,
0.955587724715017,0.97747470972438,0.999999988569063),.UNSPECIFIED.);
#838=B_SPLINE_CURVE_WITH_KNOTS('',3,(#51090,#51091,#51092,#51093,#51094,
#51095,#51096,#51097,#51098,#51099,#51100,#51101,#51102,#51103,#51104,#51105,
#51106,#51107,#51108,#51109,#51110,#51111,#51112,#51113,#51114,#51115,#51116,
#51117,#51118,#51119,#51120,#51121,#51122,#51123,#51124,#51125,#51126,#51127,
#51128,#51129,#51130,#51131,#51132,#51133,#51134,#51135,#51136,#51137,#51138,
#51139,#51140,#51141,#51142,#51143,#51144,#51145,#51146,#51147,#51148,#51149,
#51150,#51151,#51152,#51153,#51154,#51155,#51156,#51157,#51158,#51159,#51160,
#51161,#51162,#51163,#51164,#51165,#51166,#51167,#51168,#51169,#51170,#51171,
#51172,#51173,#51174,#51175,#51176,#51177,#51178,#51179,#51180,#51181,#51182,
#51183,#51184,#51185,#51186,#51187,#51188,#51189,#51190,#51191,#51192,#51193,
#51194,#51195,#51196,#51197,#51198,#51199,#51200,#51201,#51202,#51203,#51204,
#51205,#51206,#51207,#51208,#51209,#51210),.UNSPECIFIED.,.F.,.F.,(4,3,3,
3,3,3,3,3,3,3,3,3,3,3,3,3,3,3,3,3,3,3,3,3,3,3,3,3,3,3,3,3,3,3,3,3,3,3,3,
3,4),(7.98332290391144E-8,0.0312500598749225,0.0618422411603766,0.0934211205801896,
0.125000000000003,0.15556926580042,0.187159632900212,0.218750000000005,
0.234375000000005,0.242187500000005,0.246093750000005,0.248046875000005,
0.249023437500006,0.250000000000006,0.450377472834497,0.499981371599594,
0.500000000000035,0.625000000000049,0.687500000000057,0.71875000000006,
0.734375000000062,0.742187500000063,0.749511718750063,0.750000000000063,
0.765918986321078,0.781838150966254,0.79775750405352,0.813677169065249,
0.829597013916694,0.845517162064315,0.859375000000035,0.867187500000033,
0.871093750000032,0.873046875000031,0.874023437500031,0.875000000000031,
0.899836671865672,0.924877490179526,0.949727578183808,0.974863761652447,
0.999999945121086),.UNSPECIFIED.);
#839=B_SPLINE_CURVE_WITH_KNOTS('',3,(#51247,#51248,#51249,#51250,#51251,
#51252,#51253,#51254,#51255,#51256,#51257,#51258,#51259,#51260,#51261,#51262,
#51263,#51264,#51265,#51266,#51267,#51268,#51269,#51270,#51271,#51272,#51273,
#51274,#51275,#51276,#51277,#51278,#51279,#51280),.UNSPECIFIED.,.F.,.F.,
(4,3,3,3,3,3,3,3,3,3,3,4),(1.02990837813416E-11,0.133918786859822,0.21381289071477,
0.25,0.377666333223483,0.484760468447434,0.5,0.631307102429207,0.75,0.754458269127967,
0.879638408390619,0.999999987393856),.UNSPECIFIED.);
#840=B_SPLINE_CURVE_WITH_KNOTS('',3,(#51281,#51282,#51283,#51284,#51285,
#51286,#51287,#51288,#51289,#51290,#51291,#51292,#51293,#51294,#51295,#51296,
#51297,#51298,#51299,#51300,#51301,#51302,#51303,#51304,#51305,#51306,#51307,
#51308,#51309,#51310,#51311,#51312,#51313,#51314,#51315,#51316,#51317,#51318,
#51319,#51320,#51321,#51322,#51323,#51324,#51325,#51326,#51327,#51328,#51329,
#51330,#51331,#51332,#51333,#51334,#51335,#51336,#51337,#51338,#51339,#51340,
#51341),.UNSPECIFIED.,.F.,.F.,(4,3,3,3,3,3,3,3,3,3,3,3,3,3,3,3,3,3,3,3,
4),(7.31797006928123E-11,0.100715529220303,0.175357764610152,0.238678478425238,
0.25,0.301434000969269,0.351119460711998,0.400021887779728,0.450010943889864,
0.497472186324765,0.5,0.500001800462764,0.54755125219235,0.598163439144263,
0.647566149279604,0.698783074639802,0.75,0.81286007931633,0.88802726687967,
0.987428003542778,0.999999999992996),.UNSPECIFIED.);
#841=B_SPLINE_CURVE_WITH_KNOTS('',3,(#51424,#51425,#51426,#51427,#51428,
#51429,#51430,#51431,#51432,#51433,#51434,#51435,#51436,#51437,#51438,#51439,
#51440,#51441,#51442,#51443,#51444,#51445,#51446,#51447,#51448,#51449,#51450,
#51451,#51452,#51453,#51454,#51455,#51456,#51457,#51458,#51459,#51460,#51461,
#51462,#51463,#51464,#51465,#51466,#51467,#51468,#51469,#51470,#51471,#51472),
 .UNSPECIFIED.,.F.,.F.,(4,3,3,3,3,3,3,3,3,3,3,3,3,3,3,3,4),(0.,0.0772490783748716,
0.125628580660424,0.206837347558675,0.250000000000001,0.333280273269906,
0.368977328446765,0.374999999999999,0.423220960550615,0.471880842368208,
0.499999999999997,0.601986585180624,0.703425665210588,0.731721858235954,
0.83332819110189,0.936212051837402,1.),.UNSPECIFIED.);
#842=B_SPLINE_CURVE_WITH_KNOTS('',3,(#51473,#51474,#51475,#51476,#51477,
#51478,#51479,#51480,#51481,#51482,#51483,#51484,#51485,#51486,#51487,#51488,
#51489,#51490,#51491,#51492,#51493,#51494,#51495,#51496,#51497,#51498,#51499,
#51500,#51501,#51502,#51503,#51504,#51505,#51506,#51507,#51508,#51509,#51510,
#51511,#51512,#51513,#51514,#51515,#51516,#51517,#51518,#51519,#51520,#51521,
#51522,#51523,#51524),.UNSPECIFIED.,.F.,.F.,(4,3,3,3,3,3,3,3,3,3,3,3,3,
3,3,3,3,4),(0.,0.0673552999085671,0.136367280704923,0.208456935206561,0.250000000000025,
0.329907800933807,0.375000000000035,0.437500000000039,0.468750000000042,
0.484375000000041,0.495400419983993,0.50000000000004,0.586602629559447,
0.675549917512404,0.768876331728931,0.865001499097696,0.965889321645426,
1.),.UNSPECIFIED.);
#843=B_SPLINE_CURVE_WITH_KNOTS('',3,(#51565,#51566,#51567,#51568,#51569,
#51570,#51571,#51572,#51573,#51574,#51575,#51576,#51577,#51578,#51579,#51580,
#51581,#51582,#51583,#51584,#51585,#51586,#51587,#51588,#51589,#51590,#51591,
#51592,#51593,#51594,#51595,#51596,#51597,#51598,#51599,#51600,#51601,#51602,
#51603,#51604,#51605,#51606,#51607,#51608,#51609,#51610,#51611,#51612,#51613,
#51614,#51615,#51616,#51617,#51618,#51619,#51620,#51621,#51622,#51623,#51624,
#51625,#51626,#51627,#51628,#51629,#51630,#51631,#51632,#51633,#51634,#51635,
#51636,#51637,#51638,#51639,#51640,#51641,#51642,#51643),.UNSPECIFIED.,
 .F.,.F.,(4,3,3,3,3,3,3,3,3,3,3,3,3,3,3,3,3,3,3,3,3,3,3,3,3,3,4),(0.,0.0457033068802993,
0.0916137398494609,0.120395916002719,0.1428571428571,0.19727492470639,0.251652801985863,
0.275597882536144,0.2857142857143,0.349092790520194,0.412555793048888,0.4285714285714,
0.430653365734671,0.4960636773585,0.561515650793809,0.5714285714286,0.585415002992912,
0.649850358639306,0.7142857142857,0.740421620406485,0.795269363043043,0.850185630861512,
0.8571428571429,0.895775606041297,0.941868794237302,0.987755080875803,0.999999797081952),
 .UNSPECIFIED.);
#879=SHAPE_REPRESENTATION_RELATIONSHIP('SRR','None',#57267,#908);
#908=ADVANCED_BREP_SHAPE_REPRESENTATION('',(#976),#57059);
#939=STYLED_ITEM('',(#57444),#976);
#976=MANIFOLD_SOLID_BREP('Body1',#24539);
#1130=FACE_BOUND('',#4115,.T.);
#1131=FACE_BOUND('',#4116,.T.);
#1132=FACE_BOUND('',#4117,.T.);
#1133=FACE_BOUND('',#4118,.T.);
#1134=FACE_BOUND('',#4131,.T.);
#1135=FACE_BOUND('',#4132,.T.);
#1136=FACE_BOUND('',#4133,.T.);
#1137=FACE_BOUND('',#4134,.T.);
#1533=PLANE('',#25471);
#1534=PLANE('',#25478);
#1535=PLANE('',#25624);
#1536=PLANE('',#25628);
#1537=PLANE('',#25632);
#1538=PLANE('',#25635);
#1539=PLANE('',#25639);
#1540=PLANE('',#25643);
#2475=FACE_OUTER_BOUND('',#3980,.T.);
#2476=FACE_OUTER_BOUND('',#3981,.T.);
#2477=FACE_OUTER_BOUND('',#3982,.T.);
#2478=FACE_OUTER_BOUND('',#3983,.T.);
#2479=FACE_OUTER_BOUND('',#3984,.T.);
#2480=FACE_OUTER_BOUND('',#3985,.T.);
#2481=FACE_OUTER_BOUND('',#3986,.T.);
#2482=FACE_OUTER_BOUND('',#3987,.T.);
#2483=FACE_OUTER_BOUND('',#3988,.T.);
#2484=FACE_OUTER_BOUND('',#3989,.T.);
#2485=FACE_OUTER_BOUND('',#3990,.T.);
#2486=FACE_OUTER_BOUND('',#3991,.T.);
#2487=FACE_OUTER_BOUND('',#3992,.T.);
#2488=FACE_OUTER_BOUND('',#3993,.T.);
#2489=FACE_OUTER_BOUND('',#3994,.T.);
#2490=FACE_OUTER_BOUND('',#3995,.T.);
#2491=FACE_OUTER_BOUND('',#3996,.T.);
#2492=FACE_OUTER_BOUND('',#3997,.T.);
#2493=FACE_OUTER_BOUND('',#3998,.T.);
#2494=FACE_OUTER_BOUND('',#3999,.T.);
#2495=FACE_OUTER_BOUND('',#4000,.T.);
#2496=FACE_OUTER_BOUND('',#4001,.T.);
#2497=FACE_OUTER_BOUND('',#4002,.T.);
#2498=FACE_OUTER_BOUND('',#4003,.T.);
#2499=FACE_OUTER_BOUND('',#4004,.T.);
#2500=FACE_OUTER_BOUND('',#4005,.T.);
#2501=FACE_OUTER_BOUND('',#4006,.T.);
#2502=FACE_OUTER_BOUND('',#4007,.T.);
#2503=FACE_OUTER_BOUND('',#4008,.T.);
#2504=FACE_OUTER_BOUND('',#4009,.T.);
#2505=FACE_OUTER_BOUND('',#4010,.T.);
#2506=FACE_OUTER_BOUND('',#4011,.T.);
#2507=FACE_OUTER_BOUND('',#4012,.T.);
#2508=FACE_OUTER_BOUND('',#4013,.T.);
#2509=FACE_OUTER_BOUND('',#4014,.T.);
#2510=FACE_OUTER_BOUND('',#4015,.T.);
#2511=FACE_OUTER_BOUND('',#4016,.T.);
#2512=FACE_OUTER_BOUND('',#4017,.T.);
#2513=FACE_OUTER_BOUND('',#4018,.T.);
#2514=FACE_OUTER_BOUND('',#4019,.T.);
#2515=FACE_OUTER_BOUND('',#4020,.T.);
#2516=FACE_OUTER_BOUND('',#4021,.T.);
#2517=FACE_OUTER_BOUND('',#4022,.T.);
#2518=FACE_OUTER_BOUND('',#4023,.T.);
#2519=FACE_OUTER_BOUND('',#4024,.T.);
#2520=FACE_OUTER_BOUND('',#4025,.T.);
#2521=FACE_OUTER_BOUND('',#4026,.T.);
#2522=FACE_OUTER_BOUND('',#4027,.T.);
#2523=FACE_OUTER_BOUND('',#4028,.T.);
#2524=FACE_OUTER_BOUND('',#4029,.T.);
#2525=FACE_OUTER_BOUND('',#4030,.T.);
#2526=FACE_OUTER_BOUND('',#4031,.T.);
#2527=FACE_OUTER_BOUND('',#4032,.T.);
#2528=FACE_OUTER_BOUND('',#4033,.T.);
#2529=FACE_OUTER_BOUND('',#4034,.T.);
#2530=FACE_OUTER_BOUND('',#4035,.T.);
#2531=FACE_OUTER_BOUND('',#4036,.T.);
#2532=FACE_OUTER_BOUND('',#4037,.T.);
#2533=FACE_OUTER_BOUND('',#4038,.T.);
#2534=FACE_OUTER_BOUND('',#4039,.T.);
#2535=FACE_OUTER_BOUND('',#4040,.T.);
#2536=FACE_OUTER_BOUND('',#4041,.T.);
#2537=FACE_OUTER_BOUND('',#4042,.T.);
#2538=FACE_OUTER_BOUND('',#4043,.T.);
#2539=FACE_OUTER_BOUND('',#4044,.T.);
#2540=FACE_OUTER_BOUND('',#4045,.T.);
#2541=FACE_OUTER_BOUND('',#4046,.T.);
#2542=FACE_OUTER_BOUND('',#4047,.T.);
#2543=FACE_OUTER_BOUND('',#4048,.T.);
#2544=FACE_OUTER_BOUND('',#4049,.T.);
#2545=FACE_OUTER_BOUND('',#4050,.T.);
#2546=FACE_OUTER_BOUND('',#4051,.T.);
#2547=FACE_OUTER_BOUND('',#4052,.T.);
#2548=FACE_OUTER_BOUND('',#4053,.T.);
#2549=FACE_OUTER_BOUND('',#4054,.T.);
#2550=FACE_OUTER_BOUND('',#4055,.T.);
#2551=FACE_OUTER_BOUND('',#4056,.T.);
#2552=FACE_OUTER_BOUND('',#4057,.T.);
#2553=FACE_OUTER_BOUND('',#4058,.T.);
#2554=FACE_OUTER_BOUND('',#4059,.T.);
#2555=FACE_OUTER_BOUND('',#4060,.T.);
#2556=FACE_OUTER_BOUND('',#4061,.T.);
#2557=FACE_OUTER_BOUND('',#4062,.T.);
#2558=FACE_OUTER_BOUND('',#4063,.T.);
#2559=FACE_OUTER_BOUND('',#4064,.T.);
#2560=FACE_OUTER_BOUND('',#4065,.T.);
#2561=FACE_OUTER_BOUND('',#4066,.T.);
#2562=FACE_OUTER_BOUND('',#4067,.T.);
#2563=FACE_OUTER_BOUND('',#4068,.T.);
#2564=FACE_OUTER_BOUND('',#4069,.T.);
#2565=FACE_OUTER_BOUND('',#4070,.T.);
#2566=FACE_OUTER_BOUND('',#4071,.T.);
#2567=FACE_OUTER_BOUND('',#4072,.T.);
#2568=FACE_OUTER_BOUND('',#4073,.T.);
#2569=FACE_OUTER_BOUND('',#4074,.T.);
#2570=FACE_OUTER_BOUND('',#4075,.T.);
#2571=FACE_OUTER_BOUND('',#4076,.T.);
#2572=FACE_OUTER_BOUND('',#4077,.T.);
#2573=FACE_OUTER_BOUND('',#4078,.T.);
#2574=FACE_OUTER_BOUND('',#4079,.T.);
#2575=FACE_OUTER_BOUND('',#4080,.T.);
#2576=FACE_OUTER_BOUND('',#4081,.T.);
#2577=FACE_OUTER_BOUND('',#4082,.T.);
#2578=FACE_OUTER_BOUND('',#4083,.T.);
#2579=FACE_OUTER_BOUND('',#4084,.T.);
#2580=FACE_OUTER_BOUND('',#4085,.T.);
#2581=FACE_OUTER_BOUND('',#4086,.T.);
#2582=FACE_OUTER_BOUND('',#4087,.T.);
#2583=FACE_OUTER_BOUND('',#4088,.T.);
#2584=FACE_OUTER_BOUND('',#4089,.T.);
#2585=FACE_OUTER_BOUND('',#4090,.T.);
#2586=FACE_OUTER_BOUND('',#4091,.T.);
#2587=FACE_OUTER_BOUND('',#4092,.T.);
#2588=FACE_OUTER_BOUND('',#4093,.T.);
#2589=FACE_OUTER_BOUND('',#4094,.T.);
#2590=FACE_OUTER_BOUND('',#4095,.T.);
#2591=FACE_OUTER_BOUND('',#4096,.T.);
#2592=FACE_OUTER_BOUND('',#4097,.T.);
#2593=FACE_OUTER_BOUND('',#4098,.T.);
#2594=FACE_OUTER_BOUND('',#4099,.T.);
#2595=FACE_OUTER_BOUND('',#4100,.T.);
#2596=FACE_OUTER_BOUND('',#4101,.T.);
#2597=FACE_OUTER_BOUND('',#4102,.T.);
#2598=FACE_OUTER_BOUND('',#4103,.T.);
#2599=FACE_OUTER_BOUND('',#4104,.T.);
#2600=FACE_OUTER_BOUND('',#4105,.T.);
#2601=FACE_OUTER_BOUND('',#4106,.T.);
#2602=FACE_OUTER_BOUND('',#4107,.T.);
#2603=FACE_OUTER_BOUND('',#4108,.T.);
#2604=FACE_OUTER_BOUND('',#4109,.T.);
#2605=FACE_OUTER_BOUND('',#4110,.T.);
#2606=FACE_OUTER_BOUND('',#4111,.T.);
#2607=FACE_OUTER_BOUND('',#4112,.T.);
#2608=FACE_OUTER_BOUND('',#4113,.T.);
#2609=FACE_OUTER_BOUND('',#4114,.T.);
#2610=FACE_OUTER_BOUND('',#4119,.T.);
#2611=FACE_OUTER_BOUND('',#4120,.T.);
#2612=FACE_OUTER_BOUND('',#4121,.T.);
#2613=FACE_OUTER_BOUND('',#4122,.T.);
#2614=FACE_OUTER_BOUND('',#4123,.T.);
#2615=FACE_OUTER_BOUND('',#4124,.T.);
#2616=FACE_OUTER_BOUND('',#4125,.T.);
#2617=FACE_OUTER_BOUND('',#4126,.T.);
#2618=FACE_OUTER_BOUND('',#4127,.T.);
#2619=FACE_OUTER_BOUND('',#4128,.T.);
#2620=FACE_OUTER_BOUND('',#4129,.T.);
#2621=FACE_OUTER_BOUND('',#4130,.T.);
#3980=EDGE_LOOP('',(#17360));
#3981=EDGE_LOOP('',(#17361,#17362,#17363,#17364));
#3982=EDGE_LOOP('',(#17365,#17366,#17367,#17368));
#3983=EDGE_LOOP('',(#17369));
#3984=EDGE_LOOP('',(#17370,#17371,#17372,#17373));
#3985=EDGE_LOOP('',(#17374,#17375,#17376));
#3986=EDGE_LOOP('',(#17377,#17378,#17379,#17380));
#3987=EDGE_LOOP('',(#17381,#17382,#17383,#17384));
#3988=EDGE_LOOP('',(#17385,#17386,#17387,#17388));
#3989=EDGE_LOOP('',(#17389,#17390,#17391,#17392));
#3990=EDGE_LOOP('',(#17393,#17394,#17395,#17396));
#3991=EDGE_LOOP('',(#17397,#17398,#17399));
#3992=EDGE_LOOP('',(#17400,#17401,#17402,#17403));
#3993=EDGE_LOOP('',(#17404,#17405,#17406,#17407));
#3994=EDGE_LOOP('',(#17408,#17409,#17410,#17411));
#3995=EDGE_LOOP('',(#17412,#17413,#17414,#17415));
#3996=EDGE_LOOP('',(#17416,#17417,#17418,#17419));
#3997=EDGE_LOOP('',(#17420,#17421,#17422));
#3998=EDGE_LOOP('',(#17423,#17424,#17425,#17426));
#3999=EDGE_LOOP('',(#17427,#17428,#17429,#17430));
#4000=EDGE_LOOP('',(#17431,#17432,#17433));
#4001=EDGE_LOOP('',(#17434,#17435,#17436,#17437));
#4002=EDGE_LOOP('',(#17438,#17439,#17440,#17441));
#4003=EDGE_LOOP('',(#17442,#17443,#17444,#17445));
#4004=EDGE_LOOP('',(#17446,#17447,#17448));
#4005=EDGE_LOOP('',(#17449,#17450,#17451,#17452));
#4006=EDGE_LOOP('',(#17453,#17454,#17455,#17456));
#4007=EDGE_LOOP('',(#17457,#17458,#17459,#17460));
#4008=EDGE_LOOP('',(#17461,#17462,#17463,#17464));
#4009=EDGE_LOOP('',(#17465,#17466,#17467,#17468));
#4010=EDGE_LOOP('',(#17469,#17470,#17471,#17472));
#4011=EDGE_LOOP('',(#17473,#17474,#17475,#17476));
#4012=EDGE_LOOP('',(#17477,#17478,#17479));
#4013=EDGE_LOOP('',(#17480,#17481,#17482,#17483));
#4014=EDGE_LOOP('',(#17484,#17485,#17486,#17487));
#4015=EDGE_LOOP('',(#17488,#17489,#17490,#17491));
#4016=EDGE_LOOP('',(#17492,#17493,#17494,#17495));
#4017=EDGE_LOOP('',(#17496,#17497,#17498,#17499));
#4018=EDGE_LOOP('',(#17500,#17501,#17502));
#4019=EDGE_LOOP('',(#17503,#17504,#17505,#17506));
#4020=EDGE_LOOP('',(#17507,#17508,#17509,#17510));
#4021=EDGE_LOOP('',(#17511,#17512,#17513));
#4022=EDGE_LOOP('',(#17514,#17515,#17516,#17517));
#4023=EDGE_LOOP('',(#17518,#17519,#17520,#17521));
#4024=EDGE_LOOP('',(#17522,#17523,#17524,#17525));
#4025=EDGE_LOOP('',(#17526,#17527,#17528));
#4026=EDGE_LOOP('',(#17529,#17530,#17531,#17532));
#4027=EDGE_LOOP('',(#17533,#17534,#17535,#17536));
#4028=EDGE_LOOP('',(#17537,#17538,#17539,#17540));
#4029=EDGE_LOOP('',(#17541,#17542,#17543,#17544));
#4030=EDGE_LOOP('',(#17545,#17546,#17547,#17548));
#4031=EDGE_LOOP('',(#17549,#17550,#17551,#17552));
#4032=EDGE_LOOP('',(#17553,#17554,#17555,#17556));
#4033=EDGE_LOOP('',(#17557,#17558,#17559));
#4034=EDGE_LOOP('',(#17560,#17561,#17562,#17563));
#4035=EDGE_LOOP('',(#17564,#17565,#17566,#17567));
#4036=EDGE_LOOP('',(#17568,#17569,#17570,#17571));
#4037=EDGE_LOOP('',(#17572,#17573,#17574,#17575));
#4038=EDGE_LOOP('',(#17576,#17577,#17578,#17579));
#4039=EDGE_LOOP('',(#17580,#17581,#17582));
#4040=EDGE_LOOP('',(#17583,#17584,#17585,#17586));
#4041=EDGE_LOOP('',(#17587,#17588,#17589,#17590));
#4042=EDGE_LOOP('',(#17591,#17592,#17593));
#4043=EDGE_LOOP('',(#17594,#17595,#17596,#17597));
#4044=EDGE_LOOP('',(#17598,#17599,#17600,#17601));
#4045=EDGE_LOOP('',(#17602,#17603,#17604,#17605));
#4046=EDGE_LOOP('',(#17606,#17607,#17608));
#4047=EDGE_LOOP('',(#17609,#17610,#17611,#17612));
#4048=EDGE_LOOP('',(#17613,#17614,#17615,#17616));
#4049=EDGE_LOOP('',(#17617,#17618,#17619,#17620));
#4050=EDGE_LOOP('',(#17621,#17622,#17623,#17624));
#4051=EDGE_LOOP('',(#17625,#17626,#17627,#17628));
#4052=EDGE_LOOP('',(#17629,#17630,#17631,#17632));
#4053=EDGE_LOOP('',(#17633,#17634,#17635,#17636));
#4054=EDGE_LOOP('',(#17637,#17638,#17639));
#4055=EDGE_LOOP('',(#17640,#17641,#17642,#17643));
#4056=EDGE_LOOP('',(#17644,#17645,#17646,#17647));
#4057=EDGE_LOOP('',(#17648,#17649,#17650,#17651));
#4058=EDGE_LOOP('',(#17652,#17653,#17654,#17655));
#4059=EDGE_LOOP('',(#17656,#17657,#17658,#17659));
#4060=EDGE_LOOP('',(#17660,#17661,#17662));
#4061=EDGE_LOOP('',(#17663,#17664,#17665,#17666));
#4062=EDGE_LOOP('',(#17667,#17668,#17669,#17670));
#4063=EDGE_LOOP('',(#17671,#17672,#17673));
#4064=EDGE_LOOP('',(#17674,#17675,#17676,#17677));
#4065=EDGE_LOOP('',(#17678,#17679,#17680,#17681));
#4066=EDGE_LOOP('',(#17682,#17683,#17684,#17685));
#4067=EDGE_LOOP('',(#17686,#17687,#17688));
#4068=EDGE_LOOP('',(#17689,#17690,#17691,#17692));
#4069=EDGE_LOOP('',(#17693,#17694,#17695,#17696));
#4070=EDGE_LOOP('',(#17697,#17698,#17699,#17700));
#4071=EDGE_LOOP('',(#17701,#17702,#17703,#17704));
#4072=EDGE_LOOP('',(#17705,#17706,#17707));
#4073=EDGE_LOOP('',(#17708,#17709,#17710,#17711));
#4074=EDGE_LOOP('',(#17712,#17713,#17714));
#4075=EDGE_LOOP('',(#17715,#17716,#17717,#17718));
#4076=EDGE_LOOP('',(#17719,#17720,#17721,#17722));
#4077=EDGE_LOOP('',(#17723,#17724,#17725,#17726));
#4078=EDGE_LOOP('',(#17727,#17728,#17729,#17730));
#4079=EDGE_LOOP('',(#17731,#17732,#17733,#17734));
#4080=EDGE_LOOP('',(#17735,#17736,#17737));
#4081=EDGE_LOOP('',(#17738,#17739,#17740,#17741));
#4082=EDGE_LOOP('',(#17742,#17743,#17744,#17745));
#4083=EDGE_LOOP('',(#17746,#17747,#17748,#17749));
#4084=EDGE_LOOP('',(#17750,#17751,#17752,#17753));
#4085=EDGE_LOOP('',(#17754,#17755,#17756,#17757));
#4086=EDGE_LOOP('',(#17758,#17759,#17760));
#4087=EDGE_LOOP('',(#17761,#17762,#17763,#17764));
#4088=EDGE_LOOP('',(#17765,#17766,#17767,#17768));
#4089=EDGE_LOOP('',(#17769,#17770,#17771,#17772));
#4090=EDGE_LOOP('',(#17773,#17774,#17775,#17776));
#4091=EDGE_LOOP('',(#17777,#17778,#17779,#17780));
#4092=EDGE_LOOP('',(#17781,#17782,#17783));
#4093=EDGE_LOOP('',(#17784,#17785,#17786,#17787));
#4094=EDGE_LOOP('',(#17788,#17789,#17790,#17791));
#4095=EDGE_LOOP('',(#17792,#17793,#17794));
#4096=EDGE_LOOP('',(#17795,#17796,#17797,#17798));
#4097=EDGE_LOOP('',(#17799,#17800,#17801,#17802));
#4098=EDGE_LOOP('',(#17803,#17804,#17805,#17806));
#4099=EDGE_LOOP('',(#17807,#17808,#17809));
#4100=EDGE_LOOP('',(#17810,#17811,#17812,#17813));
#4101=EDGE_LOOP('',(#17814,#17815,#17816,#17817));
#4102=EDGE_LOOP('',(#17818,#17819,#17820,#17821));
#4103=EDGE_LOOP('',(#17822,#17823,#17824,#17825));
#4104=EDGE_LOOP('',(#17826,#17827,#17828,#17829,#17830,#17831,#17832,#17833));
#4105=EDGE_LOOP('',(#17834,#17835,#17836,#17837,#17838,#17839,#17840,#17841));
#4106=EDGE_LOOP('',(#17842,#17843,#17844,#17845,#17846,#17847,#17848,#17849));
#4107=EDGE_LOOP('',(#17850,#17851,#17852,#17853,#17854,#17855,#17856,#17857));
#4108=EDGE_LOOP('',(#17858,#17859,#17860,#17861,#17862,#17863,#17864,#17865));
#4109=EDGE_LOOP('',(#17866,#17867,#17868,#17869,#17870,#17871,#17872,#17873));
#4110=EDGE_LOOP('',(#17874));
#4111=EDGE_LOOP('',(#17875,#17876,#17877,#17878));
#4112=EDGE_LOOP('',(#17879));
#4113=EDGE_LOOP('',(#17880,#17881,#17882,#17883));
#4114=EDGE_LOOP('',(#17884,#17885,#17886,#17887,#17888,#17889,#17890,#17891,
#17892,#17893,#17894,#17895,#17896,#17897,#17898,#17899,#17900,#17901,#17902,
#17903,#17904,#17905,#17906,#17907,#17908,#17909,#17910,#17911,#17912,#17913,
#17914,#17915,#17916,#17917,#17918,#17919));
#4115=EDGE_LOOP('',(#17920));
#4116=EDGE_LOOP('',(#17921));
#4117=EDGE_LOOP('',(#17922));
#4118=EDGE_LOOP('',(#17923));
#4119=EDGE_LOOP('',(#17924,#17925,#17926,#17927));
#4120=EDGE_LOOP('',(#17928,#17929,#17930,#17931));
#4121=EDGE_LOOP('',(#17932,#17933,#17934,#17935));
#4122=EDGE_LOOP('',(#17936,#17937,#17938,#17939));
#4123=EDGE_LOOP('',(#17940,#17941,#17942,#17943));
#4124=EDGE_LOOP('',(#17944,#17945,#17946,#17947));
#4125=EDGE_LOOP('',(#17948,#17949,#17950,#17951));
#4126=EDGE_LOOP('',(#17952));
#4127=EDGE_LOOP('',(#17953,#17954,#17955,#17956));
#4128=EDGE_LOOP('',(#17957));
#4129=EDGE_LOOP('',(#17958,#17959,#17960,#17961));
#4130=EDGE_LOOP('',(#17962,#17963,#17964,#17965,#17966,#17967,#17968,#17969,
#17970,#17971,#17972,#17973,#17974,#17975,#17976,#17977,#17978,#17979,#17980,
#17981,#17982,#17983,#17984,#17985,#17986,#17987,#17988,#17989,#17990,#17991,
#17992,#17993,#17994,#17995,#17996,#17997));
#4131=EDGE_LOOP('',(#17998));
#4132=EDGE_LOOP('',(#17999));
#4133=EDGE_LOOP('',(#18000));
#4134=EDGE_LOOP('',(#18001));
#5713=LINE('',#36401,#7680);
#5714=LINE('',#36407,#7681);
#5715=LINE('',#36415,#7682);
#5716=LINE('',#50658,#7683);
#5717=LINE('',#50665,#7684);
#5718=LINE('',#51649,#7685);
#5719=LINE('',#51656,#7686);
#7680=VECTOR('',#29121,1.5);
#7681=VECTOR('',#29128,9.);
#7682=VECTOR('',#29139,1.5);
#7683=VECTOR('',#29432,1.5);
#7684=VECTOR('',#29441,1.5);
#7685=VECTOR('',#29454,1.5);
#7686=VECTOR('',#29463,1.5);
#9430=CIRCLE('',#25472,1.5);
#9431=CIRCLE('',#25474,1.5);
#9432=CIRCLE('',#25476,9.);
#9433=CIRCLE('',#25477,9.);
#9434=CIRCLE('',#25479,1.5);
#9435=CIRCLE('',#25481,1.5);
#9436=CIRCLE('',#25483,0.400000000003301);
#9437=CIRCLE('',#25484,0.400018246612719);
#9438=CIRCLE('',#25485,0.4000000000033);
#9439=CIRCLE('',#25486,0.499983844668534);
#9440=CIRCLE('',#25487,0.499989222937552);
#9441=CIRCLE('',#25488,0.4);
#9442=CIRCLE('',#25489,0.4000000000004);
#9443=CIRCLE('',#25491,0.399999999999999);
#9444=CIRCLE('',#25493,0.399999999950399);
#9445=CIRCLE('',#25494,0.400000000003299);
#9446=CIRCLE('',#25495,0.50000942462105);
#9447=CIRCLE('',#25496,0.400018241496959);
#9448=CIRCLE('',#25498,0.4000000000033);
#9449=CIRCLE('',#25499,0.499988527203264);
#9450=CIRCLE('',#25500,0.400018246602581);
#9451=CIRCLE('',#25502,0.4000000000033);
#9452=CIRCLE('',#25503,0.4000000000033);
#9453=CIRCLE('',#25505,0.4000000000004);
#9454=CIRCLE('',#25507,0.40002572214466);
#9455=CIRCLE('',#25508,0.500009686373483);
#9456=CIRCLE('',#25509,0.49998900112587);
#9457=CIRCLE('',#25510,0.4);
#9458=CIRCLE('',#25511,0.4000000000004);
#9459=CIRCLE('',#25513,0.4);
#9460=CIRCLE('',#25515,0.3999999999504);
#9461=CIRCLE('',#25516,0.4000000000033);
#9462=CIRCLE('',#25517,0.500010213165878);
#9463=CIRCLE('',#25518,0.400018241494099);
#9464=CIRCLE('',#25520,0.4000000000033);
#9465=CIRCLE('',#25521,0.499988839014698);
#9466=CIRCLE('',#25522,0.400018246604447);
#9467=CIRCLE('',#25524,0.400000000003301);
#9468=CIRCLE('',#25525,0.400000000003301);
#9469=CIRCLE('',#25527,0.400000000000399);
#9470=CIRCLE('',#25529,0.400025722143921);
#9471=CIRCLE('',#25530,0.500008606842085);
#9472=CIRCLE('',#25531,0.499984919866047);
#9473=CIRCLE('',#25532,0.4);
#9474=CIRCLE('',#25533,0.4000000000004);
#9475=CIRCLE('',#25535,0.4);
#9476=CIRCLE('',#25537,0.3999999999504);
#9477=CIRCLE('',#25538,0.400000000003302);
#9478=CIRCLE('',#25539,0.500022426641145);
#9479=CIRCLE('',#25540,0.400018241484847);
#9480=CIRCLE('',#25542,0.4000000000033);
#9481=CIRCLE('',#25543,0.499988763335309);
#9482=CIRCLE('',#25544,0.400018246619586);
#9483=CIRCLE('',#25546,0.400000000003301);
#9484=CIRCLE('',#25547,0.4000000000033);
#9485=CIRCLE('',#25549,0.400000000000401);
#9486=CIRCLE('',#25551,0.400025722154133);
#9487=CIRCLE('',#25552,0.500008887107232);
#9488=CIRCLE('',#25553,0.499989277844728);
#9489=CIRCLE('',#25554,0.4);
#9490=CIRCLE('',#25555,0.4000000000004);
#9491=CIRCLE('',#25557,0.399999999999999);
#9492=CIRCLE('',#25559,0.3999999999504);
#9493=CIRCLE('',#25560,0.400000000003299);
#9494=CIRCLE('',#25561,0.500008216044762);
#9495=CIRCLE('',#25562,0.400018241439198);
#9496=CIRCLE('',#25564,0.4000000000033);
#9497=CIRCLE('',#25565,0.499982708615474);
#9498=CIRCLE('',#25566,0.400018246543346);
#9499=CIRCLE('',#25568,0.4000000000033);
#9500=CIRCLE('',#25569,0.4000000000033);
#9501=CIRCLE('',#25571,0.400000000000399);
#9502=CIRCLE('',#25573,0.400025722215534);
#9503=CIRCLE('',#25574,0.500011264103594);
#9504=CIRCLE('',#25576,0.4000000000003);
#9505=CIRCLE('',#25577,0.400025722150869);
#9506=CIRCLE('',#25578,0.4000000000003);
#9507=CIRCLE('',#25580,0.4);
#9508=CIRCLE('',#25582,0.4);
#9509=CIRCLE('',#25583,0.399999999950402);
#9510=CIRCLE('',#25584,0.499989175301816);
#9511=CIRCLE('',#25585,0.500009622535219);
#9512=CIRCLE('',#25586,0.400000000003302);
#9513=CIRCLE('',#25588,0.4000000000033);
#9514=CIRCLE('',#25589,0.400018241481554);
#9515=CIRCLE('',#25590,0.499988814391298);
#9516=CIRCLE('',#25591,0.4);
#9517=CIRCLE('',#25592,0.4000000000004);
#9518=CIRCLE('',#25594,0.4);
#9519=CIRCLE('',#25596,0.3999999999504);
#9520=CIRCLE('',#25597,0.400000000003299);
#9521=CIRCLE('',#25598,0.500009986819179);
#9522=CIRCLE('',#25599,0.400018241441403);
#9523=CIRCLE('',#25601,0.4000000000033);
#9524=CIRCLE('',#25602,0.499988313792213);
#9525=CIRCLE('',#25603,0.400018246554086);
#9526=CIRCLE('',#25605,0.400000000003301);
#9527=CIRCLE('',#25606,0.400000000003301);
#9528=CIRCLE('',#25608,0.400000000000401);
#9529=CIRCLE('',#25610,0.400025722217637);
#9530=CIRCLE('',#25611,0.500009101578587);
#9531=CIRCLE('',#25612,9.832396974191);
#9532=CIRCLE('',#25613,9.832396974191);
#9533=CIRCLE('',#25614,9.83239697419101);
#9534=CIRCLE('',#25615,9.832396974191);
#9535=CIRCLE('',#25616,9.832396974191);
#9536=CIRCLE('',#25617,9.832396974191);
#9537=CIRCLE('',#25618,9.832396974191);
#9538=CIRCLE('',#25619,9.832396974191);
#9539=CIRCLE('',#25620,9.832396974191);
#9540=CIRCLE('',#25621,9.832396974191);
#9541=CIRCLE('',#25622,9.832396974191);
#9542=CIRCLE('',#25623,9.832396974191);
#9543=CIRCLE('',#25625,1.5);
#9544=CIRCLE('',#25627,1.5);
#9545=CIRCLE('',#25629,1.5);
#9546=CIRCLE('',#25631,1.5);
#9547=CIRCLE('',#25634,0.500022231909381);
#9548=CIRCLE('',#25636,1.5);
#9549=CIRCLE('',#25638,1.5);
#9550=CIRCLE('',#25640,1.5);
#9551=CIRCLE('',#25642,1.5);
#10751=VERTEX_POINT('',#36397);
#10752=VERTEX_POINT('',#36400);
#10753=VERTEX_POINT('',#36404);
#10754=VERTEX_POINT('',#36406);
#10755=VERTEX_POINT('',#36410);
#10756=VERTEX_POINT('',#36413);
#10757=VERTEX_POINT('',#36417);
#10758=VERTEX_POINT('',#36418);
#10759=VERTEX_POINT('',#36420);
#10760=VERTEX_POINT('',#36463);
#10761=VERTEX_POINT('',#36486);
#10762=VERTEX_POINT('',#36591);
#10763=VERTEX_POINT('',#36593);
#10764=VERTEX_POINT('',#36677);
#10765=VERTEX_POINT('',#36678);
#10766=VERTEX_POINT('',#36680);
#10767=VERTEX_POINT('',#36688);
#10768=VERTEX_POINT('',#36831);
#10769=VERTEX_POINT('',#36905);
#10770=VERTEX_POINT('',#36963);
#10771=VERTEX_POINT('',#36964);
#10772=VERTEX_POINT('',#36966);
#10773=VERTEX_POINT('',#37113);
#10774=VERTEX_POINT('',#37203);
#10775=VERTEX_POINT('',#37427);
#10776=VERTEX_POINT('',#37539);
#10777=VERTEX_POINT('',#37674);
#10778=VERTEX_POINT('',#37675);
#10779=VERTEX_POINT('',#37830);
#10780=VERTEX_POINT('',#37892);
#10781=VERTEX_POINT('',#37893);
#10782=VERTEX_POINT('',#37895);
#10783=VERTEX_POINT('',#37903);
#10784=VERTEX_POINT('',#38045);
#10785=VERTEX_POINT('',#38068);
#10786=VERTEX_POINT('',#38081);
#10787=VERTEX_POINT('',#38507);
#10788=VERTEX_POINT('',#38668);
#10789=VERTEX_POINT('',#38669);
#10790=VERTEX_POINT('',#38719);
#10791=VERTEX_POINT('',#38727);
#10792=VERTEX_POINT('',#39209);
#10793=VERTEX_POINT('',#39210);
#10794=VERTEX_POINT('',#39212);
#10795=VERTEX_POINT('',#39220);
#10796=VERTEX_POINT('',#39363);
#10797=VERTEX_POINT('',#39437);
#10798=VERTEX_POINT('',#39495);
#10799=VERTEX_POINT('',#39496);
#10800=VERTEX_POINT('',#39498);
#10801=VERTEX_POINT('',#39645);
#10802=VERTEX_POINT('',#39733);
#10803=VERTEX_POINT('',#39957);
#10804=VERTEX_POINT('',#40069);
#10805=VERTEX_POINT('',#40213);
#10806=VERTEX_POINT('',#40214);
#10807=VERTEX_POINT('',#40369);
#10808=VERTEX_POINT('',#40431);
#10809=VERTEX_POINT('',#40432);
#10810=VERTEX_POINT('',#40434);
#10811=VERTEX_POINT('',#40442);
#10812=VERTEX_POINT('',#40584);
#10813=VERTEX_POINT('',#40607);
#10814=VERTEX_POINT('',#40620);
#10815=VERTEX_POINT('',#41046);
#10816=VERTEX_POINT('',#41207);
#10817=VERTEX_POINT('',#41208);
#10818=VERTEX_POINT('',#41258);
#10819=VERTEX_POINT('',#41266);
#10820=VERTEX_POINT('',#41769);
#10821=VERTEX_POINT('',#41770);
#10822=VERTEX_POINT('',#41772);
#10823=VERTEX_POINT('',#41780);
#10824=VERTEX_POINT('',#41923);
#10825=VERTEX_POINT('',#41997);
#10826=VERTEX_POINT('',#42055);
#10827=VERTEX_POINT('',#42056);
#10828=VERTEX_POINT('',#42058);
#10829=VERTEX_POINT('',#42205);
#10830=VERTEX_POINT('',#42294);
#10831=VERTEX_POINT('',#42518);
#10832=VERTEX_POINT('',#42634);
#10833=VERTEX_POINT('',#42754);
#10834=VERTEX_POINT('',#42755);
#10835=VERTEX_POINT('',#42907);
#10836=VERTEX_POINT('',#42969);
#10837=VERTEX_POINT('',#42970);
#10838=VERTEX_POINT('',#42972);
#10839=VERTEX_POINT('',#42980);
#10840=VERTEX_POINT('',#43122);
#10841=VERTEX_POINT('',#43145);
#10842=VERTEX_POINT('',#43158);
#10843=VERTEX_POINT('',#43584);
#10844=VERTEX_POINT('',#43745);
#10845=VERTEX_POINT('',#43746);
#10846=VERTEX_POINT('',#43796);
#10847=VERTEX_POINT('',#43804);
#10848=VERTEX_POINT('',#44295);
#10849=VERTEX_POINT('',#44296);
#10850=VERTEX_POINT('',#44298);
#10851=VERTEX_POINT('',#44306);
#10852=VERTEX_POINT('',#44452);
#10853=VERTEX_POINT('',#44526);
#10854=VERTEX_POINT('',#44584);
#10855=VERTEX_POINT('',#44585);
#10856=VERTEX_POINT('',#44587);
#10857=VERTEX_POINT('',#44734);
#10858=VERTEX_POINT('',#44824);
#10859=VERTEX_POINT('',#45048);
#10860=VERTEX_POINT('',#45160);
#10861=VERTEX_POINT('',#45286);
#10862=VERTEX_POINT('',#45287);
#10863=VERTEX_POINT('',#45442);
#10864=VERTEX_POINT('',#45500);
#10865=VERTEX_POINT('',#45501);
#10866=VERTEX_POINT('',#45503);
#10867=VERTEX_POINT('',#45520);
#10868=VERTEX_POINT('',#45656);
#10869=VERTEX_POINT('',#45679);
#10870=VERTEX_POINT('',#45692);
#10871=VERTEX_POINT('',#46118);
#10872=VERTEX_POINT('',#46275);
#10873=VERTEX_POINT('',#46276);
#10874=VERTEX_POINT('',#46326);
#10875=VERTEX_POINT('',#46343);
#10876=VERTEX_POINT('',#46781);
#10877=VERTEX_POINT('',#46782);
#10878=VERTEX_POINT('',#46784);
#10879=VERTEX_POINT('',#46803);
#10880=VERTEX_POINT('',#46805);
#10881=VERTEX_POINT('',#46818);
#10882=VERTEX_POINT('',#46865);
#10883=VERTEX_POINT('',#46939);
#10884=VERTEX_POINT('',#47068);
#10885=VERTEX_POINT('',#47070);
#10886=VERTEX_POINT('',#47158);
#10887=VERTEX_POINT('',#47159);
#10888=VERTEX_POINT('',#47321);
#10889=VERTEX_POINT('',#47597);
#10890=VERTEX_POINT('',#47688);
#10891=VERTEX_POINT('',#47731);
#10892=VERTEX_POINT('',#47842);
#10893=VERTEX_POINT('',#47935);
#10894=VERTEX_POINT('',#47936);
#10895=VERTEX_POINT('',#47938);
#10896=VERTEX_POINT('',#47946);
#10897=VERTEX_POINT('',#48092);
#10898=VERTEX_POINT('',#48166);
#10899=VERTEX_POINT('',#48224);
#10900=VERTEX_POINT('',#48225);
#10901=VERTEX_POINT('',#48227);
#10902=VERTEX_POINT('',#48374);
#10903=VERTEX_POINT('',#48462);
#10904=VERTEX_POINT('',#48686);
#10905=VERTEX_POINT('',#48810);
#10906=VERTEX_POINT('',#48957);
#10907=VERTEX_POINT('',#48958);
#10908=VERTEX_POINT('',#49110);
#10909=VERTEX_POINT('',#49172);
#10910=VERTEX_POINT('',#49173);
#10911=VERTEX_POINT('',#49175);
#10912=VERTEX_POINT('',#49183);
#10913=VERTEX_POINT('',#49325);
#10914=VERTEX_POINT('',#49348);
#10915=VERTEX_POINT('',#49361);
#10916=VERTEX_POINT('',#49787);
#10917=VERTEX_POINT('',#49948);
#10918=VERTEX_POINT('',#49949);
#10919=VERTEX_POINT('',#49996);
#10920=VERTEX_POINT('',#50004);
#10921=VERTEX_POINT('',#50492);
#10922=VERTEX_POINT('',#50493);
#10923=VERTEX_POINT('',#50653);
#10924=VERTEX_POINT('',#50656);
#10925=VERTEX_POINT('',#50660);
#10926=VERTEX_POINT('',#50663);
#10927=VERTEX_POINT('',#51246);
#10928=VERTEX_POINT('',#51423);
#10929=VERTEX_POINT('',#51645);
#10930=VERTEX_POINT('',#51648);
#10931=VERTEX_POINT('',#51652);
#10932=VERTEX_POINT('',#51655);
#13225=EDGE_CURVE('',#10751,#10751,#9430,.T.);
#13226=EDGE_CURVE('',#10751,#10752,#5713,.T.);
#13227=EDGE_CURVE('',#10752,#10752,#9431,.T.);
#13228=EDGE_CURVE('',#10753,#10753,#9432,.T.);
#13229=EDGE_CURVE('',#10753,#10754,#5714,.T.);
#13230=EDGE_CURVE('',#10754,#10754,#9433,.T.);
#13231=EDGE_CURVE('',#10755,#10755,#9434,.T.);
#13232=EDGE_CURVE('',#10756,#10756,#9435,.T.);
#13233=EDGE_CURVE('',#10756,#10755,#5715,.T.);
#13234=EDGE_CURVE('',#10757,#10758,#9436,.T.);
#13235=EDGE_CURVE('',#10759,#10757,#9437,.T.);
#13236=EDGE_CURVE('',#10758,#10759,#9438,.T.);
#13237=EDGE_CURVE('',#10760,#10759,#664,.T.);
#13238=EDGE_CURVE('',#10761,#10757,#665,.T.);
#13239=EDGE_CURVE('',#10760,#10761,#666,.T.);
#13240=EDGE_CURVE('',#10761,#10762,#9439,.T.);
#13241=EDGE_CURVE('',#10763,#10762,#667,.T.);
#13242=EDGE_CURVE('',#10760,#10763,#668,.T.);
#13243=EDGE_CURVE('',#10764,#10765,#9440,.T.);
#13244=EDGE_CURVE('',#10766,#10765,#669,.T.);
#13245=EDGE_CURVE('',#10767,#10766,#670,.T.);
#13246=EDGE_CURVE('',#10767,#10764,#671,.T.);
#13247=EDGE_CURVE('',#10768,#10767,#672,.T.);
#13248=EDGE_CURVE('',#10768,#10769,#9441,.T.);
#13249=EDGE_CURVE('',#10769,#10764,#673,.T.);
#13250=EDGE_CURVE('',#10770,#10771,#9442,.T.);
#13251=EDGE_CURVE('',#10771,#10772,#54,.T.);
#13252=EDGE_CURVE('',#10772,#10768,#9443,.T.);
#13253=EDGE_CURVE('',#10770,#10768,#674,.T.);
#13254=EDGE_CURVE('',#10769,#10772,#9444,.T.);
#13255=EDGE_CURVE('',#10773,#10772,#675,.T.);
#13256=EDGE_CURVE('',#10773,#10774,#9445,.T.);
#13257=EDGE_CURVE('',#10774,#10769,#676,.T.);
#13258=EDGE_CURVE('',#10774,#10775,#677,.T.);
#13259=EDGE_CURVE('',#10764,#10775,#678,.T.);
#13260=EDGE_CURVE('',#10775,#10776,#9446,.T.);
#13261=EDGE_CURVE('',#10765,#10776,#679,.T.);
#13262=EDGE_CURVE('',#10777,#10778,#680,.T.);
#13263=EDGE_CURVE('',#10776,#10778,#681,.T.);
#13264=EDGE_CURVE('',#10775,#10777,#682,.T.);
#13265=EDGE_CURVE('',#10774,#10779,#9447,.T.);
#13266=EDGE_CURVE('',#10779,#10777,#683,.T.);
#13267=EDGE_CURVE('',#10779,#10773,#9448,.T.);
#13268=EDGE_CURVE('',#10780,#10781,#9449,.T.);
#13269=EDGE_CURVE('',#10782,#10781,#684,.T.);
#13270=EDGE_CURVE('',#10783,#10782,#685,.T.);
#13271=EDGE_CURVE('',#10783,#10780,#686,.T.);
#13272=EDGE_CURVE('',#10783,#10784,#687,.T.);
#13273=EDGE_CURVE('',#10784,#10785,#9450,.T.);
#13274=EDGE_CURVE('',#10780,#10785,#688,.T.);
#13275=EDGE_CURVE('',#10785,#10786,#9451,.T.);
#13276=EDGE_CURVE('',#10786,#10784,#9452,.T.);
#13277=EDGE_CURVE('',#10786,#10773,#55,.T.);
#13278=EDGE_CURVE('',#10784,#10779,#689,.T.);
#13279=EDGE_CURVE('',#10786,#10771,#690,.T.);
#13280=EDGE_CURVE('',#10771,#10787,#9453,.T.);
#13281=EDGE_CURVE('',#10785,#10787,#691,.T.);
#13282=EDGE_CURVE('',#10787,#10770,#9454,.T.);
#13283=EDGE_CURVE('',#10788,#10789,#692,.T.);
#13284=EDGE_CURVE('',#10790,#10789,#693,.T.);
#13285=EDGE_CURVE('',#10791,#10790,#9455,.T.);
#13286=EDGE_CURVE('',#10791,#10788,#694,.T.);
#13287=EDGE_CURVE('',#10791,#10787,#695,.T.);
#13288=EDGE_CURVE('',#10788,#10770,#696,.T.);
#13289=EDGE_CURVE('',#10780,#10791,#697,.T.);
#13290=EDGE_CURVE('',#10781,#10790,#698,.T.);
#13291=EDGE_CURVE('',#10792,#10793,#9456,.T.);
#13292=EDGE_CURVE('',#10794,#10793,#699,.T.);
#13293=EDGE_CURVE('',#10795,#10794,#700,.T.);
#13294=EDGE_CURVE('',#10795,#10792,#701,.T.);
#13295=EDGE_CURVE('',#10796,#10795,#702,.T.);
#13296=EDGE_CURVE('',#10796,#10797,#9457,.T.);
#13297=EDGE_CURVE('',#10797,#10792,#703,.T.);
#13298=EDGE_CURVE('',#10798,#10799,#9458,.T.);
#13299=EDGE_CURVE('',#10799,#10800,#56,.T.);
#13300=EDGE_CURVE('',#10800,#10796,#9459,.T.);
#13301=EDGE_CURVE('',#10798,#10796,#704,.T.);
#13302=EDGE_CURVE('',#10797,#10800,#9460,.T.);
#13303=EDGE_CURVE('',#10801,#10800,#705,.T.);
#13304=EDGE_CURVE('',#10801,#10802,#9461,.T.);
#13305=EDGE_CURVE('',#10802,#10797,#706,.T.);
#13306=EDGE_CURVE('',#10802,#10803,#707,.T.);
#13307=EDGE_CURVE('',#10792,#10803,#708,.T.);
#13308=EDGE_CURVE('',#10803,#10804,#9462,.T.);
#13309=EDGE_CURVE('',#10793,#10804,#709,.T.);
#13310=EDGE_CURVE('',#10805,#10806,#710,.T.);
#13311=EDGE_CURVE('',#10804,#10806,#711,.T.);
#13312=EDGE_CURVE('',#10803,#10805,#712,.T.);
#13313=EDGE_CURVE('',#10802,#10807,#9463,.T.);
#13314=EDGE_CURVE('',#10807,#10805,#713,.T.);
#13315=EDGE_CURVE('',#10807,#10801,#9464,.T.);
#13316=EDGE_CURVE('',#10808,#10809,#9465,.T.);
#13317=EDGE_CURVE('',#10810,#10809,#714,.T.);
#13318=EDGE_CURVE('',#10811,#10810,#715,.T.);
#13319=EDGE_CURVE('',#10811,#10808,#716,.T.);
#13320=EDGE_CURVE('',#10811,#10812,#717,.T.);
#13321=EDGE_CURVE('',#10812,#10813,#9466,.T.);
#13322=EDGE_CURVE('',#10808,#10813,#718,.T.);
#13323=EDGE_CURVE('',#10813,#10814,#9467,.T.);
#13324=EDGE_CURVE('',#10814,#10812,#9468,.T.);
#13325=EDGE_CURVE('',#10814,#10801,#57,.T.);
#13326=EDGE_CURVE('',#10812,#10807,#719,.T.);
#13327=EDGE_CURVE('',#10814,#10799,#720,.T.);
#13328=EDGE_CURVE('',#10799,#10815,#9469,.T.);
#13329=EDGE_CURVE('',#10813,#10815,#721,.T.);
#13330=EDGE_CURVE('',#10815,#10798,#9470,.T.);
#13331=EDGE_CURVE('',#10816,#10817,#722,.T.);
#13332=EDGE_CURVE('',#10818,#10817,#723,.T.);
#13333=EDGE_CURVE('',#10819,#10818,#9471,.T.);
#13334=EDGE_CURVE('',#10819,#10816,#724,.T.);
#13335=EDGE_CURVE('',#10819,#10815,#725,.T.);
#13336=EDGE_CURVE('',#10816,#10798,#726,.T.);
#13337=EDGE_CURVE('',#10808,#10819,#727,.T.);
#13338=EDGE_CURVE('',#10809,#10818,#728,.T.);
#13339=EDGE_CURVE('',#10820,#10821,#9472,.T.);
#13340=EDGE_CURVE('',#10822,#10821,#729,.T.);
#13341=EDGE_CURVE('',#10823,#10822,#730,.T.);
#13342=EDGE_CURVE('',#10823,#10820,#731,.T.);
#13343=EDGE_CURVE('',#10824,#10823,#732,.T.);
#13344=EDGE_CURVE('',#10824,#10825,#9473,.T.);
#13345=EDGE_CURVE('',#10825,#10820,#733,.T.);
#13346=EDGE_CURVE('',#10826,#10827,#9474,.T.);
#13347=EDGE_CURVE('',#10827,#10828,#58,.T.);
#13348=EDGE_CURVE('',#10828,#10824,#9475,.T.);
#13349=EDGE_CURVE('',#10826,#10824,#734,.T.);
#13350=EDGE_CURVE('',#10825,#10828,#9476,.T.);
#13351=EDGE_CURVE('',#10829,#10828,#735,.T.);
#13352=EDGE_CURVE('',#10829,#10830,#9477,.T.);
#13353=EDGE_CURVE('',#10830,#10825,#736,.T.);
#13354=EDGE_CURVE('',#10830,#10831,#737,.T.);
#13355=EDGE_CURVE('',#10820,#10831,#738,.T.);
#13356=EDGE_CURVE('',#10831,#10832,#9478,.T.);
#13357=EDGE_CURVE('',#10821,#10832,#739,.T.);
#13358=EDGE_CURVE('',#10833,#10834,#740,.T.);
#13359=EDGE_CURVE('',#10832,#10834,#741,.T.);
#13360=EDGE_CURVE('',#10831,#10833,#742,.T.);
#13361=EDGE_CURVE('',#10830,#10835,#9479,.T.);
#13362=EDGE_CURVE('',#10835,#10833,#743,.T.);
#13363=EDGE_CURVE('',#10835,#10829,#9480,.T.);
#13364=EDGE_CURVE('',#10836,#10837,#9481,.T.);
#13365=EDGE_CURVE('',#10838,#10837,#744,.T.);
#13366=EDGE_CURVE('',#10839,#10838,#745,.T.);
#13367=EDGE_CURVE('',#10839,#10836,#746,.T.);
#13368=EDGE_CURVE('',#10839,#10840,#747,.T.);
#13369=EDGE_CURVE('',#10840,#10841,#9482,.T.);
#13370=EDGE_CURVE('',#10836,#10841,#748,.T.);
#13371=EDGE_CURVE('',#10841,#10842,#9483,.T.);
#13372=EDGE_CURVE('',#10842,#10840,#9484,.T.);
#13373=EDGE_CURVE('',#10842,#10829,#59,.T.);
#13374=EDGE_CURVE('',#10840,#10835,#749,.T.);
#13375=EDGE_CURVE('',#10842,#10827,#750,.T.);
#13376=EDGE_CURVE('',#10827,#10843,#9485,.T.);
#13377=EDGE_CURVE('',#10841,#10843,#751,.T.);
#13378=EDGE_CURVE('',#10843,#10826,#9486,.T.);
#13379=EDGE_CURVE('',#10844,#10845,#752,.T.);
#13380=EDGE_CURVE('',#10846,#10845,#753,.T.);
#13381=EDGE_CURVE('',#10847,#10846,#9487,.T.);
#13382=EDGE_CURVE('',#10847,#10844,#754,.T.);
#13383=EDGE_CURVE('',#10847,#10843,#755,.T.);
#13384=EDGE_CURVE('',#10844,#10826,#756,.T.);
#13385=EDGE_CURVE('',#10836,#10847,#757,.T.);
#13386=EDGE_CURVE('',#10837,#10846,#758,.T.);
#13387=EDGE_CURVE('',#10848,#10849,#9488,.T.);
#13388=EDGE_CURVE('',#10850,#10849,#759,.T.);
#13389=EDGE_CURVE('',#10851,#10850,#760,.T.);
#13390=EDGE_CURVE('',#10851,#10848,#761,.T.);
#13391=EDGE_CURVE('',#10852,#10851,#762,.T.);
#13392=EDGE_CURVE('',#10852,#10853,#9489,.T.);
#13393=EDGE_CURVE('',#10853,#10848,#763,.T.);
#13394=EDGE_CURVE('',#10854,#10855,#9490,.T.);
#13395=EDGE_CURVE('',#10855,#10856,#60,.T.);
#13396=EDGE_CURVE('',#10856,#10852,#9491,.T.);
#13397=EDGE_CURVE('',#10854,#10852,#764,.T.);
#13398=EDGE_CURVE('',#10853,#10856,#9492,.T.);
#13399=EDGE_CURVE('',#10857,#10856,#765,.T.);
#13400=EDGE_CURVE('',#10857,#10858,#9493,.T.);
#13401=EDGE_CURVE('',#10858,#10853,#766,.T.);
#13402=EDGE_CURVE('',#10858,#10859,#767,.T.);
#13403=EDGE_CURVE('',#10848,#10859,#768,.T.);
#13404=EDGE_CURVE('',#10859,#10860,#9494,.T.);
#13405=EDGE_CURVE('',#10849,#10860,#769,.T.);
#13406=EDGE_CURVE('',#10861,#10862,#770,.T.);
#13407=EDGE_CURVE('',#10860,#10862,#771,.T.);
#13408=EDGE_CURVE('',#10859,#10861,#772,.T.);
#13409=EDGE_CURVE('',#10858,#10863,#9495,.T.);
#13410=EDGE_CURVE('',#10863,#10861,#773,.T.);
#13411=EDGE_CURVE('',#10863,#10857,#9496,.T.);
#13412=EDGE_CURVE('',#10864,#10865,#9497,.T.);
#13413=EDGE_CURVE('',#10866,#10865,#774,.T.);
#13414=EDGE_CURVE('',#10867,#10866,#775,.T.);
#13415=EDGE_CURVE('',#10867,#10864,#776,.T.);
#13416=EDGE_CURVE('',#10867,#10868,#777,.T.);
#13417=EDGE_CURVE('',#10868,#10869,#9498,.T.);
#13418=EDGE_CURVE('',#10864,#10869,#778,.T.);
#13419=EDGE_CURVE('',#10869,#10870,#9499,.T.);
#13420=EDGE_CURVE('',#10870,#10868,#9500,.T.);
#13421=EDGE_CURVE('',#10870,#10857,#61,.T.);
#13422=EDGE_CURVE('',#10868,#10863,#779,.T.);
#13423=EDGE_CURVE('',#10870,#10855,#780,.T.);
#13424=EDGE_CURVE('',#10855,#10871,#9501,.T.);
#13425=EDGE_CURVE('',#10869,#10871,#781,.T.);
#13426=EDGE_CURVE('',#10871,#10854,#9502,.T.);
#13427=EDGE_CURVE('',#10872,#10873,#782,.T.);
#13428=EDGE_CURVE('',#10874,#10873,#783,.T.);
#13429=EDGE_CURVE('',#10875,#10874,#9503,.T.);
#13430=EDGE_CURVE('',#10875,#10872,#784,.T.);
#13431=EDGE_CURVE('',#10875,#10871,#785,.T.);
#13432=EDGE_CURVE('',#10872,#10854,#786,.T.);
#13433=EDGE_CURVE('',#10864,#10875,#787,.T.);
#13434=EDGE_CURVE('',#10865,#10874,#788,.T.);
#13435=EDGE_CURVE('',#10876,#10877,#9504,.T.);
#13436=EDGE_CURVE('',#10878,#10876,#9505,.T.);
#13437=EDGE_CURVE('',#10877,#10878,#9506,.T.);
#13438=EDGE_CURVE('',#10877,#10879,#62,.T.);
#13439=EDGE_CURVE('',#10879,#10880,#9507,.T.);
#13440=EDGE_CURVE('',#10876,#10880,#789,.T.);
#13441=EDGE_CURVE('',#10880,#10881,#9508,.T.);
#13442=EDGE_CURVE('',#10881,#10879,#9509,.T.);
#13443=EDGE_CURVE('',#10880,#10882,#790,.T.);
#13444=EDGE_CURVE('',#10881,#10883,#791,.T.);
#13445=EDGE_CURVE('',#10882,#10883,#792,.T.);
#13446=EDGE_CURVE('',#10883,#10884,#9510,.T.);
#13447=EDGE_CURVE('',#10885,#10884,#793,.T.);
#13448=EDGE_CURVE('',#10882,#10885,#794,.T.);
#13449=EDGE_CURVE('',#10886,#10887,#9511,.T.);
#13450=EDGE_CURVE('',#10884,#10887,#795,.T.);
#13451=EDGE_CURVE('',#10883,#10886,#796,.T.);
#13452=EDGE_CURVE('',#10888,#10881,#797,.T.);
#13453=EDGE_CURVE('',#10888,#10886,#798,.T.);
#13454=EDGE_CURVE('',#10889,#10879,#799,.T.);
#13455=EDGE_CURVE('',#10889,#10888,#9512,.T.);
#13456=EDGE_CURVE('',#10890,#10889,#9513,.T.);
#13457=EDGE_CURVE('',#10888,#10890,#9514,.T.);
#13458=EDGE_CURVE('',#10890,#10891,#800,.T.);
#13459=EDGE_CURVE('',#10886,#10891,#801,.T.);
#13460=EDGE_CURVE('',#10891,#10892,#802,.T.);
#13461=EDGE_CURVE('',#10887,#10892,#803,.T.);
#13462=EDGE_CURVE('',#10893,#10894,#9515,.T.);
#13463=EDGE_CURVE('',#10895,#10894,#804,.T.);
#13464=EDGE_CURVE('',#10896,#10895,#805,.T.);
#13465=EDGE_CURVE('',#10896,#10893,#806,.T.);
#13466=EDGE_CURVE('',#10897,#10896,#807,.T.);
#13467=EDGE_CURVE('',#10897,#10898,#9516,.T.);
#13468=EDGE_CURVE('',#10898,#10893,#808,.T.);
#13469=EDGE_CURVE('',#10899,#10900,#9517,.T.);
#13470=EDGE_CURVE('',#10900,#10901,#63,.T.);
#13471=EDGE_CURVE('',#10901,#10897,#9518,.T.);
#13472=EDGE_CURVE('',#10899,#10897,#809,.T.);
#13473=EDGE_CURVE('',#10898,#10901,#9519,.T.);
#13474=EDGE_CURVE('',#10902,#10901,#810,.T.);
#13475=EDGE_CURVE('',#10902,#10903,#9520,.T.);
#13476=EDGE_CURVE('',#10903,#10898,#811,.T.);
#13477=EDGE_CURVE('',#10903,#10904,#812,.T.);
#13478=EDGE_CURVE('',#10893,#10904,#813,.T.);
#13479=EDGE_CURVE('',#10904,#10905,#9521,.T.);
#13480=EDGE_CURVE('',#10894,#10905,#814,.T.);
#13481=EDGE_CURVE('',#10906,#10907,#815,.T.);
#13482=EDGE_CURVE('',#10905,#10907,#816,.T.);
#13483=EDGE_CURVE('',#10904,#10906,#817,.T.);
#13484=EDGE_CURVE('',#10903,#10908,#9522,.T.);
#13485=EDGE_CURVE('',#10908,#10906,#818,.T.);
#13486=EDGE_CURVE('',#10908,#10902,#9523,.T.);
#13487=EDGE_CURVE('',#10909,#10910,#9524,.T.);
#13488=EDGE_CURVE('',#10911,#10910,#819,.T.);
#13489=EDGE_CURVE('',#10912,#10911,#820,.T.);
#13490=EDGE_CURVE('',#10912,#10909,#821,.T.);
#13491=EDGE_CURVE('',#10912,#10913,#822,.T.);
#13492=EDGE_CURVE('',#10913,#10914,#9525,.T.);
#13493=EDGE_CURVE('',#10909,#10914,#823,.T.);
#13494=EDGE_CURVE('',#10914,#10915,#9526,.T.);
#13495=EDGE_CURVE('',#10915,#10913,#9527,.T.);
#13496=EDGE_CURVE('',#10915,#10902,#64,.T.);
#13497=EDGE_CURVE('',#10913,#10908,#824,.T.);
#13498=EDGE_CURVE('',#10915,#10900,#825,.T.);
#13499=EDGE_CURVE('',#10900,#10916,#9528,.T.);
#13500=EDGE_CURVE('',#10914,#10916,#826,.T.);
#13501=EDGE_CURVE('',#10916,#10899,#9529,.T.);
#13502=EDGE_CURVE('',#10917,#10918,#827,.T.);
#13503=EDGE_CURVE('',#10919,#10918,#828,.T.);
#13504=EDGE_CURVE('',#10920,#10919,#9530,.T.);
#13505=EDGE_CURVE('',#10920,#10917,#829,.T.);
#13506=EDGE_CURVE('',#10920,#10916,#830,.T.);
#13507=EDGE_CURVE('',#10917,#10899,#831,.T.);
#13508=EDGE_CURVE('',#10909,#10920,#832,.T.);
#13509=EDGE_CURVE('',#10910,#10919,#833,.T.);
#13510=EDGE_CURVE('',#10921,#10922,#834,.T.);
#13511=EDGE_CURVE('',#10766,#10922,#9531,.T.);
#13512=EDGE_CURVE('',#10763,#10778,#9532,.T.);
#13513=EDGE_CURVE('',#10762,#10921,#835,.T.);
#13514=EDGE_CURVE('',#10794,#10789,#9533,.T.);
#13515=EDGE_CURVE('',#10782,#10806,#9534,.T.);
#13516=EDGE_CURVE('',#10822,#10817,#9535,.T.);
#13517=EDGE_CURVE('',#10810,#10834,#9536,.T.);
#13518=EDGE_CURVE('',#10850,#10845,#9537,.T.);
#13519=EDGE_CURVE('',#10838,#10862,#9538,.T.);
#13520=EDGE_CURVE('',#10895,#10873,#9539,.T.);
#13521=EDGE_CURVE('',#10866,#10907,#9540,.T.);
#13522=EDGE_CURVE('',#10885,#10918,#9541,.T.);
#13523=EDGE_CURVE('',#10911,#10892,#9542,.T.);
#13524=EDGE_CURVE('',#10923,#10923,#9543,.T.);
#13525=EDGE_CURVE('',#10924,#10924,#9544,.T.);
#13526=EDGE_CURVE('',#10924,#10923,#5716,.T.);
#13527=EDGE_CURVE('',#10925,#10925,#9545,.T.);
#13528=EDGE_CURVE('',#10926,#10926,#9546,.T.);
#13529=EDGE_CURVE('',#10926,#10925,#5717,.T.);
#13530=EDGE_CURVE('',#10759,#10890,#836,.T.);
#13531=EDGE_CURVE('',#10758,#10889,#65,.T.);
#13532=EDGE_CURVE('',#10758,#10877,#837,.T.);
#13533=EDGE_CURVE('',#10757,#10878,#838,.T.);
#13534=EDGE_CURVE('',#10927,#10878,#839,.T.);
#13535=EDGE_CURVE('',#10761,#10927,#840,.T.);
#13536=EDGE_CURVE('',#10927,#10921,#9547,.T.);
#13537=EDGE_CURVE('',#10928,#10922,#841,.T.);
#13538=EDGE_CURVE('',#10927,#10928,#842,.T.);
#13539=EDGE_CURVE('',#10928,#10876,#843,.T.);
#13540=EDGE_CURVE('',#10929,#10929,#9548,.T.);
#13541=EDGE_CURVE('',#10929,#10930,#5718,.T.);
#13542=EDGE_CURVE('',#10930,#10930,#9549,.T.);
#13543=EDGE_CURVE('',#10931,#10931,#9550,.T.);
#13544=EDGE_CURVE('',#10931,#10932,#5719,.T.);
#13545=EDGE_CURVE('',#10932,#10932,#9551,.T.);
#17360=ORIENTED_EDGE('',*,*,#13225,.F.);
#17361=ORIENTED_EDGE('',*,*,#13225,.T.);
#17362=ORIENTED_EDGE('',*,*,#13226,.T.);
#17363=ORIENTED_EDGE('',*,*,#13227,.F.);
#17364=ORIENTED_EDGE('',*,*,#13226,.F.);
#17365=ORIENTED_EDGE('',*,*,#13228,.T.);
#17366=ORIENTED_EDGE('',*,*,#13229,.T.);
#17367=ORIENTED_EDGE('',*,*,#13230,.F.);
#17368=ORIENTED_EDGE('',*,*,#13229,.F.);
#17369=ORIENTED_EDGE('',*,*,#13231,.T.);
#17370=ORIENTED_EDGE('',*,*,#13232,.T.);
#17371=ORIENTED_EDGE('',*,*,#13233,.T.);
#17372=ORIENTED_EDGE('',*,*,#13231,.F.);
#17373=ORIENTED_EDGE('',*,*,#13233,.F.);
#17374=ORIENTED_EDGE('',*,*,#13234,.F.);
#17375=ORIENTED_EDGE('',*,*,#13235,.F.);
#17376=ORIENTED_EDGE('',*,*,#13236,.F.);
#17377=ORIENTED_EDGE('',*,*,#13237,.T.);
#17378=ORIENTED_EDGE('',*,*,#13235,.T.);
#17379=ORIENTED_EDGE('',*,*,#13238,.F.);
#17380=ORIENTED_EDGE('',*,*,#13239,.F.);
#17381=ORIENTED_EDGE('',*,*,#13240,.T.);
#17382=ORIENTED_EDGE('',*,*,#13241,.F.);
#17383=ORIENTED_EDGE('',*,*,#13242,.F.);
#17384=ORIENTED_EDGE('',*,*,#13239,.T.);
#17385=ORIENTED_EDGE('',*,*,#13243,.T.);
#17386=ORIENTED_EDGE('',*,*,#13244,.F.);
#17387=ORIENTED_EDGE('',*,*,#13245,.F.);
#17388=ORIENTED_EDGE('',*,*,#13246,.T.);
#17389=ORIENTED_EDGE('',*,*,#13247,.F.);
#17390=ORIENTED_EDGE('',*,*,#13248,.T.);
#17391=ORIENTED_EDGE('',*,*,#13249,.T.);
#17392=ORIENTED_EDGE('',*,*,#13246,.F.);
#17393=ORIENTED_EDGE('',*,*,#13250,.T.);
#17394=ORIENTED_EDGE('',*,*,#13251,.T.);
#17395=ORIENTED_EDGE('',*,*,#13252,.T.);
#17396=ORIENTED_EDGE('',*,*,#13253,.F.);
#17397=ORIENTED_EDGE('',*,*,#13248,.F.);
#17398=ORIENTED_EDGE('',*,*,#13252,.F.);
#17399=ORIENTED_EDGE('',*,*,#13254,.F.);
#17400=ORIENTED_EDGE('',*,*,#13254,.T.);
#17401=ORIENTED_EDGE('',*,*,#13255,.F.);
#17402=ORIENTED_EDGE('',*,*,#13256,.T.);
#17403=ORIENTED_EDGE('',*,*,#13257,.T.);
#17404=ORIENTED_EDGE('',*,*,#13249,.F.);
#17405=ORIENTED_EDGE('',*,*,#13257,.F.);
#17406=ORIENTED_EDGE('',*,*,#13258,.T.);
#17407=ORIENTED_EDGE('',*,*,#13259,.F.);
#17408=ORIENTED_EDGE('',*,*,#13260,.T.);
#17409=ORIENTED_EDGE('',*,*,#13261,.F.);
#17410=ORIENTED_EDGE('',*,*,#13243,.F.);
#17411=ORIENTED_EDGE('',*,*,#13259,.T.);
#17412=ORIENTED_EDGE('',*,*,#13262,.T.);
#17413=ORIENTED_EDGE('',*,*,#13263,.F.);
#17414=ORIENTED_EDGE('',*,*,#13260,.F.);
#17415=ORIENTED_EDGE('',*,*,#13264,.T.);
#17416=ORIENTED_EDGE('',*,*,#13258,.F.);
#17417=ORIENTED_EDGE('',*,*,#13265,.T.);
#17418=ORIENTED_EDGE('',*,*,#13266,.T.);
#17419=ORIENTED_EDGE('',*,*,#13264,.F.);
#17420=ORIENTED_EDGE('',*,*,#13256,.F.);
#17421=ORIENTED_EDGE('',*,*,#13267,.F.);
#17422=ORIENTED_EDGE('',*,*,#13265,.F.);
#17423=ORIENTED_EDGE('',*,*,#13268,.T.);
#17424=ORIENTED_EDGE('',*,*,#13269,.F.);
#17425=ORIENTED_EDGE('',*,*,#13270,.F.);
#17426=ORIENTED_EDGE('',*,*,#13271,.T.);
#17427=ORIENTED_EDGE('',*,*,#13272,.T.);
#17428=ORIENTED_EDGE('',*,*,#13273,.T.);
#17429=ORIENTED_EDGE('',*,*,#13274,.F.);
#17430=ORIENTED_EDGE('',*,*,#13271,.F.);
#17431=ORIENTED_EDGE('',*,*,#13275,.F.);
#17432=ORIENTED_EDGE('',*,*,#13273,.F.);
#17433=ORIENTED_EDGE('',*,*,#13276,.F.);
#17434=ORIENTED_EDGE('',*,*,#13267,.T.);
#17435=ORIENTED_EDGE('',*,*,#13277,.F.);
#17436=ORIENTED_EDGE('',*,*,#13276,.T.);
#17437=ORIENTED_EDGE('',*,*,#13278,.T.);
#17438=ORIENTED_EDGE('',*,*,#13255,.T.);
#17439=ORIENTED_EDGE('',*,*,#13251,.F.);
#17440=ORIENTED_EDGE('',*,*,#13279,.F.);
#17441=ORIENTED_EDGE('',*,*,#13277,.T.);
#17442=ORIENTED_EDGE('',*,*,#13280,.T.);
#17443=ORIENTED_EDGE('',*,*,#13281,.F.);
#17444=ORIENTED_EDGE('',*,*,#13275,.T.);
#17445=ORIENTED_EDGE('',*,*,#13279,.T.);
#17446=ORIENTED_EDGE('',*,*,#13250,.F.);
#17447=ORIENTED_EDGE('',*,*,#13282,.F.);
#17448=ORIENTED_EDGE('',*,*,#13280,.F.);
#17449=ORIENTED_EDGE('',*,*,#13283,.T.);
#17450=ORIENTED_EDGE('',*,*,#13284,.F.);
#17451=ORIENTED_EDGE('',*,*,#13285,.F.);
#17452=ORIENTED_EDGE('',*,*,#13286,.T.);
#17453=ORIENTED_EDGE('',*,*,#13287,.T.);
#17454=ORIENTED_EDGE('',*,*,#13282,.T.);
#17455=ORIENTED_EDGE('',*,*,#13288,.F.);
#17456=ORIENTED_EDGE('',*,*,#13286,.F.);
#17457=ORIENTED_EDGE('',*,*,#13274,.T.);
#17458=ORIENTED_EDGE('',*,*,#13281,.T.);
#17459=ORIENTED_EDGE('',*,*,#13287,.F.);
#17460=ORIENTED_EDGE('',*,*,#13289,.F.);
#17461=ORIENTED_EDGE('',*,*,#13285,.T.);
#17462=ORIENTED_EDGE('',*,*,#13290,.F.);
#17463=ORIENTED_EDGE('',*,*,#13268,.F.);
#17464=ORIENTED_EDGE('',*,*,#13289,.T.);
#17465=ORIENTED_EDGE('',*,*,#13291,.T.);
#17466=ORIENTED_EDGE('',*,*,#13292,.F.);
#17467=ORIENTED_EDGE('',*,*,#13293,.F.);
#17468=ORIENTED_EDGE('',*,*,#13294,.T.);
#17469=ORIENTED_EDGE('',*,*,#13295,.F.);
#17470=ORIENTED_EDGE('',*,*,#13296,.T.);
#17471=ORIENTED_EDGE('',*,*,#13297,.T.);
#17472=ORIENTED_EDGE('',*,*,#13294,.F.);
#17473=ORIENTED_EDGE('',*,*,#13298,.T.);
#17474=ORIENTED_EDGE('',*,*,#13299,.T.);
#17475=ORIENTED_EDGE('',*,*,#13300,.T.);
#17476=ORIENTED_EDGE('',*,*,#13301,.F.);
#17477=ORIENTED_EDGE('',*,*,#13296,.F.);
#17478=ORIENTED_EDGE('',*,*,#13300,.F.);
#17479=ORIENTED_EDGE('',*,*,#13302,.F.);
#17480=ORIENTED_EDGE('',*,*,#13302,.T.);
#17481=ORIENTED_EDGE('',*,*,#13303,.F.);
#17482=ORIENTED_EDGE('',*,*,#13304,.T.);
#17483=ORIENTED_EDGE('',*,*,#13305,.T.);
#17484=ORIENTED_EDGE('',*,*,#13297,.F.);
#17485=ORIENTED_EDGE('',*,*,#13305,.F.);
#17486=ORIENTED_EDGE('',*,*,#13306,.T.);
#17487=ORIENTED_EDGE('',*,*,#13307,.F.);
#17488=ORIENTED_EDGE('',*,*,#13308,.T.);
#17489=ORIENTED_EDGE('',*,*,#13309,.F.);
#17490=ORIENTED_EDGE('',*,*,#13291,.F.);
#17491=ORIENTED_EDGE('',*,*,#13307,.T.);
#17492=ORIENTED_EDGE('',*,*,#13310,.T.);
#17493=ORIENTED_EDGE('',*,*,#13311,.F.);
#17494=ORIENTED_EDGE('',*,*,#13308,.F.);
#17495=ORIENTED_EDGE('',*,*,#13312,.T.);
#17496=ORIENTED_EDGE('',*,*,#13306,.F.);
#17497=ORIENTED_EDGE('',*,*,#13313,.T.);
#17498=ORIENTED_EDGE('',*,*,#13314,.T.);
#17499=ORIENTED_EDGE('',*,*,#13312,.F.);
#17500=ORIENTED_EDGE('',*,*,#13304,.F.);
#17501=ORIENTED_EDGE('',*,*,#13315,.F.);
#17502=ORIENTED_EDGE('',*,*,#13313,.F.);
#17503=ORIENTED_EDGE('',*,*,#13316,.T.);
#17504=ORIENTED_EDGE('',*,*,#13317,.F.);
#17505=ORIENTED_EDGE('',*,*,#13318,.F.);
#17506=ORIENTED_EDGE('',*,*,#13319,.T.);
#17507=ORIENTED_EDGE('',*,*,#13320,.T.);
#17508=ORIENTED_EDGE('',*,*,#13321,.T.);
#17509=ORIENTED_EDGE('',*,*,#13322,.F.);
#17510=ORIENTED_EDGE('',*,*,#13319,.F.);
#17511=ORIENTED_EDGE('',*,*,#13323,.F.);
#17512=ORIENTED_EDGE('',*,*,#13321,.F.);
#17513=ORIENTED_EDGE('',*,*,#13324,.F.);
#17514=ORIENTED_EDGE('',*,*,#13315,.T.);
#17515=ORIENTED_EDGE('',*,*,#13325,.F.);
#17516=ORIENTED_EDGE('',*,*,#13324,.T.);
#17517=ORIENTED_EDGE('',*,*,#13326,.T.);
#17518=ORIENTED_EDGE('',*,*,#13303,.T.);
#17519=ORIENTED_EDGE('',*,*,#13299,.F.);
#17520=ORIENTED_EDGE('',*,*,#13327,.F.);
#17521=ORIENTED_EDGE('',*,*,#13325,.T.);
#17522=ORIENTED_EDGE('',*,*,#13328,.T.);
#17523=ORIENTED_EDGE('',*,*,#13329,.F.);
#17524=ORIENTED_EDGE('',*,*,#13323,.T.);
#17525=ORIENTED_EDGE('',*,*,#13327,.T.);
#17526=ORIENTED_EDGE('',*,*,#13298,.F.);
#17527=ORIENTED_EDGE('',*,*,#13330,.F.);
#17528=ORIENTED_EDGE('',*,*,#13328,.F.);
#17529=ORIENTED_EDGE('',*,*,#13331,.T.);
#17530=ORIENTED_EDGE('',*,*,#13332,.F.);
#17531=ORIENTED_EDGE('',*,*,#13333,.F.);
#17532=ORIENTED_EDGE('',*,*,#13334,.T.);
#17533=ORIENTED_EDGE('',*,*,#13335,.T.);
#17534=ORIENTED_EDGE('',*,*,#13330,.T.);
#17535=ORIENTED_EDGE('',*,*,#13336,.F.);
#17536=ORIENTED_EDGE('',*,*,#13334,.F.);
#17537=ORIENTED_EDGE('',*,*,#13322,.T.);
#17538=ORIENTED_EDGE('',*,*,#13329,.T.);
#17539=ORIENTED_EDGE('',*,*,#13335,.F.);
#17540=ORIENTED_EDGE('',*,*,#13337,.F.);
#17541=ORIENTED_EDGE('',*,*,#13333,.T.);
#17542=ORIENTED_EDGE('',*,*,#13338,.F.);
#17543=ORIENTED_EDGE('',*,*,#13316,.F.);
#17544=ORIENTED_EDGE('',*,*,#13337,.T.);
#17545=ORIENTED_EDGE('',*,*,#13339,.T.);
#17546=ORIENTED_EDGE('',*,*,#13340,.F.);
#17547=ORIENTED_EDGE('',*,*,#13341,.F.);
#17548=ORIENTED_EDGE('',*,*,#13342,.T.);
#17549=ORIENTED_EDGE('',*,*,#13343,.F.);
#17550=ORIENTED_EDGE('',*,*,#13344,.T.);
#17551=ORIENTED_EDGE('',*,*,#13345,.T.);
#17552=ORIENTED_EDGE('',*,*,#13342,.F.);
#17553=ORIENTED_EDGE('',*,*,#13346,.T.);
#17554=ORIENTED_EDGE('',*,*,#13347,.T.);
#17555=ORIENTED_EDGE('',*,*,#13348,.T.);
#17556=ORIENTED_EDGE('',*,*,#13349,.F.);
#17557=ORIENTED_EDGE('',*,*,#13344,.F.);
#17558=ORIENTED_EDGE('',*,*,#13348,.F.);
#17559=ORIENTED_EDGE('',*,*,#13350,.F.);
#17560=ORIENTED_EDGE('',*,*,#13350,.T.);
#17561=ORIENTED_EDGE('',*,*,#13351,.F.);
#17562=ORIENTED_EDGE('',*,*,#13352,.T.);
#17563=ORIENTED_EDGE('',*,*,#13353,.T.);
#17564=ORIENTED_EDGE('',*,*,#13345,.F.);
#17565=ORIENTED_EDGE('',*,*,#13353,.F.);
#17566=ORIENTED_EDGE('',*,*,#13354,.T.);
#17567=ORIENTED_EDGE('',*,*,#13355,.F.);
#17568=ORIENTED_EDGE('',*,*,#13356,.T.);
#17569=ORIENTED_EDGE('',*,*,#13357,.F.);
#17570=ORIENTED_EDGE('',*,*,#13339,.F.);
#17571=ORIENTED_EDGE('',*,*,#13355,.T.);
#17572=ORIENTED_EDGE('',*,*,#13358,.T.);
#17573=ORIENTED_EDGE('',*,*,#13359,.F.);
#17574=ORIENTED_EDGE('',*,*,#13356,.F.);
#17575=ORIENTED_EDGE('',*,*,#13360,.T.);
#17576=ORIENTED_EDGE('',*,*,#13354,.F.);
#17577=ORIENTED_EDGE('',*,*,#13361,.T.);
#17578=ORIENTED_EDGE('',*,*,#13362,.T.);
#17579=ORIENTED_EDGE('',*,*,#13360,.F.);
#17580=ORIENTED_EDGE('',*,*,#13352,.F.);
#17581=ORIENTED_EDGE('',*,*,#13363,.F.);
#17582=ORIENTED_EDGE('',*,*,#13361,.F.);
#17583=ORIENTED_EDGE('',*,*,#13364,.T.);
#17584=ORIENTED_EDGE('',*,*,#13365,.F.);
#17585=ORIENTED_EDGE('',*,*,#13366,.F.);
#17586=ORIENTED_EDGE('',*,*,#13367,.T.);
#17587=ORIENTED_EDGE('',*,*,#13368,.T.);
#17588=ORIENTED_EDGE('',*,*,#13369,.T.);
#17589=ORIENTED_EDGE('',*,*,#13370,.F.);
#17590=ORIENTED_EDGE('',*,*,#13367,.F.);
#17591=ORIENTED_EDGE('',*,*,#13371,.F.);
#17592=ORIENTED_EDGE('',*,*,#13369,.F.);
#17593=ORIENTED_EDGE('',*,*,#13372,.F.);
#17594=ORIENTED_EDGE('',*,*,#13363,.T.);
#17595=ORIENTED_EDGE('',*,*,#13373,.F.);
#17596=ORIENTED_EDGE('',*,*,#13372,.T.);
#17597=ORIENTED_EDGE('',*,*,#13374,.T.);
#17598=ORIENTED_EDGE('',*,*,#13351,.T.);
#17599=ORIENTED_EDGE('',*,*,#13347,.F.);
#17600=ORIENTED_EDGE('',*,*,#13375,.F.);
#17601=ORIENTED_EDGE('',*,*,#13373,.T.);
#17602=ORIENTED_EDGE('',*,*,#13376,.T.);
#17603=ORIENTED_EDGE('',*,*,#13377,.F.);
#17604=ORIENTED_EDGE('',*,*,#13371,.T.);
#17605=ORIENTED_EDGE('',*,*,#13375,.T.);
#17606=ORIENTED_EDGE('',*,*,#13346,.F.);
#17607=ORIENTED_EDGE('',*,*,#13378,.F.);
#17608=ORIENTED_EDGE('',*,*,#13376,.F.);
#17609=ORIENTED_EDGE('',*,*,#13379,.T.);
#17610=ORIENTED_EDGE('',*,*,#13380,.F.);
#17611=ORIENTED_EDGE('',*,*,#13381,.F.);
#17612=ORIENTED_EDGE('',*,*,#13382,.T.);
#17613=ORIENTED_EDGE('',*,*,#13383,.T.);
#17614=ORIENTED_EDGE('',*,*,#13378,.T.);
#17615=ORIENTED_EDGE('',*,*,#13384,.F.);
#17616=ORIENTED_EDGE('',*,*,#13382,.F.);
#17617=ORIENTED_EDGE('',*,*,#13370,.T.);
#17618=ORIENTED_EDGE('',*,*,#13377,.T.);
#17619=ORIENTED_EDGE('',*,*,#13383,.F.);
#17620=ORIENTED_EDGE('',*,*,#13385,.F.);
#17621=ORIENTED_EDGE('',*,*,#13381,.T.);
#17622=ORIENTED_EDGE('',*,*,#13386,.F.);
#17623=ORIENTED_EDGE('',*,*,#13364,.F.);
#17624=ORIENTED_EDGE('',*,*,#13385,.T.);
#17625=ORIENTED_EDGE('',*,*,#13387,.T.);
#17626=ORIENTED_EDGE('',*,*,#13388,.F.);
#17627=ORIENTED_EDGE('',*,*,#13389,.F.);
#17628=ORIENTED_EDGE('',*,*,#13390,.T.);
#17629=ORIENTED_EDGE('',*,*,#13391,.F.);
#17630=ORIENTED_EDGE('',*,*,#13392,.T.);
#17631=ORIENTED_EDGE('',*,*,#13393,.T.);
#17632=ORIENTED_EDGE('',*,*,#13390,.F.);
#17633=ORIENTED_EDGE('',*,*,#13394,.T.);
#17634=ORIENTED_EDGE('',*,*,#13395,.T.);
#17635=ORIENTED_EDGE('',*,*,#13396,.T.);
#17636=ORIENTED_EDGE('',*,*,#13397,.F.);
#17637=ORIENTED_EDGE('',*,*,#13392,.F.);
#17638=ORIENTED_EDGE('',*,*,#13396,.F.);
#17639=ORIENTED_EDGE('',*,*,#13398,.F.);
#17640=ORIENTED_EDGE('',*,*,#13398,.T.);
#17641=ORIENTED_EDGE('',*,*,#13399,.F.);
#17642=ORIENTED_EDGE('',*,*,#13400,.T.);
#17643=ORIENTED_EDGE('',*,*,#13401,.T.);
#17644=ORIENTED_EDGE('',*,*,#13393,.F.);
#17645=ORIENTED_EDGE('',*,*,#13401,.F.);
#17646=ORIENTED_EDGE('',*,*,#13402,.T.);
#17647=ORIENTED_EDGE('',*,*,#13403,.F.);
#17648=ORIENTED_EDGE('',*,*,#13404,.T.);
#17649=ORIENTED_EDGE('',*,*,#13405,.F.);
#17650=ORIENTED_EDGE('',*,*,#13387,.F.);
#17651=ORIENTED_EDGE('',*,*,#13403,.T.);
#17652=ORIENTED_EDGE('',*,*,#13406,.T.);
#17653=ORIENTED_EDGE('',*,*,#13407,.F.);
#17654=ORIENTED_EDGE('',*,*,#13404,.F.);
#17655=ORIENTED_EDGE('',*,*,#13408,.T.);
#17656=ORIENTED_EDGE('',*,*,#13402,.F.);
#17657=ORIENTED_EDGE('',*,*,#13409,.T.);
#17658=ORIENTED_EDGE('',*,*,#13410,.T.);
#17659=ORIENTED_EDGE('',*,*,#13408,.F.);
#17660=ORIENTED_EDGE('',*,*,#13400,.F.);
#17661=ORIENTED_EDGE('',*,*,#13411,.F.);
#17662=ORIENTED_EDGE('',*,*,#13409,.F.);
#17663=ORIENTED_EDGE('',*,*,#13412,.T.);
#17664=ORIENTED_EDGE('',*,*,#13413,.F.);
#17665=ORIENTED_EDGE('',*,*,#13414,.F.);
#17666=ORIENTED_EDGE('',*,*,#13415,.T.);
#17667=ORIENTED_EDGE('',*,*,#13416,.T.);
#17668=ORIENTED_EDGE('',*,*,#13417,.T.);
#17669=ORIENTED_EDGE('',*,*,#13418,.F.);
#17670=ORIENTED_EDGE('',*,*,#13415,.F.);
#17671=ORIENTED_EDGE('',*,*,#13419,.F.);
#17672=ORIENTED_EDGE('',*,*,#13417,.F.);
#17673=ORIENTED_EDGE('',*,*,#13420,.F.);
#17674=ORIENTED_EDGE('',*,*,#13411,.T.);
#17675=ORIENTED_EDGE('',*,*,#13421,.F.);
#17676=ORIENTED_EDGE('',*,*,#13420,.T.);
#17677=ORIENTED_EDGE('',*,*,#13422,.T.);
#17678=ORIENTED_EDGE('',*,*,#13399,.T.);
#17679=ORIENTED_EDGE('',*,*,#13395,.F.);
#17680=ORIENTED_EDGE('',*,*,#13423,.F.);
#17681=ORIENTED_EDGE('',*,*,#13421,.T.);
#17682=ORIENTED_EDGE('',*,*,#13424,.T.);
#17683=ORIENTED_EDGE('',*,*,#13425,.F.);
#17684=ORIENTED_EDGE('',*,*,#13419,.T.);
#17685=ORIENTED_EDGE('',*,*,#13423,.T.);
#17686=ORIENTED_EDGE('',*,*,#13394,.F.);
#17687=ORIENTED_EDGE('',*,*,#13426,.F.);
#17688=ORIENTED_EDGE('',*,*,#13424,.F.);
#17689=ORIENTED_EDGE('',*,*,#13427,.T.);
#17690=ORIENTED_EDGE('',*,*,#13428,.F.);
#17691=ORIENTED_EDGE('',*,*,#13429,.F.);
#17692=ORIENTED_EDGE('',*,*,#13430,.T.);
#17693=ORIENTED_EDGE('',*,*,#13431,.T.);
#17694=ORIENTED_EDGE('',*,*,#13426,.T.);
#17695=ORIENTED_EDGE('',*,*,#13432,.F.);
#17696=ORIENTED_EDGE('',*,*,#13430,.F.);
#17697=ORIENTED_EDGE('',*,*,#13418,.T.);
#17698=ORIENTED_EDGE('',*,*,#13425,.T.);
#17699=ORIENTED_EDGE('',*,*,#13431,.F.);
#17700=ORIENTED_EDGE('',*,*,#13433,.F.);
#17701=ORIENTED_EDGE('',*,*,#13429,.T.);
#17702=ORIENTED_EDGE('',*,*,#13434,.F.);
#17703=ORIENTED_EDGE('',*,*,#13412,.F.);
#17704=ORIENTED_EDGE('',*,*,#13433,.T.);
#17705=ORIENTED_EDGE('',*,*,#13435,.F.);
#17706=ORIENTED_EDGE('',*,*,#13436,.F.);
#17707=ORIENTED_EDGE('',*,*,#13437,.F.);
#17708=ORIENTED_EDGE('',*,*,#13435,.T.);
#17709=ORIENTED_EDGE('',*,*,#13438,.T.);
#17710=ORIENTED_EDGE('',*,*,#13439,.T.);
#17711=ORIENTED_EDGE('',*,*,#13440,.F.);
#17712=ORIENTED_EDGE('',*,*,#13441,.F.);
#17713=ORIENTED_EDGE('',*,*,#13439,.F.);
#17714=ORIENTED_EDGE('',*,*,#13442,.F.);
#17715=ORIENTED_EDGE('',*,*,#13443,.F.);
#17716=ORIENTED_EDGE('',*,*,#13441,.T.);
#17717=ORIENTED_EDGE('',*,*,#13444,.T.);
#17718=ORIENTED_EDGE('',*,*,#13445,.F.);
#17719=ORIENTED_EDGE('',*,*,#13446,.T.);
#17720=ORIENTED_EDGE('',*,*,#13447,.F.);
#17721=ORIENTED_EDGE('',*,*,#13448,.F.);
#17722=ORIENTED_EDGE('',*,*,#13445,.T.);
#17723=ORIENTED_EDGE('',*,*,#13449,.T.);
#17724=ORIENTED_EDGE('',*,*,#13450,.F.);
#17725=ORIENTED_EDGE('',*,*,#13446,.F.);
#17726=ORIENTED_EDGE('',*,*,#13451,.T.);
#17727=ORIENTED_EDGE('',*,*,#13444,.F.);
#17728=ORIENTED_EDGE('',*,*,#13452,.F.);
#17729=ORIENTED_EDGE('',*,*,#13453,.T.);
#17730=ORIENTED_EDGE('',*,*,#13451,.F.);
#17731=ORIENTED_EDGE('',*,*,#13442,.T.);
#17732=ORIENTED_EDGE('',*,*,#13454,.F.);
#17733=ORIENTED_EDGE('',*,*,#13455,.T.);
#17734=ORIENTED_EDGE('',*,*,#13452,.T.);
#17735=ORIENTED_EDGE('',*,*,#13455,.F.);
#17736=ORIENTED_EDGE('',*,*,#13456,.F.);
#17737=ORIENTED_EDGE('',*,*,#13457,.F.);
#17738=ORIENTED_EDGE('',*,*,#13453,.F.);
#17739=ORIENTED_EDGE('',*,*,#13457,.T.);
#17740=ORIENTED_EDGE('',*,*,#13458,.T.);
#17741=ORIENTED_EDGE('',*,*,#13459,.F.);
#17742=ORIENTED_EDGE('',*,*,#13460,.T.);
#17743=ORIENTED_EDGE('',*,*,#13461,.F.);
#17744=ORIENTED_EDGE('',*,*,#13449,.F.);
#17745=ORIENTED_EDGE('',*,*,#13459,.T.);
#17746=ORIENTED_EDGE('',*,*,#13462,.T.);
#17747=ORIENTED_EDGE('',*,*,#13463,.F.);
#17748=ORIENTED_EDGE('',*,*,#13464,.F.);
#17749=ORIENTED_EDGE('',*,*,#13465,.T.);
#17750=ORIENTED_EDGE('',*,*,#13466,.F.);
#17751=ORIENTED_EDGE('',*,*,#13467,.T.);
#17752=ORIENTED_EDGE('',*,*,#13468,.T.);
#17753=ORIENTED_EDGE('',*,*,#13465,.F.);
#17754=ORIENTED_EDGE('',*,*,#13469,.T.);
#17755=ORIENTED_EDGE('',*,*,#13470,.T.);
#17756=ORIENTED_EDGE('',*,*,#13471,.T.);
#17757=ORIENTED_EDGE('',*,*,#13472,.F.);
#17758=ORIENTED_EDGE('',*,*,#13467,.F.);
#17759=ORIENTED_EDGE('',*,*,#13471,.F.);
#17760=ORIENTED_EDGE('',*,*,#13473,.F.);
#17761=ORIENTED_EDGE('',*,*,#13473,.T.);
#17762=ORIENTED_EDGE('',*,*,#13474,.F.);
#17763=ORIENTED_EDGE('',*,*,#13475,.T.);
#17764=ORIENTED_EDGE('',*,*,#13476,.T.);
#17765=ORIENTED_EDGE('',*,*,#13468,.F.);
#17766=ORIENTED_EDGE('',*,*,#13476,.F.);
#17767=ORIENTED_EDGE('',*,*,#13477,.T.);
#17768=ORIENTED_EDGE('',*,*,#13478,.F.);
#17769=ORIENTED_EDGE('',*,*,#13479,.T.);
#17770=ORIENTED_EDGE('',*,*,#13480,.F.);
#17771=ORIENTED_EDGE('',*,*,#13462,.F.);
#17772=ORIENTED_EDGE('',*,*,#13478,.T.);
#17773=ORIENTED_EDGE('',*,*,#13481,.T.);
#17774=ORIENTED_EDGE('',*,*,#13482,.F.);
#17775=ORIENTED_EDGE('',*,*,#13479,.F.);
#17776=ORIENTED_EDGE('',*,*,#13483,.T.);
#17777=ORIENTED_EDGE('',*,*,#13477,.F.);
#17778=ORIENTED_EDGE('',*,*,#13484,.T.);
#17779=ORIENTED_EDGE('',*,*,#13485,.T.);
#17780=ORIENTED_EDGE('',*,*,#13483,.F.);
#17781=ORIENTED_EDGE('',*,*,#13475,.F.);
#17782=ORIENTED_EDGE('',*,*,#13486,.F.);
#17783=ORIENTED_EDGE('',*,*,#13484,.F.);
#17784=ORIENTED_EDGE('',*,*,#13487,.T.);
#17785=ORIENTED_EDGE('',*,*,#13488,.F.);
#17786=ORIENTED_EDGE('',*,*,#13489,.F.);
#17787=ORIENTED_EDGE('',*,*,#13490,.T.);
#17788=ORIENTED_EDGE('',*,*,#13491,.T.);
#17789=ORIENTED_EDGE('',*,*,#13492,.T.);
#17790=ORIENTED_EDGE('',*,*,#13493,.F.);
#17791=ORIENTED_EDGE('',*,*,#13490,.F.);
#17792=ORIENTED_EDGE('',*,*,#13494,.F.);
#17793=ORIENTED_EDGE('',*,*,#13492,.F.);
#17794=ORIENTED_EDGE('',*,*,#13495,.F.);
#17795=ORIENTED_EDGE('',*,*,#13486,.T.);
#17796=ORIENTED_EDGE('',*,*,#13496,.F.);
#17797=ORIENTED_EDGE('',*,*,#13495,.T.);
#17798=ORIENTED_EDGE('',*,*,#13497,.T.);
#17799=ORIENTED_EDGE('',*,*,#13474,.T.);
#17800=ORIENTED_EDGE('',*,*,#13470,.F.);
#17801=ORIENTED_EDGE('',*,*,#13498,.F.);
#17802=ORIENTED_EDGE('',*,*,#13496,.T.);
#17803=ORIENTED_EDGE('',*,*,#13499,.T.);
#17804=ORIENTED_EDGE('',*,*,#13500,.F.);
#17805=ORIENTED_EDGE('',*,*,#13494,.T.);
#17806=ORIENTED_EDGE('',*,*,#13498,.T.);
#17807=ORIENTED_EDGE('',*,*,#13469,.F.);
#17808=ORIENTED_EDGE('',*,*,#13501,.F.);
#17809=ORIENTED_EDGE('',*,*,#13499,.F.);
#17810=ORIENTED_EDGE('',*,*,#13502,.T.);
#17811=ORIENTED_EDGE('',*,*,#13503,.F.);
#17812=ORIENTED_EDGE('',*,*,#13504,.F.);
#17813=ORIENTED_EDGE('',*,*,#13505,.T.);
#17814=ORIENTED_EDGE('',*,*,#13506,.T.);
#17815=ORIENTED_EDGE('',*,*,#13501,.T.);
#17816=ORIENTED_EDGE('',*,*,#13507,.F.);
#17817=ORIENTED_EDGE('',*,*,#13505,.F.);
#17818=ORIENTED_EDGE('',*,*,#13493,.T.);
#17819=ORIENTED_EDGE('',*,*,#13500,.T.);
#17820=ORIENTED_EDGE('',*,*,#13506,.F.);
#17821=ORIENTED_EDGE('',*,*,#13508,.F.);
#17822=ORIENTED_EDGE('',*,*,#13504,.T.);
#17823=ORIENTED_EDGE('',*,*,#13509,.F.);
#17824=ORIENTED_EDGE('',*,*,#13487,.F.);
#17825=ORIENTED_EDGE('',*,*,#13508,.T.);
#17826=ORIENTED_EDGE('',*,*,#13510,.T.);
#17827=ORIENTED_EDGE('',*,*,#13511,.F.);
#17828=ORIENTED_EDGE('',*,*,#13244,.T.);
#17829=ORIENTED_EDGE('',*,*,#13261,.T.);
#17830=ORIENTED_EDGE('',*,*,#13263,.T.);
#17831=ORIENTED_EDGE('',*,*,#13512,.F.);
#17832=ORIENTED_EDGE('',*,*,#13241,.T.);
#17833=ORIENTED_EDGE('',*,*,#13513,.T.);
#17834=ORIENTED_EDGE('',*,*,#13284,.T.);
#17835=ORIENTED_EDGE('',*,*,#13514,.F.);
#17836=ORIENTED_EDGE('',*,*,#13292,.T.);
#17837=ORIENTED_EDGE('',*,*,#13309,.T.);
#17838=ORIENTED_EDGE('',*,*,#13311,.T.);
#17839=ORIENTED_EDGE('',*,*,#13515,.F.);
#17840=ORIENTED_EDGE('',*,*,#13269,.T.);
#17841=ORIENTED_EDGE('',*,*,#13290,.T.);
#17842=ORIENTED_EDGE('',*,*,#13332,.T.);
#17843=ORIENTED_EDGE('',*,*,#13516,.F.);
#17844=ORIENTED_EDGE('',*,*,#13340,.T.);
#17845=ORIENTED_EDGE('',*,*,#13357,.T.);
#17846=ORIENTED_EDGE('',*,*,#13359,.T.);
#17847=ORIENTED_EDGE('',*,*,#13517,.F.);
#17848=ORIENTED_EDGE('',*,*,#13317,.T.);
#17849=ORIENTED_EDGE('',*,*,#13338,.T.);
#17850=ORIENTED_EDGE('',*,*,#13380,.T.);
#17851=ORIENTED_EDGE('',*,*,#13518,.F.);
#17852=ORIENTED_EDGE('',*,*,#13388,.T.);
#17853=ORIENTED_EDGE('',*,*,#13405,.T.);
#17854=ORIENTED_EDGE('',*,*,#13407,.T.);
#17855=ORIENTED_EDGE('',*,*,#13519,.F.);
#17856=ORIENTED_EDGE('',*,*,#13365,.T.);
#17857=ORIENTED_EDGE('',*,*,#13386,.T.);
#17858=ORIENTED_EDGE('',*,*,#13428,.T.);
#17859=ORIENTED_EDGE('',*,*,#13520,.F.);
#17860=ORIENTED_EDGE('',*,*,#13463,.T.);
#17861=ORIENTED_EDGE('',*,*,#13480,.T.);
#17862=ORIENTED_EDGE('',*,*,#13482,.T.);
#17863=ORIENTED_EDGE('',*,*,#13521,.F.);
#17864=ORIENTED_EDGE('',*,*,#13413,.T.);
#17865=ORIENTED_EDGE('',*,*,#13434,.T.);
#17866=ORIENTED_EDGE('',*,*,#13503,.T.);
#17867=ORIENTED_EDGE('',*,*,#13522,.F.);
#17868=ORIENTED_EDGE('',*,*,#13447,.T.);
#17869=ORIENTED_EDGE('',*,*,#13450,.T.);
#17870=ORIENTED_EDGE('',*,*,#13461,.T.);
#17871=ORIENTED_EDGE('',*,*,#13523,.F.);
#17872=ORIENTED_EDGE('',*,*,#13488,.T.);
#17873=ORIENTED_EDGE('',*,*,#13509,.T.);
#17874=ORIENTED_EDGE('',*,*,#13524,.T.);
#17875=ORIENTED_EDGE('',*,*,#13525,.T.);
#17876=ORIENTED_EDGE('',*,*,#13526,.T.);
#17877=ORIENTED_EDGE('',*,*,#13524,.F.);
#17878=ORIENTED_EDGE('',*,*,#13526,.F.);
#17879=ORIENTED_EDGE('',*,*,#13527,.T.);
#17880=ORIENTED_EDGE('',*,*,#13528,.T.);
#17881=ORIENTED_EDGE('',*,*,#13529,.T.);
#17882=ORIENTED_EDGE('',*,*,#13527,.F.);
#17883=ORIENTED_EDGE('',*,*,#13529,.F.);
#17884=ORIENTED_EDGE('',*,*,#13262,.F.);
#17885=ORIENTED_EDGE('',*,*,#13266,.F.);
#17886=ORIENTED_EDGE('',*,*,#13278,.F.);
#17887=ORIENTED_EDGE('',*,*,#13272,.F.);
#17888=ORIENTED_EDGE('',*,*,#13270,.T.);
#17889=ORIENTED_EDGE('',*,*,#13515,.T.);
#17890=ORIENTED_EDGE('',*,*,#13310,.F.);
#17891=ORIENTED_EDGE('',*,*,#13314,.F.);
#17892=ORIENTED_EDGE('',*,*,#13326,.F.);
#17893=ORIENTED_EDGE('',*,*,#13320,.F.);
#17894=ORIENTED_EDGE('',*,*,#13318,.T.);
#17895=ORIENTED_EDGE('',*,*,#13517,.T.);
#17896=ORIENTED_EDGE('',*,*,#13358,.F.);
#17897=ORIENTED_EDGE('',*,*,#13362,.F.);
#17898=ORIENTED_EDGE('',*,*,#13374,.F.);
#17899=ORIENTED_EDGE('',*,*,#13368,.F.);
#17900=ORIENTED_EDGE('',*,*,#13366,.T.);
#17901=ORIENTED_EDGE('',*,*,#13519,.T.);
#17902=ORIENTED_EDGE('',*,*,#13406,.F.);
#17903=ORIENTED_EDGE('',*,*,#13410,.F.);
#17904=ORIENTED_EDGE('',*,*,#13422,.F.);
#17905=ORIENTED_EDGE('',*,*,#13416,.F.);
#17906=ORIENTED_EDGE('',*,*,#13414,.T.);
#17907=ORIENTED_EDGE('',*,*,#13521,.T.);
#17908=ORIENTED_EDGE('',*,*,#13481,.F.);
#17909=ORIENTED_EDGE('',*,*,#13485,.F.);
#17910=ORIENTED_EDGE('',*,*,#13497,.F.);
#17911=ORIENTED_EDGE('',*,*,#13491,.F.);
#17912=ORIENTED_EDGE('',*,*,#13489,.T.);
#17913=ORIENTED_EDGE('',*,*,#13523,.T.);
#17914=ORIENTED_EDGE('',*,*,#13460,.F.);
#17915=ORIENTED_EDGE('',*,*,#13458,.F.);
#17916=ORIENTED_EDGE('',*,*,#13530,.F.);
#17917=ORIENTED_EDGE('',*,*,#13237,.F.);
#17918=ORIENTED_EDGE('',*,*,#13242,.T.);
#17919=ORIENTED_EDGE('',*,*,#13512,.T.);
#17920=ORIENTED_EDGE('',*,*,#13230,.T.);
#17921=ORIENTED_EDGE('',*,*,#13232,.F.);
#17922=ORIENTED_EDGE('',*,*,#13528,.F.);
#17923=ORIENTED_EDGE('',*,*,#13525,.F.);
#17924=ORIENTED_EDGE('',*,*,#13456,.T.);
#17925=ORIENTED_EDGE('',*,*,#13531,.F.);
#17926=ORIENTED_EDGE('',*,*,#13236,.T.);
#17927=ORIENTED_EDGE('',*,*,#13530,.T.);
#17928=ORIENTED_EDGE('',*,*,#13454,.T.);
#17929=ORIENTED_EDGE('',*,*,#13438,.F.);
#17930=ORIENTED_EDGE('',*,*,#13532,.F.);
#17931=ORIENTED_EDGE('',*,*,#13531,.T.);
#17932=ORIENTED_EDGE('',*,*,#13437,.T.);
#17933=ORIENTED_EDGE('',*,*,#13533,.F.);
#17934=ORIENTED_EDGE('',*,*,#13234,.T.);
#17935=ORIENTED_EDGE('',*,*,#13532,.T.);
#17936=ORIENTED_EDGE('',*,*,#13238,.T.);
#17937=ORIENTED_EDGE('',*,*,#13533,.T.);
#17938=ORIENTED_EDGE('',*,*,#13534,.F.);
#17939=ORIENTED_EDGE('',*,*,#13535,.F.);
#17940=ORIENTED_EDGE('',*,*,#13536,.T.);
#17941=ORIENTED_EDGE('',*,*,#13513,.F.);
#17942=ORIENTED_EDGE('',*,*,#13240,.F.);
#17943=ORIENTED_EDGE('',*,*,#13535,.T.);
#17944=ORIENTED_EDGE('',*,*,#13537,.T.);
#17945=ORIENTED_EDGE('',*,*,#13510,.F.);
#17946=ORIENTED_EDGE('',*,*,#13536,.F.);
#17947=ORIENTED_EDGE('',*,*,#13538,.T.);
#17948=ORIENTED_EDGE('',*,*,#13534,.T.);
#17949=ORIENTED_EDGE('',*,*,#13436,.T.);
#17950=ORIENTED_EDGE('',*,*,#13539,.F.);
#17951=ORIENTED_EDGE('',*,*,#13538,.F.);
#17952=ORIENTED_EDGE('',*,*,#13540,.F.);
#17953=ORIENTED_EDGE('',*,*,#13540,.T.);
#17954=ORIENTED_EDGE('',*,*,#13541,.T.);
#17955=ORIENTED_EDGE('',*,*,#13542,.F.);
#17956=ORIENTED_EDGE('',*,*,#13541,.F.);
#17957=ORIENTED_EDGE('',*,*,#13543,.F.);
#17958=ORIENTED_EDGE('',*,*,#13543,.T.);
#17959=ORIENTED_EDGE('',*,*,#13544,.T.);
#17960=ORIENTED_EDGE('',*,*,#13545,.F.);
#17961=ORIENTED_EDGE('',*,*,#13544,.F.);
#17962=ORIENTED_EDGE('',*,*,#13440,.T.);
#17963=ORIENTED_EDGE('',*,*,#13443,.T.);
#17964=ORIENTED_EDGE('',*,*,#13448,.T.);
#17965=ORIENTED_EDGE('',*,*,#13522,.T.);
#17966=ORIENTED_EDGE('',*,*,#13502,.F.);
#17967=ORIENTED_EDGE('',*,*,#13507,.T.);
#17968=ORIENTED_EDGE('',*,*,#13472,.T.);
#17969=ORIENTED_EDGE('',*,*,#13466,.T.);
#17970=ORIENTED_EDGE('',*,*,#13464,.T.);
#17971=ORIENTED_EDGE('',*,*,#13520,.T.);
#17972=ORIENTED_EDGE('',*,*,#13427,.F.);
#17973=ORIENTED_EDGE('',*,*,#13432,.T.);
#17974=ORIENTED_EDGE('',*,*,#13397,.T.);
#17975=ORIENTED_EDGE('',*,*,#13391,.T.);
#17976=ORIENTED_EDGE('',*,*,#13389,.T.);
#17977=ORIENTED_EDGE('',*,*,#13518,.T.);
#17978=ORIENTED_EDGE('',*,*,#13379,.F.);
#17979=ORIENTED_EDGE('',*,*,#13384,.T.);
#17980=ORIENTED_EDGE('',*,*,#13349,.T.);
#17981=ORIENTED_EDGE('',*,*,#13343,.T.);
#17982=ORIENTED_EDGE('',*,*,#13341,.T.);
#17983=ORIENTED_EDGE('',*,*,#13516,.T.);
#17984=ORIENTED_EDGE('',*,*,#13331,.F.);
#17985=ORIENTED_EDGE('',*,*,#13336,.T.);
#17986=ORIENTED_EDGE('',*,*,#13301,.T.);
#17987=ORIENTED_EDGE('',*,*,#13295,.T.);
#17988=ORIENTED_EDGE('',*,*,#13293,.T.);
#17989=ORIENTED_EDGE('',*,*,#13514,.T.);
#17990=ORIENTED_EDGE('',*,*,#13283,.F.);
#17991=ORIENTED_EDGE('',*,*,#13288,.T.);
#17992=ORIENTED_EDGE('',*,*,#13253,.T.);
#17993=ORIENTED_EDGE('',*,*,#13247,.T.);
#17994=ORIENTED_EDGE('',*,*,#13245,.T.);
#17995=ORIENTED_EDGE('',*,*,#13511,.T.);
#17996=ORIENTED_EDGE('',*,*,#13537,.F.);
#17997=ORIENTED_EDGE('',*,*,#13539,.T.);
#17998=ORIENTED_EDGE('',*,*,#13228,.F.);
#17999=ORIENTED_EDGE('',*,*,#13227,.T.);
#18000=ORIENTED_EDGE('',*,*,#13545,.T.);
#18001=ORIENTED_EDGE('',*,*,#13542,.T.);
#22838=CYLINDRICAL_SURFACE('',#25473,1.5);
#22839=CYLINDRICAL_SURFACE('',#25475,9.);
#22840=CYLINDRICAL_SURFACE('',#25480,1.5);
#22841=CYLINDRICAL_SURFACE('',#25626,1.5);
#22842=CYLINDRICAL_SURFACE('',#25630,1.5);
#22843=CYLINDRICAL_SURFACE('',#25637,1.5);
#22844=CYLINDRICAL_SURFACE('',#25641,1.5);
#23467=ADVANCED_FACE('',(#2475),#1533,.F.);
#23468=ADVANCED_FACE('',(#2476),#22838,.T.);
#23469=ADVANCED_FACE('',(#2477),#22839,.F.);
#23470=ADVANCED_FACE('',(#2478),#1534,.T.);
#23471=ADVANCED_FACE('',(#2479),#22840,.T.);
#23472=ADVANCED_FACE('',(#2480),#254,.T.);
#23473=ADVANCED_FACE('',(#2481),#162,.T.);
#23474=ADVANCED_FACE('',(#2482),#163,.F.);
#23475=ADVANCED_FACE('',(#2483),#164,.F.);
#23476=ADVANCED_FACE('',(#2484),#165,.T.);
#23477=ADVANCED_FACE('',(#2485),#166,.T.);
#23478=ADVANCED_FACE('',(#2486),#255,.T.);
#23479=ADVANCED_FACE('',(#2487),#167,.T.);
#23480=ADVANCED_FACE('',(#2488),#36,.T.);
#23481=ADVANCED_FACE('',(#2489),#168,.F.);
#23482=ADVANCED_FACE('',(#2490),#169,.F.);
#23483=ADVANCED_FACE('',(#2491),#170,.T.);
#23484=ADVANCED_FACE('',(#2492),#256,.T.);
#23485=ADVANCED_FACE('',(#2493),#171,.F.);
#23486=ADVANCED_FACE('',(#2494),#172,.T.);
#23487=ADVANCED_FACE('',(#2495),#257,.T.);
#23488=ADVANCED_FACE('',(#2496),#173,.T.);
#23489=ADVANCED_FACE('',(#2497),#37,.T.);
#23490=ADVANCED_FACE('',(#2498),#174,.T.);
#23491=ADVANCED_FACE('',(#2499),#258,.T.);
#23492=ADVANCED_FACE('',(#2500),#175,.F.);
#23493=ADVANCED_FACE('',(#2501),#176,.T.);
#23494=ADVANCED_FACE('',(#2502),#38,.T.);
#23495=ADVANCED_FACE('',(#2503),#177,.F.);
#23496=ADVANCED_FACE('',(#2504),#178,.F.);
#23497=ADVANCED_FACE('',(#2505),#179,.T.);
#23498=ADVANCED_FACE('',(#2506),#180,.T.);
#23499=ADVANCED_FACE('',(#2507),#259,.T.);
#23500=ADVANCED_FACE('',(#2508),#181,.T.);
#23501=ADVANCED_FACE('',(#2509),#39,.T.);
#23502=ADVANCED_FACE('',(#2510),#182,.F.);
#23503=ADVANCED_FACE('',(#2511),#183,.F.);
#23504=ADVANCED_FACE('',(#2512),#184,.T.);
#23505=ADVANCED_FACE('',(#2513),#260,.T.);
#23506=ADVANCED_FACE('',(#2514),#185,.F.);
#23507=ADVANCED_FACE('',(#2515),#186,.T.);
#23508=ADVANCED_FACE('',(#2516),#261,.T.);
#23509=ADVANCED_FACE('',(#2517),#187,.T.);
#23510=ADVANCED_FACE('',(#2518),#40,.T.);
#23511=ADVANCED_FACE('',(#2519),#188,.T.);
#23512=ADVANCED_FACE('',(#2520),#262,.T.);
#23513=ADVANCED_FACE('',(#2521),#189,.F.);
#23514=ADVANCED_FACE('',(#2522),#190,.T.);
#23515=ADVANCED_FACE('',(#2523),#41,.T.);
#23516=ADVANCED_FACE('',(#2524),#191,.F.);
#23517=ADVANCED_FACE('',(#2525),#192,.F.);
#23518=ADVANCED_FACE('',(#2526),#193,.T.);
#23519=ADVANCED_FACE('',(#2527),#194,.T.);
#23520=ADVANCED_FACE('',(#2528),#263,.T.);
#23521=ADVANCED_FACE('',(#2529),#195,.T.);
#23522=ADVANCED_FACE('',(#2530),#42,.T.);
#23523=ADVANCED_FACE('',(#2531),#196,.F.);
#23524=ADVANCED_FACE('',(#2532),#197,.F.);
#23525=ADVANCED_FACE('',(#2533),#198,.T.);
#23526=ADVANCED_FACE('',(#2534),#264,.T.);
#23527=ADVANCED_FACE('',(#2535),#199,.F.);
#23528=ADVANCED_FACE('',(#2536),#200,.T.);
#23529=ADVANCED_FACE('',(#2537),#265,.T.);
#23530=ADVANCED_FACE('',(#2538),#201,.T.);
#23531=ADVANCED_FACE('',(#2539),#43,.T.);
#23532=ADVANCED_FACE('',(#2540),#202,.T.);
#23533=ADVANCED_FACE('',(#2541),#266,.T.);
#23534=ADVANCED_FACE('',(#2542),#203,.F.);
#23535=ADVANCED_FACE('',(#2543),#204,.T.);
#23536=ADVANCED_FACE('',(#2544),#44,.T.);
#23537=ADVANCED_FACE('',(#2545),#205,.F.);
#23538=ADVANCED_FACE('',(#2546),#206,.F.);
#23539=ADVANCED_FACE('',(#2547),#207,.T.);
#23540=ADVANCED_FACE('',(#2548),#208,.T.);
#23541=ADVANCED_FACE('',(#2549),#267,.T.);
#23542=ADVANCED_FACE('',(#2550),#209,.T.);
#23543=ADVANCED_FACE('',(#2551),#45,.T.);
#23544=ADVANCED_FACE('',(#2552),#210,.F.);
#23545=ADVANCED_FACE('',(#2553),#211,.F.);
#23546=ADVANCED_FACE('',(#2554),#212,.T.);
#23547=ADVANCED_FACE('',(#2555),#268,.T.);
#23548=ADVANCED_FACE('',(#2556),#213,.F.);
#23549=ADVANCED_FACE('',(#2557),#214,.T.);
#23550=ADVANCED_FACE('',(#2558),#269,.T.);
#23551=ADVANCED_FACE('',(#2559),#215,.T.);
#23552=ADVANCED_FACE('',(#2560),#46,.T.);
#23553=ADVANCED_FACE('',(#2561),#216,.T.);
#23554=ADVANCED_FACE('',(#2562),#270,.T.);
#23555=ADVANCED_FACE('',(#2563),#217,.F.);
#23556=ADVANCED_FACE('',(#2564),#218,.T.);
#23557=ADVANCED_FACE('',(#2565),#47,.T.);
#23558=ADVANCED_FACE('',(#2566),#219,.F.);
#23559=ADVANCED_FACE('',(#2567),#271,.T.);
#23560=ADVANCED_FACE('',(#2568),#220,.T.);
#23561=ADVANCED_FACE('',(#2569),#272,.T.);
#23562=ADVANCED_FACE('',(#2570),#221,.T.);
#23563=ADVANCED_FACE('',(#2571),#222,.F.);
#23564=ADVANCED_FACE('',(#2572),#223,.F.);
#23565=ADVANCED_FACE('',(#2573),#48,.T.);
#23566=ADVANCED_FACE('',(#2574),#224,.T.);
#23567=ADVANCED_FACE('',(#2575),#273,.T.);
#23568=ADVANCED_FACE('',(#2576),#225,.T.);
#23569=ADVANCED_FACE('',(#2577),#226,.F.);
#23570=ADVANCED_FACE('',(#2578),#227,.F.);
#23571=ADVANCED_FACE('',(#2579),#228,.T.);
#23572=ADVANCED_FACE('',(#2580),#229,.T.);
#23573=ADVANCED_FACE('',(#2581),#274,.T.);
#23574=ADVANCED_FACE('',(#2582),#230,.T.);
#23575=ADVANCED_FACE('',(#2583),#49,.T.);
#23576=ADVANCED_FACE('',(#2584),#231,.F.);
#23577=ADVANCED_FACE('',(#2585),#232,.F.);
#23578=ADVANCED_FACE('',(#2586),#233,.T.);
#23579=ADVANCED_FACE('',(#2587),#275,.T.);
#23580=ADVANCED_FACE('',(#2588),#234,.F.);
#23581=ADVANCED_FACE('',(#2589),#235,.T.);
#23582=ADVANCED_FACE('',(#2590),#276,.T.);
#23583=ADVANCED_FACE('',(#2591),#236,.T.);
#23584=ADVANCED_FACE('',(#2592),#50,.T.);
#23585=ADVANCED_FACE('',(#2593),#237,.T.);
#23586=ADVANCED_FACE('',(#2594),#277,.T.);
#23587=ADVANCED_FACE('',(#2595),#238,.F.);
#23588=ADVANCED_FACE('',(#2596),#239,.T.);
#23589=ADVANCED_FACE('',(#2597),#51,.T.);
#23590=ADVANCED_FACE('',(#2598),#240,.F.);
#23591=ADVANCED_FACE('',(#2599),#241,.F.);
#23592=ADVANCED_FACE('',(#2600),#242,.F.);
#23593=ADVANCED_FACE('',(#2601),#243,.F.);
#23594=ADVANCED_FACE('',(#2602),#244,.F.);
#23595=ADVANCED_FACE('',(#2603),#245,.F.);
#23596=ADVANCED_FACE('',(#2604),#246,.F.);
#23597=ADVANCED_FACE('',(#2605),#1535,.T.);
#23598=ADVANCED_FACE('',(#2606),#22841,.T.);
#23599=ADVANCED_FACE('',(#2607),#1536,.T.);
#23600=ADVANCED_FACE('',(#2608),#22842,.T.);
#23601=ADVANCED_FACE('',(#2609,#1130,#1131,#1132,#1133),#1537,.F.);
#23602=ADVANCED_FACE('',(#2610),#247,.T.);
#23603=ADVANCED_FACE('',(#2611),#52,.T.);
#23604=ADVANCED_FACE('',(#2612),#248,.T.);
#23605=ADVANCED_FACE('',(#2613),#53,.T.);
#23606=ADVANCED_FACE('',(#2614),#249,.F.);
#23607=ADVANCED_FACE('',(#2615),#250,.F.);
#23608=ADVANCED_FACE('',(#2616),#251,.T.);
#23609=ADVANCED_FACE('',(#2617),#1538,.F.);
#23610=ADVANCED_FACE('',(#2618),#22843,.T.);
#23611=ADVANCED_FACE('',(#2619),#1539,.F.);
#23612=ADVANCED_FACE('',(#2620),#22844,.T.);
#23613=ADVANCED_FACE('',(#2621,#1134,#1135,#1136,#1137),#1540,.T.);
#24539=CLOSED_SHELL('',(#23467,#23468,#23469,#23470,#23471,#23472,#23473,
#23474,#23475,#23476,#23477,#23478,#23479,#23480,#23481,#23482,#23483,#23484,
#23485,#23486,#23487,#23488,#23489,#23490,#23491,#23492,#23493,#23494,#23495,
#23496,#23497,#23498,#23499,#23500,#23501,#23502,#23503,#23504,#23505,#23506,
#23507,#23508,#23509,#23510,#23511,#23512,#23513,#23514,#23515,#23516,#23517,
#23518,#23519,#23520,#23521,#23522,#23523,#23524,#23525,#23526,#23527,#23528,
#23529,#23530,#23531,#23532,#23533,#23534,#23535,#23536,#23537,#23538,#23539,
#23540,#23541,#23542,#23543,#23544,#23545,#23546,#23547,#23548,#23549,#23550,
#23551,#23552,#23553,#23554,#23555,#23556,#23557,#23558,#23559,#23560,#23561,
#23562,#23563,#23564,#23565,#23566,#23567,#23568,#23569,#23570,#23571,#23572,
#23573,#23574,#23575,#23576,#23577,#23578,#23579,#23580,#23581,#23582,#23583,
#23584,#23585,#23586,#23587,#23588,#23589,#23590,#23591,#23592,#23593,#23594,
#23595,#23596,#23597,#23598,#23599,#23600,#23601,#23602,#23603,#23604,#23605,
#23606,#23607,#23608,#23609,#23610,#23611,#23612,#23613));
#25470=AXIS2_PLACEMENT_3D('',#36395,#29113,#29114);
#25471=AXIS2_PLACEMENT_3D('',#36396,#29115,#29116);
#25472=AXIS2_PLACEMENT_3D('',#36398,#29117,#29118);
#25473=AXIS2_PLACEMENT_3D('',#36399,#29119,#29120);
#25474=AXIS2_PLACEMENT_3D('',#36402,#29122,#29123);
#25475=AXIS2_PLACEMENT_3D('',#36403,#29124,#29125);
#25476=AXIS2_PLACEMENT_3D('',#36405,#29126,#29127);
#25477=AXIS2_PLACEMENT_3D('',#36408,#29129,#29130);
#25478=AXIS2_PLACEMENT_3D('',#36409,#29131,#29132);
#25479=AXIS2_PLACEMENT_3D('',#36411,#29133,#29134);
#25480=AXIS2_PLACEMENT_3D('',#36412,#29135,#29136);
#25481=AXIS2_PLACEMENT_3D('',#36414,#29137,#29138);
#25482=AXIS2_PLACEMENT_3D('',#36416,#29140,#29141);
#25483=AXIS2_PLACEMENT_3D('',#36419,#29142,#29143);
#25484=AXIS2_PLACEMENT_3D('',#36421,#29144,#29145);
#25485=AXIS2_PLACEMENT_3D('',#36422,#29146,#29147);
#25486=AXIS2_PLACEMENT_3D('',#36592,#29148,#29149);
#25487=AXIS2_PLACEMENT_3D('',#36679,#29150,#29151);
#25488=AXIS2_PLACEMENT_3D('',#36906,#29152,#29153);
#25489=AXIS2_PLACEMENT_3D('',#36965,#29154,#29155);
#25490=AXIS2_PLACEMENT_3D('',#36967,#29156,#29157);
#25491=AXIS2_PLACEMENT_3D('',#36968,#29158,#29159);
#25492=AXIS2_PLACEMENT_3D('',#36979,#29160,#29161);
#25493=AXIS2_PLACEMENT_3D('',#36980,#29162,#29163);
#25494=AXIS2_PLACEMENT_3D('',#37204,#29164,#29165);
#25495=AXIS2_PLACEMENT_3D('',#37540,#29166,#29167);
#25496=AXIS2_PLACEMENT_3D('',#37831,#29168,#29169);
#25497=AXIS2_PLACEMENT_3D('',#37854,#29170,#29171);
#25498=AXIS2_PLACEMENT_3D('',#37855,#29172,#29173);
#25499=AXIS2_PLACEMENT_3D('',#37894,#29174,#29175);
#25500=AXIS2_PLACEMENT_3D('',#38069,#29176,#29177);
#25501=AXIS2_PLACEMENT_3D('',#38080,#29178,#29179);
#25502=AXIS2_PLACEMENT_3D('',#38082,#29180,#29181);
#25503=AXIS2_PLACEMENT_3D('',#38083,#29182,#29183);
#25504=AXIS2_PLACEMENT_3D('',#38108,#29184,#29185);
#25505=AXIS2_PLACEMENT_3D('',#38508,#29186,#29187);
#25506=AXIS2_PLACEMENT_3D('',#38630,#29188,#29189);
#25507=AXIS2_PLACEMENT_3D('',#38631,#29190,#29191);
#25508=AXIS2_PLACEMENT_3D('',#38728,#29192,#29193);
#25509=AXIS2_PLACEMENT_3D('',#39211,#29194,#29195);
#25510=AXIS2_PLACEMENT_3D('',#39438,#29196,#29197);
#25511=AXIS2_PLACEMENT_3D('',#39497,#29198,#29199);
#25512=AXIS2_PLACEMENT_3D('',#39499,#29200,#29201);
#25513=AXIS2_PLACEMENT_3D('',#39500,#29202,#29203);
#25514=AXIS2_PLACEMENT_3D('',#39511,#29204,#29205);
#25515=AXIS2_PLACEMENT_3D('',#39512,#29206,#29207);
#25516=AXIS2_PLACEMENT_3D('',#39734,#29208,#29209);
#25517=AXIS2_PLACEMENT_3D('',#40070,#29210,#29211);
#25518=AXIS2_PLACEMENT_3D('',#40370,#29212,#29213);
#25519=AXIS2_PLACEMENT_3D('',#40393,#29214,#29215);
#25520=AXIS2_PLACEMENT_3D('',#40394,#29216,#29217);
#25521=AXIS2_PLACEMENT_3D('',#40433,#29218,#29219);
#25522=AXIS2_PLACEMENT_3D('',#40608,#29220,#29221);
#25523=AXIS2_PLACEMENT_3D('',#40619,#29222,#29223);
#25524=AXIS2_PLACEMENT_3D('',#40621,#29224,#29225);
#25525=AXIS2_PLACEMENT_3D('',#40622,#29226,#29227);
#25526=AXIS2_PLACEMENT_3D('',#40647,#29228,#29229);
#25527=AXIS2_PLACEMENT_3D('',#41047,#29230,#29231);
#25528=AXIS2_PLACEMENT_3D('',#41169,#29232,#29233);
#25529=AXIS2_PLACEMENT_3D('',#41170,#29234,#29235);
#25530=AXIS2_PLACEMENT_3D('',#41267,#29236,#29237);
#25531=AXIS2_PLACEMENT_3D('',#41771,#29238,#29239);
#25532=AXIS2_PLACEMENT_3D('',#41998,#29240,#29241);
#25533=AXIS2_PLACEMENT_3D('',#42057,#29242,#29243);
#25534=AXIS2_PLACEMENT_3D('',#42059,#29244,#29245);
#25535=AXIS2_PLACEMENT_3D('',#42060,#29246,#29247);
#25536=AXIS2_PLACEMENT_3D('',#42071,#29248,#29249);
#25537=AXIS2_PLACEMENT_3D('',#42072,#29250,#29251);
#25538=AXIS2_PLACEMENT_3D('',#42295,#29252,#29253);
#25539=AXIS2_PLACEMENT_3D('',#42635,#29254,#29255);
#25540=AXIS2_PLACEMENT_3D('',#42908,#29256,#29257);
#25541=AXIS2_PLACEMENT_3D('',#42931,#29258,#29259);
#25542=AXIS2_PLACEMENT_3D('',#42932,#29260,#29261);
#25543=AXIS2_PLACEMENT_3D('',#42971,#29262,#29263);
#25544=AXIS2_PLACEMENT_3D('',#43146,#29264,#29265);
#25545=AXIS2_PLACEMENT_3D('',#43157,#29266,#29267);
#25546=AXIS2_PLACEMENT_3D('',#43159,#29268,#29269);
#25547=AXIS2_PLACEMENT_3D('',#43160,#29270,#29271);
#25548=AXIS2_PLACEMENT_3D('',#43185,#29272,#29273);
#25549=AXIS2_PLACEMENT_3D('',#43585,#29274,#29275);
#25550=AXIS2_PLACEMENT_3D('',#43707,#29276,#29277);
#25551=AXIS2_PLACEMENT_3D('',#43708,#29278,#29279);
#25552=AXIS2_PLACEMENT_3D('',#43805,#29280,#29281);
#25553=AXIS2_PLACEMENT_3D('',#44297,#29282,#29283);
#25554=AXIS2_PLACEMENT_3D('',#44527,#29284,#29285);
#25555=AXIS2_PLACEMENT_3D('',#44586,#29286,#29287);
#25556=AXIS2_PLACEMENT_3D('',#44588,#29288,#29289);
#25557=AXIS2_PLACEMENT_3D('',#44589,#29290,#29291);
#25558=AXIS2_PLACEMENT_3D('',#44600,#29292,#29293);
#25559=AXIS2_PLACEMENT_3D('',#44601,#29294,#29295);
#25560=AXIS2_PLACEMENT_3D('',#44825,#29296,#29297);
#25561=AXIS2_PLACEMENT_3D('',#45161,#29298,#29299);
#25562=AXIS2_PLACEMENT_3D('',#45443,#29300,#29301);
#25563=AXIS2_PLACEMENT_3D('',#45466,#29302,#29303);
#25564=AXIS2_PLACEMENT_3D('',#45467,#29304,#29305);
#25565=AXIS2_PLACEMENT_3D('',#45502,#29306,#29307);
#25566=AXIS2_PLACEMENT_3D('',#45680,#29308,#29309);
#25567=AXIS2_PLACEMENT_3D('',#45691,#29310,#29311);
#25568=AXIS2_PLACEMENT_3D('',#45693,#29312,#29313);
#25569=AXIS2_PLACEMENT_3D('',#45694,#29314,#29315);
#25570=AXIS2_PLACEMENT_3D('',#45719,#29316,#29317);
#25571=AXIS2_PLACEMENT_3D('',#46119,#29318,#29319);
#25572=AXIS2_PLACEMENT_3D('',#46241,#29320,#29321);
#25573=AXIS2_PLACEMENT_3D('',#46242,#29322,#29323);
#25574=AXIS2_PLACEMENT_3D('',#46344,#29324,#29325);
#25575=AXIS2_PLACEMENT_3D('',#46780,#29326,#29327);
#25576=AXIS2_PLACEMENT_3D('',#46783,#29328,#29329);
#25577=AXIS2_PLACEMENT_3D('',#46785,#29330,#29331);
#25578=AXIS2_PLACEMENT_3D('',#46786,#29332,#29333);
#25579=AXIS2_PLACEMENT_3D('',#46804,#29334,#29335);
#25580=AXIS2_PLACEMENT_3D('',#46806,#29336,#29337);
#25581=AXIS2_PLACEMENT_3D('',#46817,#29338,#29339);
#25582=AXIS2_PLACEMENT_3D('',#46819,#29340,#29341);
#25583=AXIS2_PLACEMENT_3D('',#46820,#29342,#29343);
#25584=AXIS2_PLACEMENT_3D('',#47069,#29344,#29345);
#25585=AXIS2_PLACEMENT_3D('',#47160,#29346,#29347);
#25586=AXIS2_PLACEMENT_3D('',#47686,#29348,#29349);
#25587=AXIS2_PLACEMENT_3D('',#47687,#29350,#29351);
#25588=AXIS2_PLACEMENT_3D('',#47689,#29352,#29353);
#25589=AXIS2_PLACEMENT_3D('',#47690,#29354,#29355);
#25590=AXIS2_PLACEMENT_3D('',#47937,#29356,#29357);
#25591=AXIS2_PLACEMENT_3D('',#48167,#29358,#29359);
#25592=AXIS2_PLACEMENT_3D('',#48226,#29360,#29361);
#25593=AXIS2_PLACEMENT_3D('',#48228,#29362,#29363);
#25594=AXIS2_PLACEMENT_3D('',#48229,#29364,#29365);
#25595=AXIS2_PLACEMENT_3D('',#48240,#29366,#29367);
#25596=AXIS2_PLACEMENT_3D('',#48241,#29368,#29369);
#25597=AXIS2_PLACEMENT_3D('',#48463,#29370,#29371);
#25598=AXIS2_PLACEMENT_3D('',#48811,#29372,#29373);
#25599=AXIS2_PLACEMENT_3D('',#49111,#29374,#29375);
#25600=AXIS2_PLACEMENT_3D('',#49134,#29376,#29377);
#25601=AXIS2_PLACEMENT_3D('',#49135,#29378,#29379);
#25602=AXIS2_PLACEMENT_3D('',#49174,#29380,#29381);
#25603=AXIS2_PLACEMENT_3D('',#49349,#29382,#29383);
#25604=AXIS2_PLACEMENT_3D('',#49360,#29384,#29385);
#25605=AXIS2_PLACEMENT_3D('',#49362,#29386,#29387);
#25606=AXIS2_PLACEMENT_3D('',#49363,#29388,#29389);
#25607=AXIS2_PLACEMENT_3D('',#49388,#29390,#29391);
#25608=AXIS2_PLACEMENT_3D('',#49788,#29392,#29393);
#25609=AXIS2_PLACEMENT_3D('',#49910,#29394,#29395);
#25610=AXIS2_PLACEMENT_3D('',#49911,#29396,#29397);
#25611=AXIS2_PLACEMENT_3D('',#50005,#29398,#29399);
#25612=AXIS2_PLACEMENT_3D('',#50501,#29400,#29401);
#25613=AXIS2_PLACEMENT_3D('',#50502,#29402,#29403);
#25614=AXIS2_PLACEMENT_3D('',#50606,#29404,#29405);
#25615=AXIS2_PLACEMENT_3D('',#50607,#29406,#29407);
#25616=AXIS2_PLACEMENT_3D('',#50617,#29408,#29409);
#25617=AXIS2_PLACEMENT_3D('',#50618,#29410,#29411);
#25618=AXIS2_PLACEMENT_3D('',#50628,#29412,#29413);
#25619=AXIS2_PLACEMENT_3D('',#50629,#29414,#29415);
#25620=AXIS2_PLACEMENT_3D('',#50639,#29416,#29417);
#25621=AXIS2_PLACEMENT_3D('',#50640,#29418,#29419);
#25622=AXIS2_PLACEMENT_3D('',#50650,#29420,#29421);
#25623=AXIS2_PLACEMENT_3D('',#50651,#29422,#29423);
#25624=AXIS2_PLACEMENT_3D('',#50652,#29424,#29425);
#25625=AXIS2_PLACEMENT_3D('',#50654,#29426,#29427);
#25626=AXIS2_PLACEMENT_3D('',#50655,#29428,#29429);
#25627=AXIS2_PLACEMENT_3D('',#50657,#29430,#29431);
#25628=AXIS2_PLACEMENT_3D('',#50659,#29433,#29434);
#25629=AXIS2_PLACEMENT_3D('',#50661,#29435,#29436);
#25630=AXIS2_PLACEMENT_3D('',#50662,#29437,#29438);
#25631=AXIS2_PLACEMENT_3D('',#50664,#29439,#29440);
#25632=AXIS2_PLACEMENT_3D('',#50666,#29442,#29443);
#25633=AXIS2_PLACEMENT_3D('',#50704,#29444,#29445);
#25634=AXIS2_PLACEMENT_3D('',#51386,#29446,#29447);
#25635=AXIS2_PLACEMENT_3D('',#51644,#29448,#29449);
#25636=AXIS2_PLACEMENT_3D('',#51646,#29450,#29451);
#25637=AXIS2_PLACEMENT_3D('',#51647,#29452,#29453);
#25638=AXIS2_PLACEMENT_3D('',#51650,#29455,#29456);
#25639=AXIS2_PLACEMENT_3D('',#51651,#29457,#29458);
#25640=AXIS2_PLACEMENT_3D('',#51653,#29459,#29460);
#25641=AXIS2_PLACEMENT_3D('',#51654,#29461,#29462);
#25642=AXIS2_PLACEMENT_3D('',#51657,#29464,#29465);
#25643=AXIS2_PLACEMENT_3D('',#51658,#29466,#29467);
#29113=DIRECTION('axis',(0.,0.,1.));
#29114=DIRECTION('refdir',(1.,0.,0.));
#29115=DIRECTION('center_axis',(-1.,0.,0.));
#29116=DIRECTION('ref_axis',(0.,0.,1.));
#29117=DIRECTION('center_axis',(-1.,0.,0.));
#29118=DIRECTION('ref_axis',(0.,1.,-7.80005689667481E-12));
#29119=DIRECTION('center_axis',(1.,0.,0.));
#29120=DIRECTION('ref_axis',(0.,-1.,7.80005689667481E-12));
#29121=DIRECTION('',(-1.,0.,0.));
#29122=DIRECTION('center_axis',(-1.,0.,0.));
#29123=DIRECTION('ref_axis',(0.,-1.,7.80005689667481E-12));
#29124=DIRECTION('center_axis',(-1.,0.,0.));
#29125=DIRECTION('ref_axis',(0.,0.866025403788329,0.499999999993262));
#29126=DIRECTION('center_axis',(1.,0.,0.));
#29127=DIRECTION('ref_axis',(0.,0.866025403788329,0.499999999993262));
#29128=DIRECTION('',(-1.,0.,0.));
#29129=DIRECTION('center_axis',(1.,0.,0.));
#29130=DIRECTION('ref_axis',(0.,-0.866025403788329,-0.499999999993262));
#29131=DIRECTION('center_axis',(-1.,0.,0.));
#29132=DIRECTION('ref_axis',(0.,0.,1.));
#29133=DIRECTION('center_axis',(-1.,0.,0.));
#29134=DIRECTION('ref_axis',(0.,0.499999999993262,-0.866025403788329));
#29135=DIRECTION('center_axis',(1.,0.,0.));
#29136=DIRECTION('ref_axis',(0.,-0.499999999993262,0.866025403788329));
#29137=DIRECTION('center_axis',(-1.,0.,0.));
#29138=DIRECTION('ref_axis',(0.,-0.499999999993262,0.866025403788329));
#29139=DIRECTION('',(-1.,0.,0.));
#29140=DIRECTION('center_axis',(-0.909343589801517,-0.351779907850729,0.222137642283841));
#29141=DIRECTION('ref_axis',(-0.184944722510291,0.820060785619066,0.541567869712958));
#29142=DIRECTION('center_axis',(0.909343589801493,0.351779907850753,-0.2221376422839));
#29143=DIRECTION('ref_axis',(-0.341106909868786,0.936079511754707,0.0860303650627931));
#29144=DIRECTION('center_axis',(-1.6864379156382E-6,0.0915162499593412,
-0.995803583037607));
#29145=DIRECTION('ref_axis',(-0.34113926666238,0.936068028098637,0.0860270161785332));
#29146=DIRECTION('center_axis',(-9.8391347151436E-16,-0.864344564896165,
0.502900062770387));
#29147=DIRECTION('ref_axis',(0.0165957593644498,0.502830803827501,0.864225528142572));
#29148=DIRECTION('center_axis',(0.872337072829626,0.488810663329849,0.00960035322651945));
#29149=DIRECTION('ref_axis',(0.357490239572424,-0.624340021233245,-0.69455040601595));
#29150=DIRECTION('center_axis',(-0.872337165983214,0.252719928315943,0.418521811470274));
#29151=DIRECTION('ref_axis',(-0.357492608063605,-0.913666211044819,-0.193424636421748));
#29152=DIRECTION('center_axis',(0.,-0.816631319604251,0.577159672743531));
#29153=DIRECTION('ref_axis',(1.,0.,0.));
#29154=DIRECTION('center_axis',(0.,0.0033519474796912,0.999994382208267));
#29155=DIRECTION('ref_axis',(1.,0.,0.));
#29156=DIRECTION('center_axis',(1.,2.42086419888004E-12,-4.76508631093348E-9));
#29157=DIRECTION('ref_axis',(4.76508363468576E-9,-0.00168336254192495,0.999998583144272));
#29158=DIRECTION('center_axis',(1.51830655795334E-16,0.0033519474626319,
-0.999994382208324));
#29159=DIRECTION('ref_axis',(-0.0165957593611889,0.999856663884339,0.00335148583545193));
#29160=DIRECTION('center_axis',(-3.10862446895044E-14,0.816631319604264,
-0.577159672743512));
#29161=DIRECTION('ref_axis',(0.818873283807973,0.33127484328694,0.468725424177909));
#29162=DIRECTION('center_axis',(-0.909343584374911,-0.016486906074352,0.415719169012309));
#29163=DIRECTION('ref_axis',(0.341106909670097,0.542544239120665,0.767653453566317));
#29164=DIRECTION('center_axis',(0.9093435898015,-0.0164868874227782,0.415719157881892));
#29165=DIRECTION('ref_axis',(0.0165957593541801,0.999856663884451,0.00335148583689117));
#29166=DIRECTION('center_axis',(-0.872334653160836,-0.252721554400087,-0.41852606709304));
#29167=DIRECTION('ref_axis',(0.357508978425797,-0.913652443783903,-0.193459407402805));
#29168=DIRECTION('center_axis',(1.15170725409523E-6,-0.816634222548046,
0.577155565304556));
#29169=DIRECTION('ref_axis',(-0.999999999666746,1.39449692278666E-5,2.17266316248917E-5));
#29170=DIRECTION('center_axis',(-0.909343589801518,0.0164868874227569,-0.415719157881855));
#29171=DIRECTION('ref_axis',(-0.184944722510292,0.879041925861211,0.439409538123383));
#29172=DIRECTION('center_axis',(-1.35716939467332E-15,0.00335194746035888,
-0.999994382208332));
#29173=DIRECTION('ref_axis',(-1.,-1.17865786493649E-10,-3.93724966170751E-13));
#29174=DIRECTION('center_axis',(0.872337121117555,0.252719440142821,-0.418522199762732));
#29175=DIRECTION('ref_axis',(0.357492026988926,-0.913666559888409,0.19342406256986));
#29176=DIRECTION('center_axis',(-1.68628111100734E-6,-0.81663307513297,
-0.577157188810835));
#29177=DIRECTION('ref_axis',(-0.341139266645681,0.542535595401582,-0.767645183971539));
#29178=DIRECTION('center_axis',(-0.909343589801519,0.0164868874292406,0.415719157881595));
#29179=DIRECTION('ref_axis',(-0.184944722510296,0.87904192585435,-0.439409538137107));
#29180=DIRECTION('center_axis',(0.909343589801544,-0.0164868874292662,-0.415719157881539));
#29181=DIRECTION('ref_axis',(-0.341106909868691,0.542544237518575,-0.76765345461036));
#29182=DIRECTION('center_axis',(-1.61391540184803E-16,0.00335194747587369,
0.99999438220828));
#29183=DIRECTION('ref_axis',(0.016595759364439,0.999856663884241,-0.00335148584869172));
#29184=DIRECTION('center_axis',(0.999995050428565,0.00314628644158368,3.89202510670605E-13));
#29185=DIRECTION('ref_axis',(5.29618892397034E-9,-1.68342965936362E-6,0.999999999998583));
#29186=DIRECTION('center_axis',(-0.909343590214608,-0.0164868860208534,
-0.415719157033859));
#29187=DIRECTION('ref_axis',(-0.0165957582094495,0.999856663906389,-0.00335148496028424));
#29188=DIRECTION('center_axis',(1.33226762954886E-14,-0.00335194747968279,
-0.999994382208267));
#29189=DIRECTION('ref_axis',(0.701214746224632,0.712946119051022,-0.00238977137213218));
#29190=DIRECTION('center_axis',(-1.72180181182493E-5,-0.816644232415063,
-0.577141401535839));
#29191=DIRECTION('ref_axis',(0.999999999425232,2.7958306584923E-6,-3.37893227556071E-5));
#29192=DIRECTION('center_axis',(0.872334424881579,-0.252721294015423,0.418526700125207));
#29193=DIRECTION('ref_axis',(-0.357509234129503,-0.913652180043168,0.193460180436447));
#29194=DIRECTION('center_axis',(-0.872337165908837,0.488810485061077,-0.00960097226811875));
#29195=DIRECTION('ref_axis',(-0.357492574939675,-0.624343693581199,0.694545902837521));
#29196=DIRECTION('center_axis',(0.,0.0915192788336707,0.995803304675057));
#29197=DIRECTION('ref_axis',(1.,0.,0.));
#29198=DIRECTION('center_axis',(0.,0.86769651237392,0.497094319434588));
#29199=DIRECTION('ref_axis',(1.,0.,0.));
#29200=DIRECTION('center_axis',(1.,-4.12985136017776E-9,-2.38437093081533E-9));
#29201=DIRECTION('ref_axis',(4.76873489842038E-9,0.8651823496475,0.501457377908064));
#29202=DIRECTION('center_axis',(5.42101086242752E-18,-0.864344564902831,
-0.502900062758931));
#29203=DIRECTION('ref_axis',(-0.0165957593611997,0.502830803816073,-0.864225528149283));
#29204=DIRECTION('center_axis',(-2.22044604925032E-15,-0.091519278833694,
-0.995803304675055));
#29205=DIRECTION('ref_axis',(0.818873283807975,0.571565546381172,-0.0525297178322415));
#29206=DIRECTION('center_axis',(-0.909343584373447,0.351779908167727,0.222137664002207));
#29207=DIRECTION('ref_axis',(0.341106909670685,0.9360795116516,-0.0860303669701453));
#29208=DIRECTION('center_axis',(0.909343589801524,0.351779907854156,0.222137642278383));
#29209=DIRECTION('ref_axis',(0.0165957593541706,0.502830803817422,-0.864225528148633));
#29210=DIRECTION('center_axis',(-0.872334659306141,-0.488814972476424,0.00960025291910624));
#29211=DIRECTION('ref_axis',(0.357509612665106,-0.624368160481923,0.694515138084452));
#29212=DIRECTION('center_axis',(1.15170339592403E-6,0.091514270219573,0.995803764978247));
#29213=DIRECTION('ref_axis',(-0.999999999666746,2.57883005308933E-5,-1.21338575712886E-6));
#29214=DIRECTION('center_axis',(-0.909343589801512,-0.351779907854202,-0.222137642278361));
#29215=DIRECTION('ref_axis',(-0.184944722510301,0.820060785610628,-0.541567869725733));
#29216=DIRECTION('center_axis',(-3.57959140632929E-17,-0.864344564903985,
-0.502900062756946));
#29217=DIRECTION('ref_axis',(-1.,-5.92716031326802E-11,1.01871380838448E-10));
#29218=DIRECTION('center_axis',(0.87233712123921,-0.236091136889651,-0.42812255487213));
#29219=DIRECTION('ref_axis',(0.357492075733543,-0.28932299193772,0.887970507462905));
#29220=DIRECTION('center_axis',(-1.68626957992325E-6,-0.908149325054355,
0.418646394228443));
#29221=DIRECTION('ref_axis',(-0.341139266648757,-0.393532432712662,-0.853672200059017));
#29222=DIRECTION('center_axis',(-0.909343589801511,0.368266795279956,0.193581515597778));
#29223=DIRECTION('ref_axis',(-0.1849447225103,0.0589811402353276,-0.980977407850012));
#29224=DIRECTION('center_axis',(0.909343589801499,-0.368266795279986,-0.193581515597776));
#29225=DIRECTION('ref_axis',(-0.341106909868806,-0.393535274236167,-0.853683819673079));
#29226=DIRECTION('center_axis',(2.71050543116904E-18,0.867696512372032,
0.497094319437884));
#29227=DIRECTION('ref_axis',(0.0165957593644693,0.497025860056731,-0.867577013991256));
#29228=DIRECTION('center_axis',(0.99999505042847,0.00157314323581978,-0.00272476401205455));
#29229=DIRECTION('ref_axis',(-1.62748491112573E-10,0.866025429650388,0.499999955198858));
#29230=DIRECTION('center_axis',(-0.909343590214268,-0.368266793842775,-0.193581516392936));
#29231=DIRECTION('ref_axis',(-0.0165957582102913,0.497025860836397,-0.867577013566671));
#29232=DIRECTION('center_axis',(0.,-0.867696512373919,-0.497094319434589));
#29233=DIRECTION('ref_axis',(0.701214746224636,0.354403456808009,-0.618624336313771));
#29234=DIRECTION('center_axis',(-1.72180195932569E-5,-0.908141231516168,
0.418663950351399));
#29235=DIRECTION('ref_axis',(0.999999999425232,-2.7864497681015E-5,-1.93159206798986E-5));
#29236=DIRECTION('center_axis',(0.872334413842153,0.236094117750599,0.428126427577455));
#29237=DIRECTION('ref_axis',(-0.35750837102373,-0.289287102352822,0.887975639902507));
#29238=DIRECTION('center_axis',(-0.872337161491928,0.236090560831439,-0.42812279052452));
#29239=DIRECTION('ref_axis',(-0.357491177692246,0.289326452437243,0.887969741484636));
#29240=DIRECTION('center_axis',(0.,0.908150598437932,0.418643631931534));
#29241=DIRECTION('ref_axis',(1.,0.,0.));
#29242=DIRECTION('center_axis',(0.,0.864344564894221,-0.502900062773729));
#29243=DIRECTION('ref_axis',(1.,0.,0.));
#29244=DIRECTION('center_axis',(1.,-4.13180676296342E-9,2.3882947650968E-9));
#29245=DIRECTION('ref_axis',(4.7723861707432E-9,0.866865647562842,-0.498541822794693));
#29246=DIRECTION('center_axis',(-4.54009659728305E-16,-0.867696512365431,
0.497094319449405));
#29247=DIRECTION('ref_axis',(-0.0165957593611997,-0.497025860068278,-0.867577013984703));
#29248=DIRECTION('center_axis',(-4.44089209850062E-15,-0.908150598437929,
-0.41864363193154));
#29249=DIRECTION('ref_axis',(0.818873283807975,0.24029070309425,-0.521255142010144));
#29250=DIRECTION('center_axis',(-0.909343584372254,0.368266814251329,-0.193581505010677));
#29251=DIRECTION('ref_axis',(0.341106909671091,0.393535272534209,-0.853683820536658));
#29252=DIRECTION('center_axis',(0.909343589801533,0.36826679527692,-0.19358151560345));
#29253=DIRECTION('ref_axis',(0.0165957593541802,-0.497025860067054,-0.867577013985539));
#29254=DIRECTION('center_axis',(-0.872335303813278,-0.236092825490624,0.428125326829481));
#29255=DIRECTION('ref_axis',(0.357518325797022,0.289256956575762,0.887981452391784));
#29256=DIRECTION('center_axis',(1.15182100555332E-6,0.908148492690305,0.41864819983251));
#29257=DIRECTION('ref_axis',(-0.999999999666752,1.18433208703558E-5,-2.29397212159883E-5));
#29258=DIRECTION('center_axis',(-0.90934358980152,-0.368266795276941,0.193581515603471));
#29259=DIRECTION('ref_axis',(-0.184944722510296,-0.0589811402505156,-0.9809774078491));
#29260=DIRECTION('center_axis',(-1.16345885865374E-15,-0.867696512364302,
0.497094319451376));
#29261=DIRECTION('ref_axis',(-1.,5.85957252551265E-11,1.02278664219265E-10));
#29262=DIRECTION('center_axis',(0.872337121208026,-0.488810576952673,-0.00960035528969041));
#29263=DIRECTION('ref_axis',(0.357492065497932,0.624343502497626,0.694546336823555));
#29264=DIRECTION('center_axis',(-1.68643573492616E-6,-0.0915162499578196,
0.995803583037746));
#29265=DIRECTION('ref_axis',(-0.341139266673693,-0.936068028094749,-0.086027016175985));
#29266=DIRECTION('center_axis',(-0.909343589801517,0.351779907850729,-0.222137642283841));
#29267=DIRECTION('ref_axis',(-0.184944722510291,-0.820060785619066,-0.541567869712958));
#29268=DIRECTION('center_axis',(0.909343589801493,-0.351779907850753,0.2221376422839));
#29269=DIRECTION('ref_axis',(-0.341106909868786,-0.936079511754707,-0.0860303650627931));
#29270=DIRECTION('center_axis',(-9.89334482376699E-16,0.864344564896165,
-0.502900062770387));
#29271=DIRECTION('ref_axis',(0.0165957593644802,-0.502830803827501,-0.864225528142571));
#29272=DIRECTION('center_axis',(0.999995050428028,-0.00157314330632356,
-0.00272476413353121));
#29273=DIRECTION('ref_axis',(-1.09147368725947E-8,0.866023669196806,-0.500003004381874));
#29274=DIRECTION('center_axis',(-0.909343590213997,-0.351779907820795,0.222137640642713));
#29275=DIRECTION('ref_axis',(-0.0165957582109795,-0.502830803070625,-0.864225528605093));
#29276=DIRECTION('center_axis',(-1.77635683939847E-14,-0.864344564894251,
0.502900062773677));
#29277=DIRECTION('ref_axis',(0.701214746224631,-0.358542662243024,-0.616234564941639));
#29278=DIRECTION('center_axis',(-1.72180172530394E-5,-0.0914969991021175,
0.995805351893053));
#29279=DIRECTION('ref_axis',(0.999999999425232,-3.06603499728098E-5,1.44733980403473E-5));
#29280=DIRECTION('center_axis',(0.872334418927631,0.488815412109119,0.00959971034899223));
#29281=DIRECTION('ref_axis',(-0.357508592704786,0.624366331201059,0.694517307635146));
#29282=DIRECTION('center_axis',(-0.872337088253931,-0.252719995041193,-0.418521933192315));
#29283=DIRECTION('ref_axis',(-0.357492387674659,0.913666486545701,0.19342374238419));
#29284=DIRECTION('center_axis',(0.,0.816631319604251,-0.577159672743531));
#29285=DIRECTION('ref_axis',(1.,0.,0.));
#29286=DIRECTION('center_axis',(0.,-0.00335194747960493,-0.999994382208267));
#29287=DIRECTION('ref_axis',(1.,0.,0.));
#29288=DIRECTION('center_axis',(1.,2.42058998900158E-12,4.77239700262987E-9));
#29289=DIRECTION('ref_axis',(4.77238616670059E-9,0.00168330521887406,-0.999998583240767));
#29290=DIRECTION('center_axis',(1.51830655795334E-16,-0.0033519474626319,
0.999994382208324));
#29291=DIRECTION('ref_axis',(-0.0165957593611889,-0.999856663884339,-0.00335148583545193));
#29292=DIRECTION('center_axis',(-3.10862446895044E-14,-0.816631319604264,
0.577159672743512));
#29293=DIRECTION('ref_axis',(0.818873283807973,-0.33127484328694,-0.468725424177909));
#29294=DIRECTION('center_axis',(-0.909343584372272,0.0164869060835493,-0.415719169017717));
#29295=DIRECTION('ref_axis',(0.341106909671091,-0.54254423911736,-0.767653453568212));
#29296=DIRECTION('center_axis',(0.9093435898015,0.016486887422769,-0.415719157881893));
#29297=DIRECTION('ref_axis',(0.01659575935417,-0.999856663884451,-0.00335148583689154));
#29298=DIRECTION('center_axis',(-0.872334977453413,0.2527212762883,0.418525559103105));
#29299=DIRECTION('ref_axis',(0.357507402186026,0.913653676946343,0.193456496361912));
#29300=DIRECTION('center_axis',(1.15166574883469E-6,0.816634222527976,-0.577155565332953));
#29301=DIRECTION('ref_axis',(-0.999999999666747,-1.3944963123932E-5,-2.172655107418E-5));
#29302=DIRECTION('center_axis',(-0.909343589801518,-0.0164868874227569,
0.415719157881854));
#29303=DIRECTION('ref_axis',(-0.184944722510291,-0.879041925861207,-0.439409538123392));
#29304=DIRECTION('center_axis',(3.05791507767584E-15,-0.00335194746035888,
0.999994382208332));
#29305=DIRECTION('ref_axis',(-1.,1.17874460205389E-10,3.98169149435635E-13));
#29306=DIRECTION('center_axis',(0.872336706091693,-0.252719795504182,0.418522850230927));
#29307=DIRECTION('ref_axis',(0.357487400579544,0.913671323189871,-0.193410112474378));
#29308=DIRECTION('center_axis',(-1.68617080662445E-6,0.816633075161264,
0.577157188770802));
#29309=DIRECTION('ref_axis',(-0.341139266540615,-0.542535595355228,0.767645184050991));
#29310=DIRECTION('center_axis',(-0.909343589801519,-0.0164868874292406,
-0.415719157881595));
#29311=DIRECTION('ref_axis',(-0.184944722510296,-0.87904192585435,0.439409538137107));
#29312=DIRECTION('center_axis',(0.909343589801512,0.0164868874292142,0.415719157881612));
#29313=DIRECTION('ref_axis',(-0.341106909868779,-0.542544237518574,0.767653454610322));
#29314=DIRECTION('center_axis',(-1.59898644615292E-16,-0.00335194747587375,
-0.99999438220828));
#29315=DIRECTION('ref_axis',(0.0165957593644498,-0.999856663884241,0.00335148584869178));
#29316=DIRECTION('center_axis',(0.999995050428519,-0.00314628645604584,
-3.89202510576123E-13));
#29317=DIRECTION('ref_axis',(5.29426700772326E-9,1.68281880237154E-6,-0.999999999998584));
#29318=DIRECTION('center_axis',(-0.909343590214001,0.0164868860229314,0.415719157035105));
#29319=DIRECTION('ref_axis',(-0.0165957582109798,-0.999856663906358,0.00335148496194759));
#29320=DIRECTION('center_axis',(1.33226762954886E-14,0.00335194747968279,
0.999994382208267));
#29321=DIRECTION('ref_axis',(0.701214746224632,-0.712946119051022,0.00238977137213218));
#29322=DIRECTION('center_axis',(-1.72180378594051E-5,0.816644232407161,
0.57714140154702));
#29323=DIRECTION('ref_axis',(0.999999999425228,-2.79588956264274E-6,3.37894403045313E-5));
#29324=DIRECTION('center_axis',(0.872334340382926,0.252721365861299,-0.418526832862464));
#29325=DIRECTION('ref_axis',(-0.357509057710921,0.913652418969074,-0.193459378078731));
#29326=DIRECTION('center_axis',(-1.33226762954919E-14,0.86434456489425,
-0.502900062773679));
#29327=DIRECTION('ref_axis',(0.701214746224629,0.35854266224302,0.616234564941643));
#29328=DIRECTION('center_axis',(0.,-0.864344564894221,0.502900062773729));
#29329=DIRECTION('ref_axis',(1.,0.,0.));
#29330=DIRECTION('center_axis',(-1.7218016834779E-5,0.0914969991024323,
-0.995805351893024));
#29331=DIRECTION('ref_axis',(0.999999999425232,3.06603442363514E-5,-1.44733981459298E-5));
#29332=DIRECTION('center_axis',(-0.909343590214593,0.351779907820795,-0.222137640640273));
#29333=DIRECTION('ref_axis',(-0.0165957582094507,0.502830803069125,0.864225528605995));
#29334=DIRECTION('center_axis',(1.,4.212129460891E-9,-2.43187398740037E-9));
#29335=DIRECTION('ref_axis',(4.86374121739737E-9,-0.866866002087437,0.498541206346019));
#29336=DIRECTION('center_axis',(-4.54009659728305E-16,0.867696512365431,
-0.497094319449405));
#29337=DIRECTION('ref_axis',(-0.0165957593611997,0.497025860068278,0.867577013984703));
#29338=DIRECTION('center_axis',(-4.44089209850062E-15,0.908150598437929,
0.41864363193154));
#29339=DIRECTION('ref_axis',(0.818873283807975,-0.24029070309425,0.521255142010144));
#29340=DIRECTION('center_axis',(0.,-0.908150598437932,-0.418643631931534));
#29341=DIRECTION('ref_axis',(1.,0.,0.));
#29342=DIRECTION('center_axis',(-0.90934358437491,-0.368266814242001,0.193581505015946));
#29343=DIRECTION('ref_axis',(0.341106909670097,-0.393535272530976,0.853683820538545));
#29344=DIRECTION('center_axis',(-0.872337165954994,-0.23609055663585,0.428122783744317));
#29345=DIRECTION('ref_axis',(-0.357492608396839,-0.289322455852271,-0.887970467685291));
#29346=DIRECTION('center_axis',(-0.872334654387134,0.236093427908942,-0.428126317870655));
#29347=DIRECTION('ref_axis',(0.357509141512415,-0.28928500211756,-0.887976013913044));
#29348=DIRECTION('center_axis',(0.9093435898015,-0.368266795276978,0.193581515603494));
#29349=DIRECTION('ref_axis',(0.0165957593541708,0.497025860067054,0.867577013985539));
#29350=DIRECTION('center_axis',(-0.90934358980152,0.368266795276941,-0.193581515603471));
#29351=DIRECTION('ref_axis',(-0.184944722510296,0.0589811402505156,0.9809774078491));
#29352=DIRECTION('center_axis',(2.04681325985981E-15,0.867696512364302,
-0.497094319451376));
#29353=DIRECTION('ref_axis',(-1.,-5.85977525160398E-11,-1.02288660952578E-10));
#29354=DIRECTION('center_axis',(1.15181146809394E-6,-0.908148492693187,
-0.418648199826257));
#29355=DIRECTION('ref_axis',(-0.999999999666753,-1.18433108705755E-5,2.29397223096969E-5));
#29356=DIRECTION('center_axis',(-0.87233721909546,-0.488810390102957,0.00960097433567008));
#29357=DIRECTION('ref_axis',(-0.35749205135526,0.624342897076992,-0.69454688832887));
#29358=DIRECTION('center_axis',(0.,-0.0915192788337281,-0.995803304675052));
#29359=DIRECTION('ref_axis',(1.,0.,0.));
#29360=DIRECTION('center_axis',(0.,-0.86769651237392,-0.497094319434588));
#29361=DIRECTION('ref_axis',(1.,0.,0.));
#29362=DIRECTION('center_axis',(1.,4.22162271441645E-9,2.43735514986856E-9));
#29363=DIRECTION('ref_axis',(4.87470318552635E-9,-0.865182573208305,-0.501456992190413));
#29364=DIRECTION('center_axis',(1.35525271560688E-18,0.864344564902831,
0.502900062758931));
#29365=DIRECTION('ref_axis',(-0.016595759361191,-0.502830803816073,0.864225528149283));
#29366=DIRECTION('center_axis',(-2.22044604925032E-15,0.091519278833694,
0.995803304675055));
#29367=DIRECTION('ref_axis',(0.818873283807975,-0.571565546381172,0.0525297178322415));
#29368=DIRECTION('center_axis',(-0.909343584370803,-0.351779908167854,-0.222137664012828));
#29369=DIRECTION('ref_axis',(0.341106909671707,-0.936079511651572,0.0860303669663984));
#29370=DIRECTION('center_axis',(0.909343589801524,-0.351779907854152,-0.222137642278389));
#29371=DIRECTION('ref_axis',(0.0165957593541805,-0.502830803817418,0.864225528148635));
#29372=DIRECTION('center_axis',(-0.872335148377002,0.488814099296658,-0.00960027264571843));
#29373=DIRECTION('ref_axis',(0.357508508680803,0.624367614508793,-0.694516197200201));
#29374=DIRECTION('center_axis',(1.15179046766159E-6,-0.0915142700473301,
-0.995803764994076));
#29375=DIRECTION('ref_axis',(-0.999999999666754,-2.57879850815794E-5,1.21326932795859E-6));
#29376=DIRECTION('center_axis',(-0.909343589801512,0.351779907854202,0.222137642278361));
#29377=DIRECTION('ref_axis',(-0.184944722510301,-0.820060785610628,0.541567869725733));
#29378=DIRECTION('center_axis',(-2.59499130955602E-17,0.864344564903985,
0.502900062756946));
#29379=DIRECTION('ref_axis',(-1.,5.92813457518923E-11,-1.0188810609777E-10));
#29380=DIRECTION('center_axis',(0.872337163237809,0.236091097930777,0.428122490780446));
#29381=DIRECTION('ref_axis',(0.357491458240221,0.289324548017128,-0.887970249051152));
#29382=DIRECTION('center_axis',(-1.68635658201456E-6,0.908149325052148,
-0.418646394233229));
#29383=DIRECTION('ref_axis',(-0.341139266558313,0.393532432703947,0.853672200099177));
#29384=DIRECTION('center_axis',(-0.909343589801511,-0.368266795279956,-0.193581515597778));
#29385=DIRECTION('ref_axis',(-0.1849447225103,-0.0589811402353276,0.980977407850012));
#29386=DIRECTION('center_axis',(0.909343589801501,0.368266795279979,0.19358151559778));
#29387=DIRECTION('ref_axis',(-0.341106909868806,0.393535274236167,0.853683819673079));
#29388=DIRECTION('center_axis',(1.35525271558452E-18,-0.867696512372032,
-0.497094319437884));
#29389=DIRECTION('ref_axis',(0.0165957593644498,-0.497025860056731,0.867577013991256));
#29390=DIRECTION('center_axis',(0.999995050428592,-0.00157314321649704,
0.00272476397858654));
#29391=DIRECTION('ref_axis',(4.67404295639049E-10,-0.866025329508561,-0.500000128649572));
#29392=DIRECTION('center_axis',(-0.909343590213624,0.368266793844967,0.19358151639179));
#29393=DIRECTION('ref_axis',(-0.0165957582118193,-0.497025860834913,0.867577013567492));
#29394=DIRECTION('center_axis',(0.,0.867696512373919,0.497094319434589));
#29395=DIRECTION('ref_axis',(0.701214746224636,-0.354403456808009,0.618624336313771));
#29396=DIRECTION('center_axis',(-1.7218041121248E-5,0.908141231519907,-0.418663950343286));
#29397=DIRECTION('ref_axis',(0.999999999425228,2.78645745094749E-5,1.93160359156296E-5));
#29398=DIRECTION('center_axis',(0.872334911744233,-0.236093655852982,-0.428125667787106));
#29399=DIRECTION('ref_axis',(-0.357507870022192,0.289286581381741,-0.887976011334012));
#29400=DIRECTION('center_axis',(1.,0.,0.));
#29401=DIRECTION('ref_axis',(0.,0.981895700022487,0.189422370055255));
#29402=DIRECTION('center_axis',(-1.,0.,0.));
#29403=DIRECTION('ref_axis',(0.,0.654992470158046,0.755635404170729));
#29404=DIRECTION('center_axis',(1.,0.,0.));
#29405=DIRECTION('ref_axis',(0.,0.654992434517533,-0.755635435064288));
#29406=DIRECTION('center_axis',(-1.,0.,0.));
#29407=DIRECTION('ref_axis',(0.,0.981895710396792,-0.189422316278677));
#29408=DIRECTION('center_axis',(1.,0.,0.));
#29409=DIRECTION('ref_axis',(0.,-0.326903271294508,-0.945057803108862));
#29410=DIRECTION('center_axis',(-1.,0.,0.));
#29411=DIRECTION('ref_axis',(0.,0.326903317255781,-0.945057787210479));
#29412=DIRECTION('center_axis',(1.,0.,0.));
#29413=DIRECTION('ref_axis',(0.,-0.981895688630785,-0.189422429105626));
#29414=DIRECTION('center_axis',(-1.,0.,0.));
#29415=DIRECTION('ref_axis',(0.,-0.65499239314391,-0.75563547092736));
#29416=DIRECTION('center_axis',(1.,0.,0.));
#29417=DIRECTION('ref_axis',(0.,-0.654992632839938,0.755635263156376));
#29418=DIRECTION('center_axis',(-1.,0.,0.));
#29419=DIRECTION('ref_axis',(0.,-0.981896389769016,0.189418794628653));
#29420=DIRECTION('center_axis',(1.,0.,0.));
#29421=DIRECTION('ref_axis',(0.,0.32690326548914,0.945057805116987));
#29422=DIRECTION('center_axis',(-1.,0.,0.));
#29423=DIRECTION('ref_axis',(0.,-0.32690305834171,0.945057876770961));
#29424=DIRECTION('center_axis',(-1.,0.,0.));
#29425=DIRECTION('ref_axis',(0.,0.,1.));
#29426=DIRECTION('center_axis',(-1.,0.,0.));
#29427=DIRECTION('ref_axis',(0.,0.500000000006722,0.866025403780558));
#29428=DIRECTION('center_axis',(1.,0.,0.));
#29429=DIRECTION('ref_axis',(0.,-0.500000000006722,-0.866025403780558));
#29430=DIRECTION('center_axis',(-1.,0.,0.));
#29431=DIRECTION('ref_axis',(0.,-0.500000000006722,-0.866025403780558));
#29432=DIRECTION('',(-1.,0.,0.));
#29433=DIRECTION('center_axis',(-1.,0.,0.));
#29434=DIRECTION('ref_axis',(0.,0.,1.));
#29435=DIRECTION('center_axis',(-1.,0.,0.));
#29436=DIRECTION('ref_axis',(0.,-1.,7.80005689667481E-12));
#29437=DIRECTION('center_axis',(1.,0.,0.));
#29438=DIRECTION('ref_axis',(0.,1.,-7.80005689667481E-12));
#29439=DIRECTION('center_axis',(-1.,0.,0.));
#29440=DIRECTION('ref_axis',(0.,1.,-7.80005689667481E-12));
#29441=DIRECTION('',(-1.,0.,0.));
#29442=DIRECTION('center_axis',(1.,0.,0.));
#29443=DIRECTION('ref_axis',(0.,1.,0.));
#29444=DIRECTION('center_axis',(0.999995050427998,0.00157314331111629,0.00272476414181539));
#29445=DIRECTION('ref_axis',(-1.20457054480573E-8,-0.866023489464513,0.500003315684714));
#29446=DIRECTION('center_axis',(0.872335130168889,-0.488814142273061,-0.00959973890682644));
#29447=DIRECTION('ref_axis',(-0.357518018969466,-0.624385691970657,-0.694495049496015));
#29448=DIRECTION('center_axis',(-1.,0.,0.));
#29449=DIRECTION('ref_axis',(0.,0.,1.));
#29450=DIRECTION('center_axis',(-1.,0.,0.));
#29451=DIRECTION('ref_axis',(0.,-0.499999999993262,0.866025403788329));
#29452=DIRECTION('center_axis',(1.,0.,0.));
#29453=DIRECTION('ref_axis',(0.,0.499999999993262,-0.866025403788329));
#29454=DIRECTION('',(-1.,0.,0.));
#29455=DIRECTION('center_axis',(-1.,0.,0.));
#29456=DIRECTION('ref_axis',(0.,0.499999999993262,-0.866025403788329));
#29457=DIRECTION('center_axis',(-1.,0.,0.));
#29458=DIRECTION('ref_axis',(0.,0.,1.));
#29459=DIRECTION('center_axis',(-1.,0.,0.));
#29460=DIRECTION('ref_axis',(0.,-0.500000000006722,-0.866025403780558));
#29461=DIRECTION('center_axis',(1.,0.,0.));
#29462=DIRECTION('ref_axis',(0.,0.500000000006722,0.866025403780558));
#29463=DIRECTION('',(-1.,0.,0.));
#29464=DIRECTION('center_axis',(-1.,0.,0.));
#29465=DIRECTION('ref_axis',(0.,0.500000000006722,0.866025403780558));
#29466=DIRECTION('center_axis',(1.,0.,0.));
#29467=DIRECTION('ref_axis',(0.,1.,0.));
#36395=CARTESIAN_POINT('',(0.,0.,0.));
#36396=CARTESIAN_POINT('Origin',(7.4,0.,0.));
#36397=CARTESIAN_POINT('',(7.4,-12.,9.33005511289567E-11));
#36398=CARTESIAN_POINT('Origin',(7.4,-13.5,1.05000452776949E-10));
#36399=CARTESIAN_POINT('Origin',(7.4,-13.5,1.05000452776949E-10));
#36400=CARTESIAN_POINT('',(6.,-12.,9.33005511289567E-11));
#36401=CARTESIAN_POINT('',(7.4,-12.,9.33005511289567E-11));
#36402=CARTESIAN_POINT('Origin',(6.,-13.5,1.05000452776949E-10));
#36403=CARTESIAN_POINT('Origin',(-6.,0.,0.));
#36404=CARTESIAN_POINT('',(6.,-7.79422863409496,-4.49999999993936));
#36405=CARTESIAN_POINT('Origin',(6.,0.,0.));
#36406=CARTESIAN_POINT('',(-6.,-7.79422863409496,-4.49999999993936));
#36407=CARTESIAN_POINT('',(-6.,-7.79422863409496,-4.49999999993936));
#36408=CARTESIAN_POINT('Origin',(-6.,0.,0.));
#36409=CARTESIAN_POINT('Origin',(-7.4,0.,0.));
#36410=CARTESIAN_POINT('',(-7.4,-5.99999999991914,10.3923048454599));
#36411=CARTESIAN_POINT('Origin',(-7.4,-6.74999999990903,11.6913429511424));
#36412=CARTESIAN_POINT('Origin',(-6.,-6.74999999990903,11.6913429511424));
#36413=CARTESIAN_POINT('',(-6.,-5.99999999991914,10.3923048454599));
#36414=CARTESIAN_POINT('Origin',(-6.,-6.74999999990903,11.6913429511424));
#36415=CARTESIAN_POINT('',(-6.,-5.99999999991914,10.3923048454599));
#36416=CARTESIAN_POINT('Origin',(-5.599999999997,9.91330329119812,16.8993688492357));
#36417=CARTESIAN_POINT('',(-5.73644346284594,10.2877335024464,16.9337808604212));
#36418=CARTESIAN_POINT('',(-5.593361696257,10.1144356127388,17.245059060506));
#36419=CARTESIAN_POINT('Origin',(-5.599999999997,9.91330329119812,16.8993688492357));
#36420=CARTESIAN_POINT('',(-5.99999988457187,9.91329944048963,16.8993703246792));
#36421=CARTESIAN_POINT('Origin',(-5.59998163813197,9.91328781245746,16.899368578592));
#36422=CARTESIAN_POINT('Origin',(-5.6,9.91330329122126,16.8993688492756));
#36423=CARTESIAN_POINT('Ctrl Pts',(-5.71725976045777,6.24680066004962,7.76998179728242));
#36424=CARTESIAN_POINT('Ctrl Pts',(-5.71831534155782,6.59326365245468,8.0322873967129));
#36425=CARTESIAN_POINT('Ctrl Pts',(-5.72040693333068,7.31940961543903,8.6580789671924));
#36426=CARTESIAN_POINT('Ctrl Pts',(-5.72308360876896,8.29718047263615,9.7712913738905));
#36427=CARTESIAN_POINT('Ctrl Pts',(-5.72473138802017,9.14170425907276,11.09270696355));
#36428=CARTESIAN_POINT('Ctrl Pts',(-5.72548313711387,9.77722230302052,12.5261363218648));
#36429=CARTESIAN_POINT('Ctrl Pts',(-5.72532322728419,10.1890896765162,14.0392347180325));
#36430=CARTESIAN_POINT('Ctrl Pts',(-5.72405908827357,10.3627203405144,15.5563821125621));
#36431=CARTESIAN_POINT('Ctrl Pts',(-5.72276356923005,10.3310899357146,16.5600586046216));
#36432=CARTESIAN_POINT('Ctrl Pts',(-5.72204265313815,10.2826264054644,17.0373217472724));
#36433=CARTESIAN_POINT('Ctrl Pts',(-5.89609285952037,6.21373560947317,7.81372501070344));
#36434=CARTESIAN_POINT('Ctrl Pts',(-5.89699918874521,6.55804829801922,8.07502465641679));
#36435=CARTESIAN_POINT('Ctrl Pts',(-5.89878323011297,7.27965106221252,8.69820511837471));
#36436=CARTESIAN_POINT('Ctrl Pts',(-5.90106053656845,8.25103625935808,9.80606453249069));
#36437=CARTESIAN_POINT('Ctrl Pts',(-5.90245598645081,9.09015375604841,11.1204741768065));
#36438=CARTESIAN_POINT('Ctrl Pts',(-5.90309184480868,9.72171466792549,12.5458529340524));
#36439=CARTESIAN_POINT('Ctrl Pts',(-5.90295661080893,10.1313156291003,14.0503359021025));
#36440=CARTESIAN_POINT('Ctrl Pts',(-5.90188725304236,10.3045491222434,15.5587605290979));
#36441=CARTESIAN_POINT('Ctrl Pts',(-5.9007872150631,10.2737083057292,16.5568806432025));
#36442=CARTESIAN_POINT('Ctrl Pts',(-5.90017436173646,10.2258509289961,17.0315264876768));
#36443=CARTESIAN_POINT('Ctrl Pts',(-6.00525587186972,6.12207143860163,7.93499146478545));
#36444=CARTESIAN_POINT('Ctrl Pts',(-6.00574428560245,6.46106668108027,8.19265050892015));
#36445=CARTESIAN_POINT('Ctrl Pts',(-6.00669083800828,7.17158216493795,8.80708017905286));
#36446=CARTESIAN_POINT('Ctrl Pts',(-6.00789177595026,8.12777738756055,9.89880924904528));
#36447=CARTESIAN_POINT('Ctrl Pts',(-6.00861945068644,8.95391379465674,11.1937955392773));
#36448=CARTESIAN_POINT('Ctrl Pts',(-6.00895004139444,9.57571950519377,12.5976933827114));
#36449=CARTESIAN_POINT('Ctrl Pts',(-6.00887976204827,9.97922213092208,14.0795974958299));
#36450=CARTESIAN_POINT('Ctrl Pts',(-6.00832366160711,10.1501988766356,15.565149471362));
#36451=CARTESIAN_POINT('Ctrl Pts',(-6.00774632916138,10.1202032839983,16.5484119161439));
#36452=CARTESIAN_POINT('Ctrl Pts',(-6.00742377484676,10.0732750596108,17.0159525992194));
#36453=CARTESIAN_POINT('Ctrl Pts',(-5.99983168827394,6.00920933186455,8.08430153208114));
#36454=CARTESIAN_POINT('Ctrl Pts',(-5.99980403842103,6.34189025785474,8.33716995126331));
#36455=CARTESIAN_POINT('Ctrl Pts',(-5.99972489362897,7.03929972274239,8.94027820900691));
#36456=CARTESIAN_POINT('Ctrl Pts',(-5.99961167767651,7.97770097450654,10.0116798962465));
#36457=CARTESIAN_POINT('Ctrl Pts',(-5.99952863066508,8.78858003993403,11.2827506176984));
#36458=CARTESIAN_POINT('Ctrl Pts',(-5.99948914891546,9.39881401793521,12.660502777851));
#36459=CARTESIAN_POINT('Ctrl Pts',(-5.99949759662813,9.79487483211952,14.1150785938901));
#36460=CARTESIAN_POINT('Ctrl Pts',(-5.99956378228369,9.96265493708979,15.5729418984143));
#36461=CARTESIAN_POINT('Ctrl Pts',(-5.99962308473657,9.93321402551191,16.5381081995503));
#36462=CARTESIAN_POINT('Ctrl Pts',(-5.99965460768659,9.88715810520574,16.9969550810575));
#36463=CARTESIAN_POINT('',(-5.99998887464722,6.09546019355616,8.13557730976511));
#36464=CARTESIAN_POINT('Ctrl Pts',(-6.,6.09546019494773,8.13557730903106));
#36465=CARTESIAN_POINT('Ctrl Pts',(-6.,6.47284397463733,8.42688307326927));
#36466=CARTESIAN_POINT('Ctrl Pts',(-6.,6.8254268304029,8.74185019914476));
#36467=CARTESIAN_POINT('Ctrl Pts',(-6.,7.15537157648669,9.08219270087464));
#36468=CARTESIAN_POINT('Ctrl Pts',(-6.,7.48531632257071,9.42253520260476));
#36469=CARTESIAN_POINT('Ctrl Pts',(-6.,7.79262295897292,9.78825308018931));
#36470=CARTESIAN_POINT('Ctrl Pts',(-6.,8.07150656503307,10.1733979622484));
#36471=CARTESIAN_POINT('Ctrl Pts',(-6.,8.35039017109301,10.5585428443073));
#36472=CARTESIAN_POINT('Ctrl Pts',(-6.,8.60085074681092,10.9631147308407));
#36473=CARTESIAN_POINT('Ctrl Pts',(-6.,8.82146093284314,11.384374132216));
#36474=CARTESIAN_POINT('Ctrl Pts',(-6.,9.04207111887552,11.8056335335917));
#36475=CARTESIAN_POINT('Ctrl Pts',(-6.,9.23283091522216,12.2435804498092));
#36476=CARTESIAN_POINT('Ctrl Pts',(-6.,9.39100132241203,12.6919789552476));
#36477=CARTESIAN_POINT('Ctrl Pts',(-6.,9.5491717296018,13.1403774606856));
#36478=CARTESIAN_POINT('Ctrl Pts',(-6.,9.67475274763484,13.5992275553444));
#36479=CARTESIAN_POINT('Ctrl Pts',(-6.,9.76681039134521,14.065832740215));
#36480=CARTESIAN_POINT('Ctrl Pts',(-6.,9.85886803505566,14.5324379250859));
#36481=CARTESIAN_POINT('Ctrl Pts',(-6.,9.9174023044434,15.0067982001686));
#36482=CARTESIAN_POINT('Ctrl Pts',(-6.,9.94189523595854,15.4800412482395));
#36483=CARTESIAN_POINT('Ctrl Pts',(-6.,9.9663881501459,15.9532839615094));
#36484=CARTESIAN_POINT('Ctrl Pts',(-6.,9.95683977462647,16.4254094493483));
#36485=CARTESIAN_POINT('Ctrl Pts',(-6.,9.91329811959712,16.8993691888704));
#36486=CARTESIAN_POINT('',(-5.73278802440778,6.65588397732571,8.10254612026116));
#36487=CARTESIAN_POINT('Ctrl Pts',(-5.732788629548,6.65588508129815,8.10254480509131));
#36488=CARTESIAN_POINT('Ctrl Pts',(-5.73461480965429,7.28539041399694,8.63201072418106));
#36489=CARTESIAN_POINT('Ctrl Pts',(-5.73605973935097,7.85267746609106,9.23785132036226));
#36490=CARTESIAN_POINT('Ctrl Pts',(-5.73818934987832,8.82745380303726,10.5699124264369));
#36491=CARTESIAN_POINT('Ctrl Pts',(-5.73887403070899,9.23545520796598,11.295703388267));
#36492=CARTESIAN_POINT('Ctrl Pts',(-5.73948314350432,9.86673753303504,12.8258684760636));
#36493=CARTESIAN_POINT('Ctrl Pts',(-5.73940757546898,10.0903327813959,13.630101659641));
#36494=CARTESIAN_POINT('Ctrl Pts',(-5.73849619057271,10.3386823732913,15.2703413022844));
#36495=CARTESIAN_POINT('Ctrl Pts',(-5.7376603737792,10.3633358169702,16.1063565631604));
#36496=CARTESIAN_POINT('Ctrl Pts',(-5.73644356975675,10.2877321238833,16.9337807346159));
#36497=CARTESIAN_POINT('Ctrl Pts',(-5.99998887464722,6.09546019355616,8.13557730976511));
#36498=CARTESIAN_POINT('Ctrl Pts',(-5.99998547921825,6.11100675442636,8.12982511321127));
#36499=CARTESIAN_POINT('Ctrl Pts',(-5.99924702936141,6.12766659220297,8.12414369074788));
#36500=CARTESIAN_POINT('Ctrl Pts',(-5.99757111922383,6.14539399483326,8.1186593693785));
#36501=CARTESIAN_POINT('Ctrl Pts',(-5.99675849849762,6.1539897151385,8.1160001139005));
#36502=CARTESIAN_POINT('Ctrl Pts',(-5.99572521918872,6.16283590510732,8.11338762463451));
#36503=CARTESIAN_POINT('Ctrl Pts',(-5.99444641739924,6.17192415080112,8.11083892421808));
#36504=CARTESIAN_POINT('Ctrl Pts',(-5.99208335737192,6.18871805138383,8.10612925605431));
#36505=CARTESIAN_POINT('Ctrl Pts',(-5.98888154550485,6.20634057735348,8.10163637476274));
#36506=CARTESIAN_POINT('Ctrl Pts',(-5.98471929678868,6.2247122040356,8.09746910711326));
#36507=CARTESIAN_POINT('Ctrl Pts',(-5.98052075454122,6.24324402566355,8.09326550216895));
#36508=CARTESIAN_POINT('Ctrl Pts',(-5.97534531555817,6.26253869227697,8.08939271396174));
#36509=CARTESIAN_POINT('Ctrl Pts',(-5.96906451712721,6.28247648632352,8.0859850126498));
#36510=CARTESIAN_POINT('Ctrl Pts',(-5.96708036809606,6.28877497769776,8.08490849549504));
#36511=CARTESIAN_POINT('Ctrl Pts',(-5.96498585612993,6.29513733212402,8.08387858902862));
#36512=CARTESIAN_POINT('Ctrl Pts',(-5.96277675262812,6.30155884067799,8.08290011214028));
#36513=CARTESIAN_POINT('Ctrl Pts',(-5.96276819005269,6.30158373070752,8.08289631952388));
#36514=CARTESIAN_POINT('Ctrl Pts',(-5.96275962575552,6.30160862162516,8.08289252768054));
#36515=CARTESIAN_POINT('Ctrl Pts',(-5.96275105973646,6.30163351343065,8.08288873661048));
#36516=CARTESIAN_POINT('Ctrl Pts',(-5.95814393011898,6.31502126957647,8.08084975548942));
#36517=CARTESIAN_POINT('Ctrl Pts',(-5.95303858385639,6.32866657460956,8.07903412755458));
#36518=CARTESIAN_POINT('Ctrl Pts',(-5.94741092738046,6.34252571709171,8.07747974063197));
#36519=CARTESIAN_POINT('Ctrl Pts',(-5.9445970991425,6.34945528833279,8.07670254717067));
#36520=CARTESIAN_POINT('Ctrl Pts',(-5.94165265231472,6.35643830389429,8.07599068280171));
#36521=CARTESIAN_POINT('Ctrl Pts',(-5.93857476871761,6.36346828407662,8.07534936047085));
#36522=CARTESIAN_POINT('Ctrl Pts',(-5.93703582691906,6.36698327416778,8.07502869930542));
#36523=CARTESIAN_POINT('Ctrl Pts',(-5.93546352269515,6.37051000428783,8.07472567506216));
#36524=CARTESIAN_POINT('Ctrl Pts',(-5.93385750052388,6.37404762303365,8.07444096290844));
#36525=CARTESIAN_POINT('Ctrl Pts',(-5.93279072795071,6.37639742537131,8.07425184776279));
#36526=CARTESIAN_POINT('Ctrl Pts',(-5.93143880138408,6.37933801246212,8.07402708026044));
#36527=CARTESIAN_POINT('Ctrl Pts',(-5.93033826070994,6.38170074903567,8.07385531940472));
#36528=CARTESIAN_POINT('Ctrl Pts',(-5.92978194146144,6.38289510365233,8.07376849492615));
#36529=CARTESIAN_POINT('Ctrl Pts',(-5.9292907651449,6.38394211949884,8.07369460520274));
#36530=CARTESIAN_POINT('Ctrl Pts',(-5.92893791716396,6.38469226970929,8.07364245316878));
#36531=CARTESIAN_POINT('Ctrl Pts',(-5.92289625201354,6.39753677110612,8.07274947618402));
#36532=CARTESIAN_POINT('Ctrl Pts',(-5.91606342401493,6.4112632443089,8.07205752186807));
#36533=CARTESIAN_POINT('Ctrl Pts',(-5.90830129090174,6.4257653898265,8.07169387381413));
#36534=CARTESIAN_POINT('Ctrl Pts',(-5.90691979809071,6.42834645993764,8.07162915227884));
#36535=CARTESIAN_POINT('Ctrl Pts',(-5.90550885030405,6.43095199112076,8.07157490355159));
#36536=CARTESIAN_POINT('Ctrl Pts',(-5.90406764675699,6.43358123433491,8.07153194448689));
#36537=CARTESIAN_POINT('Ctrl Pts',(-5.89615881854175,6.44800961466963,8.07129619994988));
#36538=CARTESIAN_POINT('Ctrl Pts',(-5.88733820569935,6.46315548487182,8.07139869495401));
#36539=CARTESIAN_POINT('Ctrl Pts',(-5.87749024056837,6.47888151010761,8.0719744125043));
#36540=CARTESIAN_POINT('Ctrl Pts',(-5.86842267263249,6.49336133414135,8.07250450759804));
#36541=CARTESIAN_POINT('Ctrl Pts',(-5.85848396636633,6.50833316775113,8.07343572352348));
#36542=CARTESIAN_POINT('Ctrl Pts',(-5.84759199118979,6.52365222601063,8.07489256489634));
#36543=CARTESIAN_POINT('Ctrl Pts',(-5.8394675843952,6.53507882761346,8.07597923391242));
#36544=CARTESIAN_POINT('Ctrl Pts',(-5.83081293488375,6.54669795905989,8.07735867445034));
#36545=CARTESIAN_POINT('Ctrl Pts',(-5.8215980603499,6.55843293498189,8.07909108415474));
#36546=CARTESIAN_POINT('Ctrl Pts',(-5.80973305411518,6.57354280565538,8.08132172244159));
#36547=CARTESIAN_POINT('Ctrl Pts',(-5.79693781470784,6.58884594900205,8.08413740289622));
#36548=CARTESIAN_POINT('Ctrl Pts',(-5.78318272732981,6.60416096633479,8.08766122688759));
#36549=CARTESIAN_POINT('Ctrl Pts',(-5.77029728532473,6.61850771399437,8.09096226223757));
#36550=CARTESIAN_POINT('Ctrl Pts',(-5.75656940843594,6.6328650694371,8.09488457325179));
#36551=CARTESIAN_POINT('Ctrl Pts',(-5.74199708174794,6.64704591625766,8.09954446852334));
#36552=CARTESIAN_POINT('Ctrl Pts',(-5.73896289923755,6.64999858663946,8.10051473037897));
#36553=CARTESIAN_POINT('Ctrl Pts',(-5.73589219231249,6.65294345964691,8.10151702941778));
#36554=CARTESIAN_POINT('Ctrl Pts',(-5.7327850837695,6.65587860746633,8.10255251599254));
#36555=CARTESIAN_POINT('Ctrl Pts',(-6.05078733404053,6.21937608458398,8.31745500825333));
#36556=CARTESIAN_POINT('Ctrl Pts',(-6.05137679754613,6.24108609553353,8.30091555233655));
#36557=CARTESIAN_POINT('Ctrl Pts',(-6.04678918860765,6.29703472795143,8.2611303180236));
#36558=CARTESIAN_POINT('Ctrl Pts',(-6.01457192808413,6.39377016385395,8.20334817451699));
#36559=CARTESIAN_POINT('Ctrl Pts',(-5.94621587675347,6.50229665753326,8.15279007607915));
#36560=CARTESIAN_POINT('Ctrl Pts',(-5.84828986776081,6.60216364521869,8.12168124521672));
#36561=CARTESIAN_POINT('Ctrl Pts',(-5.76396986597587,6.65916518418619,8.11648706068094));
#36562=CARTESIAN_POINT('Ctrl Pts',(-5.71704487350945,6.68377535583102,8.11892530572803));
#36563=CARTESIAN_POINT('Ctrl Pts',(-5.71196257432753,6.68636226063928,8.11924826849545));
#36564=CARTESIAN_POINT('Ctrl Pts',(-5.91199258851529,6.05011231896361,8.08989903605235));
#36565=CARTESIAN_POINT('Ctrl Pts',(-5.91253370828238,6.06964670142851,8.07500751342556));
#36566=CARTESIAN_POINT('Ctrl Pts',(-5.90832434009387,6.12024088422482,8.03909466970484));
#36567=CARTESIAN_POINT('Ctrl Pts',(-5.87845614354468,6.20859036946667,7.98674208030229));
#36568=CARTESIAN_POINT('Ctrl Pts',(-5.81472572690307,6.30843918680031,7.94097921734113));
#36569=CARTESIAN_POINT('Ctrl Pts',(-5.72321219984663,6.40070331179899,7.9131149693122));
#36570=CARTESIAN_POINT('Ctrl Pts',(-5.64441899272344,6.45346152161701,7.90887821946799));
#36571=CARTESIAN_POINT('Ctrl Pts',(-5.60062844116605,6.47624545205135,7.91138088985345));
#36572=CARTESIAN_POINT('Ctrl Pts',(-5.59588636767232,6.47864049401491,7.91170558345452));
#36573=CARTESIAN_POINT('Ctrl Pts',(-6.02856994163684,5.87036955877751,7.85795328373691));
#36574=CARTESIAN_POINT('Ctrl Pts',(-6.02941873278482,5.90046478652428,7.83503197831369));
#36575=CARTESIAN_POINT('Ctrl Pts',(-6.02279786501192,5.97674408746066,7.78079086085649));
#36576=CARTESIAN_POINT('Ctrl Pts',(-5.97860852335649,6.10429897334357,7.70442875673926));
#36577=CARTESIAN_POINT('Ctrl Pts',(-5.88754256740064,6.24419084675625,7.63901853366117));
#36578=CARTESIAN_POINT('Ctrl Pts',(-5.75869070430417,6.37188881584455,7.59917623945032));
#36579=CARTESIAN_POINT('Ctrl Pts',(-5.64770213594862,6.4452055625109,7.59265250311272));
#36580=CARTESIAN_POINT('Ctrl Pts',(-5.58549485259654,6.47719013590213,7.59599015744902));
#36581=CARTESIAN_POINT('Ctrl Pts',(-5.57875178789665,6.48055677169745,7.59642913085163));
#36582=CARTESIAN_POINT('Ctrl Pts',(-6.32411122307629,5.79795599112006,7.77364115833111));
#36583=CARTESIAN_POINT('Ctrl Pts',(-6.32542204434578,5.84442666570434,7.73827529736239));
#36584=CARTESIAN_POINT('Ctrl Pts',(-6.31518050053343,5.9605959104862,7.65551810315682));
#36585=CARTESIAN_POINT('Ctrl Pts',(-6.2493862815084,6.14925123617853,7.54144392085583));
#36586=CARTESIAN_POINT('Ctrl Pts',(-6.1169400851386,6.35166156312029,7.44482117005616));
#36587=CARTESIAN_POINT('Ctrl Pts',(-5.93147165227156,6.53460575418067,7.38562894665993));
#36588=CARTESIAN_POINT('Ctrl Pts',(-5.77166730225767,6.63980826589821,7.37507275783575));
#36589=CARTESIAN_POINT('Ctrl Pts',(-5.68156295277533,6.68599000877552,7.37946868324932));
#36590=CARTESIAN_POINT('Ctrl Pts',(-5.67178918527753,6.69085488542317,7.3800595832833));
#36591=CARTESIAN_POINT('',(-5.72001857355568,6.64700964721696,7.39409311766332));
#36592=CARTESIAN_POINT('Origin',(-5.8987579215779,6.95916957771643,7.74135710698279));
#36593=CARTESIAN_POINT('',(-5.99999998746764,6.44014606542557,7.42970690919143));
#36594=CARTESIAN_POINT('Ctrl Pts',(-6.00000002220353,6.44014619802302,7.42970706216311));
#36595=CARTESIAN_POINT('Ctrl Pts',(-5.95906904703314,6.47976101005719,7.41728042107866));
#36596=CARTESIAN_POINT('Ctrl Pts',(-5.91529115572005,6.51678863678942,7.40807178321115));
#36597=CARTESIAN_POINT('Ctrl Pts',(-5.86865681612109,6.55130284293238,7.40207822663037));
#36598=CARTESIAN_POINT('Ctrl Pts',(-5.82202247652213,6.58581704907534,7.3960846700496));
#36599=CARTESIAN_POINT('Ctrl Pts',(-5.77253147336175,6.61781748381247,7.39330579278897));
#36600=CARTESIAN_POINT('Ctrl Pts',(-5.72001867760868,6.6470098289392,7.39409331980232));
#36601=CARTESIAN_POINT('Ctrl Pts',(-5.99998887464722,6.09546019355616,8.13557730976511));
#36602=CARTESIAN_POINT('Ctrl Pts',(-5.99998548962721,6.09908966555976,8.10734133180911));
#36603=CARTESIAN_POINT('Ctrl Pts',(-5.99998569058181,6.10340241851193,8.0796204247349));
#36604=CARTESIAN_POINT('Ctrl Pts',(-5.99998246305821,6.10842621161674,8.05243269583343));
#36605=CARTESIAN_POINT('Ctrl Pts',(-5.99998128988673,6.11025230849801,8.04255023731652));
#36606=CARTESIAN_POINT('Ctrl Pts',(-5.99997935490184,6.11217188802552,8.03273815173794));
#36607=CARTESIAN_POINT('Ctrl Pts',(-5.99997573731162,6.11418488655801,8.02299697961942));
#36608=CARTESIAN_POINT('Ctrl Pts',(-5.99996193796901,6.12186349433934,7.98583915817959));
#36609=CARTESIAN_POINT('Ctrl Pts',(-5.99992695587156,6.13090233978705,7.94971604561126));
#36610=CARTESIAN_POINT('Ctrl Pts',(-5.99991596216633,6.14126851094962,7.91458364660781));
#36611=CARTESIAN_POINT('Ctrl Pts',(-5.99990553965583,6.15109609186687,7.8812766050195));
#36612=CARTESIAN_POINT('Ctrl Pts',(-5.99990306372909,6.1621404443772,7.84887553209668));
#36613=CARTESIAN_POINT('Ctrl Pts',(-5.99990503429433,6.17439332140972,7.81739276335889));
#36614=CARTESIAN_POINT('Ctrl Pts',(-5.99990615565766,6.18136590304599,7.79947728321676));
#36615=CARTESIAN_POINT('Ctrl Pts',(-5.99990893829224,6.1887300454836,7.78185864041553));
#36616=CARTESIAN_POINT('Ctrl Pts',(-5.99991563402973,6.19649203440266,7.7645342226708));
#36617=CARTESIAN_POINT('Ctrl Pts',(-5.99991845242869,6.1997592445525,7.75724195337154));
#36618=CARTESIAN_POINT('Ctrl Pts',(-5.99992643742721,6.20320569045125,7.74975283151406));
#36619=CARTESIAN_POINT('Ctrl Pts',(-5.99993172356156,6.20668978085882,7.74241141820367));
#36620=CARTESIAN_POINT('Ctrl Pts',(-5.99993707718041,6.21021835029205,7.73497628203515));
#36621=CARTESIAN_POINT('Ctrl Pts',(-5.99993939007667,6.21378540141034,7.72769295558882));
#36622=CARTESIAN_POINT('Ctrl Pts',(-5.99994434414875,6.21719223499444,7.72090801999296));
#36623=CARTESIAN_POINT('Ctrl Pts',(-5.99994517942683,6.2177666419404,7.71976405036899));
#36624=CARTESIAN_POINT('Ctrl Pts',(-5.99994612554702,6.21833638344123,7.71863421773668));
#36625=CARTESIAN_POINT('Ctrl Pts',(-5.99994725311684,6.21890037837763,7.71752014509275));
#36626=CARTESIAN_POINT('Ctrl Pts',(-5.9999739635128,6.23226055161525,7.69112947638033));
#36627=CARTESIAN_POINT('Ctrl Pts',(-5.99995992531238,6.24654172946454,7.66574054511034));
#36628=CARTESIAN_POINT('Ctrl Pts',(-5.99993534254208,6.26167056867004,7.64131941866416));
#36629=CARTESIAN_POINT('Ctrl Pts',(-5.9999120470352,6.27600719443074,7.61817709123521));
#36630=CARTESIAN_POINT('Ctrl Pts',(-5.9998806732924,6.29110549459433,7.59590273476373));
#36631=CARTESIAN_POINT('Ctrl Pts',(-5.99986484539969,6.30694581008885,7.57447640629471));
#36632=CARTESIAN_POINT('Ctrl Pts',(-5.99984908651931,6.32271705907836,7.55314350030978));
#36633=CARTESIAN_POINT('Ctrl Pts',(-5.99985008116883,6.33922486146098,7.53265019329587));
#36634=CARTESIAN_POINT('Ctrl Pts',(-5.99987209092983,6.35648736495212,7.51299767308082));
#36635=CARTESIAN_POINT('Ctrl Pts',(-5.99989343825301,6.37323031099825,7.49393664373473));
#36636=CARTESIAN_POINT('Ctrl Pts',(-5.99993510456538,6.39068433272936,7.47566639388829));
#36637=CARTESIAN_POINT('Ctrl Pts',(-5.99996736242159,6.40888164182049,7.45821957055967));
#36638=CARTESIAN_POINT('Ctrl Pts',(-5.99998541956038,6.41906803901105,7.44845327647471));
#36639=CARTESIAN_POINT('Ctrl Pts',(-5.99999986746529,6.42948753754744,7.43894559930852));
#36640=CARTESIAN_POINT('Ctrl Pts',(-5.99999986894896,6.44014594987542,7.42970677588644));
#36641=CARTESIAN_POINT('Ctrl Pts',(6.05076594298383,10.3129892342082,1.22620019878532));
#36642=CARTESIAN_POINT('Ctrl Pts',(6.05141715339522,10.3095618497228,1.25273481980966));
#36643=CARTESIAN_POINT('Ctrl Pts',(6.04716023846436,10.3030216335477,1.32055479041099));
#36644=CARTESIAN_POINT('Ctrl Pts',(6.01566436669805,10.3011133365561,1.43300903845304));
#36645=CARTESIAN_POINT('Ctrl Pts',(5.94752234234302,10.3114150966028,1.55314313783514));
#36646=CARTESIAN_POINT('Ctrl Pts',(5.84909941351561,10.3344537772754,1.65630672975824));
#36647=CARTESIAN_POINT('Ctrl Pts',(5.76414056613767,10.358630474181,1.70872457384661));
#36648=CARTESIAN_POINT('Ctrl Pts',(5.71688012150772,10.3731536343596,1.72893354987749));
#36649=CARTESIAN_POINT('Ctrl Pts',(5.71193038493101,10.3746858130558,1.73095764713588));
#36650=CARTESIAN_POINT('Ctrl Pts',(5.91195398463708,10.0312610302219,1.19351178706232));
#36651=CARTESIAN_POINT('Ctrl Pts',(5.91255178532836,10.0281685311092,1.21738790649602));
#36652=CARTESIAN_POINT('Ctrl Pts',(5.90864761849278,10.0223078652808,1.27867029765757));
#36653=CARTESIAN_POINT('Ctrl Pts',(5.8794545808466,10.0209225268295,1.38114550802042));
#36654=CARTESIAN_POINT('Ctrl Pts',(5.81592995132105,10.0310514474921,1.4912833203987));
#36655=CARTESIAN_POINT('Ctrl Pts',(5.7239554292842,10.053099985886,1.58614623982501));
#36656=CARTESIAN_POINT('Ctrl Pts',(5.64456681575892,10.075974957363,1.6343728591383));
#36657=CARTESIAN_POINT('Ctrl Pts',(5.60046479938737,10.0896338081727,1.65295820241385));
#36658=CARTESIAN_POINT('Ctrl Pts',(5.59584656161539,10.0910739675031,1.65481961370909));
#36659=CARTESIAN_POINT('Ctrl Pts',(6.02852441748326,9.74057618693592,1.15323046382272));
#36660=CARTESIAN_POINT('Ctrl Pts',(6.02946196048018,9.735828951765,1.19002894035524));
#36661=CARTESIAN_POINT('Ctrl Pts',(6.02330619665441,9.72690801122379,1.28256626988032));
#36662=CARTESIAN_POINT('Ctrl Pts',(5.98006577432888,9.72424621979883,1.43102946984614));
#36663=CARTESIAN_POINT('Ctrl Pts',(5.88925233756573,9.73731875155346,1.58604362930984));
#36664=CARTESIAN_POINT('Ctrl Pts',(5.75974090924188,9.76671869076749,1.71798797258565));
#36665=CARTESIAN_POINT('Ctrl Pts',(5.64791671092265,9.79794966063946,1.78532744029789));
#36666=CARTESIAN_POINT('Ctrl Pts',(5.5852625769881,9.81697297564258,1.81150815891621));
#36667=CARTESIAN_POINT('Ctrl Pts',(5.57869530741879,9.81898275134499,1.81413330240522));
#36668=CARTESIAN_POINT('Ctrl Pts',(6.32406684675164,9.63147436024286,1.13176005092088));
#36669=CARTESIAN_POINT('Ctrl Pts',(6.32551458769723,9.62416742424068,1.18859131639995));
#36670=CARTESIAN_POINT('Ctrl Pts',(6.31597877248707,9.61045235182775,1.32968892101247));
#36671=CARTESIAN_POINT('Ctrl Pts',(6.25154861315667,9.60555139342322,1.54996264460781));
#36672=CARTESIAN_POINT('Ctrl Pts',(6.11942760311156,9.62275449059315,1.7753099581504));
#36673=CARTESIAN_POINT('Ctrl Pts',(5.93299887882128,9.66302863226776,1.96541145925877));
#36674=CARTESIAN_POINT('Ctrl Pts',(5.77199435470564,9.70679608296843,2.06263963985118));
#36675=CARTESIAN_POINT('Ctrl Pts',(5.68123821408197,9.73389630361412,2.10065607808985));
#36676=CARTESIAN_POINT('Ctrl Pts',(5.67171894552347,9.73676395577024,2.1044707560063));
#36677=CARTESIAN_POINT('',(5.73278523421135,10.3449523238712,1.71289271684915));
#36678=CARTESIAN_POINT('',(5.72001553852396,9.72697684558834,2.05943436519823));
#36679=CARTESIAN_POINT('Origin',(5.89875809739164,10.1838003793526,2.15614465708099));
#36680=CARTESIAN_POINT('',(5.999999988605,9.65438797224885,1.86247647806753));
#36681=CARTESIAN_POINT('Ctrl Pts',(6.00000005199597,9.65438817668948,1.86247651750723));
#36682=CARTESIAN_POINT('Ctrl Pts',(5.95914560526064,9.66341676699531,1.90292211689277));
#36683=CARTESIAN_POINT('Ctrl Pts',(5.91541907066705,9.67394092583593,1.93956812259589));
#36684=CARTESIAN_POINT('Ctrl Pts',(5.86878902309983,9.6860048617978,1.97246300793595));
#36685=CARTESIAN_POINT('Ctrl Pts',(5.8221589755326,9.69806879775966,2.005357893276));
#36686=CARTESIAN_POINT('Ctrl Pts',(5.7726251819321,9.7116719571993,2.0345015539125));
#36687=CARTESIAN_POINT('Ctrl Pts',(5.72001606109123,9.72697818110479,2.05943464798176));
#36688=CARTESIAN_POINT('',(5.99998738510661,10.0933419068162,1.21103477369025));
#36689=CARTESIAN_POINT('Ctrl Pts',(5.99998738510661,10.0933419068162,1.21103477369025));
#36690=CARTESIAN_POINT('Ctrl Pts',(5.99998486187685,10.0708534763626,1.22818435848599));
#36691=CARTESIAN_POINT('Ctrl Pts',(5.99998575125151,10.0491424232848,1.24566234602253));
#36692=CARTESIAN_POINT('Ctrl Pts',(5.99998220172071,10.0282383838849,1.26348392485136));
#36693=CARTESIAN_POINT('Ctrl Pts',(5.9999810788975,10.0216258083253,1.26912142554399));
#36694=CARTESIAN_POINT('Ctrl Pts',(5.9999792883417,10.0150937600636,1.27479302580716));
#36695=CARTESIAN_POINT('Ctrl Pts',(5.99997621692473,10.0086425621615,1.28049853326882));
#36696=CARTESIAN_POINT('Ctrl Pts',(5.99996211490628,9.97902271150216,1.30669464157516));
#36697=CARTESIAN_POINT('Ctrl Pts',(5.99992503046489,9.95111114927153,1.33360519795231));
#36698=CARTESIAN_POINT('Ctrl Pts',(5.99991423108135,9.92484903553856,1.36122131801052));
#36699=CARTESIAN_POINT('Ctrl Pts',(5.99990487784502,9.90210368572874,1.38513935893827));
#36700=CARTESIAN_POINT('Ctrl Pts',(5.99990278201543,9.88061743467843,1.4095991312432));
#36701=CARTESIAN_POINT('Ctrl Pts',(5.99990421744039,9.86039663880491,1.43458775228001));
#36702=CARTESIAN_POINT('Ctrl Pts',(5.9999051516139,9.84723695980441,1.45085032837081));
#36703=CARTESIAN_POINT('Ctrl Pts',(5.99990793441967,9.83461274768095,1.46733727486941));
#36704=CARTESIAN_POINT('Ctrl Pts',(5.99991541529783,9.82252505006016,1.48405677334895));
#36705=CARTESIAN_POINT('Ctrl Pts',(5.99991831505952,9.81783957843132,1.49053763829377));
#36706=CARTESIAN_POINT('Ctrl Pts',(5.99992637047857,9.8130737739939,1.49727174220381));
#36707=CARTESIAN_POINT('Ctrl Pts',(5.99993172018365,9.80845502960049,1.50396438277711));
#36708=CARTESIAN_POINT('Ctrl Pts',(5.99993713803762,9.80377744788307,1.51074227965135));
#36709=CARTESIAN_POINT('Ctrl Pts',(5.99993950798813,9.79925089617219,1.51747738340903));
#36710=CARTESIAN_POINT('Ctrl Pts',(5.99994451737579,9.79507593996524,1.52382456677347));
#36711=CARTESIAN_POINT('Ctrl Pts',(5.99994535116368,9.79438103908289,1.52488102415929));
#36712=CARTESIAN_POINT('Ctrl Pts',(5.99994629295769,9.79369579857702,1.52592665612043));
#36713=CARTESIAN_POINT('Ctrl Pts',(5.99994741064945,9.7930210497323,1.52695978247457));
#36714=CARTESIAN_POINT('Ctrl Pts',(5.99997420500895,9.7768453349225,1.55172686047367));
#36715=CARTESIAN_POINT('Ctrl Pts',(5.99996028565684,9.76199767903545,1.57679079684059));
#36716=CARTESIAN_POINT('Ctrl Pts',(5.99993572431047,9.74841211997671,1.60210482022966));
#36717=CARTESIAN_POINT('Ctrl Pts',(5.99991395264929,9.73636961284882,1.62454366914126));
#36718=CARTESIAN_POINT('Ctrl Pts',(5.99988491856912,9.72531845430559,1.64718009827664));
#36719=CARTESIAN_POINT('Ctrl Pts',(5.9998683047256,9.71523554983366,1.67000758547262));
#36720=CARTESIAN_POINT('Ctrl Pts',(5.99985059014724,9.70448461185646,1.69434748670864));
#36721=CARTESIAN_POINT('Ctrl Pts',(5.99984847396064,9.69483366624625,1.71890568866634));
#36722=CARTESIAN_POINT('Ctrl Pts',(5.99986814609526,9.68629032422623,1.74369683123673));
#36723=CARTESIAN_POINT('Ctrl Pts',(5.99988721410777,9.67800934426949,1.76772664933938));
#36724=CARTESIAN_POINT('Ctrl Pts',(5.99992732030898,9.67076938299242,1.79197637886837));
#36725=CARTESIAN_POINT('Ctrl Pts',(5.99996104571487,9.66461289211092,1.81645815869563));
#36726=CARTESIAN_POINT('Ctrl Pts',(5.99998205295574,9.6607780713449,1.83170763107814));
#36727=CARTESIAN_POINT('Ctrl Pts',(5.99999988350975,9.65736434128087,1.84704704982016));
#36728=CARTESIAN_POINT('Ctrl Pts',(5.99999988745995,9.6543877773096,1.86247644046082));
#36729=CARTESIAN_POINT('Ctrl Pts',(5.99998738510661,10.0933419068162,1.21103477369025));
#36730=CARTESIAN_POINT('Ctrl Pts',(5.99998441904465,10.0961480732035,1.22745270725951));
#36731=CARTESIAN_POINT('Ctrl Pts',(5.99923974683307,10.0995757628645,1.24479982112044));
#36732=CARTESIAN_POINT('Ctrl Pts',(5.99754903871016,10.1037122322766,1.26297222218984));
#36733=CARTESIAN_POINT('Ctrl Pts',(5.99682966762832,10.1054722382975,1.27070430772234));
#36734=CARTESIAN_POINT('Ctrl Pts',(5.99593880558416,10.1073606499676,1.27858524270412));
#36735=CARTESIAN_POINT('Ctrl Pts',(5.99485951760923,10.109384630221,1.28660438308776));
#36736=CARTESIAN_POINT('Ctrl Pts',(5.99246751490685,10.1138703340814,1.30437703127238));
#36737=CARTESIAN_POINT('Ctrl Pts',(5.98914967992163,10.1190220691058,1.32283170632383));
#36738=CARTESIAN_POINT('Ctrl Pts',(5.98476329112109,10.1249037655265,1.34182449996128));
#36739=CARTESIAN_POINT('Ctrl Pts',(5.98056287386319,10.130536093228,1.3600120482608));
#36740=CARTESIAN_POINT('Ctrl Pts',(5.97538295501154,10.1368376689458,1.37869350108863));
#36741=CARTESIAN_POINT('Ctrl Pts',(5.96909418209851,10.1438652718173,1.39769699124418));
#36742=CARTESIAN_POINT('Ctrl Pts',(5.96738486869547,10.1457754021314,1.40286221518796));
#36743=CARTESIAN_POINT('Ctrl Pts',(5.96559359347928,10.1477391785027,1.40805094260893));
#36744=CARTESIAN_POINT('Ctrl Pts',(5.96371764325191,10.1497577676557,1.41325904326785));
#36745=CARTESIAN_POINT('Ctrl Pts',(5.96344414271051,10.1500520639639,1.41401834824787));
#36746=CARTESIAN_POINT('Ctrl Pts',(5.96316884223256,10.1503475253814,1.41477806446667));
#36747=CARTESIAN_POINT('Ctrl Pts',(5.96289173637458,10.1506441544023,1.41553818059405));
#36748=CARTESIAN_POINT('Ctrl Pts',(5.95830642825136,10.1555525149422,1.42811592499401));
#36749=CARTESIAN_POINT('Ctrl Pts',(5.9532266748501,10.1607806414693,1.44080394687483));
#36750=CARTESIAN_POINT('Ctrl Pts',(5.94762863090485,10.1663393817787,1.45354595744594));
#36751=CARTESIAN_POINT('Ctrl Pts',(5.94482960893222,10.1691187519334,1.4599169627315));
#36752=CARTESIAN_POINT('Ctrl Pts',(5.94190097307532,10.1719807843508,1.46630144268669));
#36753=CARTESIAN_POINT('Ctrl Pts',(5.9388399270167,10.1749267438764,1.47269125767461));
#36754=CARTESIAN_POINT('Ctrl Pts',(5.93730940398739,10.1763997236392,1.47588616516857));
#36755=CARTESIAN_POINT('Ctrl Pts',(5.93574577516673,10.1778936858389,1.47908240474024));
#36756=CARTESIAN_POINT('Ctrl Pts',(5.93414868741022,10.1794087883726,1.48227891189157));
#36757=CARTESIAN_POINT('Ctrl Pts',(5.93308462549516,10.1804182275201,1.4844085891789));
#36758=CARTESIAN_POINT('Ctrl Pts',(5.93173682914368,10.1816910636254,1.4870663279203));
#36759=CARTESIAN_POINT('Ctrl Pts',(5.93064071602891,10.1827204106847,1.48919534164818));
#36760=CARTESIAN_POINT('Ctrl Pts',(5.93009163462014,10.1832360466403,1.49026183911203));
#36761=CARTESIAN_POINT('Ctrl Pts',(5.92960660183023,10.1836902190877,1.49119622911705));
#36762=CARTESIAN_POINT('Ctrl Pts',(5.92925668657071,10.1840176761403,1.49186814347237));
#36763=CARTESIAN_POINT('Ctrl Pts',(5.92324503182682,10.1896434917922,1.50341184444495));
#36764=CARTESIAN_POINT('Ctrl Pts',(5.91644346846693,10.1958846454291,1.51562382600558));
#36765=CARTESIAN_POINT('Ctrl Pts',(5.90871316153225,10.2027984780577,1.5283486336031));
#36766=CARTESIAN_POINT('Ctrl Pts',(5.90756562565091,10.2038248113049,1.53023758489891));
#36767=CARTESIAN_POINT('Ctrl Pts',(5.9063976103785,10.2048659743285,1.53213774426546));
#36768=CARTESIAN_POINT('Ctrl Pts',(5.90520864835011,10.2059221612598,1.53404850168093));
#36769=CARTESIAN_POINT('Ctrl Pts',(5.89737762539582,10.2128786694627,1.54663358415056));
#36770=CARTESIAN_POINT('Ctrl Pts',(5.88863728924836,10.2204871202784,1.55968229442971));
#36771=CARTESIAN_POINT('Ctrl Pts',(5.87887072452031,10.2287962590974,1.57300928454709));
#36772=CARTESIAN_POINT('Ctrl Pts',(5.86988433341336,10.2364416465257,1.58527168681525));
#36773=CARTESIAN_POINT('Ctrl Pts',(5.86002895799353,10.244680267378,1.5977698555925));
#36774=CARTESIAN_POINT('Ctrl Pts',(5.84922133220102,10.2535479575985,1.6103174241131));
#36775=CARTESIAN_POINT('Ctrl Pts',(5.84083255094556,10.260430978433,1.62005673315545));
#36776=CARTESIAN_POINT('Ctrl Pts',(5.83187017546044,10.2676929521663,1.62982514960955));
#36777=CARTESIAN_POINT('Ctrl Pts',(5.82229987253264,10.2753496142587,1.63951416959187));
#36778=CARTESIAN_POINT('Ctrl Pts',(5.81046704628954,10.2848163942369,1.65149377888759));
#36779=CARTESIAN_POINT('Ctrl Pts',(5.79770347959874,10.2948870147308,1.66335292667562));
#36780=CARTESIAN_POINT('Ctrl Pts',(5.78397884046087,10.3055776305931,1.67487325685049));
#36781=CARTESIAN_POINT('Ctrl Pts',(5.77112683449969,10.3155885210371,1.68566110712435));
#36782=CARTESIAN_POINT('Ctrl Pts',(5.75743196461773,10.3261430317943,1.6961520930176));
#36783=CARTESIAN_POINT('Ctrl Pts',(5.74289155719727,10.3372485293759,1.70612653191595));
#36784=CARTESIAN_POINT('Ctrl Pts',(5.73956598976375,10.3397884912919,1.70840780700054));
#36785=CARTESIAN_POINT('Ctrl Pts',(5.73619629460833,10.3423572505822,1.71066187634557));
#36786=CARTESIAN_POINT('Ctrl Pts',(5.73278262924252,10.3449548518058,1.71288576550861));
#36787=CARTESIAN_POINT('Ctrl Pts',(5.99928507670662,19.6591035996724,0.0581387347865464));
#36788=CARTESIAN_POINT('Ctrl Pts',(5.99928507670662,19.6322147711509,0.0775485171687107));
#36789=CARTESIAN_POINT('Ctrl Pts',(5.99928507670662,19.20584634456,0.382071892402484));
#36790=CARTESIAN_POINT('Ctrl Pts',(5.99928507670662,18.3334692836715,0.906208303978892));
#36791=CARTESIAN_POINT('Ctrl Pts',(5.99928507670662,16.9710191689203,1.46998611787121));
#36792=CARTESIAN_POINT('Ctrl Pts',(5.99928507670662,15.5398231880517,1.82605992904551));
#36793=CARTESIAN_POINT('Ctrl Pts',(5.99928507670662,14.0709530321673,1.9661847991881));
#36794=CARTESIAN_POINT('Ctrl Pts',(5.99928507670662,12.5966749488329,1.88736642753476));
#36795=CARTESIAN_POINT('Ctrl Pts',(5.99928507670662,11.233524511613,1.60731006115195));
#36796=CARTESIAN_POINT('Ctrl Pts',(5.99928507670662,10.3852007283801,1.30897054759059));
#36797=CARTESIAN_POINT('Ctrl Pts',(5.99928507670662,10.0105704034592,1.15061624350596));
#36798=CARTESIAN_POINT('Ctrl Pts',(6.0106308768628,19.7700374649892,0.211790355550257));
#36799=CARTESIAN_POINT('Ctrl Pts',(6.0106308768628,19.7426318213209,0.231572972437534));
#36800=CARTESIAN_POINT('Ctrl Pts',(6.0106308768628,19.3080752298907,0.541942236510507));
#36801=CARTESIAN_POINT('Ctrl Pts',(6.0106308768628,18.4191308604644,1.07604164186386));
#36802=CARTESIAN_POINT('Ctrl Pts',(6.0106308768628,17.030425424612,1.6506818513714));
#36803=CARTESIAN_POINT('Ctrl Pts',(6.0106308768628,15.5719791864793,2.01353171875612));
#36804=CARTESIAN_POINT('Ctrl Pts',(6.0106308768628,14.0748590038713,2.15635960358311));
#36805=CARTESIAN_POINT('Ctrl Pts',(6.0106308768628,12.5724428536086,2.07602891618263));
#36806=CARTESIAN_POINT('Ctrl Pts',(6.0106308768628,11.1830961575752,1.79059626133241));
#36807=CARTESIAN_POINT('Ctrl Pts',(6.0106308768628,10.3186145483331,1.48657404108104));
#36808=CARTESIAN_POINT('Ctrl Pts',(6.0106308768628,9.93678102105085,1.32517327201325));
#36809=CARTESIAN_POINT('Ctrl Pts',(5.90351527164667,19.8620727363884,0.339266023847184));
#36810=CARTESIAN_POINT('Ctrl Pts',(5.90351527164667,19.8342383217458,0.359357959490708));
#36811=CARTESIAN_POINT('Ctrl Pts',(5.90351527164667,19.3928884938992,0.674577212014692));
#36812=CARTESIAN_POINT('Ctrl Pts',(5.90351527164667,18.4901992077698,1.21694232444669));
#36813=CARTESIAN_POINT('Ctrl Pts',(5.90351527164667,17.0797112838011,1.80059442158608));
#36814=CARTESIAN_POINT('Ctrl Pts',(5.90351527164667,15.5986571178186,2.16906598231467));
#36815=CARTESIAN_POINT('Ctrl Pts',(5.90351527164667,14.0780995577289,2.31413639866398));
#36816=CARTESIAN_POINT('Ctrl Pts',(5.90351527164667,12.5523389164164,2.23255103227451));
#36817=CARTESIAN_POINT('Ctrl Pts',(5.90351527164667,11.1412587327508,1.94265798864203));
#36818=CARTESIAN_POINT('Ctrl Pts',(5.90351527164667,10.2633719302693,1.63392116252431));
#36819=CARTESIAN_POINT('Ctrl Pts',(5.90351527164667,9.87556233172656,1.46999292151928));
#36820=CARTESIAN_POINT('Ctrl Pts',(5.72195021115539,19.8960951816937,0.386389630772639));
#36821=CARTESIAN_POINT('Ctrl Pts',(5.72195021115539,19.8681022643737,0.406595911496531));
#36822=CARTESIAN_POINT('Ctrl Pts',(5.72195021115539,19.4242411980539,0.723608046948767));
#36823=CARTESIAN_POINT('Ctrl Pts',(5.72195021115539,18.5164708634373,1.2690287223504));
#36824=CARTESIAN_POINT('Ctrl Pts',(5.72195021115539,17.0979306623425,1.85601222112912));
#36825=CARTESIAN_POINT('Ctrl Pts',(5.72195021115539,15.608519081026,2.22656193897816));
#36826=CARTESIAN_POINT('Ctrl Pts',(5.72195021115539,14.0792974850575,2.37246134626695));
#36827=CARTESIAN_POINT('Ctrl Pts',(5.72195021115539,12.5449071449564,2.29041216587778));
#36828=CARTESIAN_POINT('Ctrl Pts',(5.72195021115539,11.1257927980475,1.99887026163753));
#36829=CARTESIAN_POINT('Ctrl Pts',(5.72195021115539,10.2429505317845,1.68839059912861));
#36830=CARTESIAN_POINT('Ctrl Pts',(5.72195021115539,9.85293177413904,1.52352803398365));
#36831=CARTESIAN_POINT('',(6.,19.5919343770476,0.135488060647564));
#36832=CARTESIAN_POINT('Ctrl Pts',(5.99999999999968,19.5919343770476,0.135488060647564));
#36833=CARTESIAN_POINT('Ctrl Pts',(5.99999999999968,19.4672328159283,0.223609584749507));
#36834=CARTESIAN_POINT('Ctrl Pts',(6.00000000003741,19.3409290210282,0.30857593928506));
#36835=CARTESIAN_POINT('Ctrl Pts',(5.99999999795218,19.2129689489122,0.390478679261728));
#36836=CARTESIAN_POINT('Ctrl Pts',(5.99999999586003,19.0845842822652,0.472653187258653));
#36837=CARTESIAN_POINT('Ctrl Pts',(5.99999999148612,18.9545319213896,0.551743936355476));
#36838=CARTESIAN_POINT('Ctrl Pts',(5.99999999087353,18.8227278694456,0.627799960860205));
#36839=CARTESIAN_POINT('Ctrl Pts',(5.99999999026193,18.6911386719661,0.70373200604732));
#36840=CARTESIAN_POINT('Ctrl Pts',(5.9999999969562,18.5578030768095,0.776639422345871));
#36841=CARTESIAN_POINT('Ctrl Pts',(5.99999999953308,18.4226144050266,0.846524611534863));
#36842=CARTESIAN_POINT('Ctrl Pts',(5.99999999982098,18.4075105210493,0.854332497915586));
#36843=CARTESIAN_POINT('Ctrl Pts',(5.99999999999968,18.3923834863004,0.862102610062003));
#36844=CARTESIAN_POINT('Ctrl Pts',(5.99999999999968,18.3772331375584,0.869834913416259));
#36845=CARTESIAN_POINT('Ctrl Pts',(5.99999999999968,18.3604577106659,0.878396610037155));
#36846=CARTESIAN_POINT('Ctrl Pts',(5.99999999977969,18.3436541191937,0.886912855498554));
#36847=CARTESIAN_POINT('Ctrl Pts',(5.99999999940206,18.3268228429537,0.895383270618578));
#36848=CARTESIAN_POINT('Ctrl Pts',(5.99999999572729,18.1630329068859,0.97781128921898));
#36849=CARTESIAN_POINT('Ctrl Pts',(5.99999998184252,17.9966189014925,1.0558956786728));
#36850=CARTESIAN_POINT('Ctrl Pts',(5.99999998033329,17.8280125915752,1.12938237918269));
#36851=CARTESIAN_POINT('Ctrl Pts',(5.99999997882266,17.6592495761256,1.20293737946452));
#36852=CARTESIAN_POINT('Ctrl Pts',(5.99999998730998,17.4882905775836,1.27188592951145));
#36853=CARTESIAN_POINT('Ctrl Pts',(5.99999999411981,17.3155939777246,1.33601879718248));
#36854=CARTESIAN_POINT('Ctrl Pts',(5.99999999739296,17.2325870839331,1.36684436143596));
#36855=CARTESIAN_POINT('Ctrl Pts',(5.99999999999968,17.1491790978227,1.39655807182192));
#36856=CARTESIAN_POINT('Ctrl Pts',(5.99999999999968,17.0654225833735,1.42514064586644));
#36857=CARTESIAN_POINT('Ctrl Pts',(5.99999999999968,17.0325894366093,1.43634521729203));
#36858=CARTESIAN_POINT('Ctrl Pts',(5.99999999960408,16.9997023256303,1.44737475909724));
#36859=CARTESIAN_POINT('Ctrl Pts',(5.99999999898859,16.9667622518599,1.45822900233135));
#36860=CARTESIAN_POINT('Ctrl Pts',(5.99999999507854,16.7575009061637,1.52718372178683));
#36861=CARTESIAN_POINT('Ctrl Pts',(5.99999998615649,16.5461037121443,1.5890678586064));
#36862=CARTESIAN_POINT('Ctrl Pts',(5.99999998771978,16.332871847101,1.64383796968629));
#36863=CARTESIAN_POINT('Ctrl Pts',(5.99999998928308,16.1196399820578,1.69860808076618));
#36864=CARTESIAN_POINT('Ctrl Pts',(5.99999999999968,15.9045728433345,1.74626433387793));
#36865=CARTESIAN_POINT('Ctrl Pts',(5.99999999999968,15.687957017083,1.7867113382546));
#36866=CARTESIAN_POINT('Ctrl Pts',(5.99999999999968,15.6384082465009,1.79596319845002));
#36867=CARTESIAN_POINT('Ctrl Pts',(5.99999999934663,15.5887787586434,1.80484044751495));
#36868=CARTESIAN_POINT('Ctrl Pts',(5.99999999845568,15.5390764076834,1.81334072030503));
#36869=CARTESIAN_POINT('Ctrl Pts',(5.99999999449756,15.3182715860499,1.85110354602646));
#36870=CARTESIAN_POINT('Ctrl Pts',(5.99999998895126,15.0960278363158,1.88142224228069));
#36871=CARTESIAN_POINT('Ctrl Pts',(5.99999999115147,14.8730346667746,1.90421141085561));
#36872=CARTESIAN_POINT('Ctrl Pts',(5.99999999312714,14.6727988930678,1.92467484841795));
#36873=CARTESIAN_POINT('Ctrl Pts',(5.99999999999968,14.4719593375783,1.93906781008501));
#36874=CARTESIAN_POINT('Ctrl Pts',(5.99999999999968,14.2710197375948,1.94736399718564));
#36875=CARTESIAN_POINT('Ctrl Pts',(5.99999999999968,14.2042157464008,1.95012213152083));
#36876=CARTESIAN_POINT('Ctrl Pts',(5.99999999913621,14.1374011154746,1.95220403825653));
#36877=CARTESIAN_POINT('Ctrl Pts',(5.99999999780769,14.0705840962199,1.95360927362166));
#36878=CARTESIAN_POINT('Ctrl Pts',(5.99999999336877,13.8473330129415,1.95830448931711));
#36879=CARTESIAN_POINT('Ctrl Pts',(5.99999998477708,13.6240549671328,1.95544941068481));
#36880=CARTESIAN_POINT('Ctrl Pts',(5.99999998688347,13.4010803985336,1.94504158174669));
#36881=CARTESIAN_POINT('Ctrl Pts',(5.99999998863002,13.2161971643747,1.93641174971364));
#36882=CARTESIAN_POINT('Ctrl Pts',(5.99999999999968,13.0315224106363,1.9225883059491));
#36883=CARTESIAN_POINT('Ctrl Pts',(5.99999999999968,12.847248931914,1.90354302871283));
#36884=CARTESIAN_POINT('Ctrl Pts',(5.99999999999968,12.7639691565099,1.89493578679314));
#36885=CARTESIAN_POINT('Ctrl Pts',(5.99999999683349,12.6807681678412,1.88527287357867));
#36886=CARTESIAN_POINT('Ctrl Pts',(5.9999999931907,12.5976921209349,1.87455549616479));
#36887=CARTESIAN_POINT('Ctrl Pts',(5.99999998466661,12.4032953145046,1.84947698051374));
#36888=CARTESIAN_POINT('Ctrl Pts',(5.99999997595973,12.2095833836002,1.81862087709688));
#36889=CARTESIAN_POINT('Ctrl Pts',(5.99999997954448,12.0171092535684,1.78211738648701));
#36890=CARTESIAN_POINT('Ctrl Pts',(5.99999998312923,11.8246351235367,1.74561389587715));
#36891=CARTESIAN_POINT('Ctrl Pts',(5.99999999999968,11.6333993074508,1.7034631726462));
#36892=CARTESIAN_POINT('Ctrl Pts',(5.99999999999968,11.4439401120787,1.65585043723543));
#36893=CARTESIAN_POINT('Ctrl Pts',(5.99999999999968,11.3471384627997,1.63152334503285));
#36894=CARTESIAN_POINT('Ctrl Pts',(5.99999999545162,11.2508119173546,1.6057505968365));
#36895=CARTESIAN_POINT('Ctrl Pts',(5.99999999307287,11.1549261368173,1.57853425346852));
#36896=CARTESIAN_POINT('Ctrl Pts',(5.99999998940933,11.0072519921261,1.53661823415922));
#36897=CARTESIAN_POINT('Ctrl Pts',(5.99999999031157,10.8606225700356,1.49128052602001));
#36898=CARTESIAN_POINT('Ctrl Pts',(5.99999999276237,10.7149492997484,1.44250629149568));
#36899=CARTESIAN_POINT('Ctrl Pts',(5.99999999520022,10.5700458283645,1.39398980056541));
#36900=CARTESIAN_POINT('Ctrl Pts',(5.99999999786777,10.4260879908288,1.34207286643751));
#36901=CARTESIAN_POINT('Ctrl Pts',(5.99999999875688,10.2830048093639,1.2866921338031));
#36902=CARTESIAN_POINT('Ctrl Pts',(5.99999999915078,10.2196135091128,1.26215635947515));
#36903=CARTESIAN_POINT('Ctrl Pts',(5.9999999993187,10.1563941419572,1.2369400707568));
#36904=CARTESIAN_POINT('Ctrl Pts',(5.99999999931442,10.0933419069091,1.21103477539414));
#36905=CARTESIAN_POINT('',(5.73644276520376,19.8089520716694,0.442549441855652));
#36906=CARTESIAN_POINT('Origin',(5.6,19.5919343769637,0.135488060672991));
#36907=CARTESIAN_POINT('Ctrl Pts',(5.73644276397656,19.8089520717766,0.442549442640921));
#36908=CARTESIAN_POINT('Ctrl Pts',(5.7370879225674,19.446718951205,0.69823623580988));
#36909=CARTESIAN_POINT('Ctrl Pts',(5.73762563118613,19.0680988842184,0.930502845521264));
#36910=CARTESIAN_POINT('Ctrl Pts',(5.73805595552339,18.676590268373,1.13733219036651));
#36911=CARTESIAN_POINT('Ctrl Pts',(5.73812189681018,18.61659695709,1.1690259431105));
#36912=CARTESIAN_POINT('Ctrl Pts',(5.73818531654776,18.556300916891,1.20012244044563));
#36913=CARTESIAN_POINT('Ctrl Pts',(5.73824621494312,18.4957146397251,1.23061447416638));
#36914=CARTESIAN_POINT('Ctrl Pts',(5.73865147315783,18.092533465989,1.43352864087569));
#36915=CARTESIAN_POINT('Ctrl Pts',(5.73894507726634,17.6765033902989,1.6096732180909));
#36916=CARTESIAN_POINT('Ctrl Pts',(5.7391270730799,17.2512590699236,1.75775966272543));
#36917=CARTESIAN_POINT('Ctrl Pts',(5.73915087282255,17.1956495194054,1.77712504923241));
#36918=CARTESIAN_POINT('Ctrl Pts',(5.73917276390775,17.1398823261237,1.79601063417806));
#36919=CARTESIAN_POINT('Ctrl Pts',(5.73919274639726,17.0839655556887,1.81441355455165));
#36920=CARTESIAN_POINT('Ctrl Pts',(5.73934700323792,16.652310413593,1.9564767521763));
#36921=CARTESIAN_POINT('Ctrl Pts',(5.73938752575625,16.2117458758467,2.06977630384664));
#36922=CARTESIAN_POINT('Ctrl Pts',(5.73931432087029,15.7661154481004,2.15354915603658));
#36923=CARTESIAN_POINT('Ctrl Pts',(5.73930537008875,15.7116280931828,2.16379208570551));
#36924=CARTESIAN_POINT('Ctrl Pts',(5.73929471903249,15.6570649397863,2.17359359951341));
#36925=CARTESIAN_POINT('Ctrl Pts',(5.73928236767428,15.6024329608079,2.1829523100585));
#36926=CARTESIAN_POINT('Ctrl Pts',(5.73918135759826,15.1556496796064,2.25948835146391));
#36927=CARTESIAN_POINT('Ctrl Pts',(5.73896663327029,14.7042676165308,2.30640958123039));
#36928=CARTESIAN_POINT('Ctrl Pts',(5.73863815933754,14.2522694751224,2.32359660893901));
#36929=CARTESIAN_POINT('Ctrl Pts',(5.73859603617049,14.1943056876852,2.32580065610097));
#36930=CARTESIAN_POINT('Ctrl Pts',(5.73855204231838,14.136331698548,2.32751571530993));
#36931=CARTESIAN_POINT('Ctrl Pts',(5.73850617766838,14.0783558454309,2.32874153312007));
#36932=CARTESIAN_POINT('Ctrl Pts',(5.73815298353712,13.6318958576921,2.33818130114516));
#36933=CARTESIAN_POINT('Ctrl Pts',(5.73768884856023,13.185329276007,2.31860847900135));
#36934=CARTESIAN_POINT('Ctrl Pts',(5.73711370893554,12.7423972566153,2.27028161135825));
#36935=CARTESIAN_POINT('Ctrl Pts',(5.73703020600255,12.6780891805479,2.26326516697304));
#36936=CARTESIAN_POINT('Ctrl Pts',(5.73694436300473,12.6138576339778,2.2556425960222));
#36937=CARTESIAN_POINT('Ctrl Pts',(5.73685617975576,12.5497139832806,2.24741467936474));
#36938=CARTESIAN_POINT('Ctrl Pts',(5.73622837211831,12.0930527208357,2.18883724001976));
#36939=CARTESIAN_POINT('Ctrl Pts',(5.73548194777951,11.6408504952097,2.09957923971377));
#36940=CARTESIAN_POINT('Ctrl Pts',(5.73461684134438,11.1969963232995,1.98082349864726));
#36941=CARTESIAN_POINT('Ctrl Pts',(5.73452245641432,11.1485709004022,1.96786699773642));
#36942=CARTESIAN_POINT('Ctrl Pts',(5.73442665879326,11.1002447987416,1.95455935976749));
#36943=CARTESIAN_POINT('Ctrl Pts',(5.73432944840997,11.0520230339019,1.94090210805598));
#36944=CARTESIAN_POINT('Ctrl Pts',(5.73384873497255,10.813562392646,1.87336586147213));
#36945=CARTESIAN_POINT('Ctrl Pts',(5.73333347377677,10.5776535681786,1.79728037334161));
#36946=CARTESIAN_POINT('Ctrl Pts',(5.73278365815296,10.34495385425,1.71288850793682));
#36947=CARTESIAN_POINT('Ctrl Pts',(5.99999999997507,19.5919300856952,-0.135488304642611));
#36948=CARTESIAN_POINT('Ctrl Pts',(5.99999999997507,19.5922326969838,-0.0451632714418701));
#36949=CARTESIAN_POINT('Ctrl Pts',(5.99999999997507,19.592232706457,0.045163275375177));
#36950=CARTESIAN_POINT('Ctrl Pts',(5.99999999997507,19.591929935039,0.135488872436178));
#36951=CARTESIAN_POINT('Ctrl Pts',(6.00000263486111,19.8293406274304,-0.136284098535555));
#36952=CARTESIAN_POINT('Ctrl Pts',(6.00000263486111,19.8296450131565,-0.0454285037137862));
#36953=CARTESIAN_POINT('Ctrl Pts',(6.00000263486111,19.8296450228453,0.0454285076464987));
#36954=CARTESIAN_POINT('Ctrl Pts',(6.00000263486111,19.8293404729502,0.136284669412338));
#36955=CARTESIAN_POINT('Ctrl Pts',(5.83074066841606,19.9958175555672,-0.136842124818485));
#36956=CARTESIAN_POINT('Ctrl Pts',(5.83074066841606,19.9961231855639,-0.0456144897847192));
#36957=CARTESIAN_POINT('Ctrl Pts',(5.83074066841606,19.9961231954044,0.0456144937168433));
#36958=CARTESIAN_POINT('Ctrl Pts',(5.83074066841606,19.9958173984079,0.136842697860198));
#36959=CARTESIAN_POINT('Ctrl Pts',(5.5933611004422,19.9918771871015,-0.136828916807151));
#36960=CARTESIAN_POINT('Ctrl Pts',(5.5933611004422,19.9921827876475,-0.0456100876498413));
#36961=CARTESIAN_POINT('Ctrl Pts',(5.5933611004422,19.9921827974873,0.045610091584508));
#36962=CARTESIAN_POINT('Ctrl Pts',(5.5933611004422,19.9918770300063,0.136829489796775));
#36963=CARTESIAN_POINT('',(5.99999999995612,19.5919320087503,-0.135481052873273));
#36964=CARTESIAN_POINT('',(5.59336167795915,19.9918770519504,-0.136828613280939));
#36965=CARTESIAN_POINT('Origin',(5.6,19.5919343769583,-0.135488060981343));
#36966=CARTESIAN_POINT('',(5.59336169562657,19.9918770422848,0.136828655448858));
#36967=CARTESIAN_POINT('Origin',(5.59336169594597,15.0903027128352,0.0604604316820303));
#36968=CARTESIAN_POINT('Origin',(5.6,19.5919343771351,0.13548806067611));
#36969=CARTESIAN_POINT('Ctrl Pts',(5.99999999999164,19.5919320204865,-0.135477553132434));
#36970=CARTESIAN_POINT('Ctrl Pts',(5.99999999999169,19.592033064822,-0.105317242394998));
#36971=CARTESIAN_POINT('Ctrl Pts',(5.9999999999997,19.5921021554901,-0.0751629212119529));
#36972=CARTESIAN_POINT('Ctrl Pts',(5.9999999999997,19.5921363906261,-0.0450478988915754));
#36973=CARTESIAN_POINT('Ctrl Pts',(5.9999999999997,19.5921706257621,-0.014932876571189));
#36974=CARTESIAN_POINT('Ctrl Pts',(5.9999999999997,19.5921700053662,0.0151428468865298));
#36975=CARTESIAN_POINT('Ctrl Pts',(5.9999999999997,19.5921361540918,0.0452268832839701));
#36976=CARTESIAN_POINT('Ctrl Pts',(5.9999999999997,19.5921023028175,0.0753109196814013));
#36977=CARTESIAN_POINT('Ctrl Pts',(5.9999999999997,19.5920352206648,0.105403269018554));
#36978=CARTESIAN_POINT('Ctrl Pts',(5.9999999999997,19.5919343770476,0.135488060647564));
#36979=CARTESIAN_POINT('Origin',(5.6,19.5919343769637,0.135488060672991));
#36980=CARTESIAN_POINT('Origin',(5.600000004204,19.5919343763224,0.135488059063745));
#36981=CARTESIAN_POINT('Ctrl Pts',(-5.69266556774165,19.9935543480601,0.076560747550209));
#36982=CARTESIAN_POINT('Ctrl Pts',(-5.6579015041137,19.9929008980439,0.0929956066630459));
#36983=CARTESIAN_POINT('Ctrl Pts',(-5.54372918028186,19.9908051431839,0.146474485765011));
#36984=CARTESIAN_POINT('Ctrl Pts',(-5.34117686668071,19.9873503305864,0.238480887060544));
#36985=CARTESIAN_POINT('Ctrl Pts',(-5.07577939190903,19.9832027490848,0.353603093965685));
#36986=CARTESIAN_POINT('Ctrl Pts',(-4.78282515660807,19.9789919207889,0.474026380935749));
#36987=CARTESIAN_POINT('Ctrl Pts',(-4.45930905769162,19.9747249819138,0.598869507096236));
#36988=CARTESIAN_POINT('Ctrl Pts',(-4.10061553943856,19.9704191073005,0.727257554679413));
#36989=CARTESIAN_POINT('Ctrl Pts',(-3.70134298961707,19.9661195200363,0.857723092138966));
#36990=CARTESIAN_POINT('Ctrl Pts',(-3.25666212542464,19.9619190254675,0.987529865804192));
#36991=CARTESIAN_POINT('Ctrl Pts',(-2.76257283838323,19.9579585252344,1.11255112813169));
#36992=CARTESIAN_POINT('Ctrl Pts',(-2.21448293057545,19.9544123316413,1.22757275325379));
#36993=CARTESIAN_POINT('Ctrl Pts',(-1.60537183762896,19.9514853648295,1.3262010465794));
#36994=CARTESIAN_POINT('Ctrl Pts',(-0.938804294807327,19.9494592496166,
1.39847259929471));
#36995=CARTESIAN_POINT('Ctrl Pts',(-0.236508776779611,19.9485851832705,
1.43363032242854));
#36996=CARTESIAN_POINT('Ctrl Pts',(0.464364601123389,19.948749328727,1.4264261030562));
#36997=CARTESIAN_POINT('Ctrl Pts',(1.12896559565999,19.9499401821903,1.38089160685135));
#36998=CARTESIAN_POINT('Ctrl Pts',(1.73422006980435,19.9520479706928,1.30699167215705));
#36999=CARTESIAN_POINT('Ctrl Pts',(2.27384587626356,19.9547877813634,1.21535231751198));
#37000=CARTESIAN_POINT('Ctrl Pts',(2.75210517028745,19.9579163355911,1.11403613854411));
#37001=CARTESIAN_POINT('Ctrl Pts',(3.17956446864321,19.9612849529054,1.00748451984042));
#37002=CARTESIAN_POINT('Ctrl Pts',(3.56234892004249,19.9647715292712,0.8992365099518));
#37003=CARTESIAN_POINT('Ctrl Pts',(3.90388903433588,19.9682667685621,0.792414560653075));
#37004=CARTESIAN_POINT('Ctrl Pts',(4.20698277151624,19.9716805654084,0.689557632968514));
#37005=CARTESIAN_POINT('Ctrl Pts',(4.47552350917186,19.9749594106943,0.592122104802372));
#37006=CARTESIAN_POINT('Ctrl Pts',(4.7143736486654,19.9780870462951,0.500500697884532));
#37007=CARTESIAN_POINT('Ctrl Pts',(4.92834373472852,19.9810702092344,0.414472289313536));
#37008=CARTESIAN_POINT('Ctrl Pts',(5.12117579191345,19.9839201644114,0.333751104062619));
#37009=CARTESIAN_POINT('Ctrl Pts',(5.29544459285731,19.9866447487504,0.258203140894221));
#37010=CARTESIAN_POINT('Ctrl Pts',(5.45302136069377,19.989249786509,0.187774421799672));
#37011=CARTESIAN_POINT('Ctrl Pts',(5.58355472894304,19.9915339342793,0.127841695660172));
#37012=CARTESIAN_POINT('Ctrl Pts',(5.66171727448302,19.9929727783557,0.0911904475355778));
#37013=CARTESIAN_POINT('Ctrl Pts',(5.69263920831736,19.9935543971865,0.0765659156944554));
#37014=CARTESIAN_POINT('Ctrl Pts',(-5.75649916782382,19.9991143710642,0.213746605759207));
#37015=CARTESIAN_POINT('Ctrl Pts',(-5.72140302733699,19.9983747379508,0.230339439268123));
#37016=CARTESIAN_POINT('Ctrl Pts',(-5.60614021201479,19.9959920716916,0.284332231538033));
#37017=CARTESIAN_POINT('Ctrl Pts',(-5.40164894966011,19.9920036394875,0.377223723225483));
#37018=CARTESIAN_POINT('Ctrl Pts',(-5.13368112668697,19.9871027056259,0.493463372834317));
#37019=CARTESIAN_POINT('Ctrl Pts',(-4.83783506997635,19.982026814529,0.615073150075648));
#37020=CARTESIAN_POINT('Ctrl Pts',(-4.51104954848351,19.976794518307,0.74116897376691));
#37021=CARTESIAN_POINT('Ctrl Pts',(-4.14863414602773,19.9714329010045,0.870871691441195));
#37022=CARTESIAN_POINT('Ctrl Pts',(-3.74509982337592,19.965998699662,1.00270211695211));
#37023=CARTESIAN_POINT('Ctrl Pts',(-3.29553136101948,19.9606049310289,1.13389675931631));
#37024=CARTESIAN_POINT('Ctrl Pts',(-2.79585032994363,19.9554249629654,1.26028299192613));
#37025=CARTESIAN_POINT('Ctrl Pts',(-2.24138300365344,19.9506788186159,1.37658388105494));
#37026=CARTESIAN_POINT('Ctrl Pts',(-1.62500802081888,19.9466357126787,1.47632451499044));
#37027=CARTESIAN_POINT('Ctrl Pts',(-0.950336100057744,19.9437046353406,
1.54941651962382));
#37028=CARTESIAN_POINT('Ctrl Pts',(-0.239411452580767,19.9423138347391,
1.58496955781237));
#37029=CARTESIAN_POINT('Ctrl Pts',(0.470068367955475,19.9425938101752,1.57768516782441));
#37030=CARTESIAN_POINT('Ctrl Pts',(1.14282032186782,19.9444142574433,1.53163591167869));
#37031=CARTESIAN_POINT('Ctrl Pts',(1.75540154182604,19.9474213041126,1.45689782413783));
#37032=CARTESIAN_POINT('Ctrl Pts',(2.30143868160016,19.9511828297409,1.3642271613645));
#37033=CARTESIAN_POINT('Ctrl Pts',(2.78525552181212,19.9553643975143,1.26178540691853));
#37034=CARTESIAN_POINT('Ctrl Pts',(3.21756459443667,19.9597777818374,1.1540687684985));
#37035=CARTESIAN_POINT('Ctrl Pts',(3.60458630024707,19.9642729470882,1.04465768021273));
#37036=CARTESIAN_POINT('Ctrl Pts',(3.94981603924592,19.9687180881684,0.936708354815534));
#37037=CARTESIAN_POINT('Ctrl Pts',(4.2561086909295,19.973006668013,0.832784704953047));
#37038=CARTESIAN_POINT('Ctrl Pts',(4.52742310268015,19.9770781627105,0.734355145957688));
#37039=CARTESIAN_POINT('Ctrl Pts',(4.76869242285065,19.9809173370862,0.641812973636067));
#37040=CARTESIAN_POINT('Ctrl Pts',(4.98479244425756,19.9845356429339,0.554931532203396));
#37041=CARTESIAN_POINT('Ctrl Pts',(5.17951571609395,19.9879485183431,0.473419145840954));
#37042=CARTESIAN_POINT('Ctrl Pts',(5.35547336786553,19.9911666293176,0.397137560135068));
#37043=CARTESIAN_POINT('Ctrl Pts',(5.5145642915736,19.9941992385701,0.326029401375756));
#37044=CARTESIAN_POINT('Ctrl Pts',(5.64634618113553,19.9968207967888,0.265520382202669));
#37045=CARTESIAN_POINT('Ctrl Pts',(5.7252551879899,19.9984564343695,0.228516946253832));
#37046=CARTESIAN_POINT('Ctrl Pts',(5.75647210573555,19.9991166589352,0.213751969958807));
#37047=CARTESIAN_POINT('Ctrl Pts',(-5.8136196818812,19.9261275467547,0.33332821073875));
#37048=CARTESIAN_POINT('Ctrl Pts',(-5.77819705107185,19.9253120907747,0.350030686003675));
#37049=CARTESIAN_POINT('Ctrl Pts',(-5.66186629696485,19.9226772399395,0.404374549031671));
#37050=CARTESIAN_POINT('Ctrl Pts',(-5.45549726798606,19.9182211259577,0.497839527211375));
#37051=CARTESIAN_POINT('Ctrl Pts',(-5.18506580575754,19.9126623370125,0.614749759844558));
#37052=CARTESIAN_POINT('Ctrl Pts',(-4.88647423531625,19.9068337910618,0.737027952359146));
#37053=CARTESIAN_POINT('Ctrl Pts',(-4.55661570515206,19.9007648007416,0.863793230857175));
#37054=CARTESIAN_POINT('Ctrl Pts',(-4.19074002651519,19.8944919190027,0.994166830412173));
#37055=CARTESIAN_POINT('Ctrl Pts',(-3.78329010948032,19.8880827064613,1.1266635068718));
#37056=CARTESIAN_POINT('Ctrl Pts',(-3.32928741344157,19.8816683464093,1.25850416200931));
#37057=CARTESIAN_POINT('Ctrl Pts',(-2.82459972123038,19.8754505103237,1.38549071493382));
#37058=CARTESIAN_POINT('Ctrl Pts',(-2.26449815900478,19.8696881919514,1.50231378248865));
#37059=CARTESIAN_POINT('Ctrl Pts',(-1.64179011342992,19.8647044795955,1.60246108002828));
#37060=CARTESIAN_POINT('Ctrl Pts',(-0.960140287927844,19.8610141389188,
1.67580351036708));
#37061=CARTESIAN_POINT('Ctrl Pts',(-0.241865765896076,19.8591912733021,
1.71143169382191));
#37062=CARTESIAN_POINT('Ctrl Pts',(0.474899624177775,19.8595680072199,1.7041381423012));
#37063=CARTESIAN_POINT('Ctrl Pts',(1.15461838959442,19.861915384356,1.65796695719522));
#37064=CARTESIAN_POINT('Ctrl Pts',(1.77352632078311,19.8656777419918,1.58295803460786));
#37065=CARTESIAN_POINT('Ctrl Pts',(2.32516508950545,19.8703010047203,1.48990196940852));
#37066=CARTESIAN_POINT('Ctrl Pts',(2.8138948184701,19.8753745609343,1.38699877184857));
#37067=CARTESIAN_POINT('Ctrl Pts',(3.25054101930003,19.880676768205,1.27877256646152));
#37068=CARTESIAN_POINT('Ctrl Pts',(3.64139477654928,19.8860335761906,1.16882675566282));
#37069=CARTESIAN_POINT('Ctrl Pts',(3.98999701978794,19.8912934545324,1.06033726777782));
#37070=CARTESIAN_POINT('Ctrl Pts',(4.29924266842479,19.8963351143492,0.955883447536127));
#37071=CARTESIAN_POINT('Ctrl Pts',(4.57314066596504,19.9010912851556,0.85694242225947));
#37072=CARTESIAN_POINT('Ctrl Pts',(4.81668173987254,19.9055469579917,0.763909702030878));
#37073=CARTESIAN_POINT('Ctrl Pts',(5.03479661632215,19.9097171082138,0.676556823383301));
#37074=CARTESIAN_POINT('Ctrl Pts',(5.23132099559656,19.913620337409,0.594589356922334));
#37075=CARTESIAN_POINT('Ctrl Pts',(5.40889737389929,19.9172693946253,0.517866823966847));
#37076=CARTESIAN_POINT('Ctrl Pts',(5.56944911393839,19.9206762302772,0.446330460231254));
#37077=CARTESIAN_POINT('Ctrl Pts',(5.70244460071722,19.9235937945899,0.385440459384885));
#37078=CARTESIAN_POINT('Ctrl Pts',(5.78208503334231,19.925402421831,0.348196348162051));
#37079=CARTESIAN_POINT('Ctrl Pts',(5.81359216867338,19.9261317941967,0.333334948402759));
#37080=CARTESIAN_POINT('Ctrl Pts',(-5.847868485275,19.7956126342212,0.401492685916237));
#37081=CARTESIAN_POINT('Ctrl Pts',(-5.8122174502919,19.7947531586782,0.418225605367972));
#37082=CARTESIAN_POINT('Ctrl Pts',(-5.69514385494066,19.7919721680002,0.472658902359452));
#37083=CARTESIAN_POINT('Ctrl Pts',(-5.4874901169821,19.7872465641152,0.566224573560217));
#37084=CARTESIAN_POINT('Ctrl Pts',(-5.21539943498523,19.7813114381313,0.683170401131284));
#37085=CARTESIAN_POINT('Ctrl Pts',(-4.91498607991476,19.7750554590008,0.805411723710539));
#37086=CARTESIAN_POINT('Ctrl Pts',(-4.58312097074267,19.7685149979094,0.932075987565472));
#37087=CARTESIAN_POINT('Ctrl Pts',(-4.21502610849436,19.761732954918,1.06228930799929));
#37088=CARTESIAN_POINT('Ctrl Pts',(-3.80511493092991,19.7547839595059,1.19456777190076));
#37089=CARTESIAN_POINT('Ctrl Pts',(-3.34838603989262,19.7478101772206,1.32613267716697));
#37090=CARTESIAN_POINT('Ctrl Pts',(-2.84069310068318,19.7410294174041,1.45278803968532));
#37091=CARTESIAN_POINT('Ctrl Pts',(-2.27729398886718,19.7347218891001,1.56923145151833));
#37092=CARTESIAN_POINT('Ctrl Pts',(-1.65097444995275,19.7292389106163,1.66896750324683));
#37093=CARTESIAN_POINT('Ctrl Pts',(-0.965445840826782,19.7251495498199,
1.74192179778576));
#37094=CARTESIAN_POINT('Ctrl Pts',(-0.243178106912335,19.7231013691965,
1.77728502764766));
#37095=CARTESIAN_POINT('Ctrl Pts',(0.477492972686614,19.7235284512799,1.77005561694156));
#37096=CARTESIAN_POINT('Ctrl Pts',(1.1610251436121,19.7261512068074,1.72418821081852));
#37097=CARTESIAN_POINT('Ctrl Pts',(1.78347110445064,19.7303114963596,1.64955010159841));
#37098=CARTESIAN_POINT('Ctrl Pts',(2.33831781824055,19.7353929949862,1.55686100196852));
#37099=CARTESIAN_POINT('Ctrl Pts',(2.82992627546618,19.7409454228058,1.45428842720372));
#37100=CARTESIAN_POINT('Ctrl Pts',(3.26917005572502,19.7467292925962,1.3463497158952));
#37101=CARTESIAN_POINT('Ctrl Pts',(3.66236643296839,19.752557244967,1.23664639117856));
#37102=CARTESIAN_POINT('Ctrl Pts',(4.01306968582882,19.7582663860018,1.1283545242984));
#37103=CARTESIAN_POINT('Ctrl Pts',(4.32418661922986,19.7637265282549,1.02405503991256));
#37104=CARTESIAN_POINT('Ctrl Pts',(4.59974676808851,19.7688658335805,0.925227997173997));
#37105=CARTESIAN_POINT('Ctrl Pts',(4.84476901005903,19.7736686618163,0.832272126158535));
#37106=CARTESIAN_POINT('Ctrl Pts',(5.06421316650717,19.7781513272396,0.744961377308228));
#37107=CARTESIAN_POINT('Ctrl Pts',(5.26193851821112,19.7823336930188,0.663002481750077));
#37108=CARTESIAN_POINT('Ctrl Pts',(5.44060507025142,19.7862292581127,0.586255387133592));
#37109=CARTESIAN_POINT('Ctrl Pts',(5.60215053682224,19.7898511514179,0.51466232923396));
#37110=CARTESIAN_POINT('Ctrl Pts',(5.73598092682063,19.7929396095604,0.453693790309014));
#37111=CARTESIAN_POINT('Ctrl Pts',(5.81613053652334,19.794848500999,0.416388245022623));
#37112=CARTESIAN_POINT('Ctrl Pts',(5.84784089926276,19.7956180079236,0.401501580201476));
#37113=CARTESIAN_POINT('',(-5.593361696257,19.9918770425327,0.136828655009776));
#37114=CARTESIAN_POINT('Ctrl Pts',(-5.593361696257,19.9918770425327,0.136828655009776));
#37115=CARTESIAN_POINT('Ctrl Pts',(-5.53989250493793,19.9909063803029,0.161641904267682));
#37116=CARTESIAN_POINT('Ctrl Pts',(-5.47940098468457,19.9898415697195,0.189256606818882));
#37117=CARTESIAN_POINT('Ctrl Pts',(-5.37813021090341,19.9881276870329,0.234751190678744));
#37118=CARTESIAN_POINT('Ctrl Pts',(-5.34261770407618,19.9875368930449,0.250586413051278));
#37119=CARTESIAN_POINT('Ctrl Pts',(-5.28671557048504,19.9866244477965,0.275255229834141));
#37120=CARTESIAN_POINT('Ctrl Pts',(-5.25810616035191,19.9861616644341,0.287817888230927));
#37121=CARTESIAN_POINT('Ctrl Pts',(-5.22850923521242,19.985689657541,0.300699531939207));
#37122=CARTESIAN_POINT('Ctrl Pts',(-5.20855850400689,19.9853730116806,0.309355137583069));
#37123=CARTESIAN_POINT('Ctrl Pts',(-5.19652326398584,19.9851830455075,0.314557421644312));
#37124=CARTESIAN_POINT('Ctrl Pts',(-5.12232129830657,19.984016616942,0.346539419230699));
#37125=CARTESIAN_POINT('Ctrl Pts',(-5.04967091219916,19.9829067581425,0.37727618564664));
#37126=CARTESIAN_POINT('Ctrl Pts',(-4.93065570811597,19.9811527268843,0.426450734116511));
#37127=CARTESIAN_POINT('Ctrl Pts',(-4.88931070260123,19.9805531897341,0.443349812440991));
#37128=CARTESIAN_POINT('Ctrl Pts',(-4.8247832880986,19.9796344794417,0.469375730136451));
#37129=CARTESIAN_POINT('Ctrl Pts',(-4.79189210428965,19.9791702786294,0.482557659797516));
#37130=CARTESIAN_POINT('Ctrl Pts',(-4.7524209725367,19.9786209356004,0.498210233032642));
#37131=CARTESIAN_POINT('Ctrl Pts',(-4.73526946950489,19.9783839180811,0.504974530200582));
#37132=CARTESIAN_POINT('Ctrl Pts',(-4.72378284443722,19.9782255634798,0.50949622404512));
#37133=CARTESIAN_POINT('Ctrl Pts',(-4.71687145440915,19.9781305474126,0.512210984265389));
#37134=CARTESIAN_POINT('Ctrl Pts',(-4.56330035730193,19.9760235555773,0.572436934549734));
#37135=CARTESIAN_POINT('Ctrl Pts',(-4.38742083373183,19.9737389649771,0.638489520363415));
#37136=CARTESIAN_POINT('Ctrl Pts',(-4.08315840426839,19.9701290451024,0.744581222725977));
#37137=CARTESIAN_POINT('Ctrl Pts',(-3.9749970704292,19.9688956929681,0.781076603721506));
#37138=CARTESIAN_POINT('Ctrl Pts',(-3.80264428364334,19.9670302858359,0.836644690767833));
#37139=CARTESIAN_POINT('Ctrl Pts',(-3.71394019374364,19.9660938405529,0.864631898693615));
#37140=CARTESIAN_POINT('Ctrl Pts',(-3.60602861997382,19.9650025232388,0.897417528954085));
#37141=CARTESIAN_POINT('Ctrl Pts',(-3.5509669658672,19.9644582409819,0.913813976195473));
#37142=CARTESIAN_POINT('Ctrl Pts',(-3.52713214255971,19.9642253903256,0.9208385631156));
#37143=CARTESIAN_POINT('Ctrl Pts',(-3.51118960001082,19.9640702618073,0.925520708479307));
#37144=CARTESIAN_POINT('Ctrl Pts',(-3.50199535538248,19.9639811993776,0.928210295796779));
#37145=CARTESIAN_POINT('Ctrl Pts',(-3.27669483698199,19.9618064517119,0.993913481638213));
#37146=CARTESIAN_POINT('Ctrl Pts',(-3.03027743164036,19.9596513714663,1.05988700948767));
#37147=CARTESIAN_POINT('Ctrl Pts',(-2.61873506056166,19.956611727738,1.15466812421503));
#37148=CARTESIAN_POINT('Ctrl Pts',(-2.47456822635772,19.9556313892423,1.18554057428783));
#37149=CARTESIAN_POINT('Ctrl Pts',(-2.24783890928523,19.954248203717,1.22962014666199));
#37150=CARTESIAN_POINT('Ctrl Pts',(-2.17051595929998,19.9538017251389,1.24394054524097));
#37151=CARTESIAN_POINT('Ctrl Pts',(-2.01237703740728,19.9529444659006,1.27163039886662));
#37152=CARTESIAN_POINT('Ctrl Pts',(-1.93359205710365,19.9525432774048,1.2846852665418));
#37153=CARTESIAN_POINT('Ctrl Pts',(-1.51062468474186,19.9505469283039,1.3501935639087));
#37154=CARTESIAN_POINT('Ctrl Pts',(-1.1559767801875,19.9493606967916,1.39097553980188));
#37155=CARTESIAN_POINT('Ctrl Pts',(-0.599593913358566,19.9483503734994,
1.42761012316683));
#37156=CARTESIAN_POINT('Ctrl Pts',(-0.410064456082688,19.9481405087443,
1.43573575542328));
#37157=CARTESIAN_POINT('Ctrl Pts',(-0.119667517669528,19.9480101389945,
1.44096891640077));
#37158=CARTESIAN_POINT('Ctrl Pts',(-0.0218514127819169,19.9479967936825,
1.44155464996756));
#37159=CARTESIAN_POINT('Ctrl Pts',(0.126398432674336,19.9480202849448,1.44059804455932));
#37160=CARTESIAN_POINT('Ctrl Pts',(0.200904777433672,19.9480432708496,1.43966102024194));
#37161=CARTESIAN_POINT('Ctrl Pts',(0.275983255239822,19.9480843551756,1.43801840811879));
#37162=CARTESIAN_POINT('Ctrl Pts',(0.326162714454324,19.9481158958946,1.43676464195432));
#37163=CARTESIAN_POINT('Ctrl Pts',(0.353068789789541,19.948135131383,1.43600374167174));
#37164=CARTESIAN_POINT('Ctrl Pts',(0.751958403002702,19.9484512736903,1.42356233146255));
#37165=CARTESIAN_POINT('Ctrl Pts',(1.10849134902751,19.9492390334456,1.39470318783279));
#37166=CARTESIAN_POINT('Ctrl Pts',(1.61495190962454,19.9510613632109,1.33320111122525));
#37167=CARTESIAN_POINT('Ctrl Pts',(1.861097475313,19.9521283565705,1.29790236789663));
#37168=CARTESIAN_POINT('Ctrl Pts',(2.13586905138197,19.9535982703747,1.25041701195131));
#37169=CARTESIAN_POINT('Ctrl Pts',(2.2509715302899,19.954270867413,1.22889001763999));
#37170=CARTESIAN_POINT('Ctrl Pts',(2.32711612334435,19.9547281407377,1.2142965170218));
#37171=CARTESIAN_POINT('Ctrl Pts',(2.36665276250411,19.9549723509007,1.20652523542265));
#37172=CARTESIAN_POINT('Ctrl Pts',(2.68815404361998,19.9570070374924,1.14194197153519));
#37173=CARTESIAN_POINT('Ctrl Pts',(2.94945525817411,19.9590254177359,1.07926628440836));
#37174=CARTESIAN_POINT('Ctrl Pts',(3.30469052701535,19.9621143428657,0.984758426877155));
#37175=CARTESIAN_POINT('Ctrl Pts',(3.41698285779743,19.9631547324302,0.953157125885748));
#37176=CARTESIAN_POINT('Ctrl Pts',(3.57624221572307,19.9647049245996,0.906369256589431));
#37177=CARTESIAN_POINT('Ctrl Pts',(3.65357711012402,19.9654774786032,0.883126997595109));
#37178=CARTESIAN_POINT('Ctrl Pts',(3.73978528060851,19.9663691056251,0.856422973430396));
#37179=CARTESIAN_POINT('Ctrl Pts',(3.77587109517688,19.9667486282055,0.845081023173003));
#37180=CARTESIAN_POINT('Ctrl Pts',(3.7997370728423,19.9670010068933,0.837544087199959));
#37181=CARTESIAN_POINT('Ctrl Pts',(3.80983216252252,19.967108252225,0.834343254624691));
#37182=CARTESIAN_POINT('Ctrl Pts',(4.03906084107691,19.9695588041822,0.761263843168769));
#37183=CARTESIAN_POINT('Ctrl Pts',(4.23305855301844,19.9718597199617,0.69347956345791));
#37184=CARTESIAN_POINT('Ctrl Pts',(4.49143473088391,19.975118797674,0.598683154613398));
#37185=CARTESIAN_POINT('Ctrl Pts',(4.57212339183127,19.976174096764,0.568208397480002));
#37186=CARTESIAN_POINT('Ctrl Pts',(4.68500128574059,19.9776937772282,0.524633828361888));
#37187=CARTESIAN_POINT('Ctrl Pts',(4.73940145831732,19.9784378450774,0.503378483467561));
#37188=CARTESIAN_POINT('Ctrl Pts',(4.79930047116214,19.9792750322337,0.479583707595788));
#37189=CARTESIAN_POINT('Ctrl Pts',(4.82420693627534,19.9796268695674,0.469606904472261));
#37190=CARTESIAN_POINT('Ctrl Pts',(4.84064134848598,19.979859844406,0.463005422732545));
#37191=CARTESIAN_POINT('Ctrl Pts',(4.84712299735739,19.9799519755852,0.460396313650406));
#37192=CARTESIAN_POINT('Ctrl Pts',(4.93440424623526,19.9811980255666,0.425138847862602));
#37193=CARTESIAN_POINT('Ctrl Pts',(5.00681738689788,19.9822679591127,0.395120032136794));
#37194=CARTESIAN_POINT('Ctrl Pts',(5.10768181038188,19.9837998500125,0.352584597767958));
#37195=CARTESIAN_POINT('Ctrl Pts',(5.15617520024639,19.984547618408,0.33193633916448));
#37196=CARTESIAN_POINT('Ctrl Pts',(5.20935788346942,19.9853851093829,0.309001644883203));
#37197=CARTESIAN_POINT('Ctrl Pts',(5.23142340378951,19.9857362363002,0.299424863669381));
#37198=CARTESIAN_POINT('Ctrl Pts',(5.24597218217979,19.9859685524309,0.293096892180794));
#37199=CARTESIAN_POINT('Ctrl Pts',(5.25210470606373,19.9860667644056,0.290424720766036));
#37200=CARTESIAN_POINT('Ctrl Pts',(5.39106103618176,19.9883011364273,0.229721734798504));
#37201=CARTESIAN_POINT('Ctrl Pts',(5.50208873233516,19.9902201029699,0.179185362360739));
#37202=CARTESIAN_POINT('Ctrl Pts',(5.593361696298,19.9918770423734,0.136828655185692));
#37203=CARTESIAN_POINT('',(-5.73644346265602,19.8089511587379,0.442548130347095));
#37204=CARTESIAN_POINT('Origin',(-5.599999999997,19.5919343769627,0.135488060674723));
#37205=CARTESIAN_POINT('Ctrl Pts',(-5.73644387762282,19.8089519016962,0.442549068003705));
#37206=CARTESIAN_POINT('Ctrl Pts',(-5.73644352459338,19.8089518943027,0.442549230097738));
#37207=CARTESIAN_POINT('Ctrl Pts',(-5.73644317156369,19.8089518869092,0.442549392191867));
#37208=CARTESIAN_POINT('Ctrl Pts',(-5.73644281853377,19.8089518795157,0.442549554286092));
#37209=CARTESIAN_POINT('Ctrl Pts',(-5.67992286962499,19.8077681857041,0.468500774395627));
#37210=CARTESIAN_POINT('Ctrl Pts',(-5.61717023492195,19.8064997493133,0.496914686516317));
#37211=CARTESIAN_POINT('Ctrl Pts',(-5.54808233593107,19.8051527504546,0.52755683616938));
#37212=CARTESIAN_POINT('Ctrl Pts',(-5.52952171320869,19.8047908761178,0.535788920042535));
#37213=CARTESIAN_POINT('Ctrl Pts',(-5.51050375561706,19.80442329013,0.54418155326481));
#37214=CARTESIAN_POINT('Ctrl Pts',(-5.49102627418781,19.8040500071028,0.552729586232965));
#37215=CARTESIAN_POINT('Ctrl Pts',(-5.42196512499331,19.8027264604764,0.583038277953587));
#37216=CARTESIAN_POINT('Ctrl Pts',(-5.34712803363965,19.8013311509866,0.615304462994705));
#37217=CARTESIAN_POINT('Ctrl Pts',(-5.26640545181662,19.7998746698034,0.649262108181634));
#37218=CARTESIAN_POINT('Ctrl Pts',(-5.25085819544196,19.7995941499557,0.655802387291616));
#37219=CARTESIAN_POINT('Ctrl Pts',(-5.23509257167142,19.7993113637113,0.662405262900947));
#37220=CARTESIAN_POINT('Ctrl Pts',(-5.21910773525063,19.799026390464,0.669068618256093));
#37221=CARTESIAN_POINT('Ctrl Pts',(-5.19133151721783,19.7985312037231,0.680647267314643));
#37222=CARTESIAN_POINT('Ctrl Pts',(-5.16289340246033,19.7980294106306,0.692408572678255));
#37223=CARTESIAN_POINT('Ctrl Pts',(-5.13378891178081,19.7975215466356,0.704340798761004));
#37224=CARTESIAN_POINT('Ctrl Pts',(-5.06602882589204,19.7963391549454,0.732121001930149));
#37225=CARTESIAN_POINT('Ctrl Pts',(-4.99465703432228,19.7951237786661,0.760829138131545));
#37226=CARTESIAN_POINT('Ctrl Pts',(-4.91961387572591,19.7938829721629,0.790301960627574));
#37227=CARTESIAN_POINT('Ctrl Pts',(-4.82892309834609,19.7923834389814,0.825920306573258));
#37228=CARTESIAN_POINT('Ctrl Pts',(-4.73287029248815,19.7908466413634,0.86265704234701));
#37229=CARTESIAN_POINT('Ctrl Pts',(-4.63134530184612,19.7892891516912,0.900178764352119));
#37230=CARTESIAN_POINT('Ctrl Pts',(-4.61739621649649,19.7890751594886,0.905334083248527));
#37231=CARTESIAN_POINT('Ctrl Pts',(-4.60334382008669,19.7888607816979,0.910504140875635));
#37232=CARTESIAN_POINT('Ctrl Pts',(-4.58918781805959,19.7886460662023,0.915687994968418));
#37233=CARTESIAN_POINT('Ctrl Pts',(-4.55700503480212,19.7881579239823,0.927473162305002));
#37234=CARTESIAN_POINT('Ctrl Pts',(-4.52428676573379,19.7876680341698,0.939329672314043));
#37235=CARTESIAN_POINT('Ctrl Pts',(-4.49102962640135,19.7871769736762,0.951246087558308));
#37236=CARTESIAN_POINT('Ctrl Pts',(-4.45062022386591,19.7865803059666,0.965725240908554));
#37237=CARTESIAN_POINT('Ctrl Pts',(-4.40941525025059,19.785981907784,0.980292870178383));
#37238=CARTESIAN_POINT('Ctrl Pts',(-4.36740858669668,19.7853828849297,0.994927388978708));
#37239=CARTESIAN_POINT('Ctrl Pts',(-4.34640525491973,19.7850833735025,1.00224464837887));
#37240=CARTESIAN_POINT('Ctrl Pts',(-4.3252014967549,19.7847836982241,1.00957861859033));
#37241=CARTESIAN_POINT('Ctrl Pts',(-4.30379654745358,19.784484014967,1.01692648002813));
#37242=CARTESIAN_POINT('Ctrl Pts',(-4.29309407280291,19.7843341733384,1.02060041074704));
#37243=CARTESIAN_POINT('Ctrl Pts',(-4.28234130011502,19.7841843292229,1.02427781353311));
#37244=CARTESIAN_POINT('Ctrl Pts',(-4.27153813309606,19.7840345010304,1.02795832991866));
#37245=CARTESIAN_POINT('Ctrl Pts',(-4.26343575783185,19.783922129886,1.03071871720782));
#37246=CARTESIAN_POINT('Ctrl Pts',(-4.25530503573597,19.7838097676575,1.03348085583515));
#37247=CARTESIAN_POINT('Ctrl Pts',(-4.24714592611223,19.783697422145,1.03624459284066));
#37248=CARTESIAN_POINT('Ctrl Pts',(-4.24442622290431,19.7836599736408,1.03716583850916));
#37249=CARTESIAN_POINT('Ctrl Pts',(-4.24040661893564,19.7836047149147,1.0385256585289));
#37250=CARTESIAN_POINT('Ctrl Pts',(-4.23897735248378,19.7835850825318,1.03900885687057));
#37251=CARTESIAN_POINT('Ctrl Pts',(-4.23364029621417,19.7835117728056,1.04081317875577));
#37252=CARTESIAN_POINT('Ctrl Pts',(-4.22827896813906,19.7834382575236,1.04262230666689));
#37253=CARTESIAN_POINT('Ctrl Pts',(-4.22289334196019,19.7833645409097,1.04443615539268));
#37254=CARTESIAN_POINT('Ctrl Pts',(-4.1421104893463,19.7822588127816,1.07164336759298));
#37255=CARTESIAN_POINT('Ctrl Pts',(-4.05586117002453,19.7811075541515,1.09991688725499));
#37256=CARTESIAN_POINT('Ctrl Pts',(-3.96405547488631,19.7799263402454,1.12894309340335));
#37257=CARTESIAN_POINT('Ctrl Pts',(-3.91582473643939,19.7793057815875,1.14419220572412));
#37258=CARTESIAN_POINT('Ctrl Pts',(-3.86606035830127,19.7786770017245,1.15964822680068));
#37259=CARTESIAN_POINT('Ctrl Pts',(-3.81474889150123,19.7780425864392,1.17525989420485));
#37260=CARTESIAN_POINT('Ctrl Pts',(-3.71991638549903,19.7768700767626,1.20411296809142));
#37261=CARTESIAN_POINT('Ctrl Pts',(-3.61979927953566,19.7756781491646,1.23350071191893));
#37262=CARTESIAN_POINT('Ctrl Pts',(-3.51431514211601,19.7744850775374,1.26306249208537));
#37263=CARTESIAN_POINT('Ctrl Pts',(-3.46378927585294,19.7739136079407,1.27722229457061));
#37264=CARTESIAN_POINT('Ctrl Pts',(-3.41203205809547,19.7733419177578,1.29142128195551));
#37265=CARTESIAN_POINT('Ctrl Pts',(-3.35903461288398,19.7727722569973,1.30561555713677));
#37266=CARTESIAN_POINT('Ctrl Pts',(-3.24836436657796,19.7715826808503,1.33525630536862));
#37267=CARTESIAN_POINT('Ctrl Pts',(-3.13228530905258,19.7704017483376,1.3648801206481));
#37268=CARTESIAN_POINT('Ctrl Pts',(-3.01072581908244,19.7692520506645,1.39404921923668));
#37269=CARTESIAN_POINT('Ctrl Pts',(-2.9685701696663,19.768853346688,1.40416477906823));
#37270=CARTESIAN_POINT('Ctrl Pts',(-2.92501774452437,19.7684516393367,1.41439775540621));
#37271=CARTESIAN_POINT('Ctrl Pts',(-2.88136966635236,19.7680601552779,1.42441930906165));
#37272=CARTESIAN_POINT('Ctrl Pts',(-2.8718037250264,19.7679743573758,1.42661563930751));
#37273=CARTESIAN_POINT('Ctrl Pts',(-2.86223323801364,19.76788904089,1.42880200705198));
#37274=CARTESIAN_POINT('Ctrl Pts',(-2.85267198306032,19.7678043285989,1.43097527914219));
#37275=CARTESIAN_POINT('Ctrl Pts',(-2.83185440261412,19.7676198857676,1.43570711265048));
#37276=CARTESIAN_POINT('Ctrl Pts',(-2.81108054715055,19.7674383160755,1.44037668862943));
#37277=CARTESIAN_POINT('Ctrl Pts',(-2.79049311401335,19.7672607865354,1.44495366167414));
#37278=CARTESIAN_POINT('Ctrl Pts',(-2.6196797742614,19.7657878290548,1.48292867519389));
#37279=CARTESIAN_POINT('Ctrl Pts',(-2.45352912167896,19.7645067104381,1.51637189968607));
#37280=CARTESIAN_POINT('Ctrl Pts',(-2.29228332637382,19.7633930739181,1.54580449579569));
#37281=CARTESIAN_POINT('Ctrl Pts',(-2.12993500746006,19.7622718228706,1.57543833828207));
#37282=CARTESIAN_POINT('Ctrl Pts',(-1.97255885581796,19.761320314212,1.60100751447628));
#37283=CARTESIAN_POINT('Ctrl Pts',(-1.82036290435247,19.7605129043991,1.62305465711288));
#37284=CARTESIAN_POINT('Ctrl Pts',(-1.76978200408601,19.7602445693034,1.63038181865774));
#37285=CARTESIAN_POINT('Ctrl Pts',(-1.71977283800279,19.7599921471886,1.63731986544404));
#37286=CARTESIAN_POINT('Ctrl Pts',(-1.6703418370121,19.7597546916422,1.64388836755662));
#37287=CARTESIAN_POINT('Ctrl Pts',(-1.52110170714283,19.7590377752158,1.66371973023757));
#37288=CARTESIAN_POINT('Ctrl Pts',(-1.3771352506761,19.7584572456274,1.68018464462649));
#37289=CARTESIAN_POINT('Ctrl Pts',(-1.23859807970654,19.7579867069053,1.69382332829766));
#37290=CARTESIAN_POINT('Ctrl Pts',(-1.14893751809387,19.7576821766064,1.7026502159052));
#37291=CARTESIAN_POINT('Ctrl Pts',(-1.06155007351066,19.7574237245106,1.71029278196188));
#37292=CARTESIAN_POINT('Ctrl Pts',(-0.976468268211634,19.7572043404281,
1.71689112254408));
#37293=CARTESIAN_POINT('Ctrl Pts',(-0.844577106193146,19.7568642580631,
1.7271196644012));
#37294=CARTESIAN_POINT('Ctrl Pts',(-0.71822817214218,19.7566180411509,1.73484113748309));
#37295=CARTESIAN_POINT('Ctrl Pts',(-0.597515581883815,19.75644118749,1.74056201975772));
#37296=CARTESIAN_POINT('Ctrl Pts',(-0.480867236251215,19.7562702882746,
1.74609028695394));
#37297=CARTESIAN_POINT('Ctrl Pts',(-0.369481483391001,19.7561641382709,
1.74975029480863));
#37298=CARTESIAN_POINT('Ctrl Pts',(-0.263414069157,19.756101348382,1.75196323556012));
#37299=CARTESIAN_POINT('Ctrl Pts',(-0.25575142503431,19.7560968122427,1.7521231053709));
#37300=CARTESIAN_POINT('Ctrl Pts',(-0.248116526890297,19.756092502804,1.75227540725386));
#37301=CARTESIAN_POINT('Ctrl Pts',(-0.240509390808347,19.7560884122148,
1.75242029269565));
#37302=CARTESIAN_POINT('Ctrl Pts',(-0.202051679845121,19.7560677323299,
1.75315275789451));
#37303=CARTESIAN_POINT('Ctrl Pts',(-0.164303537530501,19.75605264159,1.75369573568429));
#37304=CARTESIAN_POINT('Ctrl Pts',(-0.12726676960698,19.756042009416,1.75406883492907));
#37305=CARTESIAN_POINT('Ctrl Pts',(-0.105085352581457,19.7560356417792,
1.75429228504106));
#37306=CARTESIAN_POINT('Ctrl Pts',(-0.083159099614591,19.756030865463,1.75445479314168));
#37307=CARTESIAN_POINT('Ctrl Pts',(-0.0614883187664068,19.7560274595648,
1.75456043379643));
#37308=CARTESIAN_POINT('Ctrl Pts',(-0.0416894052580165,19.7560243478595,
1.75465694947812));
#37309=CARTESIAN_POINT('Ctrl Pts',(-0.023098772166832,19.7560224658573,
1.75470533215409));
#37310=CARTESIAN_POINT('Ctrl Pts',(-0.00298939254024861,19.7560213847532,
1.75471055941785));
#37311=CARTESIAN_POINT('Ctrl Pts',(-0.00108817250963598,19.7560212825414,
1.75471105362397));
#37312=CARTESIAN_POINT('Ctrl Pts',(0.000826622955876557,19.7560211896314,
1.75471112377803));
#37313=CARTESIAN_POINT('Ctrl Pts',(0.00275729841146969,19.7560211070343,
1.75471074952977));
#37314=CARTESIAN_POINT('Ctrl Pts',(0.115372251369809,19.7560162891981,1.75468891989025));
#37315=CARTESIAN_POINT('Ctrl Pts',(0.233541293580167,19.756051648623,1.75316490828795));
#37316=CARTESIAN_POINT('Ctrl Pts',(0.357210305664608,19.7561526751189,1.74966615574549));
#37317=CARTESIAN_POINT('Ctrl Pts',(0.400712688642062,19.7561882126658,1.74843541838874));
#37318=CARTESIAN_POINT('Ctrl Pts',(0.444895373831161,19.7562318941872,1.7469599398188));
#37319=CARTESIAN_POINT('Ctrl Pts',(0.489755120375023,19.7562848885263,1.74521788431246));
#37320=CARTESIAN_POINT('Ctrl Pts',(0.617020182699277,19.7564352310579,1.74027575200749));
#37321=CARTESIAN_POINT('Ctrl Pts',(0.749737195266465,19.7566605042835,1.7331905062554));
#37322=CARTESIAN_POINT('Ctrl Pts',(0.887807199413158,19.7569855787757,1.72345410257963));
#37323=CARTESIAN_POINT('Ctrl Pts',(0.982313920912144,19.7572080870946,1.71678968914476));
#37324=CARTESIAN_POINT('Ctrl Pts',(1.0793279137614,19.757477368534,1.70888243905592));
#37325=CARTESIAN_POINT('Ctrl Pts',(1.17880639802586,19.7578014745625,1.69956056995609));
#37326=CARTESIAN_POINT('Ctrl Pts',(1.32359504506791,19.7582732034364,1.6859928037718));
#37327=CARTESIAN_POINT('Ctrl Pts',(1.47360658000716,19.7588610528274,1.66942884858532));
#37328=CARTESIAN_POINT('Ctrl Pts',(1.62867912020213,19.759591057639,1.64933425855342));
#37329=CARTESIAN_POINT('Ctrl Pts',(1.68661969450315,19.7598638132022,1.6418262104791));
#37330=CARTESIAN_POINT('Ctrl Pts',(1.745266335463,19.7601564163829,1.63382506353029));
#37331=CARTESIAN_POINT('Ctrl Pts',(1.80460884493939,19.7604702288167,1.62530222939973));
#37332=CARTESIAN_POINT('Ctrl Pts',(1.96234369330212,19.7613043552649,1.60264818323506));
#37333=CARTESIAN_POINT('Ctrl Pts',(2.12499858771291,19.7622883739304,1.57630875695046));
#37334=CARTESIAN_POINT('Ctrl Pts',(2.29235845918953,19.7634470127006,1.54575752526289));
#37335=CARTESIAN_POINT('Ctrl Pts',(2.31272979552248,19.7635880442386,1.54203877589601));
#37336=CARTESIAN_POINT('Ctrl Pts',(2.33317077852849,19.7637316621987,1.53825761547812));
#37337=CARTESIAN_POINT('Ctrl Pts',(2.35368096675343,19.7638779104546,1.53441308861661));
#37338=CARTESIAN_POINT('Ctrl Pts',(2.36244932396459,19.763940433379,1.53276950619505));
#37339=CARTESIAN_POINT('Ctrl Pts',(2.37123032943377,19.7640034370317,1.53111434247959));
#37340=CARTESIAN_POINT('Ctrl Pts',(2.38002394991334,19.7640669248047,1.52944752508434));
#37341=CARTESIAN_POINT('Ctrl Pts',(2.44796163818883,19.7645574181728,1.51657003953969));
#37342=CARTESIAN_POINT('Ctrl Pts',(2.516652401437,19.7650768099106,1.50299696253616));
#37343=CARTESIAN_POINT('Ctrl Pts',(2.58608013114986,19.7656266494358,1.48869496643244));
#37344=CARTESIAN_POINT('Ctrl Pts',(2.6207939960063,19.7659015691984,1.48154396838058));
#37345=CARTESIAN_POINT('Ctrl Pts',(2.65569210204061,19.7661840995595,1.47421073840017));
#37346=CARTESIAN_POINT('Ctrl Pts',(2.69077227963222,19.766474432379,1.46669112701405));
#37347=CARTESIAN_POINT('Ctrl Pts',(2.70831236842803,19.7666195987888,1.46293132132099));
#37348=CARTESIAN_POINT('Ctrl Pts',(2.72589797509413,19.766766715751,1.45912492017669));
#37349=CARTESIAN_POINT('Ctrl Pts',(2.74352882315658,19.7669158068842,1.45527140537114));
#37350=CARTESIAN_POINT('Ctrl Pts',(2.75885335747361,19.7670453952159,1.45192197375732));
#37351=CARTESIAN_POINT('Ctrl Pts',(2.77563086515661,19.7671886585484,1.44822226782758));
#37352=CARTESIAN_POINT('Ctrl Pts',(2.79016150548294,19.7673138554393,1.44499224823921));
#37353=CARTESIAN_POINT('Ctrl Pts',(2.79234833966799,19.7673326973371,1.44450613633391));
#37354=CARTESIAN_POINT('Ctrl Pts',(2.79448430511413,19.767351125253,1.4440307576573));
#37355=CARTESIAN_POINT('Ctrl Pts',(2.79655681221918,19.7673690262237,1.44356900191366));
#37356=CARTESIAN_POINT('Ctrl Pts',(2.81154965113721,19.7674985246312,1.44022858900649));
#37357=CARTESIAN_POINT('Ctrl Pts',(2.82653642438921,19.7676292907192,1.43686249766563));
#37358=CARTESIAN_POINT('Ctrl Pts',(2.84151705021888,19.7677613187565,1.43347080813785));
#37359=CARTESIAN_POINT('Ctrl Pts',(2.98776394153726,19.7690502295293,1.40035977156335));
#37360=CARTESIAN_POINT('Ctrl Pts',(3.13342495769287,19.7704594133585,1.3648091206432));
#37361=CARTESIAN_POINT('Ctrl Pts',(3.2784330609518,19.7719831585219,1.32690145389342));
#37362=CARTESIAN_POINT('Ctrl Pts',(3.40982133405652,19.7733637865086,1.29255425011828));
#37363=CARTESIAN_POINT('Ctrl Pts',(3.54067358326317,19.7748384660325,1.25627200018786));
#37364=CARTESIAN_POINT('Ctrl Pts',(3.67094621226374,19.7764026120794,1.21812030633583));
#37365=CARTESIAN_POINT('Ctrl Pts',(3.7881200872732,19.7778094851487,1.18380471877831));
#37366=CARTESIAN_POINT('Ctrl Pts',(3.90482504209593,19.7792887378654,1.1479767276728));
#37367=CARTESIAN_POINT('Ctrl Pts',(4.02103364167433,19.7808367149258,1.11068613714232));
#37368=CARTESIAN_POINT('Ctrl Pts',(4.12467629572365,19.7822173051019,1.07742787753273));
#37369=CARTESIAN_POINT('Ctrl Pts',(4.2279241350384,19.7836525606924,1.04300622655274));
#37370=CARTESIAN_POINT('Ctrl Pts',(4.33076048984269,19.785139615806,1.0074574580962));
#37371=CARTESIAN_POINT('Ctrl Pts',(4.42239072069803,19.7864646258533,0.975782454966282));
#37372=CARTESIAN_POINT('Ctrl Pts',(4.51369425993899,19.7878307615007,0.943212595677556));
#37373=CARTESIAN_POINT('Ctrl Pts',(4.60466112206805,19.7892357879126,0.909773922350126));
#37374=CARTESIAN_POINT('Ctrl Pts',(4.68608243726572,19.7904933788162,0.879844113878531));
#37375=CARTESIAN_POINT('Ctrl Pts',(4.76723402584457,19.7917821269742,0.849218261921288));
#37376=CARTESIAN_POINT('Ctrl Pts',(4.8481099504637,19.7931003253408,0.817915114826047));
#37377=CARTESIAN_POINT('Ctrl Pts',(4.92103350007437,19.7942889077828,0.789689946323553));
#37378=CARTESIAN_POINT('Ctrl Pts',(4.99373293117401,19.7955014337815,0.760914129013177));
#37379=CARTESIAN_POINT('Ctrl Pts',(5.06620476601318,19.7967367222911,0.7316012532215));
#37380=CARTESIAN_POINT('Ctrl Pts',(5.13210508904211,19.7978599988302,0.704946374290041));
#37381=CARTESIAN_POINT('Ctrl Pts',(5.19781721936355,19.7990020970862,0.677847418887374));
#37382=CARTESIAN_POINT('Ctrl Pts',(5.26333917796051,19.8001625171985,0.650314189646983));
#37383=CARTESIAN_POINT('Ctrl Pts',(5.32292135272205,19.8012177413617,0.62527693936511));
#37384=CARTESIAN_POINT('Ctrl Pts',(5.38234627172783,19.8022881159988,0.599880583260539));
#37385=CARTESIAN_POINT('Ctrl Pts',(5.44161281821192,19.8033742625133,0.574131675940057));
#37386=CARTESIAN_POINT('Ctrl Pts',(5.4953806268887,19.804359636581,0.550771746864127));
#37387=CARTESIAN_POINT('Ctrl Pts',(5.54901808656126,19.8053579912684,0.527121650695065));
#37388=CARTESIAN_POINT('Ctrl Pts',(5.60252433633247,19.8063718735624,0.503184808992108));
#37389=CARTESIAN_POINT('Ctrl Pts',(5.64725600054545,19.8072194874863,0.483173412754208));
#37390=CARTESIAN_POINT('Ctrl Pts',(5.69189596083383,19.8080779529814,0.462961605831743));
#37391=CARTESIAN_POINT('Ctrl Pts',(5.73644276371326,19.8089520713578,0.442549442048373));
#37392=CARTESIAN_POINT('Ctrl Pts',(-5.843530256069,19.9729830063932,0.275592041905464));
#37393=CARTESIAN_POINT('Ctrl Pts',(-3.895686837379,19.9313476995223,1.19822036162746));
#37394=CARTESIAN_POINT('Ctrl Pts',(0.0001633689301563,19.8897491923651,
2.12096446775537));
#37395=CARTESIAN_POINT('Ctrl Pts',(3.896013575239,19.9313511884663,1.19814296951903));
#37396=CARTESIAN_POINT('Ctrl Pts',(5.844020362859,19.9729934829082,0.27535988496917));
#37397=CARTESIAN_POINT('Ctrl Pts',(-5.843530256069,19.2592933206554,0.803936154133969));
#37398=CARTESIAN_POINT('Ctrl Pts',(-3.895686837379,19.2409363277008,1.65690464245717));
#37399=CARTESIAN_POINT('Ctrl Pts',(0.0001633689301563,19.2238042428705,
2.51235960005451));
#37400=CARTESIAN_POINT('Ctrl Pts',(3.896013575239,19.2409377645976,1.65683289399886));
#37401=CARTESIAN_POINT('Ctrl Pts',(5.844020362859,19.2592979397557,0.803721525417513));
#37402=CARTESIAN_POINT('Ctrl Pts',(-5.843530256069,17.6858134778517,1.67939840409943));
#37403=CARTESIAN_POINT('Ctrl Pts',(-3.895686837379,17.747795303743,2.42360809969946));
#37404=CARTESIAN_POINT('Ctrl Pts',(0.0001633689301563,17.8092308148508,
3.16660344766129));
#37405=CARTESIAN_POINT('Ctrl Pts',(3.896013575239,17.7477901510419,2.42354578341948));
#37406=CARTESIAN_POINT('Ctrl Pts',(5.844020362859,17.6857978816304,1.67921114184714));
#37407=CARTESIAN_POINT('Ctrl Pts',(-5.843530256069,15.061425464425,2.34071387945854));
#37408=CARTESIAN_POINT('Ctrl Pts',(-3.895686837379,15.2991206306999,3.03320174206447));
#37409=CARTESIAN_POINT('Ctrl Pts',(0.0001633689301563,15.5368877409622,
3.72636654306873));
#37410=CARTESIAN_POINT('Ctrl Pts',(3.896013575239,15.2991006887715,3.03314360515765));
#37411=CARTESIAN_POINT('Ctrl Pts',(5.844020362859,15.0613656542254,2.34053963176309));
#37412=CARTESIAN_POINT('Ctrl Pts',(-5.843530256069,12.4568749910185,2.30089104535593));
#37413=CARTESIAN_POINT('Ctrl Pts',(-3.895686837379,12.8710990247508,3.06727942102254));
#37414=CARTESIAN_POINT('Ctrl Pts',(0.0001633689301563,13.2856337337471,
3.83244175204731));
#37415=CARTESIAN_POINT('Ctrl Pts',(3.896013575239,12.8710642570284,3.06721524556422));
#37416=CARTESIAN_POINT('Ctrl Pts',(5.844020362859,12.4567707616288,2.30069820237451));
#37417=CARTESIAN_POINT('Ctrl Pts',(-5.843530256069,10.8186489886147,1.86225011026657));
#37418=CARTESIAN_POINT('Ctrl Pts',(-3.895686837379,11.3231612494621,2.74792678860542));
#37419=CARTESIAN_POINT('Ctrl Pts',(0.0001633689301563,11.8270703511712,
3.63585972809697));
#37420=CARTESIAN_POINT('Ctrl Pts',(3.896013575239,11.3231189857497,2.74785231616274));
#37421=CARTESIAN_POINT('Ctrl Pts',(5.844020362859,10.8185220403858,1.86202725132894));
#37422=CARTESIAN_POINT('Ctrl Pts',(-5.843530256069,10.0864302299624,1.57297372755727));
#37423=CARTESIAN_POINT('Ctrl Pts',(-3.895686837379,10.6220961848295,2.52888112716319));
#37424=CARTESIAN_POINT('Ctrl Pts',(0.0001633689301563,11.1575638447486,
3.48561783754201));
#37425=CARTESIAN_POINT('Ctrl Pts',(3.896013575239,10.6220512742479,2.52880088403233));
#37426=CARTESIAN_POINT('Ctrl Pts',(5.844020362859,10.0862954426721,1.57273319675619));
#37427=CARTESIAN_POINT('',(-5.73278769720861,10.3449530899586,1.712890664259));
#37428=CARTESIAN_POINT('Ctrl Pts',(-5.73644356954166,19.8089503607377,0.442546999707748));
#37429=CARTESIAN_POINT('Ctrl Pts',(-5.73766037024446,19.1301825683204,0.92173330072201));
#37430=CARTESIAN_POINT('Ctrl Pts',(-5.73849618482638,18.3938460451307,1.3183902211696));
#37431=CARTESIAN_POINT('Ctrl Pts',(-5.73940756701135,16.8491829816311,1.92343296529744));
#37432=CARTESIAN_POINT('Ctrl Pts',(-5.739483134547,16.0408992661184,2.13191056540138));
#37433=CARTESIAN_POINT('Ctrl Pts',(-5.73887402246419,14.4000963224447,2.35028699819193));
#37434=CARTESIAN_POINT('Ctrl Pts',(-5.73818934284575,13.5675419891499,2.35984313691093));
#37435=CARTESIAN_POINT('Ctrl Pts',(-5.73605973645477,11.9265541605029,2.18169283770349));
#37436=CARTESIAN_POINT('Ctrl Pts',(-5.73461480968224,11.1182366055945,1.99332811253109));
#37437=CARTESIAN_POINT('Ctrl Pts',(-5.732787914148,10.3449528797153,1.71289124180765));
#37438=CARTESIAN_POINT('Ctrl Pts',(5.73278688072817,10.3449507250975,1.71289711535081));
#37439=CARTESIAN_POINT('Ctrl Pts',(5.37900915639315,10.4448363651221,1.88168165915975));
#37440=CARTESIAN_POINT('Ctrl Pts',(5.01621168019062,10.5336327228737,2.03732074407881));
#37441=CARTESIAN_POINT('Ctrl Pts',(4.64600744793163,10.6117450667191,2.17807213827088));
#37442=CARTESIAN_POINT('Ctrl Pts',(4.37165126939791,10.6696336651907,2.28238216843503));
#37443=CARTESIAN_POINT('Ctrl Pts',(4.0932271486741,10.7216541652371,2.3785116388909));
#37444=CARTESIAN_POINT('Ctrl Pts',(3.81139161388638,10.7679952015392,2.4657654271308));
#37445=CARTESIAN_POINT('Ctrl Pts',(3.57235159836392,10.8072995498901,2.53977010120772));
#37446=CARTESIAN_POINT('Ctrl Pts',(3.33085752862551,10.8425181299936,2.60738913673008));
#37447=CARTESIAN_POINT('Ctrl Pts',(3.08730997420282,10.8737883242848,2.66823233499462));
#37448=CARTESIAN_POINT('Ctrl Pts',(3.04370746675433,10.8793866514071,2.6791251399411));
#37449=CARTESIAN_POINT('Ctrl Pts',(3.00003914097686,10.8848584940772,2.68980088077536));
#37450=CARTESIAN_POINT('Ctrl Pts',(2.95630729545765,10.890204737468,2.7002574814574));
#37451=CARTESIAN_POINT('Ctrl Pts',(2.75784869263507,10.9144664163677,2.74771036932422));
#37452=CARTESIAN_POINT('Ctrl Pts',(2.55807717076884,10.9362024498221,2.79066539146926));
#37453=CARTESIAN_POINT('Ctrl Pts',(2.35725950625594,10.9553925153308,2.82890669523075));
#37454=CARTESIAN_POINT('Ctrl Pts',(2.16328572644567,10.9739285816203,2.86584473179981));
#37455=CARTESIAN_POINT('Ctrl Pts',(1.96833589422108,10.9900892362504,2.8983848066184));
#37456=CARTESIAN_POINT('Ctrl Pts',(1.77265042967068,11.0038798224107,2.92637432499266));
#37457=CARTESIAN_POINT('Ctrl Pts',(1.58005635303568,11.0174525484887,2.953921672258));
#37458=CARTESIAN_POINT('Ctrl Pts',(1.3867497031393,11.0287294251743,2.9770609588758));
#37459=CARTESIAN_POINT('Ctrl Pts',(1.19295968484454,11.0377396538332,2.99568970691917));
#37460=CARTESIAN_POINT('Ctrl Pts',(0.994821339892144,11.046952057082,3.01473645317746));
#37461=CARTESIAN_POINT('Ctrl Pts',(0.79617769120483,11.0537947132516,3.02906753346601));
#37462=CARTESIAN_POINT('Ctrl Pts',(0.597273721365771,11.0583268153071,3.03862354819703));
#37463=CARTESIAN_POINT('Ctrl Pts',(0.408482784336276,11.0626284880916,3.04769369886722));
#37464=CARTESIAN_POINT('Ctrl Pts',(0.219457324631945,11.0648487064693,3.05246221354261));
#37465=CARTESIAN_POINT('Ctrl Pts',(0.030406825010438,11.0650633093697,3.05292359624673));
#37466=CARTESIAN_POINT('Ctrl Pts',(0.0202798881170744,11.0650748050814,
3.0529483113019));
#37467=CARTESIAN_POINT('Ctrl Pts',(0.0101528793726079,11.0650805518247,
3.0529606781068));
#37468=CARTESIAN_POINT('Ctrl Pts',(2.58309765375194E-5,11.0650805633313,
3.0529606995424));
#37469=CARTESIAN_POINT('Ctrl Pts',(1.72206505356609E-5,11.0650805633411,
3.05296069956063));
#37470=CARTESIAN_POINT('Ctrl Pts',(8.6103245629562E-6,11.0650805633467,
3.05296069956993));
#37471=CARTESIAN_POINT('Ctrl Pts',(-1.38233868796078E-12,11.0650805633482,
3.05296069957031));
#37472=CARTESIAN_POINT('Ctrl Pts',(-0.189404607484898,11.0650805961548,
3.05296070785262));
#37473=CARTESIAN_POINT('Ctrl Pts',(-0.378795525024171,11.0630723256102,
3.0486385112057));
#37474=CARTESIAN_POINT('Ctrl Pts',(-0.567962091433974,11.0589781342605,
3.03999720067297));
#37475=CARTESIAN_POINT('Ctrl Pts',(-0.769360885412324,11.0546191969715,
3.03079711023038));
#37476=CARTESIAN_POINT('Ctrl Pts',(-0.970505375368339,11.0478956606748,
3.01670092928917));
#37477=CARTESIAN_POINT('Ctrl Pts',(-1.17114133412378,11.0387447797368,2.99776792292822));
#37478=CARTESIAN_POINT('Ctrl Pts',(-1.36695479531859,11.0298138499047,2.97928999140808));
#37479=CARTESIAN_POINT('Ctrl Pts',(-1.56228387768899,11.0185711098174,2.95620541448577));
#37480=CARTESIAN_POINT('Ctrl Pts',(-1.75689224881912,11.0049856060652,2.92861833910982));
#37481=CARTESIAN_POINT('Ctrl Pts',(-1.95868984781945,10.9908982262547,2.90001214122645));
#37482=CARTESIAN_POINT('Ctrl Pts',(-2.15971250294576,10.974291784558,2.86656464096982));
#37483=CARTESIAN_POINT('Ctrl Pts',(-2.35969671049328,10.9551601078216,2.82844251062265));
#37484=CARTESIAN_POINT('Ctrl Pts',(-2.5596809180408,10.9360284310852,2.79032038027548));
#37485=CARTESIAN_POINT('Ctrl Pts',(-2.75862667800953,10.9143716955401,2.74752395482592));
#37486=CARTESIAN_POINT('Ctrl Pts',(-2.95627048669471,10.8902100153768,2.70026650193579));
#37487=CARTESIAN_POINT('Ctrl Pts',(-3.19876727229057,10.8605651212961,2.6422845165777));
#37488=CARTESIAN_POINT('Ctrl Pts',(-3.43931126880089,10.8270560244705,2.57756053855471));
#37489=CARTESIAN_POINT('Ctrl Pts',(-3.6775105439921,10.7895434778164,2.50646830223344));
#37490=CARTESIAN_POINT('Ctrl Pts',(-3.96232663863318,10.7446895334477,2.42146295076009));
#37491=CARTESIAN_POINT('Ctrl Pts',(-4.24379045999574,10.6941119076844,2.3273536438739));
#37492=CARTESIAN_POINT('Ctrl Pts',(-4.5212319950369,10.6376130683546,2.22484295869238));
#37493=CARTESIAN_POINT('Ctrl Pts',(-4.88826612190385,10.5628693852961,2.08922909026223));
#37494=CARTESIAN_POINT('Ctrl Pts',(-5.24826073085707,10.4777633055356,1.93891800459309));
#37495=CARTESIAN_POINT('Ctrl Pts',(-5.59966454915396,10.3818999325314,1.77558871976231));
#37496=CARTESIAN_POINT('Ctrl Pts',(-5.64417852204767,10.3697564686154,1.75489903177615));
#37497=CARTESIAN_POINT('Ctrl Pts',(-5.68855464299647,10.3574404414096,1.73400040081192));
#37498=CARTESIAN_POINT('Ctrl Pts',(-5.73278975875473,10.3449510884962,1.71289616977594));
#37499=CARTESIAN_POINT('Ctrl Pts',(5.84420424599312,10.3325630763309,1.66676549536465));
#37500=CARTESIAN_POINT('Ctrl Pts',(5.38649680477895,10.4714443877546,1.89197696257757));
#37501=CARTESIAN_POINT('Ctrl Pts',(4.35413199008094,10.731355617357,2.33432632451635));
#37502=CARTESIAN_POINT('Ctrl Pts',(2.6892293910766,10.9922428541574,2.81982521043073));
#37503=CARTESIAN_POINT('Ctrl Pts',(0.897914376059795,11.1229571043403,3.07976795890079));
#37504=CARTESIAN_POINT('Ctrl Pts',(-0.894835170638287,11.123066538772,3.07999087254476));
#37505=CARTESIAN_POINT('Ctrl Pts',(-2.68616412898614,10.9925867227746,2.82049345526273));
#37506=CARTESIAN_POINT('Ctrl Pts',(-4.35222081536794,10.7317832826312,2.33508087721848));
#37507=CARTESIAN_POINT('Ctrl Pts',(-5.38563860711213,10.47170896242,1.89240417822602));
#37508=CARTESIAN_POINT('Ctrl Pts',(-5.84432042005851,10.3325278530965,1.66670829119904));
#37509=CARTESIAN_POINT('Ctrl Pts',(5.72538510600853,10.0514967496063,1.59489562708686));
#37510=CARTESIAN_POINT('Ctrl Pts',(5.27689078630208,10.1880792428534,1.81386477497724));
#37511=CARTESIAN_POINT('Ctrl Pts',(4.26533502063675,10.4437816859558,2.2441276685875));
#37512=CARTESIAN_POINT('Ctrl Pts',(2.63420875168904,10.7005792227098,2.71656172834629));
#37513=CARTESIAN_POINT('Ctrl Pts',(0.879504392503219,10.8292887596862,2.96954569268241));
#37514=CARTESIAN_POINT('Ctrl Pts',(-0.876488283445119,10.8293965289089,
2.96976264371174));
#37515=CARTESIAN_POINT('Ctrl Pts',(-2.63120592811252,10.700917777909,2.7172120634047));
#37516=CARTESIAN_POINT('Ctrl Pts',(-4.26346240346891,10.4442025274368,2.24486177732035));
#37517=CARTESIAN_POINT('Ctrl Pts',(-5.27604986041985,10.188339433728,1.81428014237951));
#37518=CARTESIAN_POINT('Ctrl Pts',(-5.72549894105245,10.0514621102988,1.59484001174331));
#37519=CARTESIAN_POINT('Ctrl Pts',(5.71943960541124,9.77839678543227,1.74872366789884));
#37520=CARTESIAN_POINT('Ctrl Pts',(5.27224638947531,9.91364416277643,1.9653747050709));
#37521=CARTESIAN_POINT('Ctrl Pts',(4.26336592362135,10.1670212916803,2.39142245426171));
#37522=CARTESIAN_POINT('Ctrl Pts',(2.63459204266588,10.4218933752604,2.86015313741059));
#37523=CARTESIAN_POINT('Ctrl Pts',(0.879984211070912,10.5498274753047,3.11161319304617));
#37524=CARTESIAN_POINT('Ctrl Pts',(-0.876966788137325,10.5499346576453,
3.11182899606998));
#37525=CARTESIAN_POINT('Ctrl Pts',(-2.63159126948949,10.4222297095009,2.86079911077524));
#37526=CARTESIAN_POINT('Ctrl Pts',(-4.26149794683647,10.1674385327164,2.39214984759134));
#37527=CARTESIAN_POINT('Ctrl Pts',(-5.27140792789829,9.91390180831679,1.96578563564803));
#37528=CARTESIAN_POINT('Ctrl Pts',(-5.71955311537339,9.77836248755778,1.74866863471185));
#37529=CARTESIAN_POINT('Ctrl Pts',(5.83022484041109,9.69039160441613,2.02848103772045));
#37530=CARTESIAN_POINT('Ctrl Pts',(5.3755767692724,9.82613351137638,2.24824169564194));
#37531=CARTESIAN_POINT('Ctrl Pts',(4.34950254584683,10.0805769763631,2.68067956629756));
#37532=CARTESIAN_POINT('Ctrl Pts',(2.69013112778482,10.3369366903571,3.15747035215418));
#37533=CARTESIAN_POINT('Ctrl Pts',(0.899042785899667,10.4658275761937,3.41382980296367));
#37534=CARTESIAN_POINT('Ctrl Pts',(-0.895960490475546,10.4659356306253,
3.41405001720562));
#37535=CARTESIAN_POINT('Ctrl Pts',(-2.68707068653567,10.3372753366022,3.15812834094409));
#37536=CARTESIAN_POINT('Ctrl Pts',(-4.3476022823214,10.0809961755248,2.68141832841113));
#37537=CARTESIAN_POINT('Ctrl Pts',(-5.37472436608816,9.82639210091812,2.24865847853217));
#37538=CARTESIAN_POINT('Ctrl Pts',(-5.83034025009099,9.6903571840313,2.02842520243865));
#37539=CARTESIAN_POINT('',(-5.72001816061901,9.72697624291305,2.05943242314956));
#37540=CARTESIAN_POINT('Origin',(-5.89877612790054,10.1838113533859,2.15616400895824));
#37541=CARTESIAN_POINT('Ctrl Pts',(5.72001490840061,9.72697523518687,2.05943402421887));
#37542=CARTESIAN_POINT('Ctrl Pts',(5.51235198943714,9.78739731182845,2.15782078059172));
#37543=CARTESIAN_POINT('Ctrl Pts',(5.29964847952653,9.84440335009143,2.25259520759938));
#37544=CARTESIAN_POINT('Ctrl Pts',(5.08198158984127,9.8979028691542,2.34311806232899));
#37545=CARTESIAN_POINT('Ctrl Pts',(4.87630120287531,9.94845627118625,2.42865599516285));
#37546=CARTESIAN_POINT('Ctrl Pts',(4.66618904522251,9.99587865664118,2.51039747519363));
#37547=CARTESIAN_POINT('Ctrl Pts',(4.45173460952731,10.0400902988936,2.58775796338993));
#37548=CARTESIAN_POINT('Ctrl Pts',(4.43923677872028,10.0426668351297,2.5922663256884));
#37549=CARTESIAN_POINT('Ctrl Pts',(4.42672420769387,10.0452324660357,2.59675979619238));
#37550=CARTESIAN_POINT('Ctrl Pts',(4.41419691688718,10.0477871755214,2.60123825439549));
#37551=CARTESIAN_POINT('Ctrl Pts',(4.40407569623453,10.0498512114576,2.6048565517877));
#37552=CARTESIAN_POINT('Ctrl Pts',(4.39394486714726,10.0519081183605,2.60846504978682));
#37553=CARTESIAN_POINT('Ctrl Pts',(4.38380444711611,10.0539578885756,2.61206368468342));
#37554=CARTESIAN_POINT('Ctrl Pts',(4.17192365805595,10.0967871726915,2.68725599418255));
#37555=CARTESIAN_POINT('Ctrl Pts',(3.95585617378088,10.1364960011834,2.75816495889607));
#37556=CARTESIAN_POINT('Ctrl Pts',(3.73575047118406,10.1729824351331,2.82430882007291));
#37557=CARTESIAN_POINT('Ctrl Pts',(3.71382288922425,10.1766173217417,2.83089826741563));
#37558=CARTESIAN_POINT('Ctrl Pts',(3.69185523817543,10.1802202209102,2.8374403809089));
#37559=CARTESIAN_POINT('Ctrl Pts',(3.66984767104303,10.1837910278748,2.84393465629152));
#37560=CARTESIAN_POINT('Ctrl Pts',(3.54838959673465,10.2034980375156,2.87977606380628));
#37561=CARTESIAN_POINT('Ctrl Pts',(3.42571635010909,10.2222269093428,2.91416268775258));
#37562=CARTESIAN_POINT('Ctrl Pts',(3.30185884873608,10.2399551345675,2.94701908582717));
#37563=CARTESIAN_POINT('Ctrl Pts',(3.23993009804958,10.2488192471798,2.96344728486447));
#37564=CARTESIAN_POINT('Ctrl Pts',(3.17770527845606,10.2574331732445,2.97949292001389));
#37565=CARTESIAN_POINT('Ctrl Pts',(3.11518875344279,10.2657937072243,2.99514699337891));
#37566=CARTESIAN_POINT('Ctrl Pts',(3.08393049093615,10.2699739742143,3.00297403006142));
#37567=CARTESIAN_POINT('Ctrl Pts',(3.05259930187275,10.2740908918314,3.01070317587191));
#37568=CARTESIAN_POINT('Ctrl Pts',(3.02119574738027,10.2781440430835,3.01833332061816));
#37569=CARTESIAN_POINT('Ctrl Pts',(2.99854982368428,10.2810668763571,3.02383561736467));
#37570=CARTESIAN_POINT('Ctrl Pts',(2.9748857110574,10.2840806737505,3.02952098717871));
#37571=CARTESIAN_POINT('Ctrl Pts',(2.9523245541333,10.2869160467782,3.0348804082814));
#37572=CARTESIAN_POINT('Ctrl Pts',(2.94359970433979,10.2880125421334,3.0369530034173));
#37573=CARTESIAN_POINT('Ctrl Pts',(2.93503996082666,10.2890826369461,3.03897732516861));
#37574=CARTESIAN_POINT('Ctrl Pts',(2.92676855739885,10.2901117713241,3.04092564871964));
#37575=CARTESIAN_POINT('Ctrl Pts',(2.83652357254174,10.3013401217689,3.06218279460714));
#37576=CARTESIAN_POINT('Ctrl Pts',(2.74597262321716,10.3120229794392,3.08250464961453));
#37577=CARTESIAN_POINT('Ctrl Pts',(2.65513062758051,10.3221651214447,3.10187144875567));
#37578=CARTESIAN_POINT('Ctrl Pts',(2.39635416121228,10.3510564690113,3.15704055651781));
#37579=CARTESIAN_POINT('Ctrl Pts',(2.13521677961336,10.3755617409481,3.20446287311253));
#37580=CARTESIAN_POINT('Ctrl Pts',(1.87219104066715,10.3957416660273,3.24382759350234));
#37581=CARTESIAN_POINT('Ctrl Pts',(1.61422025029409,10.4155337641057,3.28243578474802));
#37582=CARTESIAN_POINT('Ctrl Pts',(1.35443247684423,10.4311650650209,3.31329332864275));
#37583=CARTESIAN_POINT('Ctrl Pts',(1.09326623534793,10.4426713053128,3.33606238398908));
#37584=CARTESIAN_POINT('Ctrl Pts',(1.02414978900039,10.445716378961,3.3420881099145));
#37585=CARTESIAN_POINT('Ctrl Pts',(0.954936781483695,10.4484724306796,3.34754708449844));
#37586=CARTESIAN_POINT('Ctrl Pts',(0.885635322910046,10.4509398774855,3.35243247792281));
#37587=CARTESIAN_POINT('Ctrl Pts',(0.622150988790217,10.4603211169571,3.37100675701921));
#37588=CARTESIAN_POINT('Ctrl Pts',(0.357387451141609,10.4655323006477,3.38129329316036));
#37589=CARTESIAN_POINT('Ctrl Pts',(0.0918656894087061,10.4665095187268,
3.3832237866013));
#37590=CARTESIAN_POINT('Ctrl Pts',(0.0612581983271671,10.4666221655903,
3.38344632037929));
#37591=CARTESIAN_POINT('Ctrl Pts',(0.0306406423813369,10.4666785268953,
3.38355777001305));
#37592=CARTESIAN_POINT('Ctrl Pts',(1.38288139147356E-5,10.4666784850131,
3.38355799146479));
#37593=CARTESIAN_POINT('Ctrl Pts',(-0.260471068774009,10.4666781287992,
3.38355987493963));
#37594=CARTESIAN_POINT('Ctrl Pts',(-0.520268343612212,10.4625922845768,
3.37554239434947));
#37595=CARTESIAN_POINT('Ctrl Pts',(-0.778903582148321,10.4544897161825,
3.35956035939152));
#37596=CARTESIAN_POINT('Ctrl Pts',(-0.813491042715138,10.4534061543816,
3.35742307134441));
#37597=CARTESIAN_POINT('Ctrl Pts',(-0.848057728692277,10.4522507238744,
3.35514327831035));
#37598=CARTESIAN_POINT('Ctrl Pts',(-0.882602510186255,10.4510235576393,
3.35272104898075));
#37599=CARTESIAN_POINT('Ctrl Pts',(-1.08260237594735,10.4439187773607,3.33869735220771));
#37600=CARTESIAN_POINT('Ctrl Pts',(-1.28186813818427,10.4344100971061,3.31990076044197));
#37601=CARTESIAN_POINT('Ctrl Pts',(-1.48021120198736,10.4224869677621,3.29648136837608));
#37602=CARTESIAN_POINT('Ctrl Pts',(-1.72460014088733,10.4077958519104,3.2676251015275));
#37603=CARTESIAN_POINT('Ctrl Pts',(-1.96757580743929,10.3894539541556,3.2317098037961));
#37604=CARTESIAN_POINT('Ctrl Pts',(-2.20877711737513,10.3674169612257,3.18901198452615));
#37605=CARTESIAN_POINT('Ctrl Pts',(-2.32937777234304,10.3563984647607,3.16766307489118));
#37606=CARTESIAN_POINT('Ctrl Pts',(-2.44953515283027,10.3444552399712,3.14461997457069));
#37607=CARTESIAN_POINT('Ctrl Pts',(-2.56920598353283,10.331576080652,3.11992579982614));
#37608=CARTESIAN_POINT('Ctrl Pts',(-2.59686203949018,10.3285996932673,3.11421894983984));
#37609=CARTESIAN_POINT('Ctrl Pts',(-2.62449215450421,10.3255732879286,3.10842397436765));
#37610=CARTESIAN_POINT('Ctrl Pts',(-2.65209572000823,10.322496739247,3.10254136005408));
#37611=CARTESIAN_POINT('Ctrl Pts',(-2.68421400384005,10.318917003732,3.09569661109696));
#37612=CARTESIAN_POINT('Ctrl Pts',(-2.7162963432974,10.3152693811637,3.08873321145855));
#37613=CARTESIAN_POINT('Ctrl Pts',(-2.74834204355002,10.3115536050379,3.08165225587728));
#37614=CARTESIAN_POINT('Ctrl Pts',(-2.77813548600742,10.308098983628,3.07506896885309));
#37615=CARTESIAN_POINT('Ctrl Pts',(-2.80789721199739,10.3045854773189,3.06838401271604));
#37616=CARTESIAN_POINT('Ctrl Pts',(-2.83762657928914,10.3010129105985,3.06159817626225));
#37617=CARTESIAN_POINT('Ctrl Pts',(-2.85923495052844,10.2984162408741,3.05666598676008));
#37618=CARTESIAN_POINT('Ctrl Pts',(-2.87983096400873,10.2959101762994,3.05191147348056));
#37619=CARTESIAN_POINT('Ctrl Pts',(-2.90158490594942,10.2932296975479,3.0468324070001));
#37620=CARTESIAN_POINT('Ctrl Pts',(-2.90976061131236,10.2922223029081,3.04492355980467));
#37621=CARTESIAN_POINT('Ctrl Pts',(-2.91809973466331,10.2911900242974,3.04296845002873));
#37622=CARTESIAN_POINT('Ctrl Pts',(-2.92671696595623,10.2901178465306,3.04093882497416));
#37623=CARTESIAN_POINT('Ctrl Pts',(-3.15178238735407,10.2621146361379,2.98792894248901));
#37624=CARTESIAN_POINT('Ctrl Pts',(-3.37318101670882,10.2308852311845,2.92969863789928));
#37625=CARTESIAN_POINT('Ctrl Pts',(-3.59074180566845,10.1965240090342,2.86679780973399));
#37626=CARTESIAN_POINT('Ctrl Pts',(-3.81369841711418,10.1613105788366,2.80233694998106));
#37627=CARTESIAN_POINT('Ctrl Pts',(-4.03262451490004,10.1228081162286,2.73297091727145));
#37628=CARTESIAN_POINT('Ctrl Pts',(-4.24735524579871,10.0811143954969,2.65924060733081));
#37629=CARTESIAN_POINT('Ctrl Pts',(-4.30221094336249,10.0704632040015,2.64040526147015));
#37630=CARTESIAN_POINT('Ctrl Pts',(-4.35679293942059,10.0596037257926,2.62128484889262));
#37631=CARTESIAN_POINT('Ctrl Pts',(-4.41109867300135,10.0485375457635,2.60188788503165));
#37632=CARTESIAN_POINT('Ctrl Pts',(-4.63913382081059,10.0020695610366,2.52043811482444));
#37633=CARTESIAN_POINT('Ctrl Pts',(-4.86229671262369,9.95195749262712,2.434116675331));
#37634=CARTESIAN_POINT('Ctrl Pts',(-5.0804825496319,9.89832400754834,2.34351848583091));
#37635=CARTESIAN_POINT('Ctrl Pts',(-5.2986683866401,9.84469052246957,2.25292029633083));
#37636=CARTESIAN_POINT('Ctrl Pts',(-5.51187730087082,9.78753563449656,2.15804500081236));
#37637=CARTESIAN_POINT('Ctrl Pts',(-5.72001753333531,9.72697463976802,2.05943208370059));
#37638=CARTESIAN_POINT('Ctrl Pts',(-5.71201821360281,10.3745893795876,1.73089321988294));
#37639=CARTESIAN_POINT('Ctrl Pts',(-5.71753470941925,10.3728819373349,1.7286358487777));
#37640=CARTESIAN_POINT('Ctrl Pts',(-5.76529494709306,10.3582189611947,1.70809774779482));
#37641=CARTESIAN_POINT('Ctrl Pts',(-5.85055921091664,10.3340058651975,1.65506459479143));
#37642=CARTESIAN_POINT('Ctrl Pts',(-5.94855788476008,10.3111442455001,1.55167544971277));
#37643=CARTESIAN_POINT('Ctrl Pts',(-6.01625188434961,10.3010076858463,1.43149053235932));
#37644=CARTESIAN_POINT('Ctrl Pts',(-6.04732974734974,10.3030375271302,1.31928535914519));
#37645=CARTESIAN_POINT('Ctrl Pts',(-6.05141080953246,10.3096109683119,1.25173107752086));
#37646=CARTESIAN_POINT('Ctrl Pts',(-6.05071568539176,10.3130319392939,1.22538737377867));
#37647=CARTESIAN_POINT('Ctrl Pts',(-5.59596286913054,10.091024988519,1.65481426090108));
#37648=CARTESIAN_POINT('Ctrl Pts',(-5.60111045497149,10.0894199224357,1.65273810722318));
#37649=CARTESIAN_POINT('Ctrl Pts',(-5.64568435427929,10.0756272036296,1.63384806964916));
#37650=CARTESIAN_POINT('Ctrl Pts',(-5.72536755241762,10.0527126854641,1.5850500029164));
#37651=CARTESIAN_POINT('Ctrl Pts',(-5.81695324569551,10.0308278463846,1.48997227540393));
#37652=CARTESIAN_POINT('Ctrl Pts',(-5.88006365701701,10.020853739627,1.37978256343051));
#37653=CARTESIAN_POINT('Ctrl Pts',(-5.90886973469154,10.0223543906179,1.27753231866074));
#37654=CARTESIAN_POINT('Ctrl Pts',(-5.91261218350735,10.0282473351447,1.21648882520907));
#37655=CARTESIAN_POINT('Ctrl Pts',(-5.9119739864041,10.0313348077132,1.19278337685752));
#37656=CARTESIAN_POINT('Ctrl Pts',(-5.5788598499786,9.8189785998903,1.81407643830995));
#37657=CARTESIAN_POINT('Ctrl Pts',(-5.58617900390802,9.81673898600098,1.8111487551284));
#37658=CARTESIAN_POINT('Ctrl Pts',(-5.64948915158139,9.79753620524486,1.78454467298062));
#37659=CARTESIAN_POINT('Ctrl Pts',(-5.76170664028583,9.76626533716724,1.71642469728939));
#37660=CARTESIAN_POINT('Ctrl Pts',(-5.89067180786221,9.73709385598877,1.58418520698851));
#37661=CARTESIAN_POINT('Ctrl Pts',(-5.98091235554539,9.72423239118939,1.42907135224037));
#37662=CARTESIAN_POINT('Ctrl Pts',(-6.02360066369486,9.72705369891453,1.28087941931778));
#37663=CARTESIAN_POINT('Ctrl Pts',(-6.02950933576142,9.73602295206567,1.18866363771198));
#37664=CARTESIAN_POINT('Ctrl Pts',(-6.02850854633718,9.74076242253544,1.15211679278597));
#37665=CARTESIAN_POINT('Ctrl Pts',(-5.67191631397939,9.7367167713257,2.104318164895));
#37666=CARTESIAN_POINT('Ctrl Pts',(-5.68252452601478,9.73352149298544,2.100064196715));
#37667=CARTESIAN_POINT('Ctrl Pts',(-5.77421599484514,9.70617344358581,2.06143883184841));
#37668=CARTESIAN_POINT('Ctrl Pts',(-5.93576401678745,9.66236705788763,1.96310123941882));
#37669=CARTESIAN_POINT('Ctrl Pts',(-6.12140704144701,9.62242031220293,1.77257821790161));
#37670=CARTESIAN_POINT('Ctrl Pts',(-6.25271357804119,9.60551370991075,1.54705882731488));
#37671=CARTESIAN_POINT('Ctrl Pts',(-6.31634136597211,9.61064011934564,1.32713332299514));
#37672=CARTESIAN_POINT('Ctrl Pts',(-6.32550161226352,9.62442663858794,1.18648879700547));
#37673=CARTESIAN_POINT('Ctrl Pts',(-6.32395631113669,9.63172107981537,1.13003563160022));
#37674=CARTESIAN_POINT('',(-5.99998809173028,10.0933467245957,1.21103470346248));
#37675=CARTESIAN_POINT('',(-5.99999999616419,9.65438802498414,1.8624761678277));
#37676=CARTESIAN_POINT('Ctrl Pts',(-5.99998809173028,10.0933467245957,1.21103470346248));
#37677=CARTESIAN_POINT('Ctrl Pts',(-5.99998614033857,10.0742249652676,1.22561744409544));
#37678=CARTESIAN_POINT('Ctrl Pts',(-5.99998781129217,10.0554651409929,1.24052926194382));
#37679=CARTESIAN_POINT('Ctrl Pts',(-6.00000062824795,10.037183037652,1.25577699121628));
#37680=CARTESIAN_POINT('Ctrl Pts',(-6.00000707142198,10.0279924954203,1.26344213221258));
#37681=CARTESIAN_POINT('Ctrl Pts',(-6.0000156689702,10.0189226652474,1.27119157323869));
#37682=CARTESIAN_POINT('Ctrl Pts',(-6.00002447527685,10.0099875859112,1.27902227748033));
#37683=CARTESIAN_POINT('Ctrl Pts',(-6.0000429277041,9.99126533290177,1.29543046150826));
#37684=CARTESIAN_POINT('Ctrl Pts',(-6.0000639885918,9.97313591895691,1.31219831393756));
#37685=CARTESIAN_POINT('Ctrl Pts',(-6.0000852622,9.95570443374821,1.3292681789178));
#37686=CARTESIAN_POINT('Ctrl Pts',(-6.0000991408704,9.94433232255919,1.34040437300642));
#37687=CARTESIAN_POINT('Ctrl Pts',(-6.00011245325909,9.93325694654117,1.35166810031643));
#37688=CARTESIAN_POINT('Ctrl Pts',(-6.00012171175544,9.92250192113295,1.3630332377823));
#37689=CARTESIAN_POINT('Ctrl Pts',(-6.0001362455576,9.90561889763326,1.38087400297164));
#37690=CARTESIAN_POINT('Ctrl Pts',(-6.00013967180241,9.8895273924494,1.39896623194891));
#37691=CARTESIAN_POINT('Ctrl Pts',(-6.0001239623281,9.8742900370339,1.41717677920137));
#37692=CARTESIAN_POINT('Ctrl Pts',(-6.00011958298751,9.87004230934187,1.42225334555701));
#37693=CARTESIAN_POINT('Ctrl Pts',(-6.00011380591212,9.86586073279952,1.42733890963523));
#37694=CARTESIAN_POINT('Ctrl Pts',(-6.0001067056879,9.86174612648125,1.43243017907439));
#37695=CARTESIAN_POINT('Ctrl Pts',(-6.00010098822784,9.85843283713094,1.4365299270229));
#37696=CARTESIAN_POINT('Ctrl Pts',(-6.00009441688859,9.85516296794322,1.44063337206656));
#37697=CARTESIAN_POINT('Ctrl Pts',(-6.00008719772681,9.85193679562792,1.44473884265702));
#37698=CARTESIAN_POINT('Ctrl Pts',(-6.00006865390159,9.84364974272975,1.45528454469337));
#37699=CARTESIAN_POINT('Ctrl Pts',(-6.00005102576008,9.83553345028822,1.46598520939338));
#37700=CARTESIAN_POINT('Ctrl Pts',(-6.00003057015005,9.82773268116427,1.47665723439913));
#37701=CARTESIAN_POINT('Ctrl Pts',(-6.00000992968066,9.81986141572172,1.48742570354556));
#37702=CARTESIAN_POINT('Ctrl Pts',(-5.99998595813747,9.81231176741329,1.49816463309059));
#37703=CARTESIAN_POINT('Ctrl Pts',(-5.99996791547376,9.80519759071623,1.50864643475104));
#37704=CARTESIAN_POINT('Ctrl Pts',(-5.99995722328368,9.80098168719531,1.51485801290091));
#37705=CARTESIAN_POINT('Ctrl Pts',(-5.99994890968004,9.79691800437195,1.52097856799308));
#37706=CARTESIAN_POINT('Ctrl Pts',(-5.99994782973511,9.7930240862629,1.5269554953353));
#37707=CARTESIAN_POINT('Ctrl Pts',(-5.99994380484361,9.77851168159836,1.54923115337734));
#37708=CARTESIAN_POINT('Ctrl Pts',(-5.99996594985734,9.76478866904984,1.57206820321156));
#37709=CARTESIAN_POINT('Ctrl Pts',(-5.9999936985603,9.75201300643072,1.59536297341009));
#37710=CARTESIAN_POINT('Ctrl Pts',(-6.00002003739057,9.73988645731992,1.61747416899025));
#37711=CARTESIAN_POINT('Ctrl Pts',(-6.00005067895151,9.72861404445652,1.63999684562807));
#37712=CARTESIAN_POINT('Ctrl Pts',(-6.00007008721526,9.71830125813383,1.66279885804127));
#37713=CARTESIAN_POINT('Ctrl Pts',(-6.00007112610654,9.71774923225662,1.66401941090746));
#37714=CARTESIAN_POINT('Ctrl Pts',(-6.00007213476147,9.7171999474611,1.66524075529511));
#37715=CARTESIAN_POINT('Ctrl Pts',(-6.00007311154295,9.7166534169473,1.66646286803396));
#37716=CARTESIAN_POINT('Ctrl Pts',(-6.00009137615566,9.70643396830422,1.68931487364968));
#37717=CARTESIAN_POINT('Ctrl Pts',(-6.0000974466336,9.6971810033845,1.71243799002433));
#37718=CARTESIAN_POINT('Ctrl Pts',(-6.0000894323575,9.68895805489599,1.73566955548174));
#37719=CARTESIAN_POINT('Ctrl Pts',(-6.00008131870306,9.68063314048201,1.75918919620504));
#37720=CARTESIAN_POINT('Ctrl Pts',(-6.00005836465151,9.67336426344868,1.78281898369511));
#37721=CARTESIAN_POINT('Ctrl Pts',(-6.00003565609075,9.66717105559036,1.80636853253183));
#37722=CARTESIAN_POINT('Ctrl Pts',(-6.00001753957099,9.66223021527243,1.82515597888002));
#37723=CARTESIAN_POINT('Ctrl Pts',(-5.99999991840194,9.65797302840061,1.84389173683365));
#37724=CARTESIAN_POINT('Ctrl Pts',(-5.99999992132011,9.65438781893335,1.86247612807742));
#37725=CARTESIAN_POINT('Ctrl Pts',(-5.72001867922509,9.72697756830105,2.05943270378453));
#37726=CARTESIAN_POINT('Ctrl Pts',(-5.77263456937867,9.71166938421254,2.03449628829274));
#37727=CARTESIAN_POINT('Ctrl Pts',(-5.82217073193389,9.69806595346106,2.00534896070888));
#37728=CARTESIAN_POINT('Ctrl Pts',(-5.86880003058777,9.68600232454907,1.97245371766885));
#37729=CARTESIAN_POINT('Ctrl Pts',(-5.91542932735784,9.67393869612445,1.93955847595777));
#37730=CARTESIAN_POINT('Ctrl Pts',(-5.95915199503842,9.66341542696136,1.90291542432145));
#37731=CARTESIAN_POINT('Ctrl Pts',(-6.00000008250642,9.65438822329311,1.86247621077463));
#37732=CARTESIAN_POINT('Ctrl Pts',(-5.73278520175299,10.3449555119164,1.71288400365943));
#37733=CARTESIAN_POINT('Ctrl Pts',(-5.74762625823566,10.3336655306276,1.70321684759683));
#37734=CARTESIAN_POINT('Ctrl Pts',(-5.76162670497642,10.3229263377101,1.69298708845874));
#37735=CARTESIAN_POINT('Ctrl Pts',(-5.77478485377481,10.3127313231399,1.68242386558445));
#37736=CARTESIAN_POINT('Ctrl Pts',(-5.78881554118989,10.3018602602861,1.67116017792474));
#37737=CARTESIAN_POINT('Ctrl Pts',(-5.80188866776032,10.2916079863685,1.65951704513893));
#37738=CARTESIAN_POINT('Ctrl Pts',(-5.81403019712682,10.2819593872248,1.64772073960543));
#37739=CARTESIAN_POINT('Ctrl Pts',(-5.81727069665296,10.2793842354454,1.64457237819743));
#37740=CARTESIAN_POINT('Ctrl Pts',(-5.82044497488178,10.2768520458908,1.64141285163079));
#37741=CARTESIAN_POINT('Ctrl Pts',(-5.8235538117211,10.2743624479256,1.63824593592917));
#37742=CARTESIAN_POINT('Ctrl Pts',(-5.83603217451932,10.2643696087266,1.62553445407319));
#37743=CARTESIAN_POINT('Ctrl Pts',(-5.84745523384838,10.2550631298136,1.61270887825643));
#37744=CARTESIAN_POINT('Ctrl Pts',(-5.85790547528079,10.2464057644275,1.60000846413517));
#37745=CARTESIAN_POINT('Ctrl Pts',(-5.8687730380341,10.2374026746692,1.5868008699998));
#37746=CARTESIAN_POINT('Ctrl Pts',(-5.8785888944447,10.2291015910019,1.57372786952288));
#37747=CARTESIAN_POINT('Ctrl Pts',(-5.88745826772452,10.2214578451449,1.56099705001076));
#37748=CARTESIAN_POINT('Ctrl Pts',(-5.89162954745436,10.2178629798543,1.55500972625071));
#37749=CARTESIAN_POINT('Ctrl Pts',(-5.89559162955099,10.2144134683544,1.54909729291484));
#37750=CARTESIAN_POINT('Ctrl Pts',(-5.89935609598258,10.2111044910471,1.54327753594125));
#37751=CARTESIAN_POINT('Ctrl Pts',(-5.90168366366344,10.2090585520603,1.53967918316314));
#37752=CARTESIAN_POINT('Ctrl Pts',(-5.90393569087849,10.207066336566,1.53611621550207));
#37753=CARTESIAN_POINT('Ctrl Pts',(-5.90611496859368,10.2051266893969,1.53259243533064));
#37754=CARTESIAN_POINT('Ctrl Pts',(-5.90944521028314,10.2021626367566,1.52720760550852));
#37755=CARTESIAN_POINT('Ctrl Pts',(-5.91260559262295,10.1993213304078,1.52191438606531));
#37756=CARTESIAN_POINT('Ctrl Pts',(-5.91560707709282,10.1965982311228,1.5167261658696));
#37757=CARTESIAN_POINT('Ctrl Pts',(-5.91808989042462,10.1943456966597,1.51243449539801));
#37758=CARTESIAN_POINT('Ctrl Pts',(-5.92046390928247,10.1921740784455,1.50821473564372));
#37759=CARTESIAN_POINT('Ctrl Pts',(-5.92273528386489,10.1900808352025,1.50407344253474));
#37760=CARTESIAN_POINT('Ctrl Pts',(-5.9238709711561,10.189034213581,1.50200279598024));
#37761=CARTESIAN_POINT('Ctrl Pts',(-5.92498099014943,10.1880071875312,1.4999517613849));
#37762=CARTESIAN_POINT('Ctrl Pts',(-5.9260660878658,10.1869994516525,1.49792110336238));
#37763=CARTESIAN_POINT('Ctrl Pts',(-5.92682745232362,10.1862923685305,1.49649628159654));
#37764=CARTESIAN_POINT('Ctrl Pts',(-5.92726381086926,10.1858856593911,1.4956732784651));
#37765=CARTESIAN_POINT('Ctrl Pts',(-5.92803487321876,10.1851664614614,1.49420743045771));
#37766=CARTESIAN_POINT('Ctrl Pts',(-5.92836273003475,10.1848606574711,1.49358414978433));
#37767=CARTESIAN_POINT('Ctrl Pts',(-5.92875078441314,10.1844984854958,1.49284443006148));
#37768=CARTESIAN_POINT('Ctrl Pts',(-5.92924734435405,10.184033813251,1.49189099663322));
#37769=CARTESIAN_POINT('Ctrl Pts',(-5.93919300113636,10.1747268388407,1.47279456766051));
#37770=CARTESIAN_POINT('Ctrl Pts',(-5.94793107627244,10.1661803928757,1.45367212129977));
#37771=CARTESIAN_POINT('Ctrl Pts',(-5.95553872313124,10.1583598358875,1.4347373834926));
#37772=CARTESIAN_POINT('Ctrl Pts',(-5.9586318177942,10.1551801768509,1.42703895353879));
#37773=CARTESIAN_POINT('Ctrl Pts',(-5.96153809959893,10.1521204767886,1.41937092680088));
#37774=CARTESIAN_POINT('Ctrl Pts',(-5.9642630307132,10.1491782414327,1.4117452974802));
#37775=CARTESIAN_POINT('Ctrl Pts',(-5.9710901981722,10.1418066299549,1.39263969584501));
#37776=CARTESIAN_POINT('Ctrl Pts',(-5.97677989684862,10.135172123484,1.37380405250111));
#37777=CARTESIAN_POINT('Ctrl Pts',(-5.98146315896994,10.1292176627262,1.35542195960802));
#37778=CARTESIAN_POINT('Ctrl Pts',(-5.98644690166057,10.1228811606237,1.33586046193365));
#37779=CARTESIAN_POINT('Ctrl Pts',(-5.99029046394656,10.1173148938422,1.31681231134461));
#37780=CARTESIAN_POINT('Ctrl Pts',(-5.99314482070217,10.1124514917611,1.29844067055225));
#37781=CARTESIAN_POINT('Ctrl Pts',(-5.99383961718569,10.1112676612335,1.29396871679453));
#37782=CARTESIAN_POINT('Ctrl Pts',(-5.99447578939983,10.1101254778785,1.28953660287938));
#37783=CARTESIAN_POINT('Ctrl Pts',(-5.99505550273689,10.1090239704676,1.28514623077354));
#37784=CARTESIAN_POINT('Ctrl Pts',(-5.99754124290847,10.10430084087,1.2663208499966));
#37785=CARTESIAN_POINT('Ctrl Pts',(-5.99899094609771,10.1003248617228,1.24826680445821));
#37786=CARTESIAN_POINT('Ctrl Pts',(-5.99961818135814,10.0970053748056,1.23110680412698));
#37787=CARTESIAN_POINT('Ctrl Pts',(-5.99986797371164,10.0956834107806,1.22427294586166));
#37788=CARTESIAN_POINT('Ctrl Pts',(-5.99998707059434,10.0944656568097,1.21758034077405));
#37789=CARTESIAN_POINT('Ctrl Pts',(-5.99998809173028,10.0933467245957,1.21103470346248));
#37790=CARTESIAN_POINT('Ctrl Pts',(-5.72202398775916,19.8960805169565,0.386352176427263));
#37791=CARTESIAN_POINT('Ctrl Pts',(-5.722744923188,19.5069870025453,0.666957542712061));
#37792=CARTESIAN_POINT('Ctrl Pts',(-5.72404047055462,18.65358895384,1.1961917425212));
#37793=CARTESIAN_POINT('Ctrl Pts',(-5.72530463330588,17.252880723512,1.80439897490435));
#37794=CARTESIAN_POINT('Ctrl Pts',(-5.72546454574842,15.7365645039447,2.20426079914038));
#37795=CARTESIAN_POINT('Ctrl Pts',(-5.72471278438522,14.1774183292184,2.3706007618924));
#37796=CARTESIAN_POINT('Ctrl Pts',(-5.72306497930087,12.6107761111604,2.29992939792902));
#37797=CARTESIAN_POINT('Ctrl Pts',(-5.72038826693908,11.1578231494624,2.009761590955));
#37798=CARTESIAN_POINT('Ctrl Pts',(-5.71829665675548,10.2528020998913,1.69379809858199));
#37799=CARTESIAN_POINT('Ctrl Pts',(-5.71724106961605,9.85241023628882,1.52490686972533));
#37800=CARTESIAN_POINT('Ctrl Pts',(-5.90002815788726,19.8627034270208,0.340121769673507));
#37801=CARTESIAN_POINT('Ctrl Pts',(-5.90064112502721,19.4755717271918,0.618895098936227));
#37802=CARTESIAN_POINT('Ctrl Pts',(-5.90174136243637,18.6265869130023,1.14467025662982));
#37803=CARTESIAN_POINT('Ctrl Pts',(-5.90281091502772,17.233624563546,1.74886350102612));
#37804=CARTESIAN_POINT('Ctrl Pts',(-5.90294617326952,15.7258951691654,2.14638243188552));
#37805=CARTESIAN_POINT('Ctrl Pts',(-5.90231020081427,14.1756917163178,2.31212465550085));
#37806=CARTESIAN_POINT('Ctrl Pts',(-5.90091450222212,12.6178122340193,2.24263139230537));
#37807=CARTESIAN_POINT('Ctrl Pts',(-5.89863680636618,11.1726809459824,1.9553149115722));
#37808=CARTESIAN_POINT('Ctrl Pts',(-5.89685246807884,10.2721886785122,1.64197819775049));
#37809=CARTESIAN_POINT('Ctrl Pts',(-5.89594599918652,9.87374136647885,1.47444506422475));
#37810=CARTESIAN_POINT('Ctrl Pts',(-6.00728101833992,19.7730197694138,0.215901419477209));
#37811=CARTESIAN_POINT('Ctrl Pts',(-6.00760398018924,19.3915708450173,0.490321734932853));
#37812=CARTESIAN_POINT('Ctrl Pts',(-6.00818204236773,18.5550176863609,1.00794402616504));
#37813=CARTESIAN_POINT('Ctrl Pts',(-6.00873885820584,17.1829706228646,1.6026646162929));
#37814=CARTESIAN_POINT('Ctrl Pts',(-6.00880922773446,15.6978212924223,1.99418148817968));
#37815=CARTESIAN_POINT('Ctrl Pts',(-6.00847821278282,14.1710746182912,2.15763405987662));
#37816=CARTESIAN_POINT('Ctrl Pts',(-6.00774960894449,12.6364830352444,2.0896700063425));
#37817=CARTESIAN_POINT('Ctrl Pts',(-6.00654717924463,11.2128937590667,1.80743882631002));
#37818=CARTESIAN_POINT('Ctrl Pts',(-6.00559946168958,10.3255097743763,1.49932376623001));
#37819=CARTESIAN_POINT('Ctrl Pts',(-6.00511047283608,9.93286787454664,1.33457276173998));
#37820=CARTESIAN_POINT('Ctrl Pts',(-5.99966790103542,19.6635731258448,0.0643074436082086));
#37821=CARTESIAN_POINT('Ctrl Pts',(-5.99963698975156,19.2892128226794,0.333628132544527));
#37822=CARTESIAN_POINT('Ctrl Pts',(-5.99957878613466,18.4680448255696,0.841727065914757));
#37823=CARTESIAN_POINT('Ctrl Pts',(-5.99951367581519,17.1215601727196,1.42537763535855));
#37824=CARTESIAN_POINT('Ctrl Pts',(-5.99950536396078,15.66378285343,1.80967927954129));
#37825=CARTESIAN_POINT('Ctrl Pts',(-5.99954420660795,14.1654483981742,1.97008249641598));
#37826=CARTESIAN_POINT('Ctrl Pts',(-5.99962585188073,12.6591804244486,1.90337383375695));
#37827=CARTESIAN_POINT('Ctrl Pts',(-5.99973680056724,11.2620763145782,1.62638694967239));
#37828=CARTESIAN_POINT('Ctrl Pts',(-5.99981416523958,10.3910398983604,1.32395870088371));
#37829=CARTESIAN_POINT('Ctrl Pts',(-5.99984092544071,10.0056993730018,1.16227925631749));
#37830=CARTESIAN_POINT('',(-5.99999988467789,19.5919337295688,0.13548398932811));
#37831=CARTESIAN_POINT('Origin',(-5.59998164335335,19.5919273324291,0.135474139597038));
#37832=CARTESIAN_POINT('Ctrl Pts',(-6.,19.5919320859607,0.135483413470245));
#37833=CARTESIAN_POINT('Ctrl Pts',(-6.,19.2032417293653,0.410171473275152));
#37834=CARTESIAN_POINT('Ctrl Pts',(-6.,18.7991432375947,0.654503356286178));
#37835=CARTESIAN_POINT('Ctrl Pts',(-6.,18.3770565530435,0.869913230869506));
#37836=CARTESIAN_POINT('Ctrl Pts',(-6.,17.9549695699687,1.08532325780287));
#37837=CARTESIAN_POINT('Ctrl Pts',(-6.,17.5148943686686,1.27181123539797));
#37838=CARTESIAN_POINT('Ctrl Pts',(-6.,17.0647735964723,1.42538956888279));
#37839=CARTESIAN_POINT('Ctrl Pts',(-6.,16.6146528242763,1.5789679023675));
#37840=CARTESIAN_POINT('Ctrl Pts',(-6.,16.1544864811841,1.69963659174199));
#37841=CARTESIAN_POINT('Ctrl Pts',(-6.,15.6870767766761,1.78685625005223));
#37842=CARTESIAN_POINT('Ctrl Pts',(-6.,15.2196670721679,1.87407590836254));
#37843=CARTESIAN_POINT('Ctrl Pts',(-6.,14.7450140062439,1.92784653560856));
#37844=CARTESIAN_POINT('Ctrl Pts',(-6.,14.2698875448941,1.94742220490056));
#37845=CARTESIAN_POINT('Ctrl Pts',(-6.,13.7947610835446,1.96699787419255));
#37846=CARTESIAN_POINT('Ctrl Pts',(-6.,13.3191612267692,1.95237858553056));
#37847=CARTESIAN_POINT('Ctrl Pts',(-6.,12.8461741667461,1.90343073178653));
#37848=CARTESIAN_POINT('Ctrl Pts',(-6.,12.3731871067227,1.85448287804245));
#37849=CARTESIAN_POINT('Ctrl Pts',(-6.,11.9028128434515,1.77120645921628));
#37850=CARTESIAN_POINT('Ctrl Pts',(-6.,11.4430952551193,1.65563717376403));
#37851=CARTESIAN_POINT('Ctrl Pts',(-6.,10.9833776667874,1.54006788831187));
#37852=CARTESIAN_POINT('Ctrl Pts',(-6.,10.5343167533944,1.39220573623369));
#37853=CARTESIAN_POINT('Ctrl Pts',(-6.,10.0933467247176,1.21103470471191));
#37854=CARTESIAN_POINT('Origin',(-5.599999999997,19.5919343769627,0.135488060674723));
#37855=CARTESIAN_POINT('Origin',(-5.6,19.5919343770088,0.135488060674804));
#37856=CARTESIAN_POINT('Ctrl Pts',(-6.05070961963225,10.3130249361011,-1.22535725240516));
#37857=CARTESIAN_POINT('Ctrl Pts',(-6.05140667375169,10.3096023136128,-1.25170873298356));
#37858=CARTESIAN_POINT('Ctrl Pts',(-6.04732759893246,10.3030271880175,-1.31927088995749));
#37859=CARTESIAN_POINT('Ctrl Pts',(-6.01624876430349,10.3009968959657,-1.43148297695375));
#37860=CARTESIAN_POINT('Ctrl Pts',(-5.94855854570417,10.3111324909314,-1.55166467988863));
#37861=CARTESIAN_POINT('Ctrl Pts',(-5.85056713415748,10.3339919100581,-1.65505066142282));
#37862=CARTESIAN_POINT('Ctrl Pts',(-5.76530747145516,10.3582031816919,-1.70808535345447));
#37863=CARTESIAN_POINT('Ctrl Pts',(-5.71754885550636,10.3728653836147,-1.72862512790978));
#37864=CARTESIAN_POINT('Ctrl Pts',(-5.7120304436856,10.3745733921892,-1.73088351326345));
#37865=CARTESIAN_POINT('Ctrl Pts',(-5.9119799714366,10.0313345995451,-1.19275674695457));
#37866=CARTESIAN_POINT('Ctrl Pts',(-5.91261995497024,10.0282455529599,-1.21646968247228));
#37867=CARTESIAN_POINT('Ctrl Pts',(-5.90887926223061,10.0223509287081,-1.27752158060179));
#37868=CARTESIAN_POINT('Ctrl Pts',(-5.8800717142639,10.0208498082042,-1.37978014786759));
#37869=CARTESIAN_POINT('Ctrl Pts',(-5.81696369720526,10.0308230995347,-1.48996890572508));
#37870=CARTESIAN_POINT('Ctrl Pts',(-5.72538322198305,10.0527061528258,-1.58504538083284));
#37871=CARTESIAN_POINT('Ctrl Pts',(-5.64570293957858,10.0756193202956,-1.63384573406177));
#37872=CARTESIAN_POINT('Ctrl Pts',(-5.60112974557925,10.0894115585813,-1.65273765411278));
#37873=CARTESIAN_POINT('Ctrl Pts',(-5.59598027839829,10.0910171857285,-1.65481477844338));
#37874=CARTESIAN_POINT('Ctrl Pts',(-6.0285097850003,9.74077481927242,-1.1520775934791));
#37875=CARTESIAN_POINT('Ctrl Pts',(-6.02951335972276,9.73603300079858,-1.18863580640333));
#37876=CARTESIAN_POINT('Ctrl Pts',(-6.0236073757172,9.72706141057504,-1.28086318017417));
#37877=CARTESIAN_POINT('Ctrl Pts',(-5.98091755192499,9.72423946816267,-1.42906490732787));
#37878=CARTESIAN_POINT('Ctrl Pts',(-5.89068175080473,9.73709969987668,-1.58417525760424));
#37879=CARTESIAN_POINT('Ctrl Pts',(-5.76172577093106,9.766268391079,-1.71641116692069));
#37880=CARTESIAN_POINT('Ctrl Pts',(-5.64951415628754,9.79753689869301,-1.78453321317423));
#37881=CARTESIAN_POINT('Ctrl Pts',(-5.586206150674,9.81673862473118,-1.81113948056136));
#37882=CARTESIAN_POINT('Ctrl Pts',(-5.57888445210631,9.81897897780365,-1.81406848190426));
#37883=CARTESIAN_POINT('Ctrl Pts',(-6.32394327601718,9.63173326085878,-1.12997458657446));
#37884=CARTESIAN_POINT('Ctrl Pts',(-6.32549286216374,9.62443529434766,-1.18644508677191));
#37885=CARTESIAN_POINT('Ctrl Pts',(-6.31633671118906,9.61064543956799,-1.32710607464008));
#37886=CARTESIAN_POINT('Ctrl Pts',(-6.25270734978457,9.6055181449323,-1.54704358343089));
#37887=CARTESIAN_POINT('Ctrl Pts',(-6.12140914137511,9.62242290629162,-1.77255538315458));
#37888=CARTESIAN_POINT('Ctrl Pts',(-5.93578135264523,9.66236535691839,-1.96307110762315));
#37889=CARTESIAN_POINT('Ctrl Pts',(-5.7742437071044,9.70616784886645,-2.0614104224421));
#37890=CARTESIAN_POINT('Ctrl Pts',(-5.68255656006243,9.73351397080183,-2.10003844602719));
#37891=CARTESIAN_POINT('Ctrl Pts',(-5.67194479924022,9.73671025575887,-2.10429427367507));
#37892=CARTESIAN_POINT('',(-5.7327877343283,10.3449530459579,-1.71289077335416));
#37893=CARTESIAN_POINT('',(-5.72001814737754,9.72697621226736,-2.05943242421435));
#37894=CARTESIAN_POINT('Origin',(-5.8987601709971,10.1837992950051,-2.15614229677139));
#37895=CARTESIAN_POINT('',(-5.9999999968135,9.65438801435697,-1.86247622312975));
#37896=CARTESIAN_POINT('Ctrl Pts',(-6.00000008328868,9.65438821225989,-1.86247626630162));
#37897=CARTESIAN_POINT('Ctrl Pts',(-5.95915137667818,9.66341555272123,-1.90291609182812));
#37898=CARTESIAN_POINT('Ctrl Pts',(-5.91542827656402,9.67393895342414,-1.9395593190579));
#37899=CARTESIAN_POINT('Ctrl Pts',(-5.86879893709647,9.6860026085962,-1.97245448346289));
#37900=CARTESIAN_POINT('Ctrl Pts',(-5.82216959562333,9.69806626428713,-2.00534964928275));
#37901=CARTESIAN_POINT('Ctrl Pts',(-5.77263377986791,9.71166961723077,-2.03449664691797));
#37902=CARTESIAN_POINT('Ctrl Pts',(-5.72001867761226,9.72697756737453,-2.0594327111465));
#37903=CARTESIAN_POINT('',(-5.99998808311063,10.09334672158,-1.2110347210661));
#37904=CARTESIAN_POINT('Ctrl Pts',(-5.99998808311063,10.09334672158,-1.2110347210661));
#37905=CARTESIAN_POINT('Ctrl Pts',(-5.99998579341327,10.0709268555555,-1.2281327269299));
#37906=CARTESIAN_POINT('Ctrl Pts',(-5.99998684305411,10.0492796321252,-1.24555661530825));
#37907=CARTESIAN_POINT('Ctrl Pts',(-5.99998299250915,10.0284346981922,-1.26332163857805));
#37908=CARTESIAN_POINT('Ctrl Pts',(-5.9999818636268,10.0223234910084,-1.26852989388725));
#37909=CARTESIAN_POINT('Ctrl Pts',(-5.99998012528455,10.0162810465041,-1.27376722624289));
#37910=CARTESIAN_POINT('Ctrl Pts',(-5.99997728635832,10.0103076348659,-1.27903349119982));
#37911=CARTESIAN_POINT('Ctrl Pts',(-5.99996366417836,9.98164507665961,-1.3043029075739));
#37912=CARTESIAN_POINT('Ctrl Pts',(-5.99992845500907,9.9545755699725,-1.33023848659307));
#37913=CARTESIAN_POINT('Ctrl Pts',(-5.99991579265607,9.92904827997819,-1.3568311348157));
#37914=CARTESIAN_POINT('Ctrl Pts',(-5.99991509569424,9.92764320568267,-1.35829484860889));
#37915=CARTESIAN_POINT('Ctrl Pts',(-5.99991446145114,9.92624279434832,-1.35976055702209));
#37916=CARTESIAN_POINT('Ctrl Pts',(-5.99991389619172,9.92484703487078,-1.36122826085182));
#37917=CARTESIAN_POINT('Ctrl Pts',(-5.99990496302787,9.90278893600095,-1.38442334332033));
#37918=CARTESIAN_POINT('Ctrl Pts',(-5.99990285601733,9.88191510379151,-1.40812762073311));
#37919=CARTESIAN_POINT('Ctrl Pts',(-5.9999038676287,9.86223177764951,-1.43232863089542));
#37920=CARTESIAN_POINT('Ctrl Pts',(-5.99990457803031,9.84840921017725,-1.44932373088269));
#37921=CARTESIAN_POINT('Ctrl Pts',(-5.99990726918065,9.83517314684603,-1.46656412244876));
#37922=CARTESIAN_POINT('Ctrl Pts',(-5.99991518239819,9.82252477117456,-1.48405885957351));
#37923=CARTESIAN_POINT('Ctrl Pts',(-5.99991811455196,9.81783805781404,-1.49054133766801));
#37924=CARTESIAN_POINT('Ctrl Pts',(-5.99992620313177,9.81307118484453,-1.49727692070492));
#37925=CARTESIAN_POINT('Ctrl Pts',(-5.99993158586974,9.80845147725634,-1.50397097353427));
#37926=CARTESIAN_POINT('Ctrl Pts',(-5.9999370371547,9.80377293957075,-1.51075027240407));
#37927=CARTESIAN_POINT('Ctrl Pts',(-5.9999394402226,9.79924553862276,-1.5174867094576));
#37928=CARTESIAN_POINT('Ctrl Pts',(-5.99994448128701,9.79506976773256,-1.52383523346148));
#37929=CARTESIAN_POINT('Ctrl Pts',(-5.99994531690624,9.79437758167727,-1.52488758041793));
#37930=CARTESIAN_POINT('Ctrl Pts',(-5.99994625961908,9.79369497785949,-1.52592919076002));
#37931=CARTESIAN_POINT('Ctrl Pts',(-5.99994737646189,9.79302277710163,-1.526958405299));
#37932=CARTESIAN_POINT('Ctrl Pts',(-5.99997425283644,9.77684653535922,-1.55172604055182));
#37933=CARTESIAN_POINT('Ctrl Pts',(-5.99996042293814,9.76199838214035,-1.57679063138343));
#37934=CARTESIAN_POINT('Ctrl Pts',(-5.99993587672946,9.74841240942493,-1.60210525746293));
#37935=CARTESIAN_POINT('Ctrl Pts',(-5.99991530960845,9.73702880437642,-1.62331623081582));
#37936=CARTESIAN_POINT('Ctrl Pts',(-5.99988812722501,9.72653125073023,-1.6447038648777));
#37937=CARTESIAN_POINT('Ctrl Pts',(-5.9998711787835,9.71689962998366,-1.66626214470264));
#37938=CARTESIAN_POINT('Ctrl Pts',(-5.99985203331414,9.70601946145499,-1.69061502609774));
#37939=CARTESIAN_POINT('Ctrl Pts',(-5.99984751258481,9.69624316928748,-1.71518651254818));
#37940=CARTESIAN_POINT('Ctrl Pts',(-5.99986529071402,9.68757637932992,-1.73999079081509));
#37941=CARTESIAN_POINT('Ctrl Pts',(-5.99988251401862,9.67918006487467,-1.76402097052225));
#37942=CARTESIAN_POINT('Ctrl Pts',(-5.99992124830363,9.67182546041951,-1.78827070432582));
#37943=CARTESIAN_POINT('Ctrl Pts',(-5.99995587878963,9.66555347191789,-1.81275252917949));
#37944=CARTESIAN_POINT('Ctrl Pts',(-5.99997917551999,9.66133415992386,-1.82922202002983));
#37945=CARTESIAN_POINT('Ctrl Pts',(-5.99999991524883,9.65760556987688,-1.84579651491695));
#37946=CARTESIAN_POINT('Ctrl Pts',(-5.99999992273905,9.65438780859768,-1.86247618343571));
#37947=CARTESIAN_POINT('Ctrl Pts',(-5.99998808311063,10.09334672158,-1.2110347210661));
#37948=CARTESIAN_POINT('Ctrl Pts',(-5.99998551891589,10.0961555650809,-1.22746603445882));
#37949=CARTESIAN_POINT('Ctrl Pts',(-5.99924019502052,10.0995867364503,-1.24482748142736));
#37950=CARTESIAN_POINT('Ctrl Pts',(-5.99754681056573,10.1037278134695,-1.26301505141432));
#37951=CARTESIAN_POINT('Ctrl Pts',(-5.99687196657425,10.105378106725,-1.2702631233394));
#37952=CARTESIAN_POINT('Ctrl Pts',(-5.99604634751327,10.1071412272894,-1.27764189205116));
#37953=CARTESIAN_POINT('Ctrl Pts',(-5.99505598209408,10.1090230777761,-1.28514264891433));
#37954=CARTESIAN_POINT('Ctrl Pts',(-5.99264929788291,10.113596157335,-1.30337021700654));
#37955=CARTESIAN_POINT('Ctrl Pts',(-5.98926946606121,10.1188704998751,-1.32232184177371));
#37956=CARTESIAN_POINT('Ctrl Pts',(-5.98476114210219,10.1249156580807,-1.34184178461827));
#37957=CARTESIAN_POINT('Ctrl Pts',(-5.98055933808551,10.1305498073257,-1.36003457089437));
#37958=CARTESIAN_POINT('Ctrl Pts',(-5.97537764155951,10.1368533912459,-1.37872127166542));
#37959=CARTESIAN_POINT('Ctrl Pts',(-5.96908599007236,10.1438834564595,-1.39772962282572));
#37960=CARTESIAN_POINT('Ctrl Pts',(-5.96754611917192,10.1456040528518,-1.40238188414008));
#37961=CARTESIAN_POINT('Ctrl Pts',(-5.96593972334642,10.1473681747883,-1.40705317486269));
#37962=CARTESIAN_POINT('Ctrl Pts',(-5.96426481079894,10.1491766784785,-1.41174048388465));
#37963=CARTESIAN_POINT('Ctrl Pts',(-5.96381007634479,10.1496676825847,-1.41301307624343));
#37964=CARTESIAN_POINT('Ctrl Pts',(-5.96335029118388,10.1501619581831,-1.41428684812407));
#37965=CARTESIAN_POINT('Ctrl Pts',(-5.96288542949712,10.1506595170982,-1.41556174614242));
#37966=CARTESIAN_POINT('Ctrl Pts',(-5.95829898371322,10.1555685622044,-1.42814022014359));
#37967=CARTESIAN_POINT('Ctrl Pts',(-5.95321825935307,10.1607972808259,-1.44082909355127));
#37968=CARTESIAN_POINT('Ctrl Pts',(-5.94761928777537,10.1663565694259,-1.45357194238132));
#37969=CARTESIAN_POINT('Ctrl Pts',(-5.94481980198652,10.1691362137259,-1.45994336679635));
#37970=CARTESIAN_POINT('Ctrl Pts',(-5.94189071237444,10.1719985095046,-1.46632826213982));
#37971=CARTESIAN_POINT('Ctrl Pts',(-5.93882920319315,10.1749447294529,-1.47271846796723));
#37972=CARTESIAN_POINT('Ctrl Pts',(-5.93729844860251,10.1764178394271,-1.47591357088094));
#37973=CARTESIAN_POINT('Ctrl Pts',(-5.93573458582514,10.1779119311141,-1.47910999970802));
#37974=CARTESIAN_POINT('Ctrl Pts',(-5.93413725899299,10.1794271634867,-1.48230668713107));
#37975=CARTESIAN_POINT('Ctrl Pts',(-5.93307814973919,10.1804318399219,-1.48442625412459));
#37976=CARTESIAN_POINT('Ctrl Pts',(-5.93173234065811,10.181702758603,-1.48708001239351));
#37977=CARTESIAN_POINT('Ctrl Pts',(-5.9306387932707,10.1827296550799,-1.48920401045017));
#37978=CARTESIAN_POINT('Ctrl Pts',(-5.93008307493992,10.1832515027864,-1.49028338265501));
#37979=CARTESIAN_POINT('Ctrl Pts',(-5.92959342275462,10.1837099577805,-1.49122653267897));
#37980=CARTESIAN_POINT('Ctrl Pts',(-5.92924452264283,10.1840364429654,-1.49189642960275));
#37981=CARTESIAN_POINT('Ctrl Pts',(-5.92334534744649,10.1895566283702,-1.50322299323332));
#37982=CARTESIAN_POINT('Ctrl Pts',(-5.9166616455774,10.1956931332343,-1.51523970801863));
#37983=CARTESIAN_POINT('Ctrl Pts',(-5.90905335711028,10.2025037329907,-1.52779298919207));
#37984=CARTESIAN_POINT('Ctrl Pts',(-5.90809035048613,10.2033657734757,-1.52938190015112));
#37985=CARTESIAN_POINT('Ctrl Pts',(-5.90711252019561,10.2042386187167,-1.53097933947511));
#37986=CARTESIAN_POINT('Ctrl Pts',(-5.90611957305421,10.2051223903042,-1.53258493413081));
#37987=CARTESIAN_POINT('Ctrl Pts',(-5.8985559999358,10.211854340821,-1.54481522522138));
#37988=CARTESIAN_POINT('Ctrl Pts',(-5.8901147942091,10.2192204202246,-1.55752239042882));
#37989=CARTESIAN_POINT('Ctrl Pts',(-5.88068120099843,10.2272683777287,-1.57053114009695));
#37990=CARTESIAN_POINT('Ctrl Pts',(-5.87365871205742,10.2332593815072,-1.58021502179936));
#37991=CARTESIAN_POINT('Ctrl Pts',(-5.86608634065068,10.2396282268125,-1.59006530425002));
#37992=CARTESIAN_POINT('Ctrl Pts',(-5.85791987654171,10.2463937661191,-1.5999909644792));
#37993=CARTESIAN_POINT('Ctrl Pts',(-5.8474691036833,10.2550517499925,-1.61269301265337));
#37994=CARTESIAN_POINT('Ctrl Pts',(-5.83604472953277,10.2643594640929,-1.62552103427835));
#37995=CARTESIAN_POINT('Ctrl Pts',(-5.82356408577863,10.2743542334951,-1.63823549129981));
#37996=CARTESIAN_POINT('Ctrl Pts',(-5.81185649569968,10.2837299247976,-1.65016241220356));
#37997=CARTESIAN_POINT('Ctrl Pts',(-5.79921845229279,10.2937105873015,-1.66198843389947));
#37998=CARTESIAN_POINT('Ctrl Pts',(-5.78561687265328,10.3043134922338,-1.67349578870636));
#37999=CARTESIAN_POINT('Ctrl Pts',(-5.77289224946348,10.3142327790781,-1.68426121137857));
#38000=CARTESIAN_POINT('Ctrl Pts',(-5.75932421188658,10.3246966185417,-1.69474796424745));
#38001=CARTESIAN_POINT('Ctrl Pts',(-5.74490757706917,10.3357133209617,-1.70473747444832));
#38002=CARTESIAN_POINT('Ctrl Pts',(-5.74093112655276,10.3387519893183,-1.70749281877799));
#38003=CARTESIAN_POINT('Ctrl Pts',(-5.73689025758254,10.341832684617,-1.71021007228805));
#38004=CARTESIAN_POINT('Ctrl Pts',(-5.73278520328664,10.3449555024461,-1.7128840178198));
#38005=CARTESIAN_POINT('Ctrl Pts',(-5.71725900098506,9.85240186273889,-1.52489737983018));
#38006=CARTESIAN_POINT('Ctrl Pts',(-5.71831458271734,10.2527966794643,-1.6937903386106));
#38007=CARTESIAN_POINT('Ctrl Pts',(-5.72040617580086,11.1578210792105,-2.00975541592047));
#38008=CARTESIAN_POINT('Ctrl Pts',(-5.72308285296501,12.6107767816378,-2.2999236291718));
#38009=CARTESIAN_POINT('Ctrl Pts',(-5.72473063324945,14.1774181660355,-2.37059488757382));
#38010=CARTESIAN_POINT('Ctrl Pts',(-5.72548238281593,15.7365634246302,-2.20425498075435));
#38011=CARTESIAN_POINT('Ctrl Pts',(-5.72532247293938,17.2528787711321,-1.80439340096888));
#38012=CARTESIAN_POINT('Ctrl Pts',(-5.72405833313342,18.6535823415443,-1.19618825603203));
#38013=CARTESIAN_POINT('Ctrl Pts',(-5.72276281321446,19.5069765306111,-0.666957242692712));
#38014=CARTESIAN_POINT('Ctrl Pts',(-5.72204189664406,19.8960667901931,-0.386355007630499));
#38015=CARTESIAN_POINT('Ctrl Pts',(-5.89595608811401,9.87373568239816,-1.47442937000013));
#38016=CARTESIAN_POINT('Ctrl Pts',(-5.89686253255657,10.2721856611528,-1.64196412804974));
#38017=CARTESIAN_POINT('Ctrl Pts',(-5.89864681126967,11.1726806565925,-1.95530224537703));
#38018=CARTESIAN_POINT('Ctrl Pts',(-5.90092442591395,12.6178137104256,-2.24261899237967));
#38019=CARTESIAN_POINT('Ctrl Pts',(-5.90232007042876,14.1756913526124,-2.3121121385942));
#38020=CARTESIAN_POINT('Ctrl Pts',(-5.90295601817132,15.7258928867575,-2.14637009402302));
#38021=CARTESIAN_POINT('Ctrl Pts',(-5.90282076518485,17.2336204409562,-1.74885165906947));
#38022=CARTESIAN_POINT('Ctrl Pts',(-5.9017512571849,18.6265772369609,-1.14466085934096));
#38023=CARTESIAN_POINT('Ctrl Pts',(-5.90065106834299,19.47555764694,-0.618889185779098));
#38024=CARTESIAN_POINT('Ctrl Pts',(-5.90003813161803,19.8626858446245,-0.340119139048481));
#38025=CARTESIAN_POINT('Ctrl Pts',(-6.00511196337079,9.93286177430145,-1.33455848991861));
#38026=CARTESIAN_POINT('Ctrl Pts',(-6.00560092878501,10.3255063448102,-1.49931113500935));
#38027=CARTESIAN_POINT('Ctrl Pts',(-6.00654858673405,11.2128931137538,-1.80742765761119));
#38028=CARTESIAN_POINT('Ctrl Pts',(-6.00775094556156,12.6364843163732,-2.08965919677582));
#38029=CARTESIAN_POINT('Ctrl Pts',(-6.00847950177932,14.1710743021289,-2.1576231816053));
#38030=CARTESIAN_POINT('Ctrl Pts',(-6.00881049544709,15.697819310256,-1.99417077940699));
#38031=CARTESIAN_POINT('Ctrl Pts',(-6.00874013038259,17.1829670424457,-1.60265433566748));
#38032=CARTESIAN_POINT('Ctrl Pts',(-6.00818335243022,18.5550088225529,-1.00793604053573));
#38033=CARTESIAN_POINT('Ctrl Pts',(-6.00760532996379,19.3915577425242,-0.490317082630804));
#38034=CARTESIAN_POINT('Ctrl Pts',(-6.00728239242838,19.7730032591172,-0.215899947647808));
#38035=CARTESIAN_POINT('Ctrl Pts',(-5.99984082028272,10.0056907570941,-1.16227147505724));
#38036=CARTESIAN_POINT('Ctrl Pts',(-5.99981405141536,10.3910341666072,-1.32395264497647));
#38037=CARTESIAN_POINT('Ctrl Pts',(-5.99973665762545,11.262073897347,-1.62638254338466));
#38038=CARTESIAN_POINT('Ctrl Pts',(-5.99962568511255,12.6591808586663,-1.90336998277106));
#38039=CARTESIAN_POINT('Ctrl Pts',(-5.99954402211993,14.1654482917451,-1.97007863120369));
#38040=CARTESIAN_POINT('Ctrl Pts',(-5.99950517213815,15.6637821447797,-1.80967547346287));
#38041=CARTESIAN_POINT('Ctrl Pts',(-5.99951348544965,17.1215588901583,-1.42537398644992));
#38042=CARTESIAN_POINT('Ctrl Pts',(-5.99957860877151,18.4680392834296,-0.841725262046986));
#38043=CARTESIAN_POINT('Ctrl Pts',(-5.99963682440262,19.2892036755591,-0.333629249611667));
#38044=CARTESIAN_POINT('Ctrl Pts',(-5.99966774289508,19.6635608898064,-0.0643114939931151));
#38045=CARTESIAN_POINT('',(-5.99999997114735,19.5919329044493,-0.135484571570026));
#38046=CARTESIAN_POINT('Ctrl Pts',(-6.,10.0933467217017,-1.2110347223169));
#38047=CARTESIAN_POINT('Ctrl Pts',(-6.,10.534316803576,-1.39220578035687));
#38048=CARTESIAN_POINT('Ctrl Pts',(-6.,10.9833777640737,-1.54006792738036));
#38049=CARTESIAN_POINT('Ctrl Pts',(-6.,11.4430953897292,-1.65563720843317));
#38050=CARTESIAN_POINT('Ctrl Pts',(-6.,11.9028130153849,-1.77120648948607));
#38051=CARTESIAN_POINT('Ctrl Pts',(-6.,12.3731873061984,-1.85448290456825));
#38052=CARTESIAN_POINT('Ctrl Pts',(-6.,12.8461743612776,-1.90343075106931));
#38053=CARTESIAN_POINT('Ctrl Pts',(-6.,13.3191614163566,-1.95237859757033));
#38054=CARTESIAN_POINT('Ctrl Pts',(-6.,13.7947612357013,-1.96699787549028));
#38055=CARTESIAN_POINT('Ctrl Pts',(-6.,14.2698876719687,-1.94742220019824));
#38056=CARTESIAN_POINT('Ctrl Pts',(-6.,14.7450141082364,-1.92784652490618));
#38057=CARTESIAN_POINT('Ctrl Pts',(-6.,15.2196671614267,-1.87407589640209));
#38058=CARTESIAN_POINT('Ctrl Pts',(-6.,15.6870768618399,-1.78685623436044));
#38059=CARTESIAN_POINT('Ctrl Pts',(-6.,16.1544865622528,-1.69963657231885));
#38060=CARTESIAN_POINT('Ctrl Pts',(-6.,16.6146529098885,-1.57896787673975));
#38061=CARTESIAN_POINT('Ctrl Pts',(-6.,17.0647736754607,-1.4253895422543));
#38062=CARTESIAN_POINT('Ctrl Pts',(-6.,17.5148944410332,-1.27181120776873));
#38063=CARTESIAN_POINT('Ctrl Pts',(-6.,17.954969624542,-1.08532323437677));
#38064=CARTESIAN_POINT('Ctrl Pts',(-6.,18.3770565919024,-0.869913211307542));
#38065=CARTESIAN_POINT('Ctrl Pts',(-6.,18.7991432606589,-0.654503340629331));
#38066=CARTESIAN_POINT('Ctrl Pts',(-6.,19.2032417387183,-0.41017146119544));
#38067=CARTESIAN_POINT('Ctrl Pts',(-6.,19.5919320853478,-0.135483412521195));
#38068=CARTESIAN_POINT('',(-5.736443569433,19.8089505408241,-0.442546871806432));
#38069=CARTESIAN_POINT('Origin',(-5.59998163814211,19.5919264032321,-0.135474791301221));
#38070=CARTESIAN_POINT('Ctrl Pts',(-5.732787989488,10.344952798621,-1.71289145292299));
#38071=CARTESIAN_POINT('Ctrl Pts',(-5.73461480973083,11.1182357741961,-1.99332781082549));
#38072=CARTESIAN_POINT('Ctrl Pts',(-5.73605973941588,11.9265526424831,-2.1816925109264));
#38073=CARTESIAN_POINT('Ctrl Pts',(-5.73818934992294,13.5675395619842,-2.35984303021664));
#38074=CARTESIAN_POINT('Ctrl Pts',(-5.73887403074496,14.4000936737092,-2.35028713240501));
#38075=CARTESIAN_POINT('Ctrl Pts',(-5.73948314352597,16.0408966746419,-2.13191112187471));
#38076=CARTESIAN_POINT('Ctrl Pts',(-5.73940757548497,16.8491806682658,-1.9234336965296));
#38077=CARTESIAN_POINT('Ctrl Pts',(-5.73849619058033,18.3938446694523,-1.31839093065865));
#38078=CARTESIAN_POINT('Ctrl Pts',(-5.73766037378413,19.1301818496608,-0.921733807345979));
#38079=CARTESIAN_POINT('Ctrl Pts',(-5.73644356975675,19.8089503602267,-0.442546999301902));
#38080=CARTESIAN_POINT('Origin',(-5.599999999997,19.5919343769573,-0.135488060979611));
#38081=CARTESIAN_POINT('',(-5.593361696257,19.9918770425242,-0.136828655319171));
#38082=CARTESIAN_POINT('Origin',(-5.599999999997,19.5919343769573,-0.135488060979611));
#38083=CARTESIAN_POINT('Origin',(-5.6,19.5919343770044,-0.135488060981261));
#38084=CARTESIAN_POINT('Ctrl Pts',(-5.59335880963393,19.9918769844261,-0.136831702173518));
#38085=CARTESIAN_POINT('Ctrl Pts',(-5.59335897597995,19.9918902023629,-0.132889263698749));
#38086=CARTESIAN_POINT('Ctrl Pts',(-5.59336249921666,19.9921701764066,-0.0456108094042529));
#38087=CARTESIAN_POINT('Ctrl Pts',(-5.59336249921666,19.9921701764069,0.0456108090956939));
#38088=CARTESIAN_POINT('Ctrl Pts',(-5.59335897597995,19.9918902023646,0.132889263387468));
#38089=CARTESIAN_POINT('Ctrl Pts',(-5.59335880963393,19.9918769844279,0.1368317018641));
#38090=CARTESIAN_POINT('Ctrl Pts',(-5.83074004395878,19.9958187405297,-0.136844915099747));
#38091=CARTESIAN_POINT('Ctrl Pts',(-5.83074021194014,19.9958318610111,-0.13290209557407));
#38092=CARTESIAN_POINT('Ctrl Pts',(-5.8307437698124,19.9961097709333,-0.0456152065241548));
#38093=CARTESIAN_POINT('Ctrl Pts',(-5.83074376981241,19.9961097709314,0.0456152062141224));
#38094=CARTESIAN_POINT('Ctrl Pts',(-5.83074021194014,19.9958318610128,0.132902095265602));
#38095=CARTESIAN_POINT('Ctrl Pts',(-5.83074004395878,19.9958187405316,0.13684491479334));
#38096=CARTESIAN_POINT('Ctrl Pts',(-6.00000347483923,19.8293408303182,-0.136286874323723));
#38097=CARTESIAN_POINT('Ctrl Pts',(-6.00000357357543,19.8293538265013,-0.132360134067916));
#38098=CARTESIAN_POINT('Ctrl Pts',(-6.0000056648227,19.8296291037059,-0.0454292086005723));
#38099=CARTESIAN_POINT('Ctrl Pts',(-6.0000056648227,19.8296291037082,0.0454292082960187));
#38100=CARTESIAN_POINT('Ctrl Pts',(-6.00000357357543,19.8293538265043,0.132360133764452));
#38101=CARTESIAN_POINT('Ctrl Pts',(-6.00000347483923,19.8293408303212,0.136286874022268));
#38102=CARTESIAN_POINT('Ctrl Pts',(-5.9999999999769,19.5919285123983,-0.135491058510798));
#38103=CARTESIAN_POINT('Ctrl Pts',(-5.99999999996753,19.5919414317191,-0.131587249061459));
#38104=CARTESIAN_POINT('Ctrl Pts',(-5.99999999976694,19.5922150808793,-0.0451639658275902));
#38105=CARTESIAN_POINT('Ctrl Pts',(-5.99999999976694,19.5922150808828,0.0451639655258831));
#38106=CARTESIAN_POINT('Ctrl Pts',(-5.99999999996752,19.591941431722,0.131587248762196));
#38107=CARTESIAN_POINT('Ctrl Pts',(-5.9999999999769,19.5919285124013,0.135491058213587));
#38108=CARTESIAN_POINT('Origin',(-5.47627593058377,-17.2218949143738,6.06772203221723E-6));
#38109=CARTESIAN_POINT('Ctrl Pts',(-6.00000000001697,19.5919329102797,-0.135482829540219));
#38110=CARTESIAN_POINT('Ctrl Pts',(-6.00000000001005,19.5919459863958,-0.131581789340447));
#38111=CARTESIAN_POINT('Ctrl Pts',(-6.00000000000347,19.591958508822,-0.127680725304212));
#38112=CARTESIAN_POINT('Ctrl Pts',(-5.9999999999973,19.5919704756381,-0.123779639821517));
#38113=CARTESIAN_POINT('Ctrl Pts',(-5.99999999993208,19.5920970397706,-0.082520754142832));
#38114=CARTESIAN_POINT('Ctrl Pts',(-5.99999999990817,19.5921614523042,-0.0412594672366372));
#38115=CARTESIAN_POINT('Ctrl Pts',(-5.99999999990817,19.5921614509438,1.4231705702387E-6));
#38116=CARTESIAN_POINT('Ctrl Pts',(-5.99999999990817,19.5921614495833,0.0412621564140265));
#38117=CARTESIAN_POINT('Ctrl Pts',(-5.99999999993208,19.5920970348205,0.0825224934060036));
#38118=CARTESIAN_POINT('Ctrl Pts',(-5.9999999999973,19.5919704760335,0.123779639519311));
#38119=CARTESIAN_POINT('Ctrl Pts',(-6.00000000000346,19.5919585091951,0.12768073253251));
#38120=CARTESIAN_POINT('Ctrl Pts',(-6.00000000001005,19.5919459867654,0.131581797037309));
#38121=CARTESIAN_POINT('Ctrl Pts',(-6.00000000001698,19.5919329106708,0.135482830646012));
#38122=CARTESIAN_POINT('Ctrl Pts',(-5.67764080611035,19.9920086654548,-0.35317650519169));
#38123=CARTESIAN_POINT('Ctrl Pts',(-3.78509387074023,19.9513483860085,-1.26988355976882));
#38124=CARTESIAN_POINT('Ctrl Pts',(-2.0656550255016E-10,19.8990602291944,
-2.18625140349313));
#38125=CARTESIAN_POINT('Ctrl Pts',(3.78509387032731,19.9513483860076,-1.26988355987377));
#38126=CARTESIAN_POINT('Ctrl Pts',(5.67764080549097,19.9920086654425,-0.353176505498152));
#38127=CARTESIAN_POINT('Ctrl Pts',(-5.67764080611035,19.9939837518553,-0.127283758352494));
#38128=CARTESIAN_POINT('Ctrl Pts',(-3.78509387074023,19.9624116465656,-0.457857765159308));
#38129=CARTESIAN_POINT('Ctrl Pts',(-2.0656550255016E-10,20.0792796545209,
-0.792979083240276));
#38130=CARTESIAN_POINT('Ctrl Pts',(3.78509387032731,19.9624116465789,-0.457857765200401));
#38131=CARTESIAN_POINT('Ctrl Pts',(5.67764080549097,19.9939837518422,-0.127283758470664));
#38132=CARTESIAN_POINT('Ctrl Pts',(-5.67764080611035,19.9940637065833,0.0986861771942666));
#38133=CARTESIAN_POINT('Ctrl Pts',(-3.78509387074023,19.9628595054405,0.355008386647923));
#38134=CARTESIAN_POINT('Ctrl Pts',(-2.0656550255016E-10,20.0865752314139,
0.615338279627633));
#38135=CARTESIAN_POINT('Ctrl Pts',(3.78509387032731,19.9628595054527,0.355008386675378));
#38136=CARTESIAN_POINT('Ctrl Pts',(5.67764080549097,19.9940637065743,0.0986861772782846));
#38137=CARTESIAN_POINT('Ctrl Pts',(-5.67764080611035,19.9922485296364,0.324585173480459));
#38138=CARTESIAN_POINT('Ctrl Pts',(-3.78509387074023,19.9526919626316,1.16710221932013));
#38139=CARTESIAN_POINT('Ctrl Pts',(-2.0656550255016E-10,19.9209469598825,
2.00982869570971));
#38140=CARTESIAN_POINT('Ctrl Pts',(3.78509387032731,19.9526919626278,1.16710221941215));
#38141=CARTESIAN_POINT('Ctrl Pts',(5.67764080549097,19.9922485296225,0.324585173755783));
#38142=CARTESIAN_POINT('Ctrl Pts',(-5.59336169625714,19.9918770425157,-0.136828655319142));
#38143=CARTESIAN_POINT('Ctrl Pts',(-5.58009644017448,19.9916362290972,-0.142984613489992));
#38144=CARTESIAN_POINT('Ctrl Pts',(-5.56074613957355,19.9912865571345,-0.151958711829183));
#38145=CARTESIAN_POINT('Ctrl Pts',(-5.53527458568659,19.9908348355144,-0.163677026593076));
#38146=CARTESIAN_POINT('Ctrl Pts',(-5.50989210816338,19.9903846936063,-0.175354361333796));
#38147=CARTESIAN_POINT('Ctrl Pts',(-5.47843096000199,19.9898333361175,-0.1897568285786));
#38148=CARTESIAN_POINT('Ctrl Pts',(-5.44083463266139,19.9891901590629,-0.206764048111785));
#38149=CARTESIAN_POINT('Ctrl Pts',(-5.41345000419988,19.9887216780723,-0.219151864183826));
#38150=CARTESIAN_POINT('Ctrl Pts',(-5.38280993341899,19.988204554942,-0.232920656878242));
#38151=CARTESIAN_POINT('Ctrl Pts',(-5.34888648441068,19.9876426410121,-0.248007586354099));
#38152=CARTESIAN_POINT('Ctrl Pts',(-5.30328426181425,19.9868872778383,-0.268288469824585));
#38153=CARTESIAN_POINT('Ctrl Pts',(-5.25174934336198,19.9860509360498,-0.290953240785525));
#38154=CARTESIAN_POINT('Ctrl Pts',(-5.19419938879444,19.9851442256669,-0.315807394008167));
#38155=CARTESIAN_POINT('Ctrl Pts',(-5.15774847931625,19.9845699347168,-0.331549482704565));
#38156=CARTESIAN_POINT('Ctrl Pts',(-5.11888420994136,19.9839674252062,-0.348168925542301));
#38157=CARTESIAN_POINT('Ctrl Pts',(-5.07758279458025,19.9833392305093,-0.365605829096777));
#38158=CARTESIAN_POINT('Ctrl Pts',(-5.01428717619997,19.9823765038944,-0.392328390139004));
#38159=CARTESIAN_POINT('Ctrl Pts',(-4.94526809252529,19.9813534060161,-0.420973376428607));
#38160=CARTESIAN_POINT('Ctrl Pts',(-4.87042927244288,19.9802806512975,-0.451284601016866));
#38161=CARTESIAN_POINT('Ctrl Pts',(-4.84061551917361,19.979853294954,-0.463359769628138));
#38162=CARTESIAN_POINT('Ctrl Pts',(-4.80987804835423,19.9794180560131,-0.475698813708442));
#38163=CARTESIAN_POINT('Ctrl Pts',(-4.77821033097395,19.9789755899773,-0.488283254179042));
#38164=CARTESIAN_POINT('Ctrl Pts',(-4.70107154376649,19.9778977954215,-0.518937452078098));
#38165=CARTESIAN_POINT('Ctrl Pts',(-4.61841362640652,19.9767770765998,-0.55105125131751));
#38166=CARTESIAN_POINT('Ctrl Pts',(-4.53013604499199,19.9756247565424,-0.58432225556632));
#38167=CARTESIAN_POINT('Ctrl Pts',(-4.50293366277614,19.9752696737441,-0.594574581918937));
#38168=CARTESIAN_POINT('Ctrl Pts',(-4.47519762071291,19.9749115925001,-0.60493642323504));
#38169=CARTESIAN_POINT('Ctrl Pts',(-4.44692485275567,19.9745508479666,-0.615397929701921));
#38170=CARTESIAN_POINT('Ctrl Pts',(-4.35781685172489,19.9734138802558,-0.648369725404562));
#38171=CARTESIAN_POINT('Ctrl Pts',(-4.26337760100315,19.9722503887103,-0.682335366219507));
#38172=CARTESIAN_POINT('Ctrl Pts',(-4.16350896254227,19.9710726333925,-0.716953413664895));
#38173=CARTESIAN_POINT('Ctrl Pts',(-4.13544397277845,19.9707416617136,-0.72668174442189));
#38174=CARTESIAN_POINT('Ctrl Pts',(-4.10695019601858,19.9704095684455,-0.736461284000019));
#38175=CARTESIAN_POINT('Ctrl Pts',(-4.07802541747408,19.9700766365274,-0.746283705314207));
#38176=CARTESIAN_POINT('Ctrl Pts',(-3.98974865350231,19.9690605474222,-0.776261171404391));
#38177=CARTESIAN_POINT('Ctrl Pts',(-3.89745734273723,19.9680365943023,-0.806640345102402));
#38178=CARTESIAN_POINT('Ctrl Pts',(-3.80108980409398,19.9670138196758,-0.837164813292626));
#38179=CARTESIAN_POINT('Ctrl Pts',(-3.75649682634983,19.9665405424001,-0.851289662280391));
#38180=CARTESIAN_POINT('Ctrl Pts',(-3.71103102503581,19.9660675268623,-0.865445191326704));
#38181=CARTESIAN_POINT('Ctrl Pts',(-3.66468636938461,19.9655957181186,-0.879603669421038));
#38182=CARTESIAN_POINT('Ctrl Pts',(-3.629247389634,19.965234933897,-0.890430419807553));
#38183=CARTESIAN_POINT('Ctrl Pts',(-3.59329450760697,19.9648748557562,-0.901258864403766));
#38184=CARTESIAN_POINT('Ctrl Pts',(-3.55682518356218,19.9645159343212,-0.912076066338966));
#38185=CARTESIAN_POINT('Ctrl Pts',(-3.51474448708024,19.9641017872438,-0.924557662950405));
#38186=CARTESIAN_POINT('Ctrl Pts',(-3.47197612954805,19.9636891723991,-0.937024514001034));
#38187=CARTESIAN_POINT('Ctrl Pts',(-3.42851638066827,19.9632788118654,-0.949455625228041));
#38188=CARTESIAN_POINT('Ctrl Pts',(-3.40678650622838,19.9630736315986,-0.955671180841545));
#38189=CARTESIAN_POINT('Ctrl Pts',(-3.38488378395104,19.9628690147478,-0.961877801491924));
#38190=CARTESIAN_POINT('Ctrl Pts',(-3.36280774484562,19.9626650525873,-0.968072805286863));
#38191=CARTESIAN_POINT('Ctrl Pts',(-3.35176972529291,19.962563071507,-0.971170307184331));
#38192=CARTESIAN_POINT('Ctrl Pts',(-3.34068837653317,19.9624612540851,-0.974264904867446));
#38193=CARTESIAN_POINT('Ctrl Pts',(-3.32956364118686,19.9623596118574,-0.977356257519711));
#38194=CARTESIAN_POINT('Ctrl Pts',(-3.3240012735137,19.9623087907436,-0.978901933845844));
#38195=CARTESIAN_POINT('Ctrl Pts',(-3.3184280591939,19.9622580134274,-0.980446798914225));
#38196=CARTESIAN_POINT('Ctrl Pts',(-3.3128439911071,19.9622072813604,-0.981990809731292));
#38197=CARTESIAN_POINT('Ctrl Pts',(-3.30725992302029,19.9621565492934,-0.983534820548359));
#38198=CARTESIAN_POINT('Ctrl Pts',(-3.30284643870994,19.9621165350483,-0.984752940852499));
#38199=CARTESIAN_POINT('Ctrl Pts',(-3.29605921844197,19.9620552223591,-0.986620236315678));
#38200=CARTESIAN_POINT('Ctrl Pts',(-3.26420947507747,19.9617675061309,-0.995382716232327));
#38201=CARTESIAN_POINT('Ctrl Pts',(-3.23246236011294,19.961485434778,-1.00399045631962));
#38202=CARTESIAN_POINT('Ctrl Pts',(-3.20081930664225,19.961208906558,-1.01244547959457));
#38203=CARTESIAN_POINT('Ctrl Pts',(-3.02528053482623,19.959674875585,-1.05934943602643));
#38204=CARTESIAN_POINT('Ctrl Pts',(-2.85294730098256,19.9583113839894,-1.10155240253784));
#38205=CARTESIAN_POINT('Ctrl Pts',(-2.68405734163335,19.9571013326502,-1.13942220670422));
#38206=CARTESIAN_POINT('Ctrl Pts',(-2.50183512028643,19.9557957592235,-1.18028147307956));
#38207=CARTESIAN_POINT('Ctrl Pts',(-2.32362196300848,19.9546687611369,-1.21609717693824));
#38208=CARTESIAN_POINT('Ctrl Pts',(-2.14968414857974,19.9536983326622,-1.24736532756201));
#38209=CARTESIAN_POINT('Ctrl Pts',(-2.13682519108344,19.9536265903643,-1.2496769342772));
#38210=CARTESIAN_POINT('Ctrl Pts',(-2.12398957691993,19.9535557043388,-1.25196368987188));
#38211=CARTESIAN_POINT('Ctrl Pts',(-2.11117740271896,19.9534856659585,-1.25422579612376));
#38212=CARTESIAN_POINT('Ctrl Pts',(-1.93621865309989,19.95252924535,-1.28511635967114));
#38213=CARTESIAN_POINT('Ctrl Pts',(-1.7656353215977,19.9517307044816,-1.31141089660614));
#38214=CARTESIAN_POINT('Ctrl Pts',(-1.59966046888125,19.9510660881632,-1.33364632095043));
#38215=CARTESIAN_POINT('Ctrl Pts',(-1.55744726884481,19.9508970530285,-1.33930156570817));
#38216=CARTESIAN_POINT('Ctrl Pts',(-1.51553191190328,19.9507366921506,-1.34469420710316));
#38217=CARTESIAN_POINT('Ctrl Pts',(-1.47391771006237,19.9505846339209,-1.34983299816217));
#38218=CARTESIAN_POINT('Ctrl Pts',(-1.30946665097347,19.9499837300033,-1.37014047961576));
#38219=CARTESIAN_POINT('Ctrl Pts',(-1.14972249295738,19.949512234599,-1.386485381975));
#38220=CARTESIAN_POINT('Ctrl Pts',(-0.994867945863715,19.949145973856,-1.39942373538886));
#38221=CARTESIAN_POINT('Ctrl Pts',(-0.92299758083666,19.9489759866403,-1.40542862320233));
#38222=CARTESIAN_POINT('Ctrl Pts',(-0.852179763116334,19.9488287115822,
-1.41069942676756));
#38223=CARTESIAN_POINT('Ctrl Pts',(-0.782429370782511,19.9487019529345,
-1.41529007975822));
#38224=CARTESIAN_POINT('Ctrl Pts',(-0.633135744668933,19.9484306389314,
-1.42511590594029));
#38225=CARTESIAN_POINT('Ctrl Pts',(-0.488734978173752,19.9482529345977,
-1.43182821637309));
#38226=CARTESIAN_POINT('Ctrl Pts',(-0.349348859034708,19.9481438619172,
-1.43595954720335));
#38227=CARTESIAN_POINT('Ctrl Pts',(-0.262235554798481,19.9480756938553,
-1.43854153945438));
#38228=CARTESIAN_POINT('Ctrl Pts',(-0.177080119018712,19.9480344392527,
-1.44011472297812));
#38229=CARTESIAN_POINT('Ctrl Pts',(-0.0939047509515874,19.9480149632798,
-1.44080217709803));
#38230=CARTESIAN_POINT('Ctrl Pts',(0.0408608604582856,19.9479834071659,
-1.44191603059744));
#38231=CARTESIAN_POINT('Ctrl Pts',(0.170426608443204,19.9480093358015,-1.44070684670635));
#38232=CARTESIAN_POINT('Ctrl Pts',(0.294722178057082,19.9480858363438,-1.43767395803733));
#38233=CARTESIAN_POINT('Ctrl Pts',(0.343048654823458,19.9481155799758,-1.43649476215566));
#38234=CARTESIAN_POINT('Ctrl Pts',(0.390578812885668,19.9481529485472,-1.43503944637556));
#38235=CARTESIAN_POINT('Ctrl Pts',(0.437309817035389,19.9481974668766,-1.43333570032628));
#38236=CARTESIAN_POINT('Ctrl Pts',(0.473889188802879,19.948232314245,-1.43200206837747));
#38237=CARTESIAN_POINT('Ctrl Pts',(0.509978917138882,19.9482715416553,-1.43051619975346));
#38238=CARTESIAN_POINT('Ctrl Pts',(0.545577925881862,19.9483149076229,-1.42889097738007));
#38239=CARTESIAN_POINT('Ctrl Pts',(0.575261242611154,19.9483510672183,-1.42753582755516));
#38240=CARTESIAN_POINT('Ctrl Pts',(0.60460338601008,19.9483901039359,-1.42608378579906));
#38241=CARTESIAN_POINT('Ctrl Pts',(0.633603956839183,19.9484318697382,-1.42454228018567));
#38242=CARTESIAN_POINT('Ctrl Pts',(0.665494340265893,19.9484777973669,-1.42284716854958));
#38243=CARTESIAN_POINT('Ctrl Pts',(0.696971606900236,19.9485270246339,-1.42104388842941));
#38244=CARTESIAN_POINT('Ctrl Pts',(0.728035441233224,19.9485793495753,-1.41914204120244));
#38245=CARTESIAN_POINT('Ctrl Pts',(0.743567358399718,19.948605512046,-1.41819111758896));
#38246=CARTESIAN_POINT('Ctrl Pts',(0.758995917489945,19.948632448546,-1.41721555217114));
#38247=CARTESIAN_POINT('Ctrl Pts',(0.774321073339735,19.9486601335504,-1.4162165167394));
#38248=CARTESIAN_POINT('Ctrl Pts',(0.78198365126463,19.9486739760527,-1.41571699902353));
#38249=CARTESIAN_POINT('Ctrl Pts',(0.789620378379354,19.9486880056576,-1.41521161380253));
#38250=CARTESIAN_POINT('Ctrl Pts',(0.79723125033673,19.9487022191044,-1.4147005065104));
#38251=CARTESIAN_POINT('Ctrl Pts',(0.804842122294106,19.9487164325513,-1.41418939921827));
#38252=CARTESIAN_POINT('Ctrl Pts',(0.8141885175813,19.9487342266443,-1.41355084271498));
#38253=CARTESIAN_POINT('Ctrl Pts',(0.819986296612124,19.9487454076543,-1.41315016332844));
#38254=CARTESIAN_POINT('Ctrl Pts',(0.912968818718277,19.9489247243383,-1.40672422337471));
#38255=CARTESIAN_POINT('Ctrl Pts',(1.01085354077577,19.949146375472,-1.39887348397393));
#38256=CARTESIAN_POINT('Ctrl Pts',(1.11358303380358,19.9494232496908,-1.38924753938107));
#38257=CARTESIAN_POINT('Ctrl Pts',(1.22623353893273,19.9497268627981,-1.37869197749938));
#38258=CARTESIAN_POINT('Ctrl Pts',(1.34471056382887,19.950096901445,-1.36600184523302));
#38259=CARTESIAN_POINT('Ctrl Pts',(1.46890925483827,19.9505514692569,-1.35068217452509));
#38260=CARTESIAN_POINT('Ctrl Pts',(1.5153837961882,19.9507215663037,-1.34494962884368));
#38261=CARTESIAN_POINT('Ctrl Pts',(1.56265915662713,19.9509035257976,-1.33884849850583));
#38262=CARTESIAN_POINT('Ctrl Pts',(1.61072854604317,19.9510983943111,-1.33235148126275));
#38263=CARTESIAN_POINT('Ctrl Pts',(1.74017460898387,19.9516231557482,-1.31485566296359));
#38264=CARTESIAN_POINT('Ctrl Pts',(1.87538176880813,19.9522413543956,-1.29449106412342));
#38265=CARTESIAN_POINT('Ctrl Pts',(2.01619359019374,19.9529742557988,-1.27071133078169));
#38266=CARTESIAN_POINT('Ctrl Pts',(2.02948594399093,19.9530434402227,-1.26846657160117));
#38267=CARTESIAN_POINT('Ctrl Pts',(2.04282820892096,19.9531136486326,-1.26619135877892));
#38268=CARTESIAN_POINT('Ctrl Pts',(2.05622023297625,19.9531849000987,-1.26388521963766));
#38269=CARTESIAN_POINT('Ctrl Pts',(2.18611588762425,19.9538760021906,-1.24151687171451));
#38270=CARTESIAN_POINT('Ctrl Pts',(2.32069562415765,19.954665116498,-1.21624008450209));
#38271=CARTESIAN_POINT('Ctrl Pts',(2.45980641014352,19.9555695145239,-1.1876232037297));
#38272=CARTESIAN_POINT('Ctrl Pts',(2.57751721920422,19.95633478533,-1.16340857389609));
#38273=CARTESIAN_POINT('Ctrl Pts',(2.69847171415293,19.9571826339952,-1.13680195572644));
#38274=CARTESIAN_POINT('Ctrl Pts',(2.82256104373563,19.9581238872826,-1.10754080826207));
#38275=CARTESIAN_POINT('Ctrl Pts',(2.92925609544617,19.9589331999649,-1.0823813553718));
#38276=CARTESIAN_POINT('Ctrl Pts',(3.03826843858179,19.959811580392,-1.05525922949466));
#38277=CARTESIAN_POINT('Ctrl Pts',(3.14952010306516,19.9607660880248,-1.02600930039865));
#38278=CARTESIAN_POINT('Ctrl Pts',(3.24640822738728,19.961597360569,-1.00053578699257));
#38279=CARTESIAN_POINT('Ctrl Pts',(3.34499460831031,19.9624863767901,-0.973448371221141));
#38280=CARTESIAN_POINT('Ctrl Pts',(3.44522290327178,19.9634379571108,-0.944640100632512));
#38281=CARTESIAN_POINT('Ctrl Pts',(3.44872500124271,19.9634712064792,-0.94363350478038));
#38282=CARTESIAN_POINT('Ctrl Pts',(3.4522291031841,19.963504532248,-0.942624808085872));
#38283=CARTESIAN_POINT('Ctrl Pts',(3.45573520662724,19.9635379346302,-0.941614006063889));
#38284=CARTESIAN_POINT('Ctrl Pts',(3.53381527373909,19.964281797521,-0.919103691980711));
#38285=CARTESIAN_POINT('Ctrl Pts',(3.61288815483183,19.9650636505888,-0.895549195410826));
#38286=CARTESIAN_POINT('Ctrl Pts',(3.69292540203938,19.9658858830604,-0.870901362357781));
#38287=CARTESIAN_POINT('Ctrl Pts',(3.6995495805477,19.9659539340598,-0.868861416561504));
#38288=CARTESIAN_POINT('Ctrl Pts',(3.70618036478951,19.966022261695,-0.866813981888607));
#38289=CARTESIAN_POINT('Ctrl Pts',(3.71281773769273,19.9660908673404,-0.864759030751817));
#38290=CARTESIAN_POINT('Ctrl Pts',(3.74627869963934,19.9664367287111,-0.854399413657385));
#38291=CARTESIAN_POINT('Ctrl Pts',(3.77990711552836,19.9667896554082,-0.84384876565254));
#38292=CARTESIAN_POINT('Ctrl Pts',(3.81370081233948,19.9671498333894,-0.833103598408753));
#38293=CARTESIAN_POINT('Ctrl Pts',(3.83394934812138,19.9673656451362,-0.826665300029194));
#38294=CARTESIAN_POINT('Ctrl Pts',(3.85425722301091,19.967584060312,-0.820157165131984));
#38295=CARTESIAN_POINT('Ctrl Pts',(3.87462396755603,19.9678051193895,-0.813578448686667));
#38296=CARTESIAN_POINT('Ctrl Pts',(3.88480733982858,19.9679156489282,-0.81028909046401));
#38297=CARTESIAN_POINT('Ctrl Pts',(3.89500542951504,19.9680268394502,-0.806982086854589));
#38298=CARTESIAN_POINT('Ctrl Pts',(3.90521817679822,19.9681386960524,-0.80365734496727));
#38299=CARTESIAN_POINT('Ctrl Pts',(3.9103245504398,19.9681946243536,-0.80199497402361));
#38300=CARTESIAN_POINT('Ctrl Pts',(3.91543458848057,19.9682507191752,-0.800328168510491));
#38301=CARTESIAN_POINT('Ctrl Pts',(3.92054828339348,19.9683069811566,-0.798656916846781));
#38302=CARTESIAN_POINT('Ctrl Pts',(3.92566197830639,19.9683632431379,-0.796985665183072));
#38303=CARTESIAN_POINT('Ctrl Pts',(3.93254611564147,19.9684391986675,-0.794730300529606));
#38304=CARTESIAN_POINT('Ctrl Pts',(3.93590033120455,19.9684762692202,-0.793629811831234));
#38305=CARTESIAN_POINT('Ctrl Pts',(3.94215184182074,19.9685453604724,-0.791578746045063));
#38306=CARTESIAN_POINT('Ctrl Pts',(3.9483863655703,19.9686144529542,-0.789528428402651));
#38307=CARTESIAN_POINT('Ctrl Pts',(3.95460391946738,19.9686835441334,-0.787478931678669));
#38308=CARTESIAN_POINT('Ctrl Pts',(4.02981766560043,19.9695193400903,-0.7626861709162));
#38309=CARTESIAN_POINT('Ctrl Pts',(4.10254807853478,19.9703549292316,-0.738014505222679));
#38310=CARTESIAN_POINT('Ctrl Pts',(4.17282587992973,19.9711860991373,-0.713586601878876));
#38311=CARTESIAN_POINT('Ctrl Pts',(4.24075388496264,19.9719894781903,-0.689975465668788));
#38312=CARTESIAN_POINT('Ctrl Pts',(4.30639057596857,19.9727887343623,-0.666591965479921));
#38313=CARTESIAN_POINT('Ctrl Pts',(4.36976383144435,19.9735803936586,-0.643536957258541));
#38314=CARTESIAN_POINT('Ctrl Pts',(4.4312145094457,19.9743480360992,-0.621181377197298));
#38315=CARTESIAN_POINT('Ctrl Pts',(4.49053701984079,19.975108541002,-0.599134582787114));
#38316=CARTESIAN_POINT('Ctrl Pts',(4.54775645035834,19.9758590147286,-0.577480233927572));
#38317=CARTESIAN_POINT('Ctrl Pts',(4.60351117578851,19.9765902778012,-0.556380193886757));
#38318=CARTESIAN_POINT('Ctrl Pts',(4.65726912327683,19.9773120217359,-0.535652705120557));
#38319=CARTESIAN_POINT('Ctrl Pts',(4.70905288636104,19.9780217932391,-0.515368113490108));
#38320=CARTESIAN_POINT('Ctrl Pts',(4.75987167760566,19.9787183384052,-0.495461517944441));
#38321=CARTESIAN_POINT('Ctrl Pts',(4.80878918171655,19.979403358028,-0.47598142251901));
#38322=CARTESIAN_POINT('Ctrl Pts',(4.85582595140891,19.9800747136533,-0.456988155099427));
#38323=CARTESIAN_POINT('Ctrl Pts',(4.90207918063831,19.9807348858088,-0.438311278317304));
#38324=CARTESIAN_POINT('Ctrl Pts',(4.94651381542896,19.9813818500243,-0.420105108591858));
#38325=CARTESIAN_POINT('Ctrl Pts',(4.98914848403816,19.9820137117629,-0.402421574654211));
#38326=CARTESIAN_POINT('Ctrl Pts',(4.98949674229069,19.9820188730805,-0.402277127967314));
#38327=CARTESIAN_POINT('Ctrl Pts',(4.9898448804389,19.9820240333899,-0.402132716123775));
#38328=CARTESIAN_POINT('Ctrl Pts',(4.99019289849271,19.98202919269,-0.401988339150492));
#38329=CARTESIAN_POINT('Ctrl Pts',(5.03325928093211,19.9826676434525,-0.384122042046895));
#38330=CARTESIAN_POINT('Ctrl Pts',(5.07448668103045,19.9832906519714,-0.366790155603053));
#38331=CARTESIAN_POINT('Ctrl Pts',(5.11389326225468,19.9838963666681,-0.350040984422825));
#38332=CARTESIAN_POINT('Ctrl Pts',(5.15369851227836,19.9845082092638,-0.33312236510072));
#38333=CARTESIAN_POINT('Ctrl Pts',(5.19164591949423,19.9851024113326,-0.316798299988091));
#38334=CARTESIAN_POINT('Ctrl Pts',(5.22775300183307,19.9856771307056,-0.30111336975242));
#38335=CARTESIAN_POINT('Ctrl Pts',(5.26453925416354,19.9862626604828,-0.285133407815299));
#38336=CARTESIAN_POINT('Ctrl Pts',(5.29941530406552,19.9868279722818,-0.269816847791514));
#38337=CARTESIAN_POINT('Ctrl Pts',(5.3323983228196,19.9873711404656,-0.25520554745017));
#38338=CARTESIAN_POINT('Ctrl Pts',(5.36641335074965,19.9879313038963,-0.240137072581005));
#38339=CARTESIAN_POINT('Ctrl Pts',(5.3984150436722,19.9884679195571,-0.225818690317629));
#38340=CARTESIAN_POINT('Ctrl Pts',(5.42842066614577,19.988978852473,-0.212290672821496));
#38341=CARTESIAN_POINT('Ctrl Pts',(5.45996866123902,19.9895160487648,-0.198067277523987));
#38342=CARTESIAN_POINT('Ctrl Pts',(5.48931013100147,19.9900248540869,-0.184717620138269));
#38343=CARTESIAN_POINT('Ctrl Pts',(5.51646318129326,19.9905027280262,-0.172282013503108));
#38344=CARTESIAN_POINT('Ctrl Pts',(5.54440810117859,19.9909945382946,-0.159483744895691));
#38345=CARTESIAN_POINT('Ctrl Pts',(5.5700351312696,19.9914535784914,-0.147653628555669));
#38346=CARTESIAN_POINT('Ctrl Pts',(5.59336166012999,19.9918770419872,-0.136828574471761));
#38347=CARTESIAN_POINT('Ctrl Pts',(-5.84637330108191,19.8012033146892,-0.398518179817078));
#38348=CARTESIAN_POINT('Ctrl Pts',(-5.81071183853046,19.8004234735737,-0.415207321699024));
#38349=CARTESIAN_POINT('Ctrl Pts',(-5.69191996061893,19.7978801854681,-0.470269915973425));
#38350=CARTESIAN_POINT('Ctrl Pts',(-5.48049741251962,19.7936452864078,-0.565143604366032));
#38351=CARTESIAN_POINT('Ctrl Pts',(-5.20215554401679,19.7885001063612,-0.684048267802473));
#38352=CARTESIAN_POINT('Ctrl Pts',(-4.89414931300705,19.7832362546721,-0.808353235124788));
#38353=CARTESIAN_POINT('Ctrl Pts',(-4.55276913238558,19.7778650102664,-0.937266430508365));
#38354=CARTESIAN_POINT('Ctrl Pts',(-4.1723835688134,19.7724100565091,-1.06997734570926));
#38355=CARTESIAN_POINT('Ctrl Pts',(-3.74657439469389,19.7669368801863,-1.20488365535651));
#38356=CARTESIAN_POINT('Ctrl Pts',(-3.27003381843662,19.761584724194,-1.33873908498052));
#38357=CARTESIAN_POINT('Ctrl Pts',(-2.73868853585576,19.7565628732899,-1.46664667446678));
#38358=CARTESIAN_POINT('Ctrl Pts',(-2.14775624696211,19.7521256584225,-1.58252476859859));
#38359=CARTESIAN_POINT('Ctrl Pts',(-1.49664356855033,19.7486057968215,-1.67793559717415));
#38360=CARTESIAN_POINT('Ctrl Pts',(-0.805427675692797,19.7463898065183,
-1.74162179620427));
#38361=CARTESIAN_POINT('Ctrl Pts',(-0.11332682193267,19.7456265332955,-1.76632927594041));
#38362=CARTESIAN_POINT('Ctrl Pts',(0.536179045116112,19.7459830344993,-1.75438694563656));
#38363=CARTESIAN_POINT('Ctrl Pts',(1.11984701057849,19.7473096705852,-1.71489328080823));
#38364=CARTESIAN_POINT('Ctrl Pts',(1.63691896308617,19.7493622962935,-1.65738847905435));
#38365=CARTESIAN_POINT('Ctrl Pts',(2.09763398182801,19.7519182398037,-1.58838117097954));
#38366=CARTESIAN_POINT('Ctrl Pts',(2.51226399849238,19.7548276213681,-1.51186339189556));
#38367=CARTESIAN_POINT('Ctrl Pts',(2.88624760872843,19.7579578014457,-1.43111102238662));
#38368=CARTESIAN_POINT('Ctrl Pts',(3.2232642926507,19.7611949382187,-1.3488210050365));
#38369=CARTESIAN_POINT('Ctrl Pts',(3.52768199159861,19.7644624365646,-1.26672665052053));
#38370=CARTESIAN_POINT('Ctrl Pts',(3.80292724591826,19.7677009282426,-1.18614757862148));
#38371=CARTESIAN_POINT('Ctrl Pts',(4.05164145124967,19.7708623531949,-1.10814408881512));
#38372=CARTESIAN_POINT('Ctrl Pts',(4.27616841473193,19.7739109745617,-1.03349245184477));
#38373=CARTESIAN_POINT('Ctrl Pts',(4.47886355116955,19.7768248933238,-0.962648114845364));
#38374=CARTESIAN_POINT('Ctrl Pts',(4.66208312282989,19.7795942073923,-0.895791076677767));
#38375=CARTESIAN_POINT('Ctrl Pts',(4.82814550069091,19.7822187964435,-0.832879638048502));
#38376=CARTESIAN_POINT('Ctrl Pts',(4.97929162616721,19.7847061436466,-0.773703187802608));
#38377=CARTESIAN_POINT('Ctrl Pts',(5.11758620004362,19.7870683005815,-0.717955657569331));
#38378=CARTESIAN_POINT('Ctrl Pts',(5.24463111737929,19.7893154169154,-0.665388285718238));
#38379=CARTESIAN_POINT('Ctrl Pts',(5.3615187146248,19.7914528178618,-0.615872998117026));
#38380=CARTESIAN_POINT('Ctrl Pts',(5.46895006327484,19.7934813185126,-0.569387115888077));
#38381=CARTESIAN_POINT('Ctrl Pts',(5.56756311198424,19.7954023289415,-0.525890087244043));
#38382=CARTESIAN_POINT('Ctrl Pts',(5.65800137343926,19.797218820486,-0.485299481939044));
#38383=CARTESIAN_POINT('Ctrl Pts',(5.74091079063728,19.7989350271782,-0.447496453563895));
#38384=CARTESIAN_POINT('Ctrl Pts',(5.80284291081797,19.8002555833714,-0.418850315846327));
#38385=CARTESIAN_POINT('Ctrl Pts',(5.83721317807521,19.8010036894276,-0.402804474198884));
#38386=CARTESIAN_POINT('Ctrl Pts',(5.84634757864291,19.8012036144135,-0.398529569715516));
#38387=CARTESIAN_POINT('Ctrl Pts',(-5.81214048419312,19.9271886646867,-0.330203432875564));
#38388=CARTESIAN_POINT('Ctrl Pts',(-5.77669382802178,19.9264355395185,-0.3468342593928));
#38389=CARTESIAN_POINT('Ctrl Pts',(-5.65860909331072,19.9239803249271,-0.401708617535871));
#38390=CARTESIAN_POINT('Ctrl Pts',(-5.44840462341083,19.9198968585245,-0.496277870204232));
#38391=CARTESIAN_POINT('Ctrl Pts',(-5.17162939492092,19.9149425108579,-0.614820284163497));
#38392=CARTESIAN_POINT('Ctrl Pts',(-4.86534603855596,19.909880421409,-0.7387553338152));
#38393=CARTESIAN_POINT('Ctrl Pts',(-4.52588138424955,19.9047214712814,-0.867287833853044));
#38394=CARTESIAN_POINT('Ctrl Pts',(-4.14764846585593,19.8994886557635,-0.999606191879825));
#38395=CARTESIAN_POINT('Ctrl Pts',(-3.72427691756136,19.8942451763706,-1.13411062738609));
#38396=CARTESIAN_POINT('Ctrl Pts',(-3.25050020752433,19.8891247812009,-1.2675631879692));
#38397=CARTESIAN_POINT('Ctrl Pts',(-2.72227770248346,19.8843277548829,-1.39508118266476));
#38398=CARTESIAN_POINT('Ctrl Pts',(-2.13486068553421,19.8800965858062,-1.51060199964442));
#38399=CARTESIAN_POINT('Ctrl Pts',(-1.48765672123667,19.8767473168803,-1.60571548174355));
#38400=CARTESIAN_POINT('Ctrl Pts',(-0.800609992034415,19.8746447210675,
-1.669201892475));
#38401=CARTESIAN_POINT('Ctrl Pts',(-0.112656412660023,19.8739243721948,
-1.69383231167287));
#38402=CARTESIAN_POINT('Ctrl Pts',(0.532982300318684,19.8742602839387,-1.68192711531958));
#38403=CARTESIAN_POINT('Ctrl Pts',(1.11313112322414,19.8755170697086,-1.64255726795672));
#38404=CARTESIAN_POINT('Ctrl Pts',(1.62709005453795,19.877467053974,-1.58523245452894));
#38405=CARTESIAN_POINT('Ctrl Pts',(2.0850410197713,19.879899708692,-1.51643993262755));
#38406=CARTESIAN_POINT('Ctrl Pts',(2.49719897995038,19.8826728584564,-1.44015860157243));
#38407=CARTESIAN_POINT('Ctrl Pts',(2.86896944957029,19.8856601881407,-1.3596538028365));
#38408=CARTESIAN_POINT('Ctrl Pts',(3.20400785789159,19.8887529453858,-1.27761408943195));
#38409=CARTESIAN_POINT('Ctrl Pts',(3.50665331445631,19.8918777347858,-1.19576758536166));
#38410=CARTESIAN_POINT('Ctrl Pts',(3.78030901488711,19.8949775130325,-1.11543015088615));
#38411=CARTESIAN_POINT('Ctrl Pts',(4.02759771536219,19.8980059766931,-1.03765922725837));
#38412=CARTESIAN_POINT('Ctrl Pts',(4.25084657576043,19.9009285722717,-0.963229152083871));
#38413=CARTESIAN_POINT('Ctrl Pts',(4.45239467788257,19.9037239882921,-0.892594428082047));
#38414=CARTESIAN_POINT('Ctrl Pts',(4.63458237839232,19.906382426305,-0.825934929847175));
#38415=CARTESIAN_POINT('Ctrl Pts',(4.79971278148409,19.9089035013971,-0.763209477131803));
#38416=CARTESIAN_POINT('Ctrl Pts',(4.95001237258897,19.9112941678028,-0.704208461835124));
#38417=CARTESIAN_POINT('Ctrl Pts',(5.08753268224754,19.9135658129625,-0.648627094581878));
#38418=CARTESIAN_POINT('Ctrl Pts',(5.21386523151555,19.91572803623,-0.596217728895906));
#38419=CARTESIAN_POINT('Ctrl Pts',(5.33009497902457,19.9177858223623,-0.546853050922317));
#38420=CARTESIAN_POINT('Ctrl Pts',(5.43691796903193,19.9197398262928,-0.500510803643336));
#38421=CARTESIAN_POINT('Ctrl Pts',(5.53496769045484,19.9215912808168,-0.45715085370538));
#38422=CARTESIAN_POINT('Ctrl Pts',(5.62488345972163,19.9233429282228,-0.416691214874567));
#38423=CARTESIAN_POINT('Ctrl Pts',(5.70730743311051,19.9249987349898,-0.379013427036684));
#38424=CARTESIAN_POINT('Ctrl Pts',(5.76887172110402,19.9262734719378,-0.350464812380915));
#38425=CARTESIAN_POINT('Ctrl Pts',(5.80303600827932,19.9269958842689,-0.334474531192277));
#38426=CARTESIAN_POINT('Ctrl Pts',(5.81211556025371,19.9271889622373,-0.33021448364458));
#38427=CARTESIAN_POINT('Ctrl Pts',(-5.75637626238554,19.9977626186407,-0.213433499454596));
#38428=CARTESIAN_POINT('Ctrl Pts',(-5.7212417718798,19.9970541325727,-0.229942253987645));
#38429=CARTESIAN_POINT('Ctrl Pts',(-5.60419197539908,19.9947462888451,-0.284416335532265));
#38430=CARTESIAN_POINT('Ctrl Pts',(-5.39580847215891,19.9909174917254,-0.378306544937947));
#38431=CARTESIAN_POINT('Ctrl Pts',(-5.12142638369196,19.9862857505659,-0.496002143975811));
#38432=CARTESIAN_POINT('Ctrl Pts',(-4.8178161221067,19.9815661749843,-0.619044934882558));
#38433=CARTESIAN_POINT('Ctrl Pts',(-4.481360887937,19.9767689878634,-0.746638039711335));
#38434=CARTESIAN_POINT('Ctrl Pts',(-4.10654736969162,19.9719161036614,-0.87797019257089));
#38435=CARTESIAN_POINT('Ctrl Pts',(-3.68708854782038,19.9670669413926,-1.01144932738823));
#38436=CARTESIAN_POINT('Ctrl Pts',(-3.21779412718355,19.9623459099046,-1.1438596304457));
#38437=CARTESIAN_POINT('Ctrl Pts',(-2.69468813599392,19.9579377644809,-1.27035675133342));
#38438=CARTESIAN_POINT('Ctrl Pts',(-2.11308889877294,19.9540643078892,-1.38493050567701));
#38439=CARTESIAN_POINT('Ctrl Pts',(-1.47241765951857,19.9510122177396,-1.47924769932181));
#38440=CARTESIAN_POINT('Ctrl Pts',(-0.792400884528206,19.9491077370756,
-1.54219437673271));
#38441=CARTESIAN_POINT('Ctrl Pts',(-0.111506716483079,19.9484625525284,
-1.56661453768189));
#38442=CARTESIAN_POINT('Ctrl Pts',(0.527523869576598,19.948762395745,-1.55481091008629));
#38443=CARTESIAN_POINT('Ctrl Pts',(1.10171891950028,19.9498970382524,-1.51577665579069));
#38444=CARTESIAN_POINT('Ctrl Pts',(1.61044309412579,19.9516678974757,-1.45893642895713));
#38445=CARTESIAN_POINT('Ctrl Pts',(2.06377799643965,19.9538858627256,-1.39071843856522));
#38446=CARTESIAN_POINT('Ctrl Pts',(2.47183506989037,19.9564223371013,-1.3150651958254));
#38447=CARTESIAN_POINT('Ctrl Pts',(2.83995875855444,19.9591620892954,-1.23521318151454));
#38448=CARTESIAN_POINT('Ctrl Pts',(3.17175878038245,19.9620052196594,-1.15382839085906));
#38449=CARTESIAN_POINT('Ctrl Pts',(3.47152170739744,19.9648838525479,-1.07262526292338));
#38450=CARTESIAN_POINT('Ctrl Pts',(3.7426081303752,19.9677449142739,-0.992910001342112));
#38451=CARTESIAN_POINT('Ctrl Pts',(3.98760666100855,19.9705450649456,-0.915732946242152));
#38452=CARTESIAN_POINT('Ctrl Pts',(4.2088142491485,19.9732517129216,-0.841863855998557));
#38453=CARTESIAN_POINT('Ctrl Pts',(4.40854095596942,19.9758444804241,-0.77175523749468));
#38454=CARTESIAN_POINT('Ctrl Pts',(4.58909944991268,19.9783136764285,-0.70558703477212));
#38455=CARTESIAN_POINT('Ctrl Pts',(4.75276676013221,19.9806584016385,-0.643319687295874));
#38456=CARTESIAN_POINT('Ctrl Pts',(4.90174511909547,19.9828846554531,-0.584746306565457));
#38457=CARTESIAN_POINT('Ctrl Pts',(5.03806430897381,19.9850026522142,-0.529565368061844));
#38458=CARTESIAN_POINT('Ctrl Pts',(5.16329886931378,19.9870210227378,-0.477531953599395));
#38459=CARTESIAN_POINT('Ctrl Pts',(5.27852170418822,19.9889441474,-0.428520527235538));
#38460=CARTESIAN_POINT('Ctrl Pts',(5.38442057514526,19.9907723867053,-0.382509782879185));
#38461=CARTESIAN_POINT('Ctrl Pts',(5.48162162183854,19.9925066527352,-0.339460568099564));
#38462=CARTESIAN_POINT('Ctrl Pts',(5.57075720614196,19.9941492809222,-0.299292035622142));
#38463=CARTESIAN_POINT('Ctrl Pts',(5.6524630478063,19.995703765092,-0.261886921501083));
#38464=CARTESIAN_POINT('Ctrl Pts',(5.71348822196319,19.9969018117002,-0.233546326127602));
#38465=CARTESIAN_POINT('Ctrl Pts',(5.74735238456856,19.9975812837714,-0.21767305554885));
#38466=CARTESIAN_POINT('Ctrl Pts',(5.75635212916742,19.9977629229845,-0.213444206476439));
#38467=CARTESIAN_POINT('Ctrl Pts',(-5.6941765526172,19.9936699861522,-0.0798130175051694));
#38468=CARTESIAN_POINT('Ctrl Pts',(-5.65936703869485,19.9930119793506,-0.0961689593110878));
#38469=CARTESIAN_POINT('Ctrl Pts',(-5.54339967720871,19.9908709134695,-0.150138978145752));
#38470=CARTESIAN_POINT('Ctrl Pts',(-5.33694689369395,19.9873310897129,-0.243159156179306));
#38471=CARTESIAN_POINT('Ctrl Pts',(-5.06513642185539,19.9830664095691,-0.359752329638969));
#38472=CARTESIAN_POINT('Ctrl Pts',(-4.76442569368369,19.9787373930848,-0.48162174086261));
#38473=CARTESIAN_POINT('Ctrl Pts',(-4.4312589705187,19.9743535227251,-0.607970698079695));
#38474=CARTESIAN_POINT('Ctrl Pts',(-4.06020584530988,19.9699355319591,-0.737989586497756));
#38475=CARTESIAN_POINT('Ctrl Pts',(-3.64507557260789,19.9655385839926,-0.870097139656122));
#38476=CARTESIAN_POINT('Ctrl Pts',(-3.18076844297609,19.9612764317549,-1.0011075155669));
#38477=CARTESIAN_POINT('Ctrl Pts',(-2.66338764491666,19.957315974944,-1.12622841344135));
#38478=CARTESIAN_POINT('Ctrl Pts',(-2.08833386770721,19.9538550859021,-1.23952129169351));
#38479=CARTESIAN_POINT('Ctrl Pts',(-1.45505107682955,19.9511463329486,-1.33275847014169));
#38480=CARTESIAN_POINT('Ctrl Pts',(-0.783022235597851,19.9494710713447,
-1.39497134133894));
#38481=CARTESIAN_POINT('Ctrl Pts',(-0.110188903088729,19.9489129492212,
-1.41910487080894));
#38482=CARTESIAN_POINT('Ctrl Pts',(0.521281123261986,19.9491710061186,-1.40743979693122));
#38483=CARTESIAN_POINT('Ctrl Pts',(1.08869926737483,19.950164268464,-1.3688622122969));
#38484=CARTESIAN_POINT('Ctrl Pts',(1.59148386677679,19.9517279966345,-1.31268020141381));
#38485=CARTESIAN_POINT('Ctrl Pts',(2.03960018331289,19.9536979748251,-1.24524120709786));
#38486=CARTESIAN_POINT('Ctrl Pts',(2.44303760720881,19.9559613841007,-1.17043793420388));
#38487=CARTESIAN_POINT('Ctrl Pts',(2.80706804720489,19.9584158367489,-1.09146748105984));
#38488=CARTESIAN_POINT('Ctrl Pts',(3.13524621669758,19.9609716532087,-1.01096521360529));
#38489=CARTESIAN_POINT('Ctrl Pts',(3.4317966606742,19.9635673037228,-0.930627086505941));
#38490=CARTESIAN_POINT('Ctrl Pts',(3.70002963338188,19.9661542544967,-0.851746359874953));
#38491=CARTESIAN_POINT('Ctrl Pts',(3.94249333603436,19.9686925339578,-0.775363949415814));
#38492=CARTESIAN_POINT('Ctrl Pts',(4.16144912038774,19.9711517597429,-0.702243626244488));
#38493=CARTESIAN_POINT('Ctrl Pts',(4.35917319283947,19.9735125811614,-0.632835389747046));
#38494=CARTESIAN_POINT('Ctrl Pts',(4.53794624447846,19.975765389239,-0.567319428639144));
#38495=CARTESIAN_POINT('Ctrl Pts',(4.70001547858408,19.977908659644,-0.505658465160906));
#38496=CARTESIAN_POINT('Ctrl Pts',(4.84755564240826,19.9799472694527,-0.447649311946973));
#38497=CARTESIAN_POINT('Ctrl Pts',(4.9825720787926,19.9818900683868,-0.392994812681759));
#38498=CARTESIAN_POINT('Ctrl Pts',(5.10662033523709,19.9837445626203,-0.341453653044119));
#38499=CARTESIAN_POINT('Ctrl Pts',(5.22075984776193,19.985514427777,-0.292902611947154));
#38500=CARTESIAN_POINT('Ctrl Pts',(5.32566908184073,19.9871996753446,-0.247321606171754));
#38501=CARTESIAN_POINT('Ctrl Pts',(5.42196592776049,19.9888008400244,-0.204672761471427));
#38502=CARTESIAN_POINT('Ctrl Pts',(5.51027491707437,19.9903197826892,-0.164876756608036));
#38503=CARTESIAN_POINT('Ctrl Pts',(5.59122442533177,19.9917594473338,-0.127818010509195));
#38504=CARTESIAN_POINT('Ctrl Pts',(5.65168521434086,19.9928706910276,-0.0997396726106242));
#38505=CARTESIAN_POINT('Ctrl Pts',(5.68523639400912,19.9935015994509,-0.0840132164337404));
#38506=CARTESIAN_POINT('Ctrl Pts',(5.69415298771922,19.9936703044405,-0.0798234694406676));
#38507=CARTESIAN_POINT('',(5.73644274981185,19.8089495938061,-0.442545696631703));
#38508=CARTESIAN_POINT('Origin',(5.599999999773,19.5919343767575,-0.135488061233534));
#38509=CARTESIAN_POINT('Ctrl Pts',(-5.73644387793648,19.8089519016389,-0.442549068206594));
#38510=CARTESIAN_POINT('Ctrl Pts',(-5.66411038116652,19.8074370301077,-0.475761118065655));
#38511=CARTESIAN_POINT('Ctrl Pts',(-5.58548128839259,19.8058476858851,-0.511218926975151));
#38512=CARTESIAN_POINT('Ctrl Pts',(-5.50055659799522,19.8041980383931,-0.548567703824968));
#38513=CARTESIAN_POINT('Ctrl Pts',(-5.41741953789741,19.8025831153119,-0.585130304065416));
#38514=CARTESIAN_POINT('Ctrl Pts',(-5.32824913024332,19.8009104082698,-0.623504915458204));
#38515=CARTESIAN_POINT('Ctrl Pts',(-5.23304537351361,19.7991952410186,-0.663306060482758));
#38516=CARTESIAN_POINT('Ctrl Pts',(-5.13477098041616,19.7974247539447,-0.704390924213256));
#38517=CARTESIAN_POINT('Ctrl Pts',(-5.03006777092705,19.7956090117501,-0.746996132649766));
#38518=CARTESIAN_POINT('Ctrl Pts',(-4.91893574337511,19.7937671147615,-0.790639464683737));
#38519=CARTESIAN_POINT('Ctrl Pts',(-4.80780371582317,19.7919252177729,-0.834282796717708));
#38520=CARTESIAN_POINT('Ctrl Pts',(-4.69024287020841,19.7900571657752,-0.878964256165504));
#38521=CARTESIAN_POINT('Ctrl Pts',(-4.56625320485967,19.7881843424896,-0.924142417267869));
#38522=CARTESIAN_POINT('Ctrl Pts',(-4.44622763757178,19.7863713956069,-0.967876178465492));
#38523=CARTESIAN_POINT('Ctrl Pts',(-4.32017775547907,19.7845539889092,-1.01207510056595));
#38524=CARTESIAN_POINT('Ctrl Pts',(-4.18810355858154,19.7827535621543,-1.05619514264032));
#38525=CARTESIAN_POINT('Ctrl Pts',(-4.05161769976433,19.7808929959147,-1.10178892231133));
#38526=CARTESIAN_POINT('Ctrl Pts',(-3.90869834525198,19.7790505502845,-1.14729878417172));
#38527=CARTESIAN_POINT('Ctrl Pts',(-3.75934549504447,19.7772521459655,-1.19206586482418));
#38528=CARTESIAN_POINT('Ctrl Pts',(-3.60999264483696,19.7754537416466,-1.23683294547664));
#38529=CARTESIAN_POINT('Ctrl Pts',(-3.45420629893429,19.7736993780091,-1.28085725073673));
#38530=CARTESIAN_POINT('Ctrl Pts',(-3.29198645733648,19.7720172810933,-1.32342041175998));
#38531=CARTESIAN_POINT('Ctrl Pts',(-3.2117504477056,19.7711852944324,-1.34447269589578));
#38532=CARTESIAN_POINT('Ctrl Pts',(-3.12994053610347,19.7703710227783,-1.36516660608575));
#38533=CARTESIAN_POINT('Ctrl Pts',(-3.04655672721603,19.7695781056132,-1.38540981940204));
#38534=CARTESIAN_POINT('Ctrl Pts',(-3.00486482277231,19.7691816470307,-1.39553142606018));
#38535=CARTESIAN_POINT('Ctrl Pts',(-2.96277943528041,19.7687905034135,-1.40554032113933));
#38536=CARTESIAN_POINT('Ctrl Pts',(-2.92030057599748,19.7684051737507,-1.41542460742403));
#38537=CARTESIAN_POINT('Ctrl Pts',(-2.89906114635602,19.7682125089192,-1.42036675056638));
#38538=CARTESIAN_POINT('Ctrl Pts',(-2.87772334819987,19.7680212960993,-1.42527773918684));
#38539=CARTESIAN_POINT('Ctrl Pts',(-2.85628718138127,19.7678315939691,-1.43015606844165));
#38540=CARTESIAN_POINT('Ctrl Pts',(-2.84556909797198,19.767736742904,-1.43259523306906));
#38541=CARTESIAN_POINT('Ctrl Pts',(-2.83482642236462,19.7676422694187,-1.43502623270797));
#38542=CARTESIAN_POINT('Ctrl Pts',(-2.82405915455031,19.7675481809229,-1.43744887792669));
#38543=CARTESIAN_POINT('Ctrl Pts',(-2.81867552064316,19.767501136675,-1.43866020053605));
#38544=CARTESIAN_POINT('Ctrl Pts',(-2.81328573868226,19.7674541886688,-1.43986943453117));
#38545=CARTESIAN_POINT('Ctrl Pts',(-2.80788980866765,19.767407337837,-1.44107655614885));
#38546=CARTESIAN_POINT('Ctrl Pts',(-2.80249387865305,19.7673604870052,-1.44228367776654));
#38547=CARTESIAN_POINT('Ctrl Pts',(-2.79531884999955,19.7672984384957,-1.44388301861298));
#38548=CARTESIAN_POINT('Ctrl Pts',(-2.79168357445871,19.7672670777872,-1.44469156006093));
#38549=CARTESIAN_POINT('Ctrl Pts',(-2.04577401164782,19.7608322829147,-1.61059337167776));
#38550=CARTESIAN_POINT('Ctrl Pts',(-1.29987675980753,19.7571533928382,-1.7099242373575));
#38551=CARTESIAN_POINT('Ctrl Pts',(-0.553962218243579,19.756216688384,-1.7426513167991));
#38552=CARTESIAN_POINT('Ctrl Pts',(-0.369309354733381,19.755984805038,-1.75075298072503));
#38553=CARTESIAN_POINT('Ctrl Pts',(-0.18465543167186,19.7559210302059,-1.75477277944571));
#38554=CARTESIAN_POINT('Ctrl Pts',(-6.23933593455217E-13,19.7560252781079,
-1.75470973806164));
#38555=CARTESIAN_POINT('Ctrl Pts',(6.9346062000257E-5,19.7560253172575,
-1.75470971438689));
#38556=CARTESIAN_POINT('Ctrl Pts',(0.000138692124836583,19.7560253564308,
-1.75470969013632));
#38557=CARTESIAN_POINT('Ctrl Pts',(0.000208038187885564,19.7560253956277,
-1.75470966530994));
#38558=CARTESIAN_POINT('Ctrl Pts',(0.465532887800232,19.7562884145047,-1.75454307569928));
#38559=CARTESIAN_POINT('Ctrl Pts',(0.93085773639074,19.7573599747505,-1.72860446382034));
#38560=CARTESIAN_POINT('Ctrl Pts',(1.39618258395941,19.7592421679926,-1.67690533849036));
#38561=CARTESIAN_POINT('Ctrl Pts',(1.62884500774375,19.7601832646136,-1.65105577582537));
#38562=CARTESIAN_POINT('Ctrl Pts',(1.86150743137938,19.761326885799,-1.6187664128127));
#38563=CARTESIAN_POINT('Ctrl Pts',(2.09416985350423,19.7626724911624,-1.58004068048147));
#38564=CARTESIAN_POINT('Ctrl Pts',(2.21050106456666,19.7633452938441,-1.56067781431586));
#38565=CARTESIAN_POINT('Ctrl Pts',(2.32683227716806,19.764068599484,-1.53970586697001));
#38566=CARTESIAN_POINT('Ctrl Pts',(2.44316348898894,19.7648422734326,-1.51712540449519));
#38567=CARTESIAN_POINT('Ctrl Pts',(2.50132909489938,19.7652291104069,-1.50583517325778));
#38568=CARTESIAN_POINT('Ctrl Pts',(2.55949470071762,19.7656285398986,-1.49414281395364));
#38569=CARTESIAN_POINT('Ctrl Pts',(2.61766030646164,19.766040544681,-1.48204840355164));
#38570=CARTESIAN_POINT('Ctrl Pts',(2.64674310933365,19.7662465470722,-1.47600119835064));
#38571=CARTESIAN_POINT('Ctrl Pts',(2.67582591219613,19.7664556933134,-1.46985348041873));
#38572=CARTESIAN_POINT('Ctrl Pts',(2.70490871505082,19.7666679810471,-1.46360525988021));
#38573=CARTESIAN_POINT('Ctrl Pts',(2.7321738427271,19.7668670007974,-1.45774755312535));
#38574=CARTESIAN_POINT('Ctrl Pts',(2.75943897039682,19.7670687816261,-1.45180151400297));
#38575=CARTESIAN_POINT('Ctrl Pts',(2.78670409806629,19.7672733215177,-1.4457671511001));
#38576=CARTESIAN_POINT('Ctrl Pts',(2.78852177324425,19.7672869575105,-1.44536486023991));
#38577=CARTESIAN_POINT('Ctrl Pts',(2.79172178017481,19.7673109945109,-1.44465563983108));
#38578=CARTESIAN_POINT('Ctrl Pts',(2.79215712359993,19.7673142662813,-1.44455910087302));
#38579=CARTESIAN_POINT('Ctrl Pts',(2.80635022699111,19.7674209328201,-1.44141172954727));
#38580=CARTESIAN_POINT('Ctrl Pts',(2.82656863123274,19.7675848277377,-1.43690147673273));
#38581=CARTESIAN_POINT('Ctrl Pts',(2.85281233632482,19.7678094196818,-1.43094097946311));
#38582=CARTESIAN_POINT('Ctrl Pts',(2.87905633539835,19.7680340141419,-1.42498041542411));
#38583=CARTESIAN_POINT('Ctrl Pts',(2.91132577031368,19.7683193068042,-1.4175695743538));
#38584=CARTESIAN_POINT('Ctrl Pts',(2.9496206410708,19.7686708437388,-1.4085690016783));
#38585=CARTESIAN_POINT('Ctrl Pts',(2.98791596514066,19.7690223848347,-1.39956832245917));
#38586=CARTESIAN_POINT('Ctrl Pts',(3.03223686770447,19.7694401714784,-1.38897787390266));
#38587=CARTESIAN_POINT('Ctrl Pts',(3.08258334876223,19.7699318308584,-1.37660610821271));
#38588=CARTESIAN_POINT('Ctrl Pts',(3.13293081631026,19.7704234998721,-1.36423410011007));
#38589=CARTESIAN_POINT('Ctrl Pts',(3.18930409848524,19.7709890441134,-1.35008070502378));
#38590=CARTESIAN_POINT('Ctrl Pts',(3.25170319528717,19.771638177437,-1.33390227483369));
#38591=CARTESIAN_POINT('Ctrl Pts',(3.31410299699454,19.7722873180937,-1.31772366188033));
#38592=CARTESIAN_POINT('Ctrl Pts',(3.38252874947358,19.7730200492131,-1.29951996794108));
#38593=CARTESIAN_POINT('Ctrl Pts',(3.45698045272428,19.7738481780564,-1.27899544831037));
#38594=CARTESIAN_POINT('Ctrl Pts',(3.53143357438562,19.7746763226767,-1.25847053765842));
#38595=CARTESIAN_POINT('Ctrl Pts',(3.61191287642663,19.7755998680385,-1.23562471280952));
#38596=CARTESIAN_POINT('Ctrl Pts',(3.69841835884734,19.7766327236699,-1.21011012356596));
#38597=CARTESIAN_POINT('Ctrl Pts',(3.77371782358943,19.7775317820188,-1.18790072296623));
#38598=CARTESIAN_POINT('Ctrl Pts',(3.85358331706806,19.7785136964691,-1.16366840616151));
#38599=CARTESIAN_POINT('Ctrl Pts',(3.93801483928324,19.779588943194,-1.13715162237394));
#38600=CARTESIAN_POINT('Ctrl Pts',(3.98561399760912,19.7801951248399,-1.12220250672752));
#38601=CARTESIAN_POINT('Ctrl Pts',(4.03466435815191,19.7808309918418,-1.10652678805407));
#38602=CARTESIAN_POINT('Ctrl Pts',(4.08516592649798,19.781498604142,-1.09007340331406));
#38603=CARTESIAN_POINT('Ctrl Pts',(4.11041671067101,19.7818324102921,-1.08184671094406));
#38604=CARTESIAN_POINT('Ctrl Pts',(4.13603028724608,19.7821741330792,-1.0734255721268));
#38605=CARTESIAN_POINT('Ctrl Pts',(4.16200666832599,19.7825240675577,-1.06480330014664));
#38606=CARTESIAN_POINT('Ctrl Pts',(4.17499485886595,19.782699034797,-1.06049216415656));
#38607=CARTESIAN_POINT('Ctrl Pts',(4.1880737499445,19.7828760537271,-1.05613074299689));
#38608=CARTESIAN_POINT('Ctrl Pts',(4.20124334141254,19.7830551581622,-1.05171818614679));
#38609=CARTESIAN_POINT('Ctrl Pts',(4.20782813714656,19.7831447103797,-1.04951190772174));
#38610=CARTESIAN_POINT('Ctrl Pts',(4.21443560793993,19.7832347838967,-1.04729284525787));
#38611=CARTESIAN_POINT('Ctrl Pts',(4.22106575379413,19.7833253830315,-1.04506089129743));
#38612=CARTESIAN_POINT('Ctrl Pts',(4.22769589964832,19.7834159821662,-1.04282893733699));
#38613=CARTESIAN_POINT('Ctrl Pts',(4.23593743769457,19.7835289199598,-1.04004674200915));
#38614=CARTESIAN_POINT('Ctrl Pts',(4.24102421646306,19.7835987614664,-1.03832624687006));
#38615=CARTESIAN_POINT('Ctrl Pts',(4.3703949931502,19.7853750230971,-0.994569322780967));
#38616=CARTESIAN_POINT('Ctrl Pts',(4.49373991369497,19.7871644677347,-0.950843620817392));
#38617=CARTESIAN_POINT('Ctrl Pts',(4.61105897939592,19.7889461132073,-0.907681610185909));
#38618=CARTESIAN_POINT('Ctrl Pts',(4.72934236291549,19.7907424031239,-0.864164824346399));
#38619=CARTESIAN_POINT('Ctrl Pts',(4.84150042403069,19.7925307626914,-0.821221103354181));
#38620=CARTESIAN_POINT('Ctrl Pts',(4.94753316407235,19.7942917588281,-0.779342573722851));
#38621=CARTESIAN_POINT('Ctrl Pts',(5.05275827019582,19.7960393417472,-0.737783025954676));
#38622=CARTESIAN_POINT('Ctrl Pts',(5.15195101100168,19.7977599793199,-0.697272434259096));
#38623=CARTESIAN_POINT('Ctrl Pts',(5.24511138779057,19.7994366989643,-0.658239440062828));
#38624=CARTESIAN_POINT('Ctrl Pts',(5.33934431488943,19.80113272259,-0.618757061144568));
#38625=CARTESIAN_POINT('Ctrl Pts',(5.42740517784177,19.8027838073779,-0.580786598554457));
#38626=CARTESIAN_POINT('Ctrl Pts',(5.50929397799366,19.8043744792903,-0.544717460517054));
#38627=CARTESIAN_POINT('Ctrl Pts',(5.59118277814556,19.8059651512028,-0.508648322479651));
#38628=CARTESIAN_POINT('Ctrl Pts',(5.66689951549702,19.8074954102507,-0.474480506728332));
#38629=CARTESIAN_POINT('Ctrl Pts',(5.73644419139414,19.8089518848421,-0.442548940794832));
#38630=CARTESIAN_POINT('Origin',(5.6,19.5919343769583,-0.135488060981343));
#38631=CARTESIAN_POINT('Origin',(5.59997427808526,19.5919309020823,-0.135464036534198));
#38632=CARTESIAN_POINT('Ctrl Pts',(5.71189864452985,10.3747304895651,-1.73098436839218));
#38633=CARTESIAN_POINT('Ctrl Pts',(5.71686764344326,10.3731922894021,-1.72895290465319));
#38634=CARTESIAN_POINT('Ctrl Pts',(5.76414615685762,10.3586634212538,-1.70873769602088));
#38635=CARTESIAN_POINT('Ctrl Pts',(5.84912002164699,10.334482886934,-1.65630729766632));
#38636=CARTESIAN_POINT('Ctrl Pts',(5.94753982152578,10.3114454163772,-1.5531434815364));
#38637=CARTESIAN_POINT('Ctrl Pts',(6.01568051672699,10.3011442171297,-1.43300892716969));
#38638=CARTESIAN_POINT('Ctrl Pts',(6.04717587912082,10.3030528288475,-1.32055362605887));
#38639=CARTESIAN_POINT('Ctrl Pts',(6.05143244177369,10.3095932145156,-1.25273304586632));
#38640=CARTESIAN_POINT('Ctrl Pts',(6.05078104094871,10.3130207230613,-1.22619796391761));
#38641=CARTESIAN_POINT('Ctrl Pts',(5.59579998485702,10.091096172154,-1.65481746119893));
#38642=CARTESIAN_POINT('Ctrl Pts',(5.60043595614829,10.0896504255744,-1.65294937270293));
#38643=CARTESIAN_POINT('Ctrl Pts',(5.64455259774951,10.0759868560455,-1.63435926048869));
#38644=CARTESIAN_POINT('Ctrl Pts',(5.72395137359632,10.0531092099547,-1.58612351386667));
#38645=CARTESIAN_POINT('Ctrl Pts',(5.81591850580226,10.0310626434678,-1.49126508712223));
#38646=CARTESIAN_POINT('Ctrl Pts',(5.87943865664269,10.0209345533178,-1.38113253481707));
#38647=CARTESIAN_POINT('Ctrl Pts',(5.90862955872158,10.022319989054,-1.27866217141058));
#38648=CARTESIAN_POINT('Ctrl Pts',(5.91253312848719,10.0281804213171,-1.2173831667632));
#38649=CARTESIAN_POINT('Ctrl Pts',(5.91193519380811,10.0312728279379,-1.19350825632173));
#38650=CARTESIAN_POINT('Ctrl Pts',(5.57863052428272,9.8189813716046,-1.81415344748554));
#38651=CARTESIAN_POINT('Ctrl Pts',(5.58522332651264,9.8169636961234,-1.81151876117067));
#38652=CARTESIAN_POINT('Ctrl Pts',(5.64790096319949,9.79793300371442,-1.78533019096301));
#38653=CARTESIAN_POINT('Ctrl Pts',(5.7597437862497,9.76669738257529,-1.71797544780278));
#38654=CARTESIAN_POINT('Ctrl Pts',(5.88924968067551,9.73729923170353,-1.58603258316671));
#38655=CARTESIAN_POINT('Ctrl Pts',(5.98006036132214,9.72422746393119,-1.43101993105616));
#38656=CARTESIAN_POINT('Ctrl Pts',(6.02329964904305,9.72688955971414,-1.28255723102518));
#38657=CARTESIAN_POINT('Ctrl Pts',(6.02945491177813,9.73581061263325,-1.19002012260145));
#38658=CARTESIAN_POINT('Ctrl Pts',(6.02851709775331,9.74055796418653,-1.15322141602788));
#38659=CARTESIAN_POINT('Ctrl Pts',(5.6716461590008,9.73678026104202,-2.10453384239488));
#38660=CARTESIAN_POINT('Ctrl Pts',(5.68120278004111,9.73390122266715,-2.10070515593161));
#38661=CARTESIAN_POINT('Ctrl Pts',(5.77199595282922,9.70678959567008,-2.06267601536369));
#38662=CARTESIAN_POINT('Ctrl Pts',(5.93303210065318,9.66301450628333,-1.96542277239424));
#38663=CARTESIAN_POINT('Ctrl Pts',(6.11945830548874,9.62274187697619,-1.775317678271));
#38664=CARTESIAN_POINT('Ctrl Pts',(6.25157930475856,9.60553947784097,-1.54996558636508));
#38665=CARTESIAN_POINT('Ctrl Pts',(6.31600990124635,9.61044110901839,-1.32968520371137));
#38666=CARTESIAN_POINT('Ctrl Pts',(6.32554536478181,9.62415685682377,-1.18858268459059));
#38667=CARTESIAN_POINT('Ctrl Pts',(6.32409714600594,9.63146424160204,-1.13174887283082));
#38668=CARTESIAN_POINT('',(5.99998739574847,10.093342129965,-1.21103206229897));
#38669=CARTESIAN_POINT('',(5.99999998791408,9.6543882121161,-1.86247524004434));
#38670=CARTESIAN_POINT('Ctrl Pts',(5.99998739574847,10.093342129965,-1.21103206229897));
#38671=CARTESIAN_POINT('Ctrl Pts',(5.99998525070341,10.0742059844227,-1.2256251864801));
#38672=CARTESIAN_POINT('Ctrl Pts',(5.99998676083935,10.0554326526012,-1.24054794704701));
#38673=CARTESIAN_POINT('Ctrl Pts',(5.99999979829476,10.03713808821,-1.25580697991203));
#38674=CARTESIAN_POINT('Ctrl Pts',(6.00000674487255,10.02739043343,-1.26393725191334));
#38675=CARTESIAN_POINT('Ctrl Pts',(6.00001622859838,10.0177786906484,-1.27216235989735));
#38676=CARTESIAN_POINT('Ctrl Pts',(6.00002591477378,10.0083195677745,-1.28047856190009));
#38677=CARTESIAN_POINT('Ctrl Pts',(6.00004505453792,9.98962845664022,-1.29691127536836));
#38678=CARTESIAN_POINT('Ctrl Pts',(6.00006657199182,9.97153445157826,-1.31370242007807));
#38679=CARTESIAN_POINT('Ctrl Pts',(6.00008776273575,9.95414192720689,-1.33079292037839));
#38680=CARTESIAN_POINT('Ctrl Pts',(6.00010095957137,9.94331048656118,-1.3414362712604));
#38681=CARTESIAN_POINT('Ctrl Pts',(6.00011344452304,9.93275077675863,-1.35219475564079));
#38682=CARTESIAN_POINT('Ctrl Pts',(6.00012222699497,9.92248320775588,-1.36304548041424));
#38683=CARTESIAN_POINT('Ctrl Pts',(6.00013667465114,9.90559248408776,-1.38089552784979));
#38684=CARTESIAN_POINT('Ctrl Pts',(6.00013999561394,9.88949456201145,-1.39899690728196));
#38685=CARTESIAN_POINT('Ctrl Pts',(6.00012430276381,9.87425199476169,-1.41721620450256));
#38686=CARTESIAN_POINT('Ctrl Pts',(6.00011929886963,9.86939167985008,-1.42302569318705));
#38687=CARTESIAN_POINT('Ctrl Pts',(6.0001124735993,9.86461804279409,-1.42884691741494));
#38688=CARTESIAN_POINT('Ctrl Pts',(6.00010395684403,9.85993227951363,-1.43467492541273));
#38689=CARTESIAN_POINT('Ctrl Pts',(6.00009905090812,9.85723312312927,-1.43803205296138));
#38690=CARTESIAN_POINT('Ctrl Pts',(6.00009358871496,9.85456311662419,-1.44139142719417));
#38691=CARTESIAN_POINT('Ctrl Pts',(6.0000876867648,9.85192240584083,-1.44475212813161));
#38692=CARTESIAN_POINT('Ctrl Pts',(6.00006914832814,9.84362774927567,-1.4553083239369));
#38693=CARTESIAN_POINT('Ctrl Pts',(6.00005144090386,9.83550486511725,-1.46601891242109));
#38694=CARTESIAN_POINT('Ctrl Pts',(6.00003089267563,9.82769828562318,-1.47670035842532));
#38695=CARTESIAN_POINT('Ctrl Pts',(6.0000101584876,9.81982105722095,-1.48747847064532));
#38696=CARTESIAN_POINT('Ctrl Pts',(5.99998607983893,9.81226624915332,-1.49822652985124));
#38697=CARTESIAN_POINT('Ctrl Pts',(5.99996800047488,9.80514747283832,-1.50871702540345));
#38698=CARTESIAN_POINT('Ctrl Pts',(5.99995733483965,9.80094786320285,-1.51490572754164));
#38699=CARTESIAN_POINT('Ctrl Pts',(5.99994905280315,9.79689929622093,-1.52100407183462));
#38700=CARTESIAN_POINT('Ctrl Pts',(5.99994795704476,9.79301903904449,-1.52696018892455));
#38701=CARTESIAN_POINT('Ctrl Pts',(5.99994404418047,9.77916295551462,-1.54822899976853));
#38702=CARTESIAN_POINT('Ctrl Pts',(5.99996395741825,9.76602634289345,-1.57000915494076));
#38703=CARTESIAN_POINT('Ctrl Pts',(5.99998991543438,9.75374722793985,-1.59221159742656));
#38704=CARTESIAN_POINT('Ctrl Pts',(6.00001572479601,9.74153843214226,-1.61428689255501));
#38705=CARTESIAN_POINT('Ctrl Pts',(6.0000467928305,9.73017813382453,-1.6367791365723));
#38706=CARTESIAN_POINT('Ctrl Pts',(6.00006725086747,9.71977349236808,-1.65955800898032));
#38707=CARTESIAN_POINT('Ctrl Pts',(6.00007042537936,9.71815898468138,-1.66309264924169));
#38708=CARTESIAN_POINT('Ctrl Pts',(6.00007335936769,9.71656741865602,-1.66663411695046));
#38709=CARTESIAN_POINT('Ctrl Pts',(6.00007601305726,9.71499911544098,-1.67018184719024));
#38710=CARTESIAN_POINT('Ctrl Pts',(6.00009313187098,9.70488207278654,-1.69306807086057));
#38711=CARTESIAN_POINT('Ctrl Pts',(6.00009752578096,9.69573653071054,-1.71621725348646));
#38712=CARTESIAN_POINT('Ctrl Pts',(6.00008809970652,9.68762372022529,-1.739465193567));
#38713=CARTESIAN_POINT('Ctrl Pts',(6.00007855620972,9.67940984694546,-1.76300273757664));
#38714=CARTESIAN_POINT('Ctrl Pts',(6.00005445424126,9.67225489482556,-1.78664049911191));
#38715=CARTESIAN_POINT('Ctrl Pts',(6.00003199298379,9.66617590604954,-1.81018726837208));
#38716=CARTESIAN_POINT('Ctrl Pts',(6.00001529302277,9.66165617354125,-1.82769430817947));
#38717=CARTESIAN_POINT('Ctrl Pts',(5.99999988409118,9.65773020436411,-1.84515053404935));
#38718=CARTESIAN_POINT('Ctrl Pts',(5.99999988834942,9.65438801533234,-1.86247520208183));
#38719=CARTESIAN_POINT('',(5.72001530599109,9.72697688177551,-2.05943446844682));
#38720=CARTESIAN_POINT('Ctrl Pts',(5.72001583931905,9.72697824478347,-2.05943475704983));
#38721=CARTESIAN_POINT('Ctrl Pts',(5.77262443161298,9.71167221606504,-2.03450172317382));
#38722=CARTESIAN_POINT('Ctrl Pts',(5.82215801015693,9.69806914525657,-2.00535807896891));
#38723=CARTESIAN_POINT('Ctrl Pts',(5.86878812167555,9.68600522339526,-1.97246301336546));
#38724=CARTESIAN_POINT('Ctrl Pts',(5.91541823319418,9.67394130153395,-1.93956794776201));
#38725=CARTESIAN_POINT('Ctrl Pts',(5.95914511084698,9.66341708212426,-1.90292156494207));
#38726=CARTESIAN_POINT('Ctrl Pts',(6.00000005305837,9.65438841513202,-1.86247527920915));
#38727=CARTESIAN_POINT('',(5.732785087834,10.3449543305438,-1.7128937574831));
#38728=CARTESIAN_POINT('Origin',(5.89877349632372,10.183812103656,-2.15616649229544));
#38729=CARTESIAN_POINT('Ctrl Pts',(5.73278241138339,10.3449569278259,-1.71288661549559));
#38730=CARTESIAN_POINT('Ctrl Pts',(5.74767875123649,10.3336216280175,-1.70318199341943));
#38731=CARTESIAN_POINT('Ctrl Pts',(5.76173634509441,10.322835658242,-1.69290604950805));
#38732=CARTESIAN_POINT('Ctrl Pts',(5.77495203195241,10.3125930760254,-1.68228739492388));
#38733=CARTESIAN_POINT('Ctrl Pts',(5.78903167351962,10.301680901132,-1.67097456252422));
#38734=CARTESIAN_POINT('Ctrl Pts',(5.80215588058894,10.291385530781,-1.65927245019434));
#38735=CARTESIAN_POINT('Ctrl Pts',(5.81434894340356,10.2816926135053,-1.64740640683436));
#38736=CARTESIAN_POINT('Ctrl Pts',(5.81704664373936,10.2795480673329,-1.64478105915564));
#38737=CARTESIAN_POINT('Ctrl Pts',(5.81969886131872,10.2774329841764,-1.64214751019764));
#38738=CARTESIAN_POINT('Ctrl Pts',(5.82230601802282,10.2753471622135,-1.63950791362413));
#38739=CARTESIAN_POINT('Ctrl Pts',(5.8343566194193,10.2657062346013,-1.6273073711309));
#38740=CARTESIAN_POINT('Ctrl Pts',(5.84544364851837,10.2566906065921,-1.61498183373302));
#38741=CARTESIAN_POINT('Ctrl Pts',(5.85563660028135,10.24826867085,-1.60274257496124));
#38742=CARTESIAN_POINT('Ctrl Pts',(5.85625540711629,10.2477573811351,-1.60199953828661));
#38743=CARTESIAN_POINT('Ctrl Pts',(5.85687092211076,10.247248278839,-1.60125680431862));
#38744=CARTESIAN_POINT('Ctrl Pts',(5.85748316207662,10.2467413566176,-1.60051441457763));
#38745=CARTESIAN_POINT('Ctrl Pts',(5.86845374327555,10.2376579388377,-1.58721171075426));
#38746=CARTESIAN_POINT('Ctrl Pts',(5.87837194703487,10.2292747699409,-1.57402408876206));
#38747=CARTESIAN_POINT('Ctrl Pts',(5.88734076941703,10.221548069533,-1.56115987641525));
#38748=CARTESIAN_POINT('Ctrl Pts',(5.89145118167163,10.2180069219118,-1.55526420652425));
#38749=CARTESIAN_POINT('Ctrl Pts',(5.8953623376495,10.2146036181259,-1.54943570552396));
#38750=CARTESIAN_POINT('Ctrl Pts',(5.89908478287728,10.2113337664291,-1.5436909432781));
#38751=CARTESIAN_POINT('Ctrl Pts',(5.90118655203684,10.2094875408886,-1.54044733232387));
#38752=CARTESIAN_POINT('Ctrl Pts',(5.9032281669301,10.2076838576228,-1.53723038063642));
#38753=CARTESIAN_POINT('Ctrl Pts',(5.90521156641127,10.2059219134952,-1.5340428035946));
#38754=CARTESIAN_POINT('Ctrl Pts',(5.90881699114517,10.2027190504322,-1.52824842418851));
#38755=CARTESIAN_POINT('Ctrl Pts',(5.91223007754269,10.1996540965837,-1.52255125712056));
#38756=CARTESIAN_POINT('Ctrl Pts',(5.91546374346187,10.1967216968648,-1.51696747377376));
#38757=CARTESIAN_POINT('Ctrl Pts',(5.91797002104723,10.1944489179598,-1.51263971964165));
#38758=CARTESIAN_POINT('Ctrl Pts',(5.92036844691872,10.1922557983517,-1.50838013033203));
#38759=CARTESIAN_POINT('Ctrl Pts',(5.92266499899361,10.1901398681883,-1.50419520066658));
#38760=CARTESIAN_POINT('Ctrl Pts',(5.92381327503106,10.1890819031065,-1.50210273583385));
#38761=CARTESIAN_POINT('Ctrl Pts',(5.9249360757642,10.188043237144,-1.5000289313888));
#38762=CARTESIAN_POINT('Ctrl Pts',(5.92603412788109,10.1870235727388,-1.49797454672763));
#38763=CARTESIAN_POINT('Ctrl Pts',(5.92680721492419,10.1863056748105,-1.49652815075182));
#38764=CARTESIAN_POINT('Ctrl Pts',(5.92725985652953,10.1858838464094,-1.49567455154667));
#38765=CARTESIAN_POINT('Ctrl Pts',(5.92804436251635,10.1851520674593,-1.49418301711905));
#38766=CARTESIAN_POINT('Ctrl Pts',(5.92837412751263,10.1848444661321,-1.49355605460602));
#38767=CARTESIAN_POINT('Ctrl Pts',(5.92876221211849,10.1844822288943,-1.49281615753072));
#38768=CARTESIAN_POINT('Ctrl Pts',(5.92925474683439,10.1840212904741,-1.49187038511312));
#38769=CARTESIAN_POINT('Ctrl Pts',(5.939199111107,10.1747148610788,-1.47277507033431));
#38770=CARTESIAN_POINT('Ctrl Pts',(5.94793617260916,10.1661689170949,-1.4536541603137));
#38771=CARTESIAN_POINT('Ctrl Pts',(5.95554256935783,10.1583490236111,-1.43472083832225));
#38772=CARTESIAN_POINT('Ctrl Pts',(5.95842928679405,10.1553812816414,-1.427535418928));
#38773=CARTESIAN_POINT('Ctrl Pts',(5.96115320544007,10.1525180805119,-1.42037646288496));
#38774=CARTESIAN_POINT('Ctrl Pts',(5.96371874216079,10.1497574026567,-1.413253735847));
#38775=CARTESIAN_POINT('Ctrl Pts',(5.97059811441644,10.1423547681552,-1.39415446107384));
#38776=CARTESIAN_POINT('Ctrl Pts',(5.97633958133714,10.1356890572738,-1.37531958504562));
#38777=CARTESIAN_POINT('Ctrl Pts',(5.98107332754243,10.1297035854556,-1.35693324828585));
#38778=CARTESIAN_POINT('Ctrl Pts',(5.98611100708851,10.1233338124166,-1.33736640447865));
#38779=CARTESIAN_POINT('Ctrl Pts',(5.99000695673524,10.1177345595621,-1.3183072745247));
#38780=CARTESIAN_POINT('Ctrl Pts',(5.99291128797468,10.1128388295157,-1.2999196848561));
#38781=CARTESIAN_POINT('Ctrl Pts',(5.99361898113252,10.1116458958002,-1.29543921402657));
#38782=CARTESIAN_POINT('Ctrl Pts',(5.99426778584006,10.1104947342988,-1.29099837052087));
#38783=CARTESIAN_POINT('Ctrl Pts',(5.99485986277889,10.1093843755169,-1.28659907171658));
#38784=CARTESIAN_POINT('Ctrl Pts',(5.99739682029324,10.1046266609859,-1.26774876117852));
#38785=CARTESIAN_POINT('Ctrl Pts',(5.99889426417414,10.100617369373,-1.24966510146631));
#38786=CARTESIAN_POINT('Ctrl Pts',(5.99956526156832,10.0972659791722,-1.23247198354656));
#38787=CARTESIAN_POINT('Ctrl Pts',(5.99985052298196,10.0958412012004,-1.22516266585727));
#38788=CARTESIAN_POINT('Ctrl Pts',(5.9999861332354,10.0945354314074,-1.21801369646564));
#38789=CARTESIAN_POINT('Ctrl Pts',(5.99998739574847,10.093342129965,-1.21103206229897));
#38790=CARTESIAN_POINT('Ctrl Pts',(5.99970218885082,10.0072537640941,-1.15840945237376));
#38791=CARTESIAN_POINT('Ctrl Pts',(5.99970218885082,10.4047340562143,-1.32642148281801));
#38792=CARTESIAN_POINT('Ctrl Pts',(5.99970218885082,11.3017776556714,-1.63820419624065));
#38793=CARTESIAN_POINT('Ctrl Pts',(5.99970218885082,12.7412413732199,-1.91712741021756));
#38794=CARTESIAN_POINT('Ctrl Pts',(5.99970218885082,14.2901880401604,-1.97136832589254));
#38795=CARTESIAN_POINT('Ctrl Pts',(5.99970218885082,15.8279955162323,-1.78467115077639));
#38796=CARTESIAN_POINT('Ctrl Pts',(5.99970218885082,17.3193006181559,-1.36141279701238));
#38797=CARTESIAN_POINT('Ctrl Pts',(5.99970218885082,18.6019975902749,-0.768446409410351));
#38798=CARTESIAN_POINT('Ctrl Pts',(5.99970218885082,19.3573547509784,-0.286407566908898));
#38799=CARTESIAN_POINT('Ctrl Pts',(5.99970218885082,19.6640972928094,-0.0649546759702413));
#38800=CARTESIAN_POINT('Ctrl Pts',(6.00690077665715,9.93465823492307,-1.33014020345178));
#38801=CARTESIAN_POINT('Ctrl Pts',(6.00690077665715,10.339650355467,-1.50132938399891));
#38802=CARTESIAN_POINT('Ctrl Pts',(6.00690077665715,11.2534797462814,-1.81894736376076));
#38803=CARTESIAN_POINT('Ctrl Pts',(6.00690077665715,12.7201657060177,-2.10314012549508));
#38804=CARTESIAN_POINT('Ctrl Pts',(6.00690077665715,14.2981396447801,-2.15840027503973));
#38805=CARTESIAN_POINT('Ctrl Pts',(6.00690077665715,15.8650159409265,-1.96817595341715));
#38806=CARTESIAN_POINT('Ctrl Pts',(6.00690077665715,17.3842794608967,-1.53697638991161));
#38807=CARTESIAN_POINT('Ctrl Pts',(6.00690077665715,18.6912061461468,-0.932814930207615));
#38808=CARTESIAN_POINT('Ctrl Pts',(6.00690077665715,19.4607068236737,-0.441751837926806));
#38809=CARTESIAN_POINT('Ctrl Pts',(6.00690077665715,19.7732356586246,-0.216119001381029));
#38810=CARTESIAN_POINT('Ctrl Pts',(5.89988022250419,9.87508958651989,-1.47105478659189));
#38811=CARTESIAN_POINT('Ctrl Pts',(5.89988022250419,10.286245577916,-1.64485099459073));
#38812=CARTESIAN_POINT('Ctrl Pts',(5.89988022250419,11.2138486392983,-1.96725713324961));
#38813=CARTESIAN_POINT('Ctrl Pts',(5.89988022250419,12.7028719549598,-2.25577385048283));
#38814=CARTESIAN_POINT('Ctrl Pts',(5.89988022250419,14.3046643763385,-2.31187033780927));
#38815=CARTESIAN_POINT('Ctrl Pts',(5.89988022250419,15.8953932477307,-2.11875179732357));
#38816=CARTESIAN_POINT('Ctrl Pts',(5.89988022250419,17.4375981966469,-1.68103603184313));
#38817=CARTESIAN_POINT('Ctrl Pts',(5.89988022250419,18.7644067021557,-1.06768839604758));
#38818=CARTESIAN_POINT('Ctrl Pts',(5.89988022250419,19.5455129178013,-0.569220407507801));
#38819=CARTESIAN_POINT('Ctrl Pts',(5.89988022250419,19.862789726409,-0.340157694318395));
#38820=CARTESIAN_POINT('Ctrl Pts',(5.72194811176411,9.85291204087539,-1.52351761197645));
#38821=CARTESIAN_POINT('Ctrl Pts',(5.72194811176411,10.2663628556535,-1.6982844223277));
#38822=CARTESIAN_POINT('Ctrl Pts',(5.72194811176411,11.199093886461,-2.02247320362448));
#38823=CARTESIAN_POINT('Ctrl Pts',(5.72194811176411,12.6964334514226,-2.31259973949581));
#38824=CARTESIAN_POINT('Ctrl Pts',(5.72194811176411,14.3070935489958,-2.36900759731379));
#38825=CARTESIAN_POINT('Ctrl Pts',(5.72194811176411,15.9067027893476,-2.17481153244808));
#38826=CARTESIAN_POINT('Ctrl Pts',(5.72194811176411,17.457448885353,-1.73466976989276));
#38827=CARTESIAN_POINT('Ctrl Pts',(5.72194811176411,18.7916594385481,-1.11790209948377));
#38828=CARTESIAN_POINT('Ctrl Pts',(5.72194811176411,19.5770864228865,-0.616677250928825));
#38829=CARTESIAN_POINT('Ctrl Pts',(5.72194811176411,19.8961309130786,-0.386337586725996));
#38830=CARTESIAN_POINT('Ctrl Pts',(5.73278343895284,10.3449559317257,-1.71288935416517));
#38831=CARTESIAN_POINT('Ctrl Pts',(5.73338951138606,10.6015227812206,-1.80593972809553));
#38832=CARTESIAN_POINT('Ctrl Pts',(5.73395354664378,10.8620214983833,-1.8889039136407));
#38833=CARTESIAN_POINT('Ctrl Pts',(5.73447555380531,11.1255734077639,-1.96144088568236));
#38834=CARTESIAN_POINT('Ctrl Pts',(5.73532470571528,11.5542947428651,-2.0794371755631));
#38835=CARTESIAN_POINT('Ctrl Pts',(5.73606264400881,11.9910976959887,-2.16984187011366));
#38836=CARTESIAN_POINT('Ctrl Pts',(5.73668942675903,12.4324355283466,-2.23165186408241));
#38837=CARTESIAN_POINT('Ctrl Pts',(5.73681690515044,12.5221971513587,-2.24422310762926));
#38838=CARTESIAN_POINT('Ctrl Pts',(5.7369397855595,12.612146198574,-2.25561146181761));
#38839=CARTESIAN_POINT('Ctrl Pts',(5.73705806849707,12.7022525780884,-2.26580840528823));
#38840=CARTESIAN_POINT('Ctrl Pts',(5.73707478430295,12.7149864582159,-2.26724944261013));
#38841=CARTESIAN_POINT('Ctrl Pts',(5.73709140829046,12.7277234803624,-2.26866668563992));
#38842=CARTESIAN_POINT('Ctrl Pts',(5.73710794046104,12.7404635562604,-2.27006012790935));
#38843=CARTESIAN_POINT('Ctrl Pts',(5.73767502813854,13.1774745354613,-2.31785808260716));
#38844=CARTESIAN_POINT('Ctrl Pts',(5.73813408874745,13.6180830602428,-2.33765179056008));
#38845=CARTESIAN_POINT('Ctrl Pts',(5.73848518360082,14.0587002405137,-2.32917720787917));
#38846=CARTESIAN_POINT('Ctrl Pts',(5.73855071706245,14.1409434542674,-2.32759538822686));
#38847=CARTESIAN_POINT('Ctrl Pts',(5.73861248895409,14.2231868244508,-2.32502868692948));
#38848=CARTESIAN_POINT('Ctrl Pts',(5.73867049959467,14.3054068119284,-2.32147536423056));
#38849=CARTESIAN_POINT('Ctrl Pts',(5.73897977936498,14.7437570626134,-2.30253106682041));
#38850=CARTESIAN_POINT('Ctrl Pts',(5.73918215114308,15.1814468350129,-2.25554274024818));
#38851=CARTESIAN_POINT('Ctrl Pts',(5.73927764630324,15.6148687029248,-2.18075653749148));
#38852=CARTESIAN_POINT('Ctrl Pts',(5.73929840881837,15.7091030921352,-2.1644965546436));
#38853=CARTESIAN_POINT('Ctrl Pts',(5.73931411902304,15.8031355368143,-2.14692253669996));
#38854=CARTESIAN_POINT('Ctrl Pts',(5.73932477703665,15.8969286328972,-2.1280370230487));
#38855=CARTESIAN_POINT('Ctrl Pts',(5.73937358626944,16.3264616798984,-2.04154929035207));
#38856=CARTESIAN_POINT('Ctrl Pts',(5.73931644080057,16.7509790383427,-1.92755545699466));
#38857=CARTESIAN_POINT('Ctrl Pts',(5.73915333155579,17.1669747746921,-1.78675913166143));
#38858=CARTESIAN_POINT('Ctrl Pts',(5.73911747417873,17.2584258508751,-1.75580695030658));
#38859=CARTESIAN_POINT('Ctrl Pts',(5.73907649564396,17.349464895975,-1.72355948667232));
#38860=CARTESIAN_POINT('Ctrl Pts',(5.73903039564377,17.4400543274668,-1.69002427007247));
#38861=CARTESIAN_POINT('Ctrl Pts',(5.73900084443013,17.4981243411746,-1.66852738621326));
#38862=CARTESIAN_POINT('Ctrl Pts',(5.73896918874359,17.5560096006854,-1.64650134931223));
#38863=CARTESIAN_POINT('Ctrl Pts',(5.73893542848779,17.6137010993935,-1.62395008432201));
#38864=CARTESIAN_POINT('Ctrl Pts',(5.73869640195945,18.0221636043077,-1.46428451152245));
#38865=CARTESIAN_POINT('Ctrl Pts',(5.73835187092069,18.4209173985343,-1.27828864360647));
#38866=CARTESIAN_POINT('Ctrl Pts',(5.73790179987834,18.8067382170266,-1.06736636396035));
#38867=CARTESIAN_POINT('Ctrl Pts',(5.73786596848425,18.8374544740072,-1.05057426090624));
#38868=CARTESIAN_POINT('Ctrl Pts',(5.73782946814598,18.868088733853,-1.03362417965316));
#38869=CARTESIAN_POINT('Ctrl Pts',(5.73779229884009,18.8986393563168,-1.01651683389843));
#38870=CARTESIAN_POINT('Ctrl Pts',(5.73741169569616,19.2114690603014,-0.84134246831089));
#38871=CARTESIAN_POINT('Ctrl Pts',(5.73696095042693,19.5155310886977,-0.649677705755805));
#38872=CARTESIAN_POINT('Ctrl Pts',(5.73644003522154,19.8089444558277,-0.442538425497627));
#38873=CARTESIAN_POINT('Ctrl Pts',(5.99999999930604,10.093342130059,-1.2110320640041));
#38874=CARTESIAN_POINT('Ctrl Pts',(5.99999999931574,10.2345701328353,-1.2690562326139));
#38875=CARTESIAN_POINT('Ctrl Pts',(5.9999999983593,10.3766480618126,-1.32363361111499));
#38876=CARTESIAN_POINT('Ctrl Pts',(5.99999999609549,10.5196451747559,-1.37484620718349));
#38877=CARTESIAN_POINT('Ctrl Pts',(5.99999999382046,10.6633506397232,-1.42631249051412));
#38878=CARTESIAN_POINT('Ctrl Pts',(5.99999999024024,10.8079848606125,-1.47438070543796));
#38879=CARTESIAN_POINT('Ctrl Pts',(5.9999999903917,10.9536373602466,-1.51908518767612));
#38880=CARTESIAN_POINT('Ctrl Pts',(5.99999999048562,11.0439530244963,-1.54680537798127));
#38881=CARTESIAN_POINT('Ctrl Pts',(5.99999999231407,11.1346605645158,-1.57323126119436));
#38882=CARTESIAN_POINT('Ctrl Pts',(5.99999999505303,11.2257838770401,-1.59836128795789));
#38883=CARTESIAN_POINT('Ctrl Pts',(5.99999999721704,11.2977790699919,-1.61821615358561));
#38884=CARTESIAN_POINT('Ctrl Pts',(5.99999999999976,11.3700338430068,-1.63726195422479));
#38885=CARTESIAN_POINT('Ctrl Pts',(5.99999999999976,11.4425636725777,-1.65549750785664));
#38886=CARTESIAN_POINT('Ctrl Pts',(5.99999999999976,11.6207224355689,-1.70029043921647));
#38887=CARTESIAN_POINT('Ctrl Pts',(5.99999998462037,11.8005057414763,-1.7402636201257));
#38888=CARTESIAN_POINT('Ctrl Pts',(5.99999998025208,11.9814335037277,-1.77525495536016));
#38889=CARTESIAN_POINT('Ctrl Pts',(5.99999997588683,12.1622357141048,-1.81022200892735));
#38890=CARTESIAN_POINT('Ctrl Pts',(5.99999998175318,12.3441803503634,-1.84021401163938));
#38891=CARTESIAN_POINT('Ctrl Pts',(5.99999999007209,12.5267747451034,-1.86511936449999));
#38892=CARTESIAN_POINT('Ctrl Pts',(5.99999999337634,12.5993008924312,-1.87501172342695));
#38893=CARTESIAN_POINT('Ctrl Pts',(5.99999999675179,12.6719294358255,-1.88410214542636));
#38894=CARTESIAN_POINT('Ctrl Pts',(5.99999999861021,12.7446291471263,-1.89238589423402));
#38895=CARTESIAN_POINT('Ctrl Pts',(5.99999999947177,12.7783326929135,-1.89622623558109));
#38896=CARTESIAN_POINT('Ctrl Pts',(5.99999999999976,12.8120515323859,-1.89989322143732));
#38897=CARTESIAN_POINT('Ctrl Pts',(5.99999999999976,12.8457823808324,-1.90338681610497));
#38898=CARTESIAN_POINT('Ctrl Pts',(5.99999999999976,13.0574331213622,-1.92530805237903));
#38899=CARTESIAN_POINT('Ctrl Pts',(5.99999998564335,13.2695715411693,-1.94033615669064));
#38900=CARTESIAN_POINT('Ctrl Pts',(5.99999998504722,13.4819409326284,-1.94851509625262));
#38901=CARTESIAN_POINT('Ctrl Pts',(5.99999998445037,13.6945673780514,-1.9567039356821));
#38902=CARTESIAN_POINT('Ctrl Pts',(5.9999999941301,13.9074259309238,-1.9580270706869));
#38903=CARTESIAN_POINT('Ctrl Pts',(5.99999999838063,14.1202649109823,-1.95247694787897));
#38904=CARTESIAN_POINT('Ctrl Pts',(5.99999999937189,14.1699005355257,-1.95118261818528));
#38905=CARTESIAN_POINT('Ctrl Pts',(5.99999999999976,14.2195350999111,-1.94951425840285));
#38906=CARTESIAN_POINT('Ctrl Pts',(5.99999999999976,14.2691654064614,-1.9474713641832));
#38907=CARTESIAN_POINT('Ctrl Pts',(5.99999999999976,14.2759025341524,-1.94719404896648));
#38908=CARTESIAN_POINT('Ctrl Pts',(5.99999999998822,14.2826395839499,-1.94690987504035));
#38909=CARTESIAN_POINT('Ctrl Pts',(5.99999999996617,14.2893765357274,-1.94661884102389));
#38910=CARTESIAN_POINT('Ctrl Pts',(5.99999999925251,14.5074225361486,-1.93719932825757));
#38911=CARTESIAN_POINT('Ctrl Pts',(5.99999999047932,14.7253659037648,-1.92058926833469));
#38912=CARTESIAN_POINT('Ctrl Pts',(5.9999999900727,14.9425466810117,-1.896835398383));
#38913=CARTESIAN_POINT('Ctrl Pts',(5.99999998966584,15.1598616306626,-1.87306685349609));
#38914=CARTESIAN_POINT('Ctrl Pts',(5.9999999969317,15.3764124894709,-1.84214572408041));
#38915=CARTESIAN_POINT('Ctrl Pts',(5.9999999994141,15.5915425240749,-1.80417066887197));
#38916=CARTESIAN_POINT('Ctrl Pts',(5.99999999977852,15.6231239934002,-1.79859586364592));
#38917=CARTESIAN_POINT('Ctrl Pts',(5.99999999999976,15.654674859378,-1.79286913108824));
#38918=CARTESIAN_POINT('Ctrl Pts',(5.99999999999976,15.686193063671,-1.78699087606494));
#38919=CARTESIAN_POINT('Ctrl Pts',(5.99999999999976,15.7318227336747,-1.77848078347155));
#38920=CARTESIAN_POINT('Ctrl Pts',(5.9999999995305,15.7773834590749,-1.76965175942691));
#38921=CARTESIAN_POINT('Ctrl Pts',(5.99999999872742,15.822872815609,-1.76050414225716));
#38922=CARTESIAN_POINT('Ctrl Pts',(5.99999999501575,16.0331161038684,-1.71822556854151));
#38923=CARTESIAN_POINT('Ctrl Pts',(5.99999998445161,16.2418360185537,-1.66914547855914));
#38924=CARTESIAN_POINT('Ctrl Pts',(5.99999998419206,16.4487787393024,-1.61332739853338));
#38925=CARTESIAN_POINT('Ctrl Pts',(5.99999998393252,16.655721460051,-1.55750931850762));
#38926=CARTESIAN_POINT('Ctrl Pts',(5.99999999999976,16.8608875382432,-1.49495305224471));
#38927=CARTESIAN_POINT('Ctrl Pts',(5.99999999999976,17.0640039415638,-1.42567351722652));
#38928=CARTESIAN_POINT('Ctrl Pts',(5.99999999999976,17.1462851294145,-1.39760880978853));
#38929=CARTESIAN_POINT('Ctrl Pts',(5.99999999597141,17.2282363682393,-1.36845265307108));
#38930=CARTESIAN_POINT('Ctrl Pts',(5.99999999157428,17.3098034003992,-1.33821915827955));
#38931=CARTESIAN_POINT('Ctrl Pts',(5.99999998233619,17.481170486579,-1.27470053108098));
#38932=CARTESIAN_POINT('Ctrl Pts',(5.99999997355916,17.6508403557923,-1.20642352175421));
#38933=CARTESIAN_POINT('Ctrl Pts',(5.99999997660579,17.818361722563,-1.13360431169194));
#38934=CARTESIAN_POINT('Ctrl Pts',(5.99999997965623,17.9860922997894,-1.06069416075198));
#38935=CARTESIAN_POINT('Ctrl Pts',(5.99999999487385,18.1516686004727,-0.983230670361461));
#38936=CARTESIAN_POINT('Ctrl Pts',(5.99999999914244,18.3146612115832,-0.901477355893947));
#38937=CARTESIAN_POINT('Ctrl Pts',(5.99999999968372,18.3353297517971,-0.891110495358455));
#38938=CARTESIAN_POINT('Ctrl Pts',(5.99999999999976,18.3559567822399,-0.880674713526301));
#38939=CARTESIAN_POINT('Ctrl Pts',(5.99999999999976,18.3765414594372,-0.870170598285201));
#38940=CARTESIAN_POINT('Ctrl Pts',(5.99999999999976,18.4906904314639,-0.811921739421176));
#38941=CARTESIAN_POINT('Ctrl Pts',(5.99999999306106,18.6035097023901,-0.751541582593229));
#38942=CARTESIAN_POINT('Ctrl Pts',(5.9999999914505,18.7150751423809,-0.689018196545716));
#38943=CARTESIAN_POINT('Ctrl Pts',(5.99999998952822,18.8482343794444,-0.614393237549431));
#38944=CARTESIAN_POINT('Ctrl Pts',(5.99999999274902,18.9796082754029,-0.536716140205771));
#38945=CARTESIAN_POINT('Ctrl Pts',(5.99999999547953,19.1092846788039,-0.45595063844579));
#38946=CARTESIAN_POINT('Ctrl Pts',(5.99999999819778,19.2383791002591,-0.375547608674738));
#38947=CARTESIAN_POINT('Ctrl Pts',(5.99999999961521,19.3657916282087,-0.2920836018942));
#38948=CARTESIAN_POINT('Ctrl Pts',(5.99999999985088,19.4915819744366,-0.205478937436434));
#38949=CARTESIAN_POINT('Ctrl Pts',(5.99999999991376,19.5251468526991,-0.182370049460026));
#38950=CARTESIAN_POINT('Ctrl Pts',(5.99999999993331,19.5585960651627,-0.15903731653548));
#38951=CARTESIAN_POINT('Ctrl Pts',(5.999999999933,19.5919303631537,-0.135478724431627));
#38952=CARTESIAN_POINT('Ctrl Pts',(-5.84353034391,10.0864246237472,-1.57297147931968));
#38953=CARTESIAN_POINT('Ctrl Pts',(-3.89568689594,10.6220908322031,-2.52887944306001));
#38954=CARTESIAN_POINT('Ctrl Pts',(0.0001666015265935,11.1575591931004,
-3.48561750059097));
#38955=CARTESIAN_POINT('Ctrl Pts',(3.896020098993,10.6220450329135,-2.52879761203758));
#38956=CARTESIAN_POINT('Ctrl Pts',(5.84403014849,10.0862871692312,-1.57272618876811));
#38957=CARTESIAN_POINT('Ctrl Pts',(-5.84353034391,10.8186450746373,-1.86224902860984));
#38958=CARTESIAN_POINT('Ctrl Pts',(-3.89568689594,11.3231575651093,-2.74792601689234));
#38959=CARTESIAN_POINT('Ctrl Pts',(0.0001666015265935,11.8270673123619,
-3.63586001146492));
#38960=CARTESIAN_POINT('Ctrl Pts',(3.896020098993,11.3231144650679,-2.74785007076882));
#38961=CARTESIAN_POINT('Ctrl Pts',(5.84403014849,10.8185156143099,-1.86202175967931));
#38962=CARTESIAN_POINT('Ctrl Pts',(-5.84353034391,12.4568729540691,-2.30089098012815));
#38963=CARTESIAN_POINT('Ctrl Pts',(-3.89568689594,12.8710971370357,-3.0672794361297));
#38964=CARTESIAN_POINT('Ctrl Pts',(0.0001666015265935,13.2856323394137,
-3.8324424808477));
#38965=CARTESIAN_POINT('Ctrl Pts',(3.896020098993,12.8710616813125,-3.06721399076156));
#38966=CARTESIAN_POINT('Ctrl Pts',(5.84403014849,12.4567666621639,-2.30069432116796));
#38967=CARTESIAN_POINT('Ctrl Pts',(-5.84353034391,15.0614254536629,-2.34071384846406));
#38968=CARTESIAN_POINT('Ctrl Pts',(-3.89568689594,15.2991206270769,-3.03320173188209));
#38969=CARTESIAN_POINT('Ctrl Pts',(0.0001666015265936,15.5368879417598,
-3.72636712888337));
#38970=CARTESIAN_POINT('Ctrl Pts',(3.896020098993,15.2991002905397,-3.0331424445665));
#38971=CARTESIAN_POINT('Ctrl Pts',(5.84403014849,15.0613644599445,-2.34053615276473));
#38972=CARTESIAN_POINT('Ctrl Pts',(-5.84353034391,17.6858135162578,-1.67939836042705));
#38973=CARTESIAN_POINT('Ctrl Pts',(-3.89568689594,17.7477953412524,-2.42360807923413));
#38974=CARTESIAN_POINT('Ctrl Pts',(0.0001666015265931,17.8092309023956,
-3.16660406681614));
#38975=CARTESIAN_POINT('Ctrl Pts',(3.896020098993,17.7477900865853,-2.42354452984376));
#38976=CARTESIAN_POINT('Ctrl Pts',(5.84403014849,17.6857976114169,-1.6792073926346));
#38977=CARTESIAN_POINT('Ctrl Pts',(-5.84353034391,19.2592933957493,-0.803936074634235));
#38978=CARTESIAN_POINT('Ctrl Pts',(-3.89568689594,19.2409363984223,-1.65690459370082));
#38979=CARTESIAN_POINT('Ctrl Pts',(0.0001666015265944,19.2238042951407,
-2.51236029214794));
#38980=CARTESIAN_POINT('Ctrl Pts',(3.896020098993,19.2409378637509,-1.65683142548429));
#38981=CARTESIAN_POINT('Ctrl Pts',(5.84403014849,19.2592981062585,-0.803717198855546));
#38982=CARTESIAN_POINT('Ctrl Pts',(-5.84353034391,19.9729831098892,-0.275591925382267));
#38983=CARTESIAN_POINT('Ctrl Pts',(-3.89568689594,19.9313477984332,-1.1982202827636));
#38984=CARTESIAN_POINT('Ctrl Pts',(0.0001666015265944,19.8897492520045,
-2.12096519186025));
#38985=CARTESIAN_POINT('Ctrl Pts',(3.896020098993,19.9313513564076,-1.19814135921599));
#38986=CARTESIAN_POINT('Ctrl Pts',(5.84403014849,19.9729937937055,-0.275355174534935));
#38987=CARTESIAN_POINT('Ctrl Pts',(-5.73278975502083,10.3449510841595,-1.7128961697678));
#38988=CARTESIAN_POINT('Ctrl Pts',(-5.37901580620726,10.4448361796299,-1.88167915312222));
#38989=CARTESIAN_POINT('Ctrl Pts',(-5.01621987753293,10.5336323549078,-2.03731789625457));
#38990=CARTESIAN_POINT('Ctrl Pts',(-4.64601513709761,10.6117448313211,-2.17806966584278));
#38991=CARTESIAN_POINT('Ctrl Pts',(-4.37166252199081,10.6696326966986,-2.28237847621087));
#38992=CARTESIAN_POINT('Ctrl Pts',(-4.09324095252986,10.7216528047211,-2.37850735433697));
#38993=CARTESIAN_POINT('Ctrl Pts',(-3.81140699867882,10.7679937575164,-2.46576099137469));
#38994=CARTESIAN_POINT('Ctrl Pts',(-3.57236698582203,10.8072982550783,-2.5397659515092));
#38995=CARTESIAN_POINT('Ctrl Pts',(-3.33087219324492,10.8425171603883,-2.60738551856862));
#38996=CARTESIAN_POINT('Ctrl Pts',(-3.08732322273381,10.8737878367289,-2.66822937065829));
#38997=CARTESIAN_POINT('Ctrl Pts',(-3.04372206931726,10.8793860437495,-2.67912189105715));
#38998=CARTESIAN_POINT('Ctrl Pts',(-3.00005508020644,10.8848577806713,-2.68979736726869));
#38999=CARTESIAN_POINT('Ctrl Pts',(-2.95632455391942,10.8902039324604,-2.70025372277678));
#39000=CARTESIAN_POINT('Ctrl Pts',(-2.75788264616247,10.9144638865531,-2.74770293757909));
#39001=CARTESIAN_POINT('Ctrl Pts',(-2.55812786428845,10.9361985805701,-2.79065506823792));
#39002=CARTESIAN_POINT('Ctrl Pts',(-2.35732700629461,10.9553876930419,-2.82889428277911));
#39003=CARTESIAN_POINT('Ctrl Pts',(-2.16336841517962,10.9739229386428,-2.86583050034239));
#39004=CARTESIAN_POINT('Ctrl Pts',(-1.96843382320251,10.9900831075099,-2.89836945730171));
#39005=CARTESIAN_POINT('Ctrl Pts',(-1.77276367380457,11.0038735436133,-2.92635857466279));
#39006=CARTESIAN_POINT('Ctrl Pts',(-1.58018406103536,11.0174461649503,-2.95390561441175));
#39007=CARTESIAN_POINT('Ctrl Pts',(-1.3868919430529,11.0287232475636,-2.97704526002274));
#39008=CARTESIAN_POINT('Ctrl Pts',(-1.19311654915955,11.0377339936928,-2.99567504720032));
#39009=CARTESIAN_POINT('Ctrl Pts',(-0.994951121524408,11.0469488807025,
-3.01472689722432));
#39010=CARTESIAN_POINT('Ctrl Pts',(-0.796280272439716,11.0537933397654,
-3.0290617895358));
#39011=CARTESIAN_POINT('Ctrl Pts',(-0.597349166591621,11.0583266053215,
-3.03862030630298));
#39012=CARTESIAN_POINT('Ctrl Pts',(-0.408571857533149,11.0626284849561,
-3.04769093940587));
#39013=CARTESIAN_POINT('Ctrl Pts',(-0.219560181608441,11.0648492036146,
-3.05246055293869));
#39014=CARTESIAN_POINT('Ctrl Pts',(-0.0305236461352285,11.0650646066962,
-3.05292367184669));
#39015=CARTESIAN_POINT('Ctrl Pts',(-0.0203559062909503,11.0650761926178,
-3.05294858170108));
#39016=CARTESIAN_POINT('Ctrl Pts',(-0.0101880945265215,11.0650819831622,
-3.05296104360322));
#39017=CARTESIAN_POINT('Ctrl Pts',(-2.02434432647914E-5,11.0650819922319,
-3.05296106047373));
#39018=CARTESIAN_POINT('Ctrl Pts',(-1.34956290334826E-5,11.0650819922379,
-3.05296106048493));
#39019=CARTESIAN_POINT('Ctrl Pts',(-6.74781482048857E-6,11.0650819922414,
-3.05296106049064));
#39020=CARTESIAN_POINT('Ctrl Pts',(-6.24391702939142E-13,11.0650819922423,
-3.05296106049087));
#39021=CARTESIAN_POINT('Ctrl Pts',(0.189391034103492,11.0650820182466,-3.0529610670559));
#39022=CARTESIAN_POINT('Ctrl Pts',(0.378768545059335,11.0630740529817,-3.04863949431656));
#39023=CARTESIAN_POINT('Ctrl Pts',(0.567921848613415,11.0589804704103,-3.03999941059282));
#39024=CARTESIAN_POINT('Ctrl Pts',(0.769326050312761,11.0546217586437,-3.03079973428636));
#39025=CARTESIAN_POINT('Ctrl Pts',(0.970476061616078,11.0478983328162,-3.01670370047049));
#39026=CARTESIAN_POINT('Ctrl Pts',(1.17111755353397,11.038747420467,-2.99777056713526));
#39027=CARTESIAN_POINT('Ctrl Pts',(1.36691637355855,11.0298173740295,-2.97929440285354));
#39028=CARTESIAN_POINT('Ctrl Pts',(1.56223092515411,11.018575855937,-2.95621227598697));
#39029=CARTESIAN_POINT('Ctrl Pts',(1.75682485384488,11.0049919071274,-2.92862831235811));
#39030=CARTESIAN_POINT('Ctrl Pts',(1.95863808969716,10.9909040027237,-2.90002100176509));
#39031=CARTESIAN_POINT('Ctrl Pts',(2.15967624153261,10.9742966294215,-2.86657163013415));
#39032=CARTESIAN_POINT('Ctrl Pts',(2.35967566109098,10.9551636073509,-2.8284469262728));
#39033=CARTESIAN_POINT('Ctrl Pts',(2.55967508064935,10.9360305852803,-2.79032222241145));
#39034=CARTESIAN_POINT('Ctrl Pts',(2.75863576793065,10.9143720907802,-2.74752252151317));
#39035=CARTESIAN_POINT('Ctrl Pts',(2.95629407467463,10.8902082476216,-2.70026117661292));
#39036=CARTESIAN_POINT('Ctrl Pts',(3.19879463434546,10.8605624129168,-2.64227776686961));
#39037=CARTESIAN_POINT('Ctrl Pts',(3.43934160302183,10.8270524690154,-2.5775523679393));
#39038=CARTESIAN_POINT('Ctrl Pts',(3.67754301047263,10.7895391923811,-2.50645885904836));
#39039=CARTESIAN_POINT('Ctrl Pts',(3.96237540988465,10.7446822089236,-2.42144788057962));
#39040=CARTESIAN_POINT('Ctrl Pts',(4.24385401127729,10.694101158698,-2.32733227970892));
#39041=CARTESIAN_POINT('Ctrl Pts',(4.52130863956216,10.6375985200971,-2.22481497999281));
#39042=CARTESIAN_POINT('Ctrl Pts',(4.88831882413484,10.5628582140876,-2.08920760763328));
#39043=CARTESIAN_POINT('Ctrl Pts',(5.24828812203085,10.477757187457,-1.93890576546615));
#39044=CARTESIAN_POINT('Ctrl Pts',(5.5996654085723,10.381900692554,-1.77558867682684));
#39045=CARTESIAN_POINT('Ctrl Pts',(5.64417809415769,10.3697575342386,-1.7548995700013));
#39046=CARTESIAN_POINT('Ctrl Pts',(5.68855289536406,10.3574418257978,-1.73400154805331));
#39047=CARTESIAN_POINT('Ctrl Pts',(5.73278665880606,10.3449528049738,-1.7128979547254));
#39048=CARTESIAN_POINT('Ctrl Pts',(-5.84422935313255,10.3326179436783,-1.66677955401275));
#39049=CARTESIAN_POINT('Ctrl Pts',(-5.39723073539493,10.4682500954886,-1.88672368606665));
#39050=CARTESIAN_POINT('Ctrl Pts',(-4.37278936862451,10.7273674796295,-2.32714772276908));
#39051=CARTESIAN_POINT('Ctrl Pts',(-2.71089230894894,10.9902717063683,-2.8158221119383));
#39052=CARTESIAN_POINT('Ctrl Pts',(-0.904516202368409,11.1231766923864,
-3.08010999588275));
#39053=CARTESIAN_POINT('Ctrl Pts',(0.905422156638638,11.1231437154035,-3.08004278635486));
#39054=CARTESIAN_POINT('Ctrl Pts',(2.71180944555921,10.9901684408322,-2.81562160453371));
#39055=CARTESIAN_POINT('Ctrl Pts',(4.37341442202404,10.7272312569814,-2.32690647824196));
#39056=CARTESIAN_POINT('Ctrl Pts',(5.39759958770343,10.4681419380673,-1.886546911375));
#39057=CARTESIAN_POINT('Ctrl Pts',(5.84433805276918,10.3325849446319,-1.66672608703151));
#39058=CARTESIAN_POINT('Ctrl Pts',(-5.72537553697924,10.0515132270061,-1.59486222014698));
#39059=CARTESIAN_POINT('Ctrl Pts',(-5.28737692922011,10.1848998766557,-1.80870858998522));
#39060=CARTESIAN_POINT('Ctrl Pts',(-4.28358980961365,10.4398181577976,-2.23709191171346));
#39061=CARTESIAN_POINT('Ctrl Pts',(-2.65541314896773,10.6985985951467,-2.71261121371761));
#39062=CARTESIAN_POINT('Ctrl Pts',(-0.88596500427895,10.829464766054,-2.96982219801529));
#39063=CARTESIAN_POINT('Ctrl Pts',(0.886852389154446,10.8294322908905,-2.96975678663163));
#39064=CARTESIAN_POINT('Ctrl Pts',(2.65631159921206,10.6984969260531,-2.71241608186123));
#39065=CARTESIAN_POINT('Ctrl Pts',(4.28420224316951,10.4396841067023,-2.23685720221533));
#39066=CARTESIAN_POINT('Ctrl Pts',(5.28773835329507,10.1847935018816,-1.80853670049365));
#39067=CARTESIAN_POINT('Ctrl Pts',(5.72548204834205,10.0514807738283,-1.59481023378505));
#39068=CARTESIAN_POINT('Ctrl Pts',(-5.71942831533579,9.77836172016708,-1.74871820725318));
#39069=CARTESIAN_POINT('Ctrl Pts',(-5.28270068923074,9.91044415240004,-1.96030029454256));
#39070=CARTESIAN_POINT('Ctrl Pts',(-4.28157574258823,10.1630390832986,-2.38447623743461));
#39071=CARTESIAN_POINT('Ctrl Pts',(-2.6557887324519,10.4198723259329,-2.8562525631157));
#39072=CARTESIAN_POINT('Ctrl Pts',(-0.88645093086578,10.5499497734634,-3.11191327809778));
#39073=CARTESIAN_POINT('Ctrl Pts',(0.887338700652733,10.5499174748729,-3.11184821214888));
#39074=CARTESIAN_POINT('Ctrl Pts',(2.65668656115258,10.4197713255722,-2.85605874443294));
#39075=CARTESIAN_POINT('Ctrl Pts',(4.28218671263831,10.1629061704207,-2.38424365348559));
#39076=CARTESIAN_POINT('Ctrl Pts',(5.28306107935149,9.91033880165622,-1.9601302077373));
#39077=CARTESIAN_POINT('Ctrl Pts',(5.7195345147545,9.77832958295092,-1.74866677484432));
#39078=CARTESIAN_POINT('Ctrl Pts',(-5.83024722549531,9.69037424501856,-2.02853375411005));
#39079=CARTESIAN_POINT('Ctrl Pts',(-5.38623690424319,9.82293988326085,-2.24315406310329));
#39080=CARTESIAN_POINT('Ctrl Pts',(-4.36805474491177,10.0765945414732,-2.67368564029794));
#39081=CARTESIAN_POINT('Ctrl Pts',(-2.71177598656107,10.3349204760671,-3.15355950681661));
#39082=CARTESIAN_POINT('Ctrl Pts',(-0.905658932461119,10.4659710001726,
-3.41420239959998));
#39083=CARTESIAN_POINT('Ctrl Pts',(0.90656579194999,10.4659384383509,-3.41413600225329));
#39084=CARTESIAN_POINT('Ctrl Pts',(2.71269166196735,10.3348187828708,-3.15336208695204));
#39085=CARTESIAN_POINT('Ctrl Pts',(4.36867635738294,10.0764609950322,-2.6734493933936));
#39086=CARTESIAN_POINT('Ctrl Pts',(5.38660332554845,9.82283413356729,-2.24298152691996));
#39087=CARTESIAN_POINT('Ctrl Pts',(5.83035519169749,9.69034198886957,-2.0284815895926));
#39088=CARTESIAN_POINT('Ctrl Pts',(-5.72001750558411,9.72697457205148,-2.05943207691667));
#39089=CARTESIAN_POINT('Ctrl Pts',(-5.49206568348151,9.79330018878959,-2.16743192710529));
#39090=CARTESIAN_POINT('Ctrl Pts',(-5.25921576351921,9.85517369883701,-2.27049947746689));
#39091=CARTESIAN_POINT('Ctrl Pts',(-5.0216601982015,9.91261925507755,-2.36800096228074));
#39092=CARTESIAN_POINT('Ctrl Pts',(-4.83340321471274,9.95814345535555,-2.44526850763242));
#39093=CARTESIAN_POINT('Ctrl Pts',(-4.64219111721331,10.0008865508324,-2.51903966348394));
#39094=CARTESIAN_POINT('Ctrl Pts',(-4.4481258687923,10.0408548470982,-2.58897722641875));
#39095=CARTESIAN_POINT('Ctrl Pts',(-4.42435514837881,10.0457504953591,-2.59754375890435));
#39096=CARTESIAN_POINT('Ctrl Pts',(-4.40054162912284,10.0506045062339,-2.60605274953309));
#39097=CARTESIAN_POINT('Ctrl Pts',(-4.37668559068971,10.0554168977595,-2.61450355613505));
#39098=CARTESIAN_POINT('Ctrl Pts',(-4.14449479000357,10.1022559001649,-2.69675524921698));
#39099=CARTESIAN_POINT('Ctrl Pts',(-3.90827758451816,10.1451475506915,-2.77352066955216));
#39100=CARTESIAN_POINT('Ctrl Pts',(-3.66827959909047,10.1840646157826,-2.84432679982134));
#39101=CARTESIAN_POINT('Ctrl Pts',(-3.54828060637662,10.2035231483282,-2.87972986495593));
#39102=CARTESIAN_POINT('Ctrl Pts',(-3.42733711572398,10.2219871680773,-2.91364387703704));
#39103=CARTESIAN_POINT('Ctrl Pts',(-3.30548427923154,10.2394481351887,-2.94601451933545));
#39104=CARTESIAN_POINT('Ctrl Pts',(-3.24455786098532,10.2481786187444,-2.96219984048465));
#39105=CARTESIAN_POINT('Ctrl Pts',(-3.18340410134152,10.2566583148036,-2.97799931187828));
#39106=CARTESIAN_POINT('Ctrl Pts',(-3.12202776956448,10.264885806214,-2.99340654821786));
#39107=CARTESIAN_POINT('Ctrl Pts',(-3.08480107734262,10.2698760407495,-3.00275152581095));
#39108=CARTESIAN_POINT('Ctrl Pts',(-3.04679094731952,10.2748650953664,-3.01212474426539));
#39109=CARTESIAN_POINT('Ctrl Pts',(-3.00927407317018,10.2796842949948,-3.02120807144621));
#39110=CARTESIAN_POINT('Ctrl Pts',(-2.98493618726443,10.2828105983815,-3.02710059276053));
#39111=CARTESIAN_POINT('Ctrl Pts',(-2.96080619766097,10.2858659691822,-3.03287201197784));
#39112=CARTESIAN_POINT('Ctrl Pts',(-2.93723584159235,10.288810155411,-3.0384451782907));
#39113=CARTESIAN_POINT('Ctrl Pts',(-2.85104375385783,10.2995764568195,-3.05882513514834));
#39114=CARTESIAN_POINT('Ctrl Pts',(-2.76462199302743,10.3098384886512,-3.07833996422562));
#39115=CARTESIAN_POINT('Ctrl Pts',(-2.67798441088526,10.3196021825765,-3.09697541649601));
#39116=CARTESIAN_POINT('Ctrl Pts',(-2.41894336054858,10.3487950278409,-3.15269427441265));
#39117=CARTESIAN_POINT('Ctrl Pts',(-2.15797485850097,10.3735347225913,-3.20055455830548));
#39118=CARTESIAN_POINT('Ctrl Pts',(-1.89556992266632,10.3939293425982,-3.24032729421704));
#39119=CARTESIAN_POINT('Ctrl Pts',(-1.63420115925437,10.4142434292769,-3.27994297739637));
#39120=CARTESIAN_POINT('Ctrl Pts',(-1.37140674786025,10.4302466213787,-3.31153518973123));
#39121=CARTESIAN_POINT('Ctrl Pts',(-1.10765056326125,10.4420212989983,-3.33483767822194));
#39122=CARTESIAN_POINT('Ctrl Pts',(-1.03553024031539,10.4452409146968,-3.34120940746858));
#39123=CARTESIAN_POINT('Ctrl Pts',(-0.963337911030768,10.4481442389793,
-3.34696109130944));
#39124=CARTESIAN_POINT('Ctrl Pts',(-0.891082862512929,10.4507326466169,
-3.35208671100954));
#39125=CARTESIAN_POINT('Ctrl Pts',(-0.627875898516178,10.4601615644549,
-3.37075805408579));
#39126=CARTESIAN_POINT('Ctrl Pts',(-0.363837180964085,10.4654134527972,
-3.3811253229753));
#39127=CARTESIAN_POINT('Ctrl Pts',(-0.0994820302231884,10.4664670531146,
-3.38320655683317));
#39128=CARTESIAN_POINT('Ctrl Pts',(-0.0663911103587122,10.466598938586,
-3.38346707735874));
#39129=CARTESIAN_POINT('Ctrl Pts',(-0.0332952257283999,10.4666650110093,
-3.38359770416469));
#39130=CARTESIAN_POINT('Ctrl Pts',(-0.000195383006570636,10.4666652029542,
-3.38359842127642));
#39131=CARTESIAN_POINT('Ctrl Pts',(0.260328417753622,10.4666667137238,-3.38360406555319));
#39132=CARTESIAN_POINT('Ctrl Pts',(0.520593752654219,10.4625913206532,-3.3755578983993));
#39133=CARTESIAN_POINT('Ctrl Pts',(0.780120363257257,10.4544573923531,-3.35946676550572));
#39134=CARTESIAN_POINT('Ctrl Pts',(0.817425956250517,10.4532881826991,-3.35715374930621));
#39135=CARTESIAN_POINT('Ctrl Pts',(0.854716282561188,10.4520350739337,-3.35467442500711));
#39136=CARTESIAN_POINT('Ctrl Pts',(0.89198991048456,10.4506980809692,-3.35202873401766));
#39137=CARTESIAN_POINT('Ctrl Pts',(1.08871979571785,10.4436414436864,-3.33806479989815));
#39138=CARTESIAN_POINT('Ctrl Pts',(1.28498476952638,10.4342486516205,-3.3194675611386));
#39139=CARTESIAN_POINT('Ctrl Pts',(1.4806027073567,10.4224868529531,-3.29636060766967));
#39140=CARTESIAN_POINT('Ctrl Pts',(1.72586245691025,10.4077402717986,-3.26738982061612));
#39141=CARTESIAN_POINT('Ctrl Pts',(1.97009186766474,10.3892874677145,-3.23128119591996));
#39142=CARTESIAN_POINT('Ctrl Pts',(2.21291486465638,10.3670517966272,-3.18823396193957));
#39143=CARTESIAN_POINT('Ctrl Pts',(2.33432636315221,10.3559339610836,-3.16671034494937));
#39144=CARTESIAN_POINT('Ctrl Pts',(2.455386465299,10.3438695379754,-3.14345318748102));
#39145=CARTESIAN_POINT('Ctrl Pts',(2.57604938841735,10.3308436213554,-3.11849411619528));
#39146=CARTESIAN_POINT('Ctrl Pts',(2.61034999432425,10.3271407702972,-3.11139905131662));
#39147=CARTESIAN_POINT('Ctrl Pts',(2.64461855856262,10.3233601803353,-3.10416652345661));
#39148=CARTESIAN_POINT('Ctrl Pts',(2.67885392870299,10.3195015097565,-3.09679721177542));
#39149=CARTESIAN_POINT('Ctrl Pts',(2.70483527669272,10.316573150499,-3.09120461410673));
#39150=CARTESIAN_POINT('Ctrl Pts',(2.73079750695558,10.3135998217514,-3.08553323762981));
#39151=CARTESIAN_POINT('Ctrl Pts',(2.75674025459381,10.3105813374921,-3.0797835523159));
#39152=CARTESIAN_POINT('Ctrl Pts',(2.79332433319526,10.3063247156824,-3.0716754312182));
#39153=CARTESIAN_POINT('Ctrl Pts',(2.82916047457324,10.3020630585324,-3.0635725282504));
#39154=CARTESIAN_POINT('Ctrl Pts',(2.86554265400224,10.297642918513,-3.05518462723504));
#39155=CARTESIAN_POINT('Ctrl Pts',(2.88895590046142,10.2947983987706,-3.04978670999011));
#39156=CARTESIAN_POINT('Ctrl Pts',(2.91259502854718,10.2918877539081,-3.04426991457996));
#39157=CARTESIAN_POINT('Ctrl Pts',(2.93680184037229,10.2888644771338,-3.0385474416855));
#39158=CARTESIAN_POINT('Ctrl Pts',(3.1828164679285,10.2581388154889,-2.98038976078138));
#39159=CARTESIAN_POINT('Ctrl Pts',(3.4253594210897,10.2234388449908,-2.9157914273284));
#39160=CARTESIAN_POINT('Ctrl Pts',(3.66417651007782,10.1847920895663,-2.84531381876157));
#39161=CARTESIAN_POINT('Ctrl Pts',(3.91060789592046,10.1449131448143,-2.77258914556676));
#39162=CARTESIAN_POINT('Ctrl Pts',(4.1530722143786,10.1008318659714,-2.69360413379684));
#39163=CARTESIAN_POINT('Ctrl Pts',(4.39129440848135,10.0525670600447,-2.60892207677239));
#39164=CARTESIAN_POINT('Ctrl Pts',(4.4105414251735,10.0486675345248,-2.60208024168975));
#39165=CARTESIAN_POINT('Ctrl Pts',(4.42976075177401,10.0447406934149,-2.59520119067901));
#39166=CARTESIAN_POINT('Ctrl Pts',(4.44895224382876,10.0407865430965,-2.58828520675295));
#39167=CARTESIAN_POINT('Ctrl Pts',(4.69665557783849,9.9897505832941,-2.49902105409841));
#39168=CARTESIAN_POINT('Ctrl Pts',(4.93972238691474,9.93416654528795,-2.40360864190788));
#39169=CARTESIAN_POINT('Ctrl Pts',(5.17793597175251,9.87405249029242,-2.30262611824544));
#39170=CARTESIAN_POINT('Ctrl Pts',(5.36154614781137,9.8277178019124,-2.22479084717491));
#39171=CARTESIAN_POINT('Ctrl Pts',(5.54227296781462,9.77869150699081,-2.14364519080835));
#39172=CARTESIAN_POINT('Ctrl Pts',(5.7200146623697,9.72697523687866,-2.05943412015819));
#39173=CARTESIAN_POINT('Ctrl Pts',(6.05077471961553,6.21842583509821,-8.31822495858353));
#39174=CARTESIAN_POINT('Ctrl Pts',(6.05142593340447,6.23969193373903,-8.30198934364668));
#39175=CARTESIAN_POINT('Ctrl Pts',(6.04716899616723,6.29515597960163,-8.26241512108273));
#39176=CARTESIAN_POINT('Ctrl Pts',(6.01567297877913,6.39159059660638,-8.20453501924637));
#39177=CARTESIAN_POINT('Ctrl Pts',(5.94753066244136,6.50078121143289,-8.15338924888124));
#39178=CARTESIAN_POINT('Ctrl Pts',(5.84910732584619,6.60164332898259,-8.12175932743906));
#39179=CARTESIAN_POINT('Ctrl Pts',(5.76414023552456,6.65913247159952,-8.11648748828758));
#39180=CARTESIAN_POINT('Ctrl Pts',(5.71687096680919,6.68389896885781,-8.11896177582376));
#39181=CARTESIAN_POINT('Ctrl Pts',(5.71191285258273,6.6864219935317,-8.11927735102364));
#39182=CARTESIAN_POINT('Ctrl Pts',(5.9119429072752,6.04924592523811,-8.09057562670355));
#39183=CARTESIAN_POINT('Ctrl Pts',(5.91254068779913,6.06837636901304,-8.07595986584746));
#39184=CARTESIAN_POINT('Ctrl Pts',(5.90863665457664,6.11851658263178,-8.04024430370093));
#39185=CARTESIAN_POINT('Ctrl Pts',(5.87944445404612,6.20656764599406,-7.9878084478441));
#39186=CARTESIAN_POINT('Ctrl Pts',(5.81592145568837,6.30701177251466,-7.94151268428573));
#39187=CARTESIAN_POINT('Ctrl Pts',(5.72394918073557,6.40018754436466,-7.91317658918676));
#39188=CARTESIAN_POINT('Ctrl Pts',(5.64455513570018,6.45339418295547,-7.9088733448521));
#39189=CARTESIAN_POINT('Ctrl Pts',(5.60044619117731,6.47632149431093,-7.91141082748276));
#39190=CARTESIAN_POINT('Ctrl Pts',(5.59582027554415,6.47865725297412,-7.91172803484192));
#39191=CARTESIAN_POINT('Ctrl Pts',(6.02852050621993,5.86900777502338,-7.85896159208741));
#39192=CARTESIAN_POINT('Ctrl Pts',(6.02945804993531,5.89850257739766,-7.83645112392778));
#39193=CARTESIAN_POINT('Ctrl Pts',(6.02330228130752,5.97418179417425,-7.78245669334098));
#39194=CARTESIAN_POINT('Ctrl Pts',(5.98006183254276,6.10142380740703,-7.70591992048359));
#39195=CARTESIAN_POINT('Ctrl Pts',(5.88924834938387,6.24220627570421,-7.63973400270886));
#39196=CARTESIAN_POINT('Ctrl Pts',(5.75973686058714,6.37117340314249,-7.59922294714483));
#39197=CARTESIAN_POINT('Ctrl Pts',(5.64790222410802,6.4451134530259,-7.59259942739894));
#39198=CARTESIAN_POINT('Ctrl Pts',(5.58523655084478,6.47730266427808,-7.59598554867957));
#39199=CARTESIAN_POINT('Ctrl Pts',(5.57865817275388,6.48058621946311,-7.59641446277799));
#39200=CARTESIAN_POINT('Ctrl Pts',(6.32408553231757,5.79586551090958,-7.7752161516984));
#39201=CARTESIAN_POINT('Ctrl Pts',(6.32553330551962,5.84143037849579,-7.74047175332521));
#39202=CARTESIAN_POINT('Ctrl Pts',(6.31599727660815,5.95676945960246,-7.6580435523049));
#39203=CARTESIAN_POINT('Ctrl Pts',(6.25156577757377,6.14508548193301,-7.54365994334047));
#39204=CARTESIAN_POINT('Ctrl Pts',(6.11944215589101,6.34884751030328,-7.44588260852661));
#39205=CARTESIAN_POINT('Ctrl Pts',(5.93300983305097,6.53362083847875,-7.38570904471001));
#39206=CARTESIAN_POINT('Ctrl Pts',(5.77198724572357,6.63971852407646,-7.37499742538782));
#39207=CARTESIAN_POINT('Ctrl Pts',(5.68121256712033,6.68619912587697,-7.37946130795072));
#39208=CARTESIAN_POINT('Ctrl Pts',(5.67167699310978,6.69094421653975,-7.38003877455295));
#39209=CARTESIAN_POINT('',(5.732785291682,6.65588487364253,-8.10254503001699));
#39210=CARTESIAN_POINT('',(5.72001552894544,6.64701088376288,-7.3940918491053));
#39211=CARTESIAN_POINT('Origin',(5.898757994352,6.95917605551496,-7.74135737489339));
#39212=CARTESIAN_POINT('',(5.99999998860446,6.44014593005993,-7.42970700294369));
#39213=CARTESIAN_POINT('Ctrl Pts',(6.0000000519944,6.44014606643596,-7.42970716027456));
#39214=CARTESIAN_POINT('Ctrl Pts',(5.95914560525917,6.47968727812811,-7.41730334914713));
#39215=CARTESIAN_POINT('Ctrl Pts',(5.91541907062042,6.51668572949036,-7.40809453517975));
#39216=CARTESIAN_POINT('Ctrl Pts',(5.86878902309971,6.5512055037961,-7.40209476752825));
#39217=CARTESIAN_POINT('Ctrl Pts',(5.82215897558057,6.5857252781007,-7.39609499987695));
#39218=CARTESIAN_POINT('Ctrl Pts',(5.77262518199994,6.61776600827662,-7.39330385120898));
#39219=CARTESIAN_POINT('Ctrl Pts',(5.72001606109489,6.64701181313427,-7.39409288290435));
#39220=CARTESIAN_POINT('',(5.99998738510675,6.09545783229234,-8.13557311354423));
#39221=CARTESIAN_POINT('Ctrl Pts',(5.99998738510675,6.09545783229234,-8.13557311354423));
#39222=CARTESIAN_POINT('Ctrl Pts',(5.99998486187689,6.09906559316439,-8.10752276907166));
#39223=CARTESIAN_POINT('Ctrl Pts',(5.99998575125142,6.10334644784103,-8.07998145178508));
#39224=CARTESIAN_POINT('Ctrl Pts',(5.9999822017205,6.10832836814456,-8.05296723319903));
#39225=CARTESIAN_POINT('Ctrl Pts',(5.99998107889726,6.10990429917679,-8.04442182444348));
#39226=CARTESIAN_POINT('Ctrl Pts',(5.99997928834143,6.11155002495211,-8.03592910458814));
#39227=CARTESIAN_POINT('Ctrl Pts',(5.99997621692443,6.11326554040231,-8.02748944959876));
#39228=CARTESIAN_POINT('Ctrl Pts',(5.99996211490585,6.12114211034623,-7.98873985231655));
#39229=CARTESIAN_POINT('Ctrl Pts',(5.99992503046442,6.13049155468325,-7.95111245217534));
#39230=CARTESIAN_POINT('Ctrl Pts',(5.99991423108089,6.14127675934099,-7.91456073449541));
#39231=CARTESIAN_POINT('Ctrl Pts',(5.99990487784457,6.15061771548782,-7.88290366327844));
#39232=CARTESIAN_POINT('Ctrl Pts',(5.99990278201506,6.16105737414897,-7.85206613788475));
#39233=CARTESIAN_POINT('Ctrl Pts',(5.99990421744016,6.17258775683501,-7.82206010445584));
#39234=CARTESIAN_POINT('Ctrl Pts',(5.99990515161376,6.18009172136025,-7.80253220009007));
#39235=CARTESIAN_POINT('Ctrl Pts',(5.99990793441964,6.18805772979702,-7.78335583843895));
#39236=CARTESIAN_POINT('Ctrl Pts',(5.99991541529791,6.1964933914083,-7.76452783598631));
#39237=CARTESIAN_POINT('Ctrl Pts',(5.99991831505963,6.19976324927403,-7.75722966605576));
#39238=CARTESIAN_POINT('Ctrl Pts',(5.99992637047872,6.20321225211258,-7.74973530638953));
#39239=CARTESIAN_POINT('Ctrl Pts',(5.99993172018384,6.20669887667019,-7.74238903612566));
#39240=CARTESIAN_POINT('Ctrl Pts',(5.99993713803786,6.21022991668828,-7.73494918309393));
#39241=CARTESIAN_POINT('Ctrl Pts',(5.9999395079884,6.21379941178357,-7.72766152244286));
#39242=CARTESIAN_POINT('Ctrl Pts',(5.99994451737609,6.2172087557156,-7.72087231262672));
#39243=CARTESIAN_POINT('Ctrl Pts',(5.99994535116398,6.21777622420938,-7.71974228211494));
#39244=CARTESIAN_POINT('Ctrl Pts',(5.999946292958,6.21833914779861,-7.71862603044698));
#39245=CARTESIAN_POINT('Ctrl Pts',(5.99994741064976,6.21889648704503,-7.71752511762765));
#39246=CARTESIAN_POINT('Ctrl Pts',(5.99997420500938,6.23225754836266,-7.69113299868253));
#39247=CARTESIAN_POINT('Ctrl Pts',(5.99996028565732,6.24653972602933,-7.66574258331808));
#39248=CARTESIAN_POINT('Ctrl Pts',(5.99993572431094,6.26166953382428,-7.64132013235762));
#39249=CARTESIAN_POINT('Ctrl Pts',(5.99991395264974,6.27508089345201,-7.6196715907991));
#39250=CARTESIAN_POINT('Ctrl Pts',(5.99988491856949,6.28915903686546,-7.59878279218735));
#39251=CARTESIAN_POINT('Ctrl Pts',(5.99986830472584,6.30388676844893,-7.57863699716864));
#39252=CARTESIAN_POINT('Ctrl Pts',(5.99985059014737,6.31959027225559,-7.55715646114912));
#39253=CARTESIAN_POINT('Ctrl Pts',(5.9998484739606,6.33603282621633,-7.53651939610242));
#39254=CARTESIAN_POINT('Ctrl Pts',(5.99986814609502,6.3532309144603,-7.51672507359564));
#39255=CARTESIAN_POINT('Ctrl Pts',(5.99988721410734,6.36990085740629,-7.49753862553458));
#39256=CARTESIAN_POINT('Ctrl Pts',(5.99992732030833,6.38728175857388,-7.47914377038259));
#39257=CARTESIAN_POINT('Ctrl Pts',(5.999961045714,6.4054053563925,-7.46157120296813));
#39258=CARTESIAN_POINT('Ctrl Pts',(5.99998205295471,6.41669437648174,-7.4506254145796));
#39259=CARTESIAN_POINT('Ctrl Pts',(5.99999988350857,6.42827183775403,-7.4399993282562));
#39260=CARTESIAN_POINT('Ctrl Pts',(5.99999988745865,6.4401458000223,-7.42970685292513));
#39261=CARTESIAN_POINT('Ctrl Pts',(5.99998738510675,6.09545783229234,-8.13557311354423));
#39262=CARTESIAN_POINT('Ctrl Pts',(5.99998441904533,6.1110792605425,-8.12979435905872));
#39263=CARTESIAN_POINT('Ctrl Pts',(5.9992397470716,6.1278161441473,-8.12408926921516));
#39264=CARTESIAN_POINT('Ctrl Pts',(5.99754903941737,6.14562213733926,-8.1185853568534));
#39265=CARTESIAN_POINT('Ctrl Pts',(5.99682966821598,6.15319832514584,-8.11624352322053));
#39266=CARTESIAN_POINT('Ctrl Pts',(5.995938805942,6.16096762335711,-8.11393846741642));
#39267=CARTESIAN_POINT('Ctrl Pts',(5.99485951760362,6.16892439542041,-8.11168171476116));
#39268=CARTESIAN_POINT('Ctrl Pts',(5.99246751504082,6.18655881107221,-8.10668012441402));
#39269=CARTESIAN_POINT('Ctrl Pts',(5.98914968027009,6.2051168950132,-8.10191432041602));
#39270=CARTESIAN_POINT('Ctrl Pts',(5.98476329171026,6.22450598415262,-8.09751162212164));
#39271=CARTESIAN_POINT('Ctrl Pts',(5.98056287493804,6.2430730249217,-8.09329558710638));
#39272=CARTESIAN_POINT('Ctrl Pts',(5.9753829567149,6.26240242359787,-8.08941218546347));
#39273=CARTESIAN_POINT('Ctrl Pts',(5.9690941845529,6.28237372842147,-8.0859965229583));
#39274=CARTESIAN_POINT('Ctrl Pts',(5.96738487036364,6.28780201137298,-8.08506813181366));
#39275=CARTESIAN_POINT('Ctrl Pts',(5.96559359427533,6.29327747202086,-8.08417444780743));
#39276=CARTESIAN_POINT('Ctrl Pts',(5.96371764308482,6.29879711683061,-8.08331854647735));
#39277=CARTESIAN_POINT('Ctrl Pts',(5.96344414264071,6.29960184208914,-8.08319376210392));
#39278=CARTESIAN_POINT('Ctrl Pts',(5.96316884226125,6.30040750604515,-8.08306978112478));
#39279=CARTESIAN_POINT('Ctrl Pts',(5.96289173650296,6.3012141001333,-8.08294661136472));
#39280=CARTESIAN_POINT('Ctrl Pts',(5.9583064281901,6.31456092699193,-8.08090850386324));
#39281=CARTESIAN_POINT('Ctrl Pts',(5.95322667453022,6.32816314002302,-8.07909218307997));
#39282=CARTESIAN_POINT('Ctrl Pts',(5.94762863024084,6.34197741559306,-8.07753518789005));
#39283=CARTESIAN_POINT('Ctrl Pts',(5.94482960809616,6.34888455337808,-8.07675669029508));
#39284=CARTESIAN_POINT('Ctrl Pts',(5.9419009720458,6.35584469171829,-8.0760430429858));
#39285=CARTESIAN_POINT('Ctrl Pts',(5.93883992577041,6.36285141390253,-8.07539941117091));
#39286=CARTESIAN_POINT('Ctrl Pts',(5.93730940263271,6.36635477499465,-8.07507759526346));
#39287=CARTESIAN_POINT('Ctrl Pts',(5.93574577369783,6.36986978092234,-8.07477328464124));
#39288=CARTESIAN_POINT('Ctrl Pts',(5.93414868582103,6.37339558875165,-8.07448714829654));
#39289=CARTESIAN_POINT('Ctrl Pts',(5.93308462461123,6.37574466133484,-8.07429650970393));
#39290=CARTESIAN_POINT('Ctrl Pts',(5.93173682852077,6.37868274802833,-8.07406994874411));
#39291=CARTESIAN_POINT('Ctrl Pts',(5.93064071574464,6.38104120075807,-8.07389688260559));
#39292=CARTESIAN_POINT('Ctrl Pts',(5.93009163329116,6.38222263485816,-8.07381018753003));
#39293=CARTESIAN_POINT('Ctrl Pts',(5.92960659975964,6.38325892810984,-8.07373631728435));
#39294=CARTESIAN_POINT('Ctrl Pts',(5.9292566846022,6.38400455129654,-8.0736839462418));
#39295=CARTESIAN_POINT('Ctrl Pts',(5.92324504417235,6.39681456652238,-8.07278419705961));
#39296=CARTESIAN_POINT('Ctrl Pts',(5.91644349452928,6.41051100296279,-8.07208320363119));
#39297=CARTESIAN_POINT('Ctrl Pts',(5.90871320068971,6.42498790319228,-8.07170835271769));
#39298=CARTESIAN_POINT('Ctrl Pts',(5.90756565183023,6.42713697419681,-8.07165270674262));
#39299=CARTESIAN_POINT('Ctrl Pts',(5.90639762303351,6.42930316709509,-8.07160429984891));
#39300=CARTESIAN_POINT('Ctrl Pts',(5.90520864691648,6.43148605064041,-8.07156360519117));
#39301=CARTESIAN_POINT('Ctrl Pts',(5.89737763223853,6.44586328903806,-8.07129557586956));
#39302=CARTESIAN_POINT('Ctrl Pts',(5.8886373033292,6.46096801579065,-8.0713603304539));
#39303=CARTESIAN_POINT('Ctrl Pts',(5.8788707448158,6.476664087043,-8.07189275843248));
#39304=CARTESIAN_POINT('Ctrl Pts',(5.86988435735373,6.49110632662129,-8.07238265506339));
#39305=CARTESIAN_POINT('Ctrl Pts',(5.86002898431128,6.50604936554337,-8.07326842358738));
#39306=CARTESIAN_POINT('Ctrl Pts',(5.84922135971914,6.5213497229377,-8.07467428281701));
#39307=CARTESIAN_POINT('Ctrl Pts',(5.84083256968025,6.53322573552555,-8.07576549928192));
#39308=CARTESIAN_POINT('Ctrl Pts',(5.83187018337614,6.54531643423985,-8.07717034591712));
#39309=CARTESIAN_POINT('Ctrl Pts',(5.82229986758076,6.55753571914848,-8.07895670244825));
#39310=CARTESIAN_POINT('Ctrl Pts',(5.81046703764842,6.57264375981402,-8.08116537073919));
#39311=CARTESIAN_POINT('Ctrl Pts',(5.79770346605293,6.58794939970163,-8.08395721212972));
#39312=CARTESIAN_POINT('Ctrl Pts',(5.7839788211146,6.60327161378152,-8.08745539557388));
#39313=CARTESIAN_POINT('Ctrl Pts',(5.77112680734696,6.61761962112088,-8.09073115986419));
#39314=CARTESIAN_POINT('Ctrl Pts',(5.75743192856449,6.63198234755227,-8.09462614689545));
#39315=CARTESIAN_POINT('Ctrl Pts',(5.74289151150233,6.64617322509536,-8.09925657783635));
#39316=CARTESIAN_POINT('Ctrl Pts',(5.73956595888168,6.64941883420004,-8.10031560810243));
#39317=CARTESIAN_POINT('Ctrl Pts',(5.7361962789524,6.65265528125112,-8.10141318019669));
#39318=CARTESIAN_POINT('Ctrl Pts',(5.73278262922815,6.65588001261884,-8.10255081990868));
#39319=CARTESIAN_POINT('Ctrl Pts',(5.99928507670221,9.87990142103655,-16.9962137655509));
#39320=CARTESIAN_POINT('Ctrl Pts',(5.99928507670221,9.88326637139441,-16.9632224657788));
#39321=CARTESIAN_POINT('Ctrl Pts',(5.99928507670221,9.93380713709435,-16.4417148893617));
#39322=CARTESIAN_POINT('Ctrl Pts',(5.99928507670221,9.95153405412758,-15.4241459871747));
#39323=CARTESIAN_POINT('Ctrl Pts',(5.99928507670221,9.75855490567037,-13.9623406694731));
#39324=CARTESIAN_POINT('Ctrl Pts',(5.99928507670221,9.35132588134331,-12.5448516866735));
#39325=CARTESIAN_POINT('Ctrl Pts',(5.99928507670221,8.73824250065081,-11.2027103817564));
#39326=CARTESIAN_POINT('Ctrl Pts',(5.99928507670221,7.93284474685238,-9.96535729518426));
#39327=CARTESIAN_POINT('Ctrl Pts',(5.99928507670221,7.00873360046685,-8.92486257056714));
#39328=CARTESIAN_POINT('Ctrl Pts',(5.99928507670221,6.32620211116035,-8.33936238043742));
#39329=CARTESIAN_POINT('Ctrl Pts',(5.99928507670221,6.00174809856699,-8.09410015407363));
#39330=CARTESIAN_POINT('Ctrl Pts',(6.01063087509513,10.0684345307133,-17.01545949762));
#39331=CARTESIAN_POINT('Ctrl Pts',(6.01063087509513,10.0718639576454,-16.9818342056501));
#39332=CARTESIAN_POINT('Ctrl Pts',(6.01063087509513,10.1233733290156,-16.4503125276442));
#39333=CARTESIAN_POINT('Ctrl Pts',(6.01063087509513,10.1414447974272,-15.4134144215648));
#39334=CARTESIAN_POINT('Ctrl Pts',(6.01063087509513,9.94474509956266,-13.9234401354667));
#39335=CARTESIAN_POINT('Ctrl Pts',(6.01063087509513,9.52975918464545,-12.4789637137856));
#39336=CARTESIAN_POINT('Ctrl Pts',(6.01063087509513,8.90489167184337,-11.1110056648205));
#39337=CARTESIAN_POINT('Ctrl Pts',(6.01063087509513,8.08411518316363,-9.85004045908981));
#39338=CARTESIAN_POINT('Ctrl Pts',(6.01063087509513,7.14224990779624,-8.78954725626183));
#39339=CARTESIAN_POINT('Ctrl Pts',(6.01063087509513,6.44671813919453,-8.19289533345759));
#39340=CARTESIAN_POINT('Ctrl Pts',(6.01063087509513,6.11602421034097,-7.94291818409647));
#39341=CARTESIAN_POINT('Ctrl Pts',(5.90351530093621,10.2248493207515,-17.0314265452415));
#39342=CARTESIAN_POINT('Ctrl Pts',(5.90351530093621,10.2283322400939,-16.9972752673821));
#39343=CARTESIAN_POINT('Ctrl Pts',(5.90351530093621,10.280645206398,-16.4574454805172));
#39344=CARTESIAN_POINT('Ctrl Pts',(5.90351530093621,10.2990025287459,-15.4045110751714));
#39345=CARTESIAN_POINT('Ctrl Pts',(5.90351530093621,10.0992161106988,-13.8911666590971));
#39346=CARTESIAN_POINT('Ctrl Pts',(5.90351530093621,9.6777947616339,-12.4243003527319));
#39347=CARTESIAN_POINT('Ctrl Pts',(5.90351530093621,9.04315065015506,-11.0349236754524));
#39348=CARTESIAN_POINT('Ctrl Pts',(5.90351530093621,8.20961533311243,-9.75436888852781));
#39349=CARTESIAN_POINT('Ctrl Pts',(5.90351530093621,7.25302050514079,-8.67728412904822));
#39350=CARTESIAN_POINT('Ctrl Pts',(5.90351530093621,6.54670317234504,-8.07138027204041));
#39351=CARTESIAN_POINT('Ctrl Pts',(5.90351530093621,6.21083235337873,-7.81749142944129));
#39352=CARTESIAN_POINT('Ctrl Pts',(5.72195027506538,10.2826708065042,-17.0373290459966));
#39353=CARTESIAN_POINT('Ctrl Pts',(5.72195027506538,10.2861735002605,-17.0029833281784));
#39354=CARTESIAN_POINT('Ctrl Pts',(5.72195027506538,10.3387835296056,-16.4600823023492));
#39355=CARTESIAN_POINT('Ctrl Pts',(5.72195027506538,10.3572465229012,-15.4012197961528));
#39356=CARTESIAN_POINT('Ctrl Pts',(5.72195027506538,10.1563190443011,-13.8792361993662));
#39357=CARTESIAN_POINT('Ctrl Pts',(5.72195027506538,9.73251872350333,-12.4040930772462));
#39358=CARTESIAN_POINT('Ctrl Pts',(5.72195027506538,9.0942605199016,-11.0067986262652));
#39359=CARTESIAN_POINT('Ctrl Pts',(5.72195027506538,8.25600867693205,-9.71900220515771));
#39360=CARTESIAN_POINT('Ctrl Pts',(5.72195027506538,7.29396881005966,-8.63578408414143));
#39361=CARTESIAN_POINT('Ctrl Pts',(5.72195027506538,6.58366440323806,-8.02646008648023));
#39362=CARTESIAN_POINT('Ctrl Pts',(5.72195027506538,6.24587985554049,-7.77112521748877));
#39363=CARTESIAN_POINT('',(6.,9.9133032909571,-16.8993688494793));
#39364=CARTESIAN_POINT('Ctrl Pts',(5.99999999999975,9.9133032909571,-16.8993688494793));
#39365=CARTESIAN_POINT('Ctrl Pts',(5.99999999999975,9.92726798889229,-16.7473133675693));
#39366=CARTESIAN_POINT('Ctrl Pts',(6.00000000003748,9.93769911293785,-16.5954478952856));
#39367=CARTESIAN_POINT('Ctrl Pts',(5.99999999795225,9.94464893033857,-16.4436798521367));
#39368=CARTESIAN_POINT('Ctrl Pts',(5.9999999958601,9.95162180848309,-16.2914082153307));
#39369=CARTESIAN_POINT('Ctrl Pts',(5.99999999148619,9.95509022596526,-16.139234192407));
#39370=CARTESIAN_POINT('Ctrl Pts',(5.9999999908736,9.95505464932154,-15.9870605228147));
#39371=CARTESIAN_POINT('Ctrl Pts',(5.999999990262,9.95501913067149,-15.8351349123105));
#39372=CARTESIAN_POINT('Ctrl Pts',(5.99999999695627,9.9514910077271,-15.6832091914971));
#39373=CARTESIAN_POINT('Ctrl Pts',(5.99999999953315,9.94441902101537,-15.5311897728051));
#39374=CARTESIAN_POINT('Ctrl Pts',(5.99999999982105,9.94362890698645,-15.5142054824956));
#39375=CARTESIAN_POINT('Ctrl Pts',(5.99999999999975,9.94279450412573,-15.497220030147));
#39376=CARTESIAN_POINT('Ctrl Pts',(5.99999999999975,9.9419157008945,-15.4802332916842));
#39377=CARTESIAN_POINT('Ctrl Pts',(5.99999999999975,9.94094263422146,-15.4614244975257));
#39378=CARTESIAN_POINT('Ctrl Pts',(5.99999999977976,9.93991612339977,-15.4426140377054));
#39379=CARTESIAN_POINT('Ctrl Pts',(5.99999999940214,9.93883607995432,-15.4238025173435));
#39380=CARTESIAN_POINT('Ctrl Pts',(5.99999999572736,9.92832587000923,-15.2407422624791));
#39381=CARTESIAN_POINT('Ctrl Pts',(5.99999998184258,9.91274193221338,-15.057581311491));
#39382=CARTESIAN_POINT('Ctrl Pts',(5.99999998033336,9.89208012672901,-14.8748206135648));
#39383=CARTESIAN_POINT('Ctrl Pts',(5.99999997882273,9.8713991178155,-14.6918900547755));
#39384=CARTESIAN_POINT('Ctrl Pts',(5.99999998731005,9.84563081442832,-14.5093609439596));
#39385=CARTESIAN_POINT('Ctrl Pts',(5.99999999411988,9.8148232071059,-14.3277348674503));
#39386=CARTESIAN_POINT('Ctrl Pts',(5.99999999739303,9.80001548195328,-14.2404360067062));
#39387=CARTESIAN_POINT('Ctrl Pts',(5.99999999999975,9.78404431694916,-14.153345716758));
#39388=CARTESIAN_POINT('Ctrl Pts',(5.99999999999975,9.76691929497133,-14.0665191605846));
#39389=CARTESIAN_POINT('Ctrl Pts',(5.99999999999975,9.76020616508213,-14.0324825356869));
#39390=CARTESIAN_POINT('Ctrl Pts',(5.99999999960415,9.75331447298792,-13.9984866912186));
#39391=CARTESIAN_POINT('Ctrl Pts',(5.99999999898866,9.74624448648212,-13.9645326289129));
#39392=CARTESIAN_POINT('Ctrl Pts',(5.99999999507861,9.70133035239358,-13.7488296277829));
#39393=CARTESIAN_POINT('Ctrl Pts',(5.99999998615656,9.64922498996124,-13.5348122190641));
#39394=CARTESIAN_POINT('Ctrl Pts',(5.99999998771986,9.59004136500335,-13.3227629515009));
#39395=CARTESIAN_POINT('Ctrl Pts',(5.99999998928315,9.53085774004545,-13.1107136839378));
#39396=CARTESIAN_POINT('Ctrl Pts',(5.99999999999975,9.46459569652831,-12.900631951729));
#39397=CARTESIAN_POINT('Ctrl Pts',(5.99999999999975,9.39131591670037,-12.6928136411459));
#39398=CARTESIAN_POINT('Ctrl Pts',(5.99999999999975,9.3745538773706,-12.645277216997));
#39399=CARTESIAN_POINT('Ctrl Pts',(5.9999999993467,9.35742705664761,-12.5978581952024));
#39400=CARTESIAN_POINT('Ctrl Pts',(5.99999999845574,9.3399373333427,-12.5505645602474));
#39401=CARTESIAN_POINT('Ctrl Pts',(5.99999999449763,9.26223848888796,-12.3404605624882));
#39402=CARTESIAN_POINT('Ctrl Pts',(5.99999998895133,9.17737337514935,-12.1328324811753));
#39403=CARTESIAN_POINT('Ctrl Pts',(5.99999999115154,9.08561278925283,-11.9283201471139));
#39404=CARTESIAN_POINT('Ctrl Pts',(5.99999999312721,9.00321675921052,-11.7446791616438));
#39405=CARTESIAN_POINT('Ctrl Pts',(5.99999999999975,8.91526165194371,-11.5635505237571));
#39406=CARTESIAN_POINT('Ctrl Pts',(5.99999999999975,8.82197656077892,-11.3853836320773));
#39407=CARTESIAN_POINT('Ctrl Pts',(5.99999999999975,8.79096317958254,-11.3261506114601));
#39408=CARTESIAN_POINT('Ctrl Pts',(5.99999999913628,8.7593588482401,-11.2672464903642));
#39409=CARTESIAN_POINT('Ctrl Pts',(5.99999999780776,8.72716730813645,-11.2086786366005));
#39410=CARTESIAN_POINT('Ctrl Pts',(5.99999999336884,8.6196079425489,-11.0129899191807));
#39411=CARTESIAN_POINT('Ctrl Pts',(5.99999998477715,8.50549634900011,-10.8210529986896));
#39412=CARTESIAN_POINT('Ctrl Pts',(5.99999998688354,8.38499562042057,-10.6331552723254));
#39413=CARTESIAN_POINT('Ctrl Pts',(5.99999998863009,8.28508034958788,-10.477356610858));
#39414=CARTESIAN_POINT('Ctrl Pts',(5.99999999999975,8.18077151927019,-10.3243353045956));
#39415=CARTESIAN_POINT('Ctrl Pts',(5.99999999999975,8.07214108602125,-10.1742724294256));
#39416=CARTESIAN_POINT('Ctrl Pts',(5.99999999999975,8.02304710815971,-10.1064536492633));
#39417=CARTESIAN_POINT('Ctrl Pts',(5.99999999683356,7.97307828550649,-10.0392309360628));
#39418=CARTESIAN_POINT('Ctrl Pts',(5.99999999319076,7.92225874095039,-9.9726436577022));
#39419=CARTESIAN_POINT('Ctrl Pts',(5.99999998466668,7.8033417060917,-9.81683034274397));
#39420=CARTESIAN_POINT('Ctrl Pts',(5.9999999759598,7.67976357121808,-9.66449894127245));
#39421=CARTESIAN_POINT('Ctrl Pts',(5.99999997954455,7.55191355600678,-9.51606320039813));
#39422=CARTESIAN_POINT('Ctrl Pts',(5.9999999831293,7.42406354079548,-9.36762745952381));
#39423=CARTESIAN_POINT('Ctrl Pts',(5.99999999999975,7.29194203564635,-9.22308774629525));
#39424=CARTESIAN_POINT('Ctrl Pts',(5.99999999999975,7.15597859955101,-9.08281763782801));
#39425=CARTESIAN_POINT('Ctrl Pts',(5.99999999999975,7.08650989506377,-9.01114849652541));
#39426=CARTESIAN_POINT('Ctrl Pts',(5.99999999545169,7.0160267676778,-8.94061363520937));
#39427=CARTESIAN_POINT('Ctrl Pts',(5.99999999307294,6.94451383265442,-8.87118228508652));
#39428=CARTESIAN_POINT('Ctrl Pts',(5.9999999894094,6.83437642276922,-8.76425073396415));
#39429=CARTESIAN_POINT('Ctrl Pts',(5.99999999031164,6.72179810473437,-8.65993478356875));
#39430=CARTESIAN_POINT('Ctrl Pts',(5.99999999276244,6.60672174345137,-8.55816514811733));
#39431=CARTESIAN_POINT('Ctrl Pts',(5.99999999520029,6.4922534941214,-8.45693330627604));
#39432=CARTESIAN_POINT('Ctrl Pts',(5.99999999786784,6.37531319152282,-8.35822062896864));
#39433=CARTESIAN_POINT('Ctrl Pts',(5.99999999875695,6.25581047945977,-8.26199732529102));
#39434=CARTESIAN_POINT('Ctrl Pts',(5.99999999915085,6.20286622544753,-8.21936673604451));
#39435=CARTESIAN_POINT('Ctrl Pts',(5.99999999931877,6.14941859523291,-8.17722530242187));
#39436=CARTESIAN_POINT('Ctrl Pts',(5.99999999931449,6.09545783381438,-8.1355731127727));
#39437=CARTESIAN_POINT('',(5.73644276520417,10.287735094912,-16.9337809954845));
#39438=CARTESIAN_POINT('Origin',(5.6,9.91330329093393,-16.8993688493888));
#39439=CARTESIAN_POINT('Ctrl Pts',(5.73644276397747,10.2877350956482,-16.9337809951853));
#39440=CARTESIAN_POINT('Ctrl Pts',(5.73708792252488,10.3280497910532,-16.4922345426347));
#39441=CARTESIAN_POINT('Ctrl Pts',(5.7376256311147,10.3398885430833,-16.0482066703703));
#39442=CARTESIAN_POINT('Ctrl Pts',(5.73805595543757,10.3232537068247,-15.6057356194698));
#39443=CARTESIAN_POINT('Ctrl Pts',(5.73812189675439,10.3207046456871,-15.5379329827125));
#39444=CARTESIAN_POINT('Ctrl Pts',(5.73818531651987,10.3174869811684,-15.4701668027555));
#39445=CARTESIAN_POINT('Ctrl Pts',(5.73824621494101,10.3136007167544,-15.4024515020653));
#39446=CARTESIAN_POINT('Ctrl Pts',(5.73865147313059,10.2877389546408,-14.9518293077615));
#39447=CARTESIAN_POINT('Ctrl Pts',(5.7389450772283,10.2322696006654,-14.503464432552));
#39448=CARTESIAN_POINT('Ctrl Pts',(5.73912707304533,10.1478940723348,-14.0611488527984));
#39449=CARTESIAN_POINT('Ctrl Pts',(5.73915087280122,10.1368602089777,-14.0033068485553));
#39450=CARTESIAN_POINT('Ctrl Pts',(5.73917276389785,10.1253320034285,-13.9455682225513));
#39451=CARTESIAN_POINT('Ctrl Pts',(5.73919274639698,10.1133110090545,-13.8879413913271));
#39452=CARTESIAN_POINT('Ctrl Pts',(5.73934700322873,10.0205137821125,-13.4430855026459));
#39453=CARTESIAN_POINT('Ctrl Pts',(5.73938752575328,9.8983518130802,-13.0048956732406));
#39454=CARTESIAN_POINT('Ctrl Pts',(5.73931432088869,9.74808603084931,-12.5770820026694));
#39455=CARTESIAN_POINT('Ctrl Pts',(5.73930537010441,9.72971298134816,-12.524773076246));
#39456=CARTESIAN_POINT('Ctrl Pts',(5.73929471904359,9.71091975480985,-12.4726192145084));
#39457=CARTESIAN_POINT('Ctrl Pts',(5.73928236767902,9.6917086361614,-12.4206271498742));
#39458=CARTESIAN_POINT('Ctrl Pts',(5.73918135761153,9.53459916217931,-11.9954334859653));
#39459=CARTESIAN_POINT('Ctrl Pts',(5.73896663330746,9.34954312181862,-11.5810645646298));
#39460=CARTESIAN_POINT('Ctrl Pts',(5.73863815941398,9.13842847138387,-11.181029202796));
#39461=CARTESIAN_POINT('Ctrl Pts',(5.73859603622718,9.11135532483154,-11.1297290398053));
#39462=CARTESIAN_POINT('Ctrl Pts',(5.73855204235336,9.08385360099182,-11.0786645361034));
#39463=CARTESIAN_POINT('Ctrl Pts',(5.73850617767971,9.05592724924063,-11.0278430391023));
#39464=CARTESIAN_POINT('Ctrl Pts',(5.73815298354927,8.84087233358326,-10.636477462656));
#39465=CARTESIAN_POINT('Ctrl Pts',(5.73768884857257,8.60063848073488,-10.2595258684371));
#39466=CARTESIAN_POINT('Ctrl Pts',(5.73711370894741,8.33732017512975,-9.90009892045526));
#39467=CARTESIAN_POINT('Ctrl Pts',(5.73703020601639,8.29908971882023,-9.8479147162477));
#39468=CARTESIAN_POINT('Ctrl Pts',(5.73694436301577,8.26037260623242,-9.79609985173272));
#39469=CARTESIAN_POINT('Ctrl Pts',(5.73685617976038,8.22117519680522,-9.74466378006768));
#39470=CARTESIAN_POINT('Ctrl Pts',(5.73622837043537,7.94211429067454,-9.37847129499271));
#39471=CARTESIAN_POINT('Ctrl Pts',(5.73548194360524,7.6387126294289,-9.03148082705006));
#39472=CARTESIAN_POINT('Ctrl Pts',(5.73461683428776,7.31393910142934,-8.70646898025495));
#39473=CARTESIAN_POINT('Ctrl Pts',(5.73452245153485,7.27850656241392,-8.6710104408445));
#39474=CARTESIAN_POINT('Ctrl Pts',(5.73442665616088,7.2428196026404,-8.63581347234199));
#39475=CARTESIAN_POINT('Ctrl Pts',(5.73432944809515,7.20688204886513,-8.60088165646185));
#39476=CARTESIAN_POINT('Ctrl Pts',(5.73384873467085,7.02916362182739,-8.42813680547361));
#39477=CARTESIAN_POINT('Ctrl Pts',(5.73333347356617,6.84531724366401,-8.26187651448214));
#39478=CARTESIAN_POINT('Ctrl Pts',(5.73278365817643,6.65588188893571,-8.10254858487398));
#39479=CARTESIAN_POINT('Ctrl Pts',(5.99999999997502,9.67862872910777,-17.034853315691));
#39480=CARTESIAN_POINT('Ctrl Pts',(5.99999999997502,9.75700380810234,-16.9899528681557));
#39481=CARTESIAN_POINT('Ctrl Pts',(5.99999999997502,9.83522889702098,-16.9447896029538));
#39482=CARTESIAN_POINT('Ctrl Pts',(5.99999999997502,9.91330177297949,-16.8993645966845));
#39483=CARTESIAN_POINT('Ctrl Pts',(6.00000263486395,9.79664482225177,-17.2408547729095));
#39484=CARTESIAN_POINT('Ctrl Pts',(6.00000263486394,9.87548026830594,-17.1956905812719));
#39485=CARTESIAN_POINT('Ctrl Pts',(6.00000263486394,9.95416475310123,-17.1502620839831));
#39486=CARTESIAN_POINT('Ctrl Pts',(6.00000263486394,10.0326962223333,-17.1045702551542));
#39487=CARTESIAN_POINT('Ctrl Pts',(5.83074066841807,9.87940002138452,-17.3853070349662));
#39488=CARTESIAN_POINT('Ctrl Pts',(5.83074066841807,9.95855828584937,-17.3399579007904));
#39489=CARTESIAN_POINT('Ctrl Pts',(5.83074066841807,10.0375649080452,-17.2943434175634));
#39490=CARTESIAN_POINT('Ctrl Pts',(5.83074066841807,10.1164179518752,-17.2484644875228));
#39491=CARTESIAN_POINT('Ctrl Pts',(5.59336110044111,9.87744127562583,-17.3818879717702));
#39492=CARTESIAN_POINT('Ctrl Pts',(5.5933611004411,9.95659189925281,-17.336543215031));
#39493=CARTESIAN_POINT('Ctrl Pts',(5.5933611004411,10.0355908967276,-17.2909331339334));
#39494=CARTESIAN_POINT('Ctrl Pts',(5.59336110044111,10.1144363291584,-17.2450586324212));
#39495=CARTESIAN_POINT('',(5.99999999995607,9.6786359708514,-17.0348513552255));
#39496=CARTESIAN_POINT('',(5.59336167792738,9.87744147097414,-17.3818877029268));
#39497=CARTESIAN_POINT('Origin',(5.6,9.67863108576213,-17.0348569102136));
#39498=CARTESIAN_POINT('',(5.59336169562615,10.114435612724,-17.2450590602278));
#39499=CARTESIAN_POINT('Origin',(5.59336169593387,7.59771250744744,-13.0386810382369));
#39500=CARTESIAN_POINT('Origin',(5.6,9.9133032910197,-16.8993688495356));
#39501=CARTESIAN_POINT('Ctrl Pts',(5.99999999999158,9.67863900758284,-17.0348496155196));
#39502=CARTESIAN_POINT('Ctrl Pts',(5.99999999999163,9.70480912503784,-17.0198569671163));
#39503=CARTESIAN_POINT('Ctrl Pts',(5.99999999999965,9.73095807855235,-17.0048396407998));
#39504=CARTESIAN_POINT('Ctrl Pts',(5.99999999999965,9.75705557048624,-16.9898117781375));
#39505=CARTESIAN_POINT('Ctrl Pts',(5.99999999999965,9.78315306242015,-16.9747839154753));
#39506=CARTESIAN_POINT('Ctrl Pts',(5.99999999999965,9.80919909277344,-16.9597455164675));
#39507=CARTESIAN_POINT('Ctrl Pts',(5.99999999999965,9.83523570690332,-16.9446741822047));
#39508=CARTESIAN_POINT('Ctrl Pts',(5.99999999999965,9.86127232103318,-16.9296028479419));
#39509=CARTESIAN_POINT('Ctrl Pts',(5.99999999999965,9.88729951893964,-16.9144985784241));
#39510=CARTESIAN_POINT('Ctrl Pts',(5.99999999999965,9.9133032909571,-16.8993688494793));
#39511=CARTESIAN_POINT('Origin',(5.6,9.91330329093393,-16.8993688493888));
#39512=CARTESIAN_POINT('Origin',(5.600000004205,9.91330328921885,-16.89936884964));
#39513=CARTESIAN_POINT('Ctrl Pts',(-5.69266449220542,10.0630786776781,-17.2766466781631));
#39514=CARTESIAN_POINT('Ctrl Pts',(-5.65790043414258,10.0769849565476,-17.2678633469364));
#39515=CARTESIAN_POINT('Ctrl Pts',(-5.5437267087947,10.1222517047768,-17.2393085839034));
#39516=CARTESIAN_POINT('Ctrl Pts',(-5.34117223040521,10.2002049877122,-17.1903129318253));
#39517=CARTESIAN_POINT('Ctrl Pts',(-5.07577265985758,10.297830631585,-17.1291595099684));
#39518=CARTESIAN_POINT('Ctrl Pts',(-4.78281831444695,10.4000147575524,-17.0653012548397));
#39519=CARTESIAN_POINT('Ctrl Pts',(-4.459303684198,10.5059980087032,-16.9991848074578));
#39520=CARTESIAN_POINT('Ctrl Pts',(-4.10061258277721,10.6150315669163,-16.9312623156144));
#39521=CARTESIAN_POINT('Ctrl Pts',(-3.70134336606163,10.7258673035538,-16.8623066013417));
#39522=CARTESIAN_POINT('Ctrl Pts',(-3.25666787469216,10.8361817865208,-16.7937662678905));
#39523=CARTESIAN_POINT('Ctrl Pts',(-2.76258823483561,10.9424713829379,-16.7278268451725));
#39524=CARTESIAN_POINT('Ctrl Pts',(-2.21451513067802,11.0403077748057,-16.6672462944136));
#39525=CARTESIAN_POINT('Ctrl Pts',(-1.60542524853154,11.1242578061128,-16.6153980051002));
#39526=CARTESIAN_POINT('Ctrl Pts',(-0.938874874821314,11.1858352943571,
-16.5775066099776));
#39527=CARTESIAN_POINT('Ctrl Pts',(-0.236583627876225,11.2158495117354,
-16.5591684729001));
#39528=CARTESIAN_POINT('Ctrl Pts',(0.464299974377318,11.2096961977306,-16.5629105136066));
#39529=CARTESIAN_POINT('Ctrl Pts',(1.12891944157671,11.1708591884219,-16.5867080644657));
#39530=CARTESIAN_POINT('Ctrl Pts',(1.7341925532243,11.1079134256571,-16.6254836732421));
#39531=CARTESIAN_POINT('Ctrl Pts',(2.27383258279207,11.0299199389491,-16.6736769266626));
#39532=CARTESIAN_POINT('Ctrl Pts',(2.75210078338438,10.9437404518917,-16.7270452561121));
#39533=CARTESIAN_POINT('Ctrl Pts',(3.17956543253272,10.853147213274,-16.7832390598775));
#39534=CARTESIAN_POINT('Ctrl Pts',(3.5623527668001,10.7611441717712,-16.8403830088143));
#39535=CARTESIAN_POINT('Ctrl Pts',(3.90389408990394,10.6703808055596,-16.8968212209322));
#39536=CARTESIAN_POINT('Ctrl Pts',(4.20698802429124,10.5830107962021,-16.9512062257095));
#39537=CARTESIAN_POINT('Ctrl Pts',(4.47552839545299,10.5002685691408,-17.0027635436686));
#39538=CARTESIAN_POINT('Ctrl Pts',(4.71437785352944,10.4224860455875,-17.0512827690776));
#39539=CARTESIAN_POINT('Ctrl Pts',(4.92834708065183,10.3494750576525,-17.0968803214851));
#39540=CARTESIAN_POINT('Ctrl Pts',(5.12117811678946,10.2809937453109,-17.1397088463255));
#39541=CARTESIAN_POINT('Ctrl Pts',(5.29544566343547,10.2169300062458,-17.1798421134489));
#39542=CARTESIAN_POINT('Ctrl Pts',(5.45302101893722,10.157239981754,-17.2173121704573));
#39543=CARTESIAN_POINT('Ctrl Pts',(5.58355363523492,10.1064790825782,-17.2492564746078));
#39544=CARTESIAN_POINT('Ctrl Pts',(5.66171595239179,10.0754576838054,-17.2688281128496));
#39545=CARTESIAN_POINT('Ctrl Pts',(5.69263813280236,10.0630831778572,-17.2766441366971));
#39546=CARTESIAN_POINT('Ctrl Pts',(-5.75649847130068,10.1846663672687,-17.2128693097372));
#39547=CARTESIAN_POINT('Ctrl Pts',(-5.72140233477174,10.1986663653251,-17.2039323534534));
#39548=CARTESIAN_POINT('Ctrl Pts',(-5.60613809903996,10.2442347264077,-17.1748721512905));
#39549=CARTESIAN_POINT('Ctrl Pts',(-5.40164464106496,10.3226877205043,-17.1249718090535));
#39550=CARTESIAN_POINT('Ctrl Pts',(-5.13367468755091,10.4209044324657,-17.0626072240043));
#39551=CARTESIAN_POINT('Ctrl Pts',(-4.83782850255198,10.5236835645344,-16.9974065461764));
#39552=CARTESIAN_POINT('Ctrl Pts',(-4.51104444500548,10.6302690096379,-16.9298277212577));
#39553=CARTESIAN_POINT('Ctrl Pts',(-4.1486314623029,10.7399132384906,-16.8603335925331));
#39554=CARTESIAN_POINT('Ctrl Pts',(-3.74510048327725,10.8513637000167,-16.7897128297027));
#39555=CARTESIAN_POINT('Ctrl Pts',(-3.29553742458152,10.962283478546,-16.7194451614527));
#39556=CARTESIAN_POINT('Ctrl Pts',(-2.7958661187274,11.0691454406598,-16.6517671786418));
#39557=CARTESIAN_POINT('Ctrl Pts',(-2.24141575844614,11.1674897314513,-16.5895078340631));
#39558=CARTESIAN_POINT('Ctrl Pts',(-1.62506220435505,11.2518450143852,-16.5361367827504));
#39559=CARTESIAN_POINT('Ctrl Pts',(-0.950407621639583,11.3136805721432,
-16.4970514102802));
#39560=CARTESIAN_POINT('Ctrl Pts',(-0.239487242992564,11.3437787953034,
-16.4780680325047));
#39561=CARTESIAN_POINT('Ctrl Pts',(0.470002985040156,11.3376139729618,-16.481950388767));
#39562=CARTESIAN_POINT('Ctrl Pts',(1.14277369818418,11.298645972153,-16.5065505464812));
#39563=CARTESIAN_POINT('Ctrl Pts',(1.75537383649425,11.2354239707746,-16.546524035722));
#39564=CARTESIAN_POINT('Ctrl Pts',(2.30142541400522,11.1570481890557,-16.596117814153));
#39565=CARTESIAN_POINT('Ctrl Pts',(2.78525130109912,11.070420416641,-16.650960905252));
#39566=CARTESIAN_POINT('Ctrl Pts',(3.21756581506068,10.9793406103684,-16.7086420451774));
#39567=CARTESIAN_POINT('Ctrl Pts',(3.60459046008406,10.8868345951884,-16.7672410214692));
#39568=CARTESIAN_POINT('Ctrl Pts',(3.94982144119845,10.7955698330654,-16.825065578703));
#39569=CARTESIAN_POINT('Ctrl Pts',(4.25611430913495,10.7077133982218,-16.8807415416324));
#39570=CARTESIAN_POINT('Ctrl Pts',(4.52742836500013,10.6245066330647,-16.9334823385126));
#39571=CARTESIAN_POINT('Ctrl Pts',(4.76869700926165,10.5462824671219,-16.9830781635062));
#39572=CARTESIAN_POINT('Ctrl Pts',(4.98479617406326,10.4728502980132,-17.0296522864356));
#39573=CARTESIAN_POINT('Ctrl Pts',(5.17951842452041,10.4039652420616,-17.0733639174592));
#39574=CARTESIAN_POINT('Ctrl Pts',(5.35547481853325,10.3395129283266,-17.1142914029171));
#39575=CARTESIAN_POINT('Ctrl Pts',(5.51456432417527,10.2794482765431,-17.1524714666152));
#39576=CARTESIAN_POINT('Ctrl Pts',(5.6463454610272,10.2283569966615,-17.1849961244044));
#39577=CARTESIAN_POINT('Ctrl Pts',(5.725254241073,10.1971289896351,-17.2049142863281));
#39578=CARTESIAN_POINT('Ctrl Pts',(5.75647140922376,10.1846721566233,-17.2128686091087));
#39579=CARTESIAN_POINT('Ctrl Pts',(-5.81361946724638,10.2517345378954,-17.0898695141078));
#39580=CARTESIAN_POINT('Ctrl Pts',(-5.77819683786477,10.2657915777574,-17.0808120712885));
#39581=CARTESIAN_POINT('Ctrl Pts',(-5.66186464174654,10.3115378871638,-17.0513579268557));
#39582=CARTESIAN_POINT('Ctrl Pts',(-5.45549338217626,10.3902536999524,-17.0007658028942));
#39583=CARTESIAN_POINT('Ctrl Pts',(-5.18505974968072,10.4887222308117,-16.9374961909567));
#39584=CARTESIAN_POINT('Ctrl Pts',(-4.88646802673155,10.5917039029127,-16.8713094772743));
#39585=CARTESIAN_POINT('Ctrl Pts',(-4.55661094832552,10.698450768387,-16.8026713211113));
#39586=CARTESIAN_POINT('Ctrl Pts',(-4.19073768336938,10.8082203686742,-16.7320525697056));
#39587=CARTESIAN_POINT('Ctrl Pts',(-3.78329110953657,10.9197603181983,-16.6602542945024));
#39588=CARTESIAN_POINT('Ctrl Pts',(-3.32929383344923,11.0307292683044,-16.588779762711));
#39589=CARTESIAN_POINT('Ctrl Pts',(-2.82461592253986,11.1375921938474,-16.5199028072177));
#39590=CARTESIAN_POINT('Ctrl Pts',(-2.26453145297425,11.235880624647,-16.4565023553868));
#39591=CARTESIAN_POINT('Ctrl Pts',(-1.64184500498462,11.3201177955775,-16.402113388426));
#39592=CARTESIAN_POINT('Ctrl Pts',(-0.960212638605293,11.381790604117,-16.3622452378034));
#39593=CARTESIAN_POINT('Ctrl Pts',(-0.241942357302399,11.4117378642006,
-16.3428500559305));
#39594=CARTESIAN_POINT('Ctrl Pts',(0.474833609088317,11.405613463525,-16.3468207371218));
#39595=CARTESIAN_POINT('Ctrl Pts',(1.15457138884398,11.3668033364056,-16.3719381825921));
#39596=CARTESIAN_POINT('Ctrl Pts',(1.77349849179209,11.3037244443956,-16.4127012242899));
#39597=CARTESIAN_POINT('Ctrl Pts',(2.32515189705749,11.2254457645873,-16.4632340183868));
#39598=CARTESIAN_POINT('Ctrl Pts',(2.81389080815452,11.1388643635119,-16.5190803431333));
#39599=CARTESIAN_POINT('Ctrl Pts',(3.25054254209914,11.0477876676189,-16.5777860337094));
#39600=CARTESIAN_POINT('Ctrl Pts',(3.64139929966152,10.9552493865708,-16.6373985951458));
#39601=CARTESIAN_POINT('Ctrl Pts',(3.99000282473668,10.8639241945068,-16.6961988316824));
#39602=CARTESIAN_POINT('Ctrl Pts',(4.29924871552588,10.7759851546574,-16.7527920773989));
#39603=CARTESIAN_POINT('Ctrl Pts',(4.57314637444018,10.692677781047,-16.8063815627452));
#39604=CARTESIAN_POINT('Ctrl Pts',(4.81668678414937,10.6143370339782,-16.85675657135));
#39605=CARTESIAN_POINT('Ctrl Pts',(5.03480081202369,10.5407725073575,-16.9040443288795));
#39606=CARTESIAN_POINT('Ctrl Pts',(5.23132417481802,10.4717385146491,-16.9484081620974));
#39607=CARTESIAN_POINT('Ctrl Pts',(5.40889929673994,10.4071198003723,-16.9899293333123));
#39608=CARTESIAN_POINT('Ctrl Pts',(5.56944961741275,10.3468714240165,-17.0286475895997));
#39609=CARTESIAN_POINT('Ctrl Pts',(5.70244435423125,10.295598206018,-17.0616190888325));
#39610=CARTESIAN_POINT('Ctrl Pts',(5.78208456369384,10.2642482618129,-17.0818074036475));
#39611=CARTESIAN_POINT('Ctrl Pts',(5.81359195404932,10.2517424965309,-17.0898698238178));
#39612=CARTESIAN_POINT('Ctrl Pts',(-5.84786850162611,10.2455091795785,-16.942757011536));
#39613=CARTESIAN_POINT('Ctrl Pts',(-5.81221746652095,10.2595705751324,-16.9336462242179));
#39614=CARTESIAN_POINT('Ctrl Pts',(-5.69514241486186,10.3053212667506,-16.9040207987418));
#39615=CARTESIAN_POINT('Ctrl Pts',(-5.48748642398773,10.3839895355852,-16.8531449384918));
#39616=CARTESIAN_POINT('Ctrl Pts',(-5.21539354735681,10.4823007198192,-16.7895316072133));
#39617=CARTESIAN_POINT('Ctrl Pts',(-4.91498002652965,10.5850367417634,-16.7229931586931));
#39618=CARTESIAN_POINT('Ctrl Pts',(-4.58311636433276,10.69146038893,-16.653997204036));
#39619=CARTESIAN_POINT('Ctrl Pts',(-4.21502391534534,10.800836602231,-16.5830176461027));
#39620=CARTESIAN_POINT('Ctrl Pts',(-3.80511608444942,10.9119176830569,-16.5108610123053));
#39621=CARTESIAN_POINT('Ctrl Pts',(-3.34839262726853,11.0223681180405,-16.4390398832391));
#39622=CARTESIAN_POINT('Ctrl Pts',(-2.84070950668018,11.128662768988,-16.3698410197423));
#39623=CARTESIAN_POINT('Ctrl Pts',(-2.27732756424709,11.2263498157947,-16.306158234012));
#39624=CARTESIAN_POINT('Ctrl Pts',(-1.65102971936692,11.3099812154025,-16.2515425131447));
#39625=CARTESIAN_POINT('Ctrl Pts',(-0.965518635472634,11.3711183727228,
-16.2115228624109));
#39626=CARTESIAN_POINT('Ctrl Pts',(-0.243255125004045,11.4007234847768,
-16.1920650191604));
#39627=CARTESIAN_POINT('Ctrl Pts',(0.477426609194236,11.394679759103,-16.1960472258656));
#39628=CARTESIAN_POINT('Ctrl Pts',(1.16097791888811,11.356270398663,-16.2212512619957));
#39629=CARTESIAN_POINT('Ctrl Pts',(1.78344318131467,11.2937116193071,-16.2621735172597));
#39630=CARTESIAN_POINT('Ctrl Pts',(2.33830463684603,11.2159798756401,-16.3129196770289));
#39631=CARTESIAN_POINT('Ctrl Pts',(2.82992234932633,11.1299242514357,-16.3690154106596));
#39632=CARTESIAN_POINT('Ctrl Pts',(3.26917171323198,11.0393373738254,-16.4279944912735));
#39633=CARTESIAN_POINT('Ctrl Pts',(3.66237112484065,10.9472446708381,-16.4878938370364));
#39634=CARTESIAN_POINT('Ctrl Pts',(4.01307568172585,10.8563152592409,-16.5469843393736));
#39635=CARTESIAN_POINT('Ctrl Pts',(4.32419287162572,10.7687191219718,-16.603862836127));
#39636=CARTESIAN_POINT('Ctrl Pts',(4.59975269123718,10.6857020288348,-16.6577271362962));
#39637=CARTESIAN_POINT('Ctrl Pts',(4.84477427515613,10.6076014135021,-16.7083643670323));
#39638=CARTESIAN_POINT('Ctrl Pts',(5.06421758701105,10.5342296300905,-16.7559017066983));
#39639=CARTESIAN_POINT('Ctrl Pts',(5.26194192432505,10.4653426280537,-16.8005029943812));
#39640=CARTESIAN_POINT('Ctrl Pts',(5.44060721984951,10.4008258962196,-16.8422499285557));
#39641=CARTESIAN_POINT('Ctrl Pts',(5.60215126518848,10.340635949735,-16.8811827769094));
#39642=CARTESIAN_POINT('Ctrl Pts',(5.73598090626615,10.2893801627774,-16.9143415437475));
#39643=CARTESIAN_POINT('Ctrl Pts',(5.81613029482418,10.2580271472924,-16.9346474073568));
#39644=CARTESIAN_POINT('Ctrl Pts',(5.84784091563367,10.2455195690895,-16.9427572183048));
#39645=CARTESIAN_POINT('',(-5.593361696257,10.114435612469,-17.2450590606623));
#39646=CARTESIAN_POINT('Ctrl Pts',(-5.593361696257,10.114435612469,-17.2450590606623));
#39647=CARTESIAN_POINT('Ctrl Pts',(-5.53988028306012,10.1354439865193,-17.23180878986));
#39648=CARTESIAN_POINT('Ctrl Pts',(-5.47937289761996,10.1588326290219,-17.2170754989487));
#39649=CARTESIAN_POINT('Ctrl Pts',(-5.378072861095,10.1973859622821,-17.1928371623116));
#39650=CARTESIAN_POINT('Ctrl Pts',(-5.34254968919255,10.2108081643024,-17.1844054697643));
#39651=CARTESIAN_POINT('Ctrl Pts',(-5.2866301917477,10.2317219773105,-17.1712769734231));
#39652=CARTESIAN_POINT('Ctrl Pts',(-5.25801175812749,10.2423733662331,-17.1645928615778));
#39653=CARTESIAN_POINT('Ctrl Pts',(-5.22840529716057,10.2532965141372,-17.1577411945075));
#39654=CARTESIAN_POINT('Ctrl Pts',(-5.20844809488337,10.2606364040394,-17.1531377696007));
#39655=CARTESIAN_POINT('Ctrl Pts',(-5.19640811531086,10.2650483759484,-17.1503710837434));
#39656=CARTESIAN_POINT('Ctrl Pts',(-5.12218902892848,10.2921680495835,-17.1333663951139));
#39657=CARTESIAN_POINT('Ctrl Pts',(-5.04952088095849,10.3182376312863,-17.1170332995621));
#39658=CARTESIAN_POINT('Ctrl Pts',(-4.93047521889172,10.3599563102957,-17.090921208127));
#39659=CARTESIAN_POINT('Ctrl Pts',(-4.86844152783038,10.3814640319628,-17.0774650732981));
#39660=CARTESIAN_POINT('Ctrl Pts',(-4.7916748832099,10.4075658113976,-17.0611442365309));
#39661=CARTESIAN_POINT('Ctrl Pts',(-4.75219305963743,10.4208496513771,-17.0528403485297));
#39662=CARTESIAN_POINT('Ctrl Pts',(-4.73503688497876,10.4265904842544,-17.0492521356902));
#39663=CARTESIAN_POINT('Ctrl Pts',(-4.72354712562239,10.4304280694972,-17.0468536144988));
#39664=CARTESIAN_POINT('Ctrl Pts',(-4.71663332011695,10.4327323041815,-17.0454135176634));
#39665=CARTESIAN_POINT('Ctrl Pts',(-4.56303751863232,10.4838416899302,-17.0134723230282));
#39666=CARTESIAN_POINT('Ctrl Pts',(-4.38712946317573,10.5399084731665,-16.9784638974453));
#39667=CARTESIAN_POINT('Ctrl Pts',(-4.08281737169274,10.6299894329539,-16.9222869539802));
#39668=CARTESIAN_POINT('Ctrl Pts',(-3.97463833981539,10.6609811182779,-16.9029696525196));
#39669=CARTESIAN_POINT('Ctrl Pts',(-3.80225728992482,10.7081749541802,-16.8735681800859));
#39670=CARTESIAN_POINT('Ctrl Pts',(-3.71353863946091,10.7319458246321,-16.8587626980378));
#39671=CARTESIAN_POINT('Ctrl Pts',(-3.60560932759541,10.7597947892436,-16.8414239018793));
#39672=CARTESIAN_POINT('Ctrl Pts',(-3.55053861674825,10.7737230309169,-16.8327539264673));
#39673=CARTESIAN_POINT('Ctrl Pts',(-3.52669987176067,10.7796903351693,-16.8290398219781));
#39674=CARTESIAN_POINT('Ctrl Pts',(-3.51075470582064,10.783667796514,-16.8265643021482));
#39675=CARTESIAN_POINT('Ctrl Pts',(-3.5015584239999,10.7859527405556,-16.825142240374));
#39676=CARTESIAN_POINT('Ctrl Pts',(-3.27623811862249,10.8417639726306,-16.7904085637452));
#39677=CARTESIAN_POINT('Ctrl Pts',(-3.02980309372394,10.8978171053894,-16.7555580309812));
#39678=CARTESIAN_POINT('Ctrl Pts',(-2.61823664503177,10.9783706192322,-16.7055410572012));
#39679=CARTESIAN_POINT('Ctrl Pts',(-2.47406217691032,11.0046130418625,-16.68925818084));
#39680=CARTESIAN_POINT('Ctrl Pts',(-2.24732199689207,11.0420890498694,-16.6660245528667));
#39681=CARTESIAN_POINT('Ctrl Pts',(-2.16999552391331,11.054265359023,-16.658479120914));
#39682=CARTESIAN_POINT('Ctrl Pts',(-2.01184975201042,11.0778120156048,-16.6438948098896));
#39683=CARTESIAN_POINT('Ctrl Pts',(-1.93305534133166,11.0889155988717,-16.6370209864462));
#39684=CARTESIAN_POINT('Ctrl Pts',(-1.51010234062083,11.1446314683416,-16.6025490483757));
#39685=CARTESIAN_POINT('Ctrl Pts',(-1.15547545530011,11.1793411116954,-16.5811403702837));
#39686=CARTESIAN_POINT('Ctrl Pts',(-0.599138400190915,11.2105411459179,
-16.5619612691803));
#39687=CARTESIAN_POINT('Ctrl Pts',(-0.409626593966499,11.2174664487711,
-16.5577208744858));
#39688=CARTESIAN_POINT('Ctrl Pts',(-0.119259702847854,11.2219241593423,
-16.5549970017463));
#39689=CARTESIAN_POINT('Ctrl Pts',(0.0274485381569757,11.2226707105659,
-16.5545430063037));
#39690=CARTESIAN_POINT('Ctrl Pts',(0.201276544692242,11.2207992343843,-16.555685031869));
#39691=CARTESIAN_POINT('Ctrl Pts',(0.276346060070852,11.2193954414903,-16.556543017445));
#39692=CARTESIAN_POINT('Ctrl Pts',(0.326519469943717,11.218324255164,-16.5571979302159));
#39693=CARTESIAN_POINT('Ctrl Pts',(0.353423748371615,11.2176742699932,-16.5575954345784));
#39694=CARTESIAN_POINT('Ctrl Pts',(0.752239173257733,11.2070497311517,-16.5640948719712));
#39695=CARTESIAN_POINT('Ctrl Pts',(1.10870726251511,11.1824492230569,-16.5792077214685));
#39696=CARTESIAN_POINT('Ctrl Pts',(1.61507798927156,11.1301017166863,-16.6115346913009));
#39697=CARTESIAN_POINT('Ctrl Pts',(1.86118050086738,11.1000689808603,-16.6301060277878));
#39698=CARTESIAN_POINT('Ctrl Pts',(2.13590510710996,11.0596864044952,-16.6551179812476));
#39699=CARTESIAN_POINT('Ctrl Pts',(2.25098815465266,11.0413827195364,-16.6664621426317));
#39700=CARTESIAN_POINT('Ctrl Pts',(2.32711994869927,11.0289750497037,-16.6741536414256));
#39701=CARTESIAN_POINT('Ctrl Pts',(2.36664743998163,11.0223685668864,-16.6782498198878));
#39702=CARTESIAN_POINT('Ctrl Pts',(2.68811795660455,10.9674606160988,-16.7123001593168));
#39703=CARTESIAN_POINT('Ctrl Pts',(2.94939629479706,10.9141967924827,-16.7453824107961));
#39704=CARTESIAN_POINT('Ctrl Pts',(3.30460395387738,10.8339032238938,-16.7953063331382));
#39705=CARTESIAN_POINT('Ctrl Pts',(3.41688819886941,10.8070585507245,-16.8120063272807));
#39706=CARTESIAN_POINT('Ctrl Pts',(3.57613710430534,10.7673178989158,-16.8367404354672));
#39707=CARTESIAN_POINT('Ctrl Pts',(3.65346719151028,10.7475775933703,-16.8490294893356));
#39708=CARTESIAN_POINT('Ctrl Pts',(3.73967048693491,10.7248990085834,-16.8631524446267));
#39709=CARTESIAN_POINT('Ctrl Pts',(3.77575436933522,10.7152671623837,-16.8691515896455));
#39710=CARTESIAN_POINT('Ctrl Pts',(3.79961909380934,10.7088667058967,-16.8731382911077));
#39711=CARTESIAN_POINT('Ctrl Pts',(3.80971292521982,10.7061487497407,-16.8748313201729));
#39712=CARTESIAN_POINT('Ctrl Pts',(4.03894258058649,10.6440870525456,-16.9134922223104));
#39713=CARTESIAN_POINT('Ctrl Pts',(4.23294189407636,10.5865357761191,-16.9493762692554));
#39714=CARTESIAN_POINT('Ctrl Pts',(4.49132149755771,10.5060702067502,-16.9995962783043));
#39715=CARTESIAN_POINT('Ctrl Pts',(4.57201147092592,10.4802061465832,-17.0157474374254));
#39716=CARTESIAN_POINT('Ctrl Pts',(4.68489158928988,10.4432294217741,-17.0388507172504));
#39717=CARTESIAN_POINT('Ctrl Pts',(4.73929293804978,10.4251937998733,-17.0501227569471));
#39718=CARTESIAN_POINT('Ctrl Pts',(4.79919343503098,10.4050054499792,-17.0627452020711));
#39719=CARTESIAN_POINT('Ctrl Pts',(4.82410056018608,10.3965411605049,-17.0680383274529));
#39720=CARTESIAN_POINT('Ctrl Pts',(4.8405354177543,10.390940564724,-17.0715408484918));
#39721=CARTESIAN_POINT('Ctrl Pts',(4.84701640186461,10.3887273506808,-17.0729250180429));
#39722=CARTESIAN_POINT('Ctrl Pts',(4.93430771376098,10.358813700624,-17.0916346102252));
#39723=CARTESIAN_POINT('Ctrl Pts',(5.00672900437769,10.3333491942336,-17.1075721097258));
#39724=CARTESIAN_POINT('Ctrl Pts',(5.10760446036601,10.297274985841,-17.1301685902159));
#39725=CARTESIAN_POINT('Ctrl Pts',(5.15610306837598,10.2797653186203,-17.1411413232466));
#39726=CARTESIAN_POINT('Ctrl Pts',(5.20929131774862,10.2603202481462,-17.1533350719783));
#39727=CARTESIAN_POINT('Ctrl Pts',(5.23135911177139,10.2522013363372,-17.1584280078407));
#39728=CARTESIAN_POINT('Ctrl Pts',(5.24590938112122,10.2468368234746,-17.1617934884257));
#39729=CARTESIAN_POINT('Ctrl Pts',(5.25204166646472,10.2445718761053,-17.1632145550785));
#39730=CARTESIAN_POINT('Ctrl Pts',(5.39102676460598,10.1931086596194,-17.1955073708392));
#39731=CARTESIAN_POINT('Ctrl Pts',(5.50207490988016,10.1502945569566,-17.2224423306575));
#39732=CARTESIAN_POINT('Ctrl Pts',(5.593361696298,10.1144356125401,-17.2450590604365));
#39733=CARTESIAN_POINT('',(-5.73644346265599,10.2877335026453,-16.9337808606183));
#39734=CARTESIAN_POINT('Origin',(-5.599999999997,9.91330329093349,-16.899368849389));
#39735=CARTESIAN_POINT('Ctrl Pts',(-5.73644387762288,10.2877346861591,-16.9337810352107));
#39736=CARTESIAN_POINT('Ctrl Pts',(-5.73644352459358,10.2877348228399,-16.9337809477608));
#39737=CARTESIAN_POINT('Ctrl Pts',(-5.73644317156403,10.2877349595207,-16.9337808603108));
#39738=CARTESIAN_POINT('Ctrl Pts',(-5.73644281853424,10.2877350962016,-16.9337807728608));
#39739=CARTESIAN_POINT('Ctrl Pts',(-5.67992307657405,10.3096175850451,-16.9197801051606));
#39740=CARTESIAN_POINT('Ctrl Pts',(-5.61717065511268,10.3335904563916,-16.9044747020212));
#39741=CARTESIAN_POINT('Ctrl Pts',(-5.54808297603754,10.3594537576529,-16.8879871425014));
#39742=CARTESIAN_POINT('Ctrl Pts',(-5.52952075197148,10.3664026145189,-16.883557325518));
#39743=CARTESIAN_POINT('Ctrl Pts',(-5.51050111168914,10.3734876798064,-16.8790422721391));
#39744=CARTESIAN_POINT('Ctrl Pts',(-5.49102186563804,10.3807044999465,-16.8744445705152));
#39745=CARTESIAN_POINT('Ctrl Pts',(-5.421960655898,10.4062908254154,-16.8581439993671));
#39746=CARTESIAN_POINT('Ctrl Pts',(-5.34712351064947,10.4335365033827,-16.8408025360917));
#39747=CARTESIAN_POINT('Ctrl Pts',(-5.26640088171051,10.4622164379704,-16.8225623695911));
#39748=CARTESIAN_POINT('Ctrl Pts',(-5.25085290357015,10.4677404775352,-16.8190491327979));
#39749=CARTESIAN_POINT('Ctrl Pts',(-5.2350865382652,10.4733175987422,-16.8155026320632));
#39750=CARTESIAN_POINT('Ctrl Pts',(-5.21910094042576,10.4789460078782,-16.8119239946774));
#39751=CARTESIAN_POINT('Ctrl Pts',(-5.19132695624702,10.4887250194524,-16.8057063343102));
#39752=CARTESIAN_POINT('Ctrl Pts',(-5.16289118481947,10.4986588865672,-16.7993916409934));
#39753=CARTESIAN_POINT('Ctrl Pts',(-5.1337891480606,10.5087377160842,-16.792986244664));
#39754=CARTESIAN_POINT('Ctrl Pts',(-5.06602703525961,10.5322055849584,-16.7780717150657));
#39755=CARTESIAN_POINT('Ctrl Pts',(-4.99465299111353,10.5564606256927,-16.7626646217621));
#39756=CARTESIAN_POINT('Ctrl Pts',(-4.91960734870379,10.5813652266411,-16.7468531387424));
#39757=CARTESIAN_POINT('Ctrl Pts',(-4.82891643643845,10.6114618572661,-16.7277453295043));
#39758=CARTESIAN_POINT('Ctrl Pts',(-4.73286349694366,10.6425084044306,-16.7080460567318));
#39759=CARTESIAN_POINT('Ctrl Pts',(-4.63133837398873,10.6742244178999,-16.6879363746291));
#39760=CARTESIAN_POINT('Ctrl Pts',(-4.61738997120669,10.6785818391729,-16.6851735319195));
#39761=CARTESIAN_POINT('Ctrl Pts',(-4.60333826776916,10.6829518303966,-16.6824029867582));
#39762=CARTESIAN_POINT('Ctrl Pts',(-4.58918296916372,10.6873335996056,-16.6796252516688));
#39763=CARTESIAN_POINT('Ctrl Pts',(-4.55700168044369,10.6972953096304,-16.6733102245267));
#39764=CARTESIAN_POINT('Ctrl Pts',(-4.52428495643809,10.7073179243454,-16.6669580163093));
#39765=CARTESIAN_POINT('Ctrl Pts',(-4.4910294131758,10.7173918284569,-16.6605748444745));
#39766=CARTESIAN_POINT('Ctrl Pts',(-4.45061997010429,10.7296328209282,-16.6528185309829));
#39767=CARTESIAN_POINT('Ctrl Pts',(-4.4094149533028,10.7419495710167,-16.6450164806071));
#39768=CARTESIAN_POINT('Ctrl Pts',(-4.36740824388631,10.7543239371829,-16.6371804442443));
#39769=CARTESIAN_POINT('Ctrl Pts',(-4.34640488917806,10.760511120266,-16.6332624260629));
#39770=CARTESIAN_POINT('Ctrl Pts',(-4.3252011074128,10.7667126935057,-16.6293359105165));
#39771=CARTESIAN_POINT('Ctrl Pts',(-4.30379613383866,10.7729262929956,-16.6254024423939));
#39772=CARTESIAN_POINT('Ctrl Pts',(-4.29309364705158,10.7760330927405,-16.6234357083326));
#39773=CARTESIAN_POINT('Ctrl Pts',(-4.28234086205917,10.7791428981615,-16.6214672360706));
#39774=CARTESIAN_POINT('Ctrl Pts',(-4.27153768256719,10.7822554080201,-16.6194972207862));
#39775=CARTESIAN_POINT('Ctrl Pts',(-4.2634352979482,10.784589790414,-16.6180197093228));
#39776=CARTESIAN_POINT('Ctrl Pts',(-4.25530456640277,10.7869256939804,-16.6165413299049));
#39777=CARTESIAN_POINT('Ctrl Pts',(-4.24714544723451,10.7892629901513,-16.6150621657675));
#39778=CARTESIAN_POINT('Ctrl Pts',(-4.24442574084509,10.790042088875,-16.6145691110551));
#39779=CARTESIAN_POINT('Ctrl Pts',(-4.24040612494836,10.7911921014736,-16.6138413435076));
#39780=CARTESIAN_POINT('Ctrl Pts',(-4.23897686402988,10.791600745692,-16.6135827432249));
#39781=CARTESIAN_POINT('Ctrl Pts',(-4.23363917081557,10.7931268613534,-16.612616979062));
#39782=CARTESIAN_POINT('Ctrl Pts',(-4.22827719948883,10.7946570374923,-16.6116486331607));
#39783=CARTESIAN_POINT('Ctrl Pts',(-4.22289092374133,10.7961912023985,-16.6106777518021));
#39784=CARTESIAN_POINT('Ctrl Pts',(-4.14210875622134,10.8192002669668,-16.5961166887915));
#39785=CARTESIAN_POINT('Ctrl Pts',(-4.05586011230241,10.8431100287053,-16.5809830331791));
#39786=CARTESIAN_POINT('Ctrl Pts',(-3.96405508318161,10.867656673159,-16.5654470829088));
#39787=CARTESIAN_POINT('Ctrl Pts',(-3.91582472241796,10.8805524102322,-16.5572851718075));
#39788=CARTESIAN_POINT('Ctrl Pts',(-3.86606072113723,10.8936232288064,-16.5490126840931));
#39789=CARTESIAN_POINT('Ctrl Pts',(-3.81474963041862,10.9068260275257,-16.5406574901261));
#39790=CARTESIAN_POINT('Ctrl Pts',(-3.71991775466438,10.93122711022,-16.5252156294078));
#39791=CARTESIAN_POINT('Ctrl Pts',(-3.61980126908533,10.9560815366103,-16.5094896077981));
#39792=CARTESIAN_POINT('Ctrl Pts',(-3.51431774214659,10.9810861271972,-16.4936755668265));
#39793=CARTESIAN_POINT('Ctrl Pts',(-3.46379272468944,10.9930629487216,-16.486100879865));
#39794=CARTESIAN_POINT('Ctrl Pts',(-3.412036380583,11.0050735980661,-16.4785064074652));
#39795=CARTESIAN_POINT('Ctrl Pts',(-3.35903983414187,11.0170811856145,-16.4709160458442));
#39796=CARTESIAN_POINT('Ctrl Pts',(-3.24836795982101,11.0421564463494,-16.4550652101997));
#39797=CARTESIAN_POINT('Ctrl Pts',(-3.13228704122553,11.0672213831024,-16.4392303151227));
#39798=CARTESIAN_POINT('Ctrl Pts',(-3.01072545229427,11.0919081379047,-16.4236498311181));
#39799=CARTESIAN_POINT('Ctrl Pts',(-2.96856990008022,11.1004690969233,-16.4182467764793));
#39800=CARTESIAN_POINT('Ctrl Pts',(-2.92501756168561,11.1091302428328,-16.4127824107507));
#39801=CARTESIAN_POINT('Ctrl Pts',(-2.88136956717368,11.1176134042915,-16.4074326091601));
#39802=CARTESIAN_POINT('Ctrl Pts',(-2.87180831191927,11.1194716723054,-16.4062607152589));
#39803=CARTESIAN_POINT('Ctrl Pts',(-2.8622425152675,11.1213215615031,-16.4050942142145));
#39804=CARTESIAN_POINT('Ctrl Pts',(-2.85268593487647,11.1231604237239,-16.4039347765108));
#39805=CARTESIAN_POINT('Ctrl Pts',(-2.83186336209958,11.1271670705424,-16.4014085092711));
#39806=CARTESIAN_POINT('Ctrl Pts',(-2.81108450308508,11.1311212182118,-16.3989158713156));
#39807=CARTESIAN_POINT('Ctrl Pts',(-2.79049215901235,11.134997151391,-16.3964730579524));
#39808=CARTESIAN_POINT('Ctrl Pts',(-2.6196898288082,11.1671459158238,-16.3762112454449));
#39809=CARTESIAN_POINT('Ctrl Pts',(-2.4535496126387,11.1954664439551,-16.3583811544424));
#39810=CARTESIAN_POINT('Ctrl Pts',(-2.29231363557507,11.2203978130869,-16.3427011640703));
#39811=CARTESIAN_POINT('Ctrl Pts',(-2.12996501605265,11.2455012263267,-16.3269129706572));
#39812=CARTESIAN_POINT('Ctrl Pts',(-1.97258856158854,11.2671693869041,-16.3133041243216));
#39813=CARTESIAN_POINT('Ctrl Pts',(-1.82039230653809,11.2858594066231,-16.3015811008586));
#39814=CARTESIAN_POINT('Ctrl Pts',(-1.76982075559219,11.2920696992751,-16.2976857916205));
#39815=CARTESIAN_POINT('Ctrl Pts',(-1.71982072511009,11.297951085905,-16.2939987443829));
#39816=CARTESIAN_POINT('Ctrl Pts',(-1.67039864250388,11.303520032287,-16.2905093604163));
#39817=CARTESIAN_POINT('Ctrl Pts',(-1.52115750354897,11.3203367234704,-16.2799723775543));
#39818=CARTESIAN_POINT('Ctrl Pts',(-1.37719003095167,11.3343061285816,-16.2712367654417));
#39819=CARTESIAN_POINT('Ctrl Pts',(-1.23865184096789,11.3458828933172,-16.2640095546856));
#39820=CARTESIAN_POINT('Ctrl Pts',(-1.14900010082279,11.3533745250753,-16.2593326347637));
#39821=CARTESIAN_POINT('Ctrl Pts',(-1.06162099566594,11.3598637351623,-16.2552876599136));
#39822=CARTESIAN_POINT('Ctrl Pts',(-0.976547038833515,11.3654683087099,
-16.251798534706));
#39823=CARTESIAN_POINT('Ctrl Pts',(-0.844653982939271,11.3741572701701,
-16.2463892249342));
#39824=CARTESIAN_POINT('Ctrl Pts',(-0.718303156836323,11.3807218990101,
-16.2423147910948));
#39825=CARTESIAN_POINT('Ctrl Pts',(-0.597588683233163,11.3855885728515,
-16.2393007710482));
#39826=CARTESIAN_POINT('Ctrl Pts',(-0.480912740331577,11.3902924309913,
-16.2363875857412));
#39827=CARTESIAN_POINT('Ctrl Pts',(-0.369501725349506,11.3934099347066,
-16.234465086433));
#39828=CARTESIAN_POINT('Ctrl Pts',(-0.263411423276765,11.3952953898795,
-16.2333039999994));
#39829=CARTESIAN_POINT('Ctrl Pts',(-0.255777298906237,11.3954310648564,
-16.2332204496837));
#39830=CARTESIAN_POINT('Ctrl Pts',(-0.248170714764654,11.3955603470126,
-16.2331408500901));
#39831=CARTESIAN_POINT('Ctrl Pts',(-0.240591686757623,11.3956833622014,
-16.2330651195921));
#39832=CARTESIAN_POINT('Ctrl Pts',(-0.202104723971215,11.396308044019,-16.2326805535428));
#39833=CARTESIAN_POINT('Ctrl Pts',(-0.164328380149182,11.3967711706233,
-16.2323957255254));
#39834=CARTESIAN_POINT('Ctrl Pts',(-0.127264465149227,11.3970891950709,
-16.2321998280071));
#39835=CARTESIAN_POINT('Ctrl Pts',(-0.105083110171538,11.397279520706,-16.2320825907322));
#39836=CARTESIAN_POINT('Ctrl Pts',(-0.083156921819576,11.3974178649977,
-16.2319972023203));
#39837=CARTESIAN_POINT('Ctrl Pts',(-0.0614862081553471,11.3975076461867,
-16.2319414342152));
#39838=CARTESIAN_POINT('Ctrl Pts',(-0.0416887212949267,11.397589666647,
-16.2318904867317));
#39839=CARTESIAN_POINT('Ctrl Pts',(-0.023099625113114,11.3976306229785,
-16.2318646674111));
#39840=CARTESIAN_POINT('Ctrl Pts',(-0.00299170375185956,11.397634612254,
-16.231861115546));
#39841=CARTESIAN_POINT('Ctrl Pts',(-0.00108910381438552,11.3976349897169,
-16.2318607794706));
#39842=CARTESIAN_POINT('Ctrl Pts',(0.000827093947327497,11.3976350040678,
-16.2318606637935));
#39843=CARTESIAN_POINT('Ctrl Pts',(0.00275919977259721,11.3976346381463,
-16.2318607795923));
#39844=CARTESIAN_POINT('Ctrl Pts',(0.115376740968219,11.3976133095128,-16.2318675292087));
#39845=CARTESIAN_POINT('Ctrl Pts',(0.233548307689586,11.3963110824309,-16.2326602020464));
#39846=CARTESIAN_POINT('Ctrl Pts',(0.357219777273745,11.3933314488223,-16.2344971561809));
#39847=CARTESIAN_POINT('Ctrl Pts',(0.400696756010732,11.3922839520352,-16.2351429414709));
#39848=CARTESIAN_POINT('Ctrl Pts',(0.444853207289354,11.3910288181089,-16.2359179991661));
#39849=CARTESIAN_POINT('Ctrl Pts',(0.489685896103932,11.3895477543126,-16.2368342378403));
#39850=CARTESIAN_POINT('Ctrl Pts',(0.61695135346722,11.3853434947332,-16.2394351421582));
#39851=CARTESIAN_POINT('Ctrl Pts',(0.749668736397475,11.3793207257544,-16.2431724844734));
#39852=CARTESIAN_POINT('Ctrl Pts',(0.887739088610556,11.3710519035528,-16.2483218252168));
#39853=CARTESIAN_POINT('Ctrl Pts',(0.982252494670568,11.3653916402317,-16.2518467074586));
#39854=CARTESIAN_POINT('Ctrl Pts',(1.07927350380205,11.3586782993934,-16.256033599861));
#39855=CARTESIAN_POINT('Ctrl Pts',(1.17875932780541,11.3507671091198,-16.260975385379));
#39856=CARTESIAN_POINT('Ctrl Pts',(1.32354861553918,11.3392533520966,-16.2681675417737));
#39857=CARTESIAN_POINT('Ctrl Pts',(1.47356075193309,11.3252028802458,-16.2769583548483));
#39858=CARTESIAN_POINT('Ctrl Pts',(1.62863385522641,11.3081658687316,-16.2876375935685));
#39859=CARTESIAN_POINT('Ctrl Pts',(1.68658092645764,11.3017995492422,-16.2916281670055));
#39860=CARTESIAN_POINT('Ctrl Pts',(1.74523421223448,11.2950160271918,-16.2958825353738));
#39861=CARTESIAN_POINT('Ctrl Pts',(1.80458351108733,11.2877912174214,-16.3004161770378));
#39862=CARTESIAN_POINT('Ctrl Pts',(1.96231932538665,11.268589453048,-16.3124654796149));
#39863=CARTESIAN_POINT('Ctrl Pts',(2.12497514213533,11.2462709846675,-16.3264872932238));
#39864=CARTESIAN_POINT('Ctrl Pts',(2.29233589177227,11.2203922801793,-16.3427662443591));
#39865=CARTESIAN_POINT('Ctrl Pts',(2.31271087216276,11.2172417320513,-16.3447480908247));
#39866=CARTESIAN_POINT('Ctrl Pts',(2.33315552275998,11.2140384090245,-16.3467633944773));
#39867=CARTESIAN_POINT('Ctrl Pts',(2.35366940187776,11.2107815052252,-16.3488126712752));
#39868=CARTESIAN_POINT('Ctrl Pts',(2.36244348092684,11.2093884809598,-16.3496891762265));
#39869=CARTESIAN_POINT('Ctrl Pts',(2.37123022445249,11.2079856546398,-16.3505718962139));
#39870=CARTESIAN_POINT('Ctrl Pts',(2.38002959914226,11.2065729651554,-16.3514608704435));
#39871=CARTESIAN_POINT('Ctrl Pts',(2.44796695689478,11.1956660093453,-16.3583243763625));
#39872=CARTESIAN_POINT('Ctrl Pts',(2.51665736075251,11.1841711117674,-16.365560699008));
#39873=CARTESIAN_POINT('Ctrl Pts',(2.58608470263645,11.172060185812,-16.3731878432196));
#39874=CARTESIAN_POINT('Ctrl Pts',(2.62079837357841,11.1660047228343,-16.3770014153254));
#39875=CARTESIAN_POINT('Ctrl Pts',(2.65569627858871,11.1597952502236,-16.3809126927319));
#39876=CARTESIAN_POINT('Ctrl Pts',(2.69077624810768,11.1534282705164,-16.3849239162302));
#39877=CARTESIAN_POINT('Ctrl Pts',(2.70831623286716,11.1502447806628,-16.3869295279793));
#39878=CARTESIAN_POINT('Ctrl Pts',(2.72590173373479,11.1470219139176,-16.3889601262475));
#39879=CARTESIAN_POINT('Ctrl Pts',(2.7435324742445,11.1437592333271,-16.3910159905811));
#39880=CARTESIAN_POINT('Ctrl Pts',(2.75885712424319,11.1409233094429,-16.3928029490664));
#39881=CARTESIAN_POINT('Ctrl Pts',(2.77563471566203,11.1377908818067,-16.3947768843287));
#39882=CARTESIAN_POINT('Ctrl Pts',(2.79016543957015,11.1350561816445,-16.3965003301687));
#39883=CARTESIAN_POINT('Ctrl Pts',(2.79235205815691,11.1346446573295,-16.39675967848));
#39884=CARTESIAN_POINT('Ctrl Pts',(2.79448781861613,11.1342422193846,-16.3970133028468));
#39885=CARTESIAN_POINT('Ctrl Pts',(2.79656013539408,11.1338513131024,-16.3972596610821));
#39886=CARTESIAN_POINT('Ctrl Pts',(2.81155090954738,11.1310235659868,-16.3990417731148));
#39887=CARTESIAN_POINT('Ctrl Pts',(2.82653561969514,11.1281742204883,-16.4008378183665));
#39888=CARTESIAN_POINT('Ctrl Pts',(2.84151418411467,11.1253033432094,-16.402647751769));
#39889=CARTESIAN_POINT('Ctrl Pts',(2.98776286620042,11.0972724847966,-16.4203196973143));
#39890=CARTESIAN_POINT('Ctrl Pts',(3.13342565900406,11.067188944468,-16.4393156419953));
#39891=CARTESIAN_POINT('Ctrl Pts',(3.27843552237667,11.0351214013139,-16.4595893383465));
#39892=CARTESIAN_POINT('Ctrl Pts',(3.40982472733808,11.0060659363815,-16.4779587429046));
#39893=CARTESIAN_POINT('Ctrl Pts',(3.5406779002364,10.9753816751959,-16.4973771362034));
#39894=CARTESIAN_POINT('Ctrl Pts',(3.67095144391563,10.943123139663,-16.5178077455709));
#39895=CARTESIAN_POINT('Ctrl Pts',(3.78812567273624,10.9141082766509,-16.5361840085432));
#39896=CARTESIAN_POINT('Ctrl Pts',(3.90483097783149,10.8838198162215,-16.5553791605345));
#39897=CARTESIAN_POINT('Ctrl Pts',(4.02103992397148,10.8522990627777,-16.5753651336091));
#39898=CARTESIAN_POINT('Ctrl Pts',(4.12468261995777,10.8241868048582,-16.5931899242141));
#39899=CARTESIAN_POINT('Ctrl Pts',(4.22793050029308,10.7950943527066,-16.6116437523539));
#39900=CARTESIAN_POINT('Ctrl Pts',(4.33076689523681,10.7650516875563,-16.6307059990957));
#39901=CARTESIAN_POINT('Ctrl Pts',(4.42239699687154,10.7382828333719,-16.6476909936328));
#39902=CARTESIAN_POINT('Ctrl Pts',(4.51370040736879,10.7107595762264,-16.6651590304519));
#39903=CARTESIAN_POINT('Ctrl Pts',(4.60466714131258,10.6825033517688,-16.6830951531163));
#39904=CARTESIAN_POINT('Ctrl Pts',(4.68608821708453,10.6572122140875,-16.6991491361406));
#39905=CARTESIAN_POINT('Ctrl Pts',(4.76723956751118,10.6313338673615,-16.7155781214801));
#39906=CARTESIAN_POINT('Ctrl Pts',(4.84811525533268,10.6048836944837,-16.7323712567022));
#39907=CARTESIAN_POINT('Ctrl Pts',(4.92103851396308,10.5810343418595,-16.7475131389664));
#39908=CARTESIAN_POINT('Ctrl Pts',(4.99373765565988,10.5567200890228,-16.7629510788517));
#39909=CARTESIAN_POINT('Ctrl Pts',(5.06620920273585,10.5319521148902,-16.7786772584776));
#39910=CARTESIAN_POINT('Ctrl Pts',(5.13210920773643,10.5094300398822,-16.7929774267202));
#39911=CARTESIAN_POINT('Ctrl Pts',(5.19782102170716,10.4865327979589,-16.8075159308807));
#39912=CARTESIAN_POINT('Ctrl Pts',(5.26334266567217,10.4632686283996,-16.8222874368434));
#39913=CARTESIAN_POINT('Ctrl Pts',(5.32292443051119,10.4421134772773,-16.8357198286658));
#39914=CARTESIAN_POINT('Ctrl Pts',(5.38234894166926,10.4206549108743,-16.8493448913841));
#39915=CARTESIAN_POINT('Ctrl Pts',(5.44161508240666,10.3988989162237,-16.8631598859357));
#39916=CARTESIAN_POINT('Ctrl Pts',(5.49538235744157,10.3791614989821,-16.87569308959));
#39917=CARTESIAN_POINT('Ctrl Pts',(5.54901928600415,10.359179284877,-16.8883826152172));
#39918=CARTESIAN_POINT('Ctrl Pts',(5.60252500722285,10.3389565104295,-16.9012289578158));
#39919=CARTESIAN_POINT('Ctrl Pts',(5.6472564469046,10.3220500227719,-16.9119686579076));
#39920=CARTESIAN_POINT('Ctrl Pts',(5.69189618355805,10.3049754018566,-16.9228179599782));
#39921=CARTESIAN_POINT('Ctrl Pts',(5.73644276371256,10.2877350949212,-16.9337809951185));
#39922=CARTESIAN_POINT('Ctrl Pts',(-5.843530256063,10.2251612018568,-17.1593147457631));
#39923=CARTESIAN_POINT('Ctrl Pts',(-3.895686837375,11.0033631167315,-16.6619433466125));
#39924=CARTESIAN_POINT('Ctrl Pts',(0.0001633689297129,11.7816837051417,
-16.1645459237592));
#39925=CARTESIAN_POINT('Ctrl Pts',(3.896013575235,11.0032978376656,-16.6619850641797));
#39926=CARTESIAN_POINT('Ctrl Pts',(5.844020362852,10.2249653863089,-17.1594398971657));
#39927=CARTESIAN_POINT('Ctrl Pts',(-5.843530256063,10.3258757938396,-16.2770692610481));
#39928=CARTESIAN_POINT('Ctrl Pts',(-3.895686837375,11.0553896787781,-15.8346873902757));
#39929=CARTESIAN_POINT('Ctrl Pts',(0.0001633689297129,11.7876693634894,
-15.3921230864179));
#39930=CARTESIAN_POINT('Ctrl Pts',(3.896013575235,11.0553282612408,-15.8347245088966));
#39931=CARTESIAN_POINT('Ctrl Pts',(5.844020362852,10.3256922294701,-16.2771805756635));
#39932=CARTESIAN_POINT('Ctrl Pts',(-5.843530256063,10.2973084286348,-14.4766645869159));
#39933=CARTESIAN_POINT('Ctrl Pts',(-3.895686837375,10.9728038432035,-14.1582375728196));
#39934=CARTESIAN_POINT('Ctrl Pts',(0.0001633689297129,11.6469744444563,
-13.8399446100658));
#39935=CARTESIAN_POINT('Ctrl Pts',(3.896013575235,10.9727472993719,-14.1582642685905));
#39936=CARTESIAN_POINT('Ctrl Pts',(5.844020362852,10.2971384566574,-14.4767447113191));
#39937=CARTESIAN_POINT('Ctrl Pts',(-5.843530256063,9.5578304148104,-11.8732201296631));
#39938=CARTESIAN_POINT('Ctrl Pts',(-3.895686837375,10.2763900787824,-11.7328262507199));
#39939=CARTESIAN_POINT('Ctrl Pts',(0.0001633689297128,10.9955719605871,
-11.5921562078845));
#39940=CARTESIAN_POINT('Ctrl Pts',(3.896013575235,10.276329759774,-11.7328380489468));
#39941=CARTESIAN_POINT('Ctrl Pts',(5.844020362852,9.55764960678671,-11.8732554563657));
#39942=CARTESIAN_POINT('Ctrl Pts',(-5.843530256063,8.22106676100552,-9.63752328128312));
#39943=CARTESIAN_POINT('Ctrl Pts',(-3.895686837375,9.09189067503903,-9.61305770160358));
#39944=CARTESIAN_POINT('Ctrl Pts',(0.0001633689297132,9.96180813993581,
-9.58947419762877));
#39945=CARTESIAN_POINT('Ctrl Pts',(3.896013575235,9.09181771358517,-9.61305967959051));
#39946=CARTESIAN_POINT('Ctrl Pts',(5.844020362852,8.22084763937311,-9.63752943746074));
#39947=CARTESIAN_POINT('Ctrl Pts',(-5.843530256063,7.02207811294743,-8.43809751774869));
#39948=CARTESIAN_POINT('Ctrl Pts',(-3.895686837375,8.04135302927588,-8.43217964834793));
#39949=CARTESIAN_POINT('Ctrl Pts',(0.0001633689297125,9.06228035038236,
-8.42461129239938));
#39950=CARTESIAN_POINT('Ctrl Pts',(3.896013575235,8.04126740236864,-8.43218028311409));
#39951=CARTESIAN_POINT('Ctrl Pts',(5.844020362852,7.0218216372639,-8.4380990068179));
#39952=CARTESIAN_POINT('Ctrl Pts',(-5.843530256063,6.40544655073385,-7.9486149548088));
#39953=CARTESIAN_POINT('Ctrl Pts',(-3.895686837375,7.5011200872024,-7.93456153010133));
#39954=CARTESIAN_POINT('Ctrl Pts',(0.0001633689297125,8.59741267407606,
-7.91992172805397));
#39955=CARTESIAN_POINT('Ctrl Pts',(3.896013575235,7.50102813928303,-7.93456275796333));
#39956=CARTESIAN_POINT('Ctrl Pts',(5.844020362852,6.40517085118626,-7.94861849100275));
#39957=CARTESIAN_POINT('',(-5.73278772553971,6.65588342589818,-8.10254678308617));
#39958=CARTESIAN_POINT('Ctrl Pts',(-5.73644356954166,10.2877321244828,-16.9337807348495));
#39959=CARTESIAN_POINT('Ctrl Pts',(-5.73766037024604,10.3633357381801,-16.1063574319785));
#39960=CARTESIAN_POINT('Ctrl Pts',(-5.73849618482932,10.3386824461305,-15.2703428362758));
#39961=CARTESIAN_POINT('Ctrl Pts',(-5.73940756701684,10.0903333007246,-13.6301040101181));
#39962=CARTESIAN_POINT('Ctrl Pts',(-5.73948313455368,9.86673834048807,-12.8258709788125));
#39963=CARTESIAN_POINT('Ctrl Pts',(-5.7388740224731,9.23545640664265,-11.2957057307492));
#39964=CARTESIAN_POINT('Ctrl Pts',(-5.73818934285567,8.82745509879148,-10.5699144590352));
#39965=CARTESIAN_POINT('Ctrl Pts',(-5.73605973646658,7.85267849992233,-9.23785246261833));
#39966=CARTESIAN_POINT('Ctrl Pts',(-5.7346148096949,7.28539108565082,-8.63201128890514));
#39967=CARTESIAN_POINT('Ctrl Pts',(-5.73278797082,6.65588387270908,-8.10254625058942));
#39968=CARTESIAN_POINT('Ctrl Pts',(5.73278688057609,6.65588777859083,-8.10254157115373));
#39969=CARTESIAN_POINT('Ctrl Pts',(5.37901145696501,6.85200131459071,-8.10465302967502));
#39970=CARTESIAN_POINT('Ctrl Pts',(5.01621448638398,7.03118682771357,-8.10373337999374));
#39971=CARTESIAN_POINT('Ctrl Pts',(4.64600910147529,7.19213776342579,-8.10100488069798));
#39972=CARTESIAN_POINT('Ctrl Pts',(4.37165673834806,7.31141552479892,-8.09898284033849));
#39973=CARTESIAN_POINT('Ctrl Pts',(4.09323566077892,7.42067530523888,-8.09596915441615));
#39974=CARTESIAN_POINT('Ctrl Pts',(3.81140241906258,7.51940929188303,-8.09247479094618));
#39975=CARTESIAN_POINT('Ctrl Pts',(3.57236173411404,7.60315186125273,-8.08951099919389));
#39976=CARTESIAN_POINT('Ctrl Pts',(3.33086640167441,7.67932161809156,-8.08620166972316));
#39977=CARTESIAN_POINT('Ctrl Pts',(3.08731701794449,7.74764923593218,-8.08286091596895));
#39978=CARTESIAN_POINT('Ctrl Pts',(3.04371732347713,7.7598811012562,-8.08226286131267));
#39979=CARTESIAN_POINT('Ctrl Pts',(3.00005180200329,7.7718617807475,-8.08166380201583));
#39980=CARTESIAN_POINT('Ctrl Pts',(2.95632275176659,7.78358991883312,-8.08106554250556));
#39981=CARTESIAN_POINT('Ctrl Pts',(2.75787639428296,7.83681326282433,-8.07835058711549));
#39982=CARTESIAN_POINT('Ctrl Pts',(2.55811712333055,7.88487916025936,-8.07569724649496));
#39983=CARTESIAN_POINT('Ctrl Pts',(2.35731173231339,7.92759052582829,-8.0731958413278));
#39984=CARTESIAN_POINT('Ctrl Pts',(2.16334914198626,7.96884642568334,-8.07077967598871));
#39985=CARTESIAN_POINT('Ctrl Pts',(1.96841051361373,8.00510644711771,-8.06850527824001));
#39986=CARTESIAN_POINT('Ctrl Pts',(1.77273628508688,8.03624111800075,-8.06645356836242));
#39987=CARTESIAN_POINT('Ctrl Pts',(1.58015286697596,8.06688399512134,-8.06443426666811));
#39988=CARTESIAN_POINT('Ctrl Pts',(1.38685690380679,8.09256199738575,-8.06263068304187));
#39989=CARTESIAN_POINT('Ctrl Pts',(1.19307761884276,8.11320098306076,-8.06111934189182));
#39990=CARTESIAN_POINT('Ctrl Pts',(0.994919648475874,8.13430633244087,-8.05957385009748));
#39991=CARTESIAN_POINT('Ctrl Pts',(0.796256267013193,8.15014186612969,-8.05833397011766));
#39992=CARTESIAN_POINT('Ctrl Pts',(0.597332590239811,8.16068573962992,-8.05748069792611));
#39993=CARTESIAN_POINT('Ctrl Pts',(0.40855170583876,8.1706919982949,-8.05667093268564));
#39994=CARTESIAN_POINT('Ctrl Pts',(0.219536393470747,8.17593270670312,-8.05620935321766));
#39995=CARTESIAN_POINT('Ctrl Pts',(0.0304961540370044,8.17644103763726,
-8.05616438298739));
#39996=CARTESIAN_POINT('Ctrl Pts',(0.0203394270745499,8.17646834916902,
-8.05616196683329));
#39997=CARTESIAN_POINT('Ctrl Pts',(0.0101826281555681,8.17648201238107,
-8.05616075310184));
#39998=CARTESIAN_POINT('Ctrl Pts',(2.57897726576351E-5,8.17648203672123,
-8.05616075233821));
#39999=CARTESIAN_POINT('Ctrl Pts',(1.71931816709343E-5,8.17648203674183,
-8.05616075233757));
#40000=CARTESIAN_POINT('Ctrl Pts',(8.59659071081628E-6,8.17648203675266,
-8.05616075233779));
#40001=CARTESIAN_POINT('Ctrl Pts',(-2.20960885290795E-13,8.17648203675372,
-8.05616075233888));
#40002=CARTESIAN_POINT('Ctrl Pts',(-0.189394108313583,8.17648206011399,
-8.05616077638705));
#40003=CARTESIAN_POINT('Ctrl Pts',(-0.378774674464551,8.17173533196982,
-8.05658262828894));
#40004=CARTESIAN_POINT('Ctrl Pts',(-0.567931019578452,8.1622056991069,-8.05735754707092));
#40005=CARTESIAN_POINT('Ctrl Pts',(-0.769333664674303,8.15205910178166,
-8.05818263539842));
#40006=CARTESIAN_POINT('Ctrl Pts',(-0.970482116019627,8.13648985922757,
-8.05940799112298));
#40007=CARTESIAN_POINT('Ctrl Pts',(-1.17112206928258,8.11551790495007,-8.06094962786347));
#40008=CARTESIAN_POINT('Ctrl Pts',(-1.36692420168941,8.09505162542053,-8.06245409273338));
#40009=CARTESIAN_POINT('Ctrl Pts',(-1.56224206214246,8.0694405548821,-8.0642597569665));
#40010=CARTESIAN_POINT('Ctrl Pts',(-1.75683930164901,8.03875939082742,-8.06628774535347));
#40011=CARTESIAN_POINT('Ctrl Pts',(-1.95864861723658,8.00694113515736,-8.06839089414134));
#40012=CARTESIAN_POINT('Ctrl Pts',(-2.15968290739831,7.96967000868949,-8.07073314300512));
#40013=CARTESIAN_POINT('Ctrl Pts',(-2.35967855880933,7.92708729785437,-8.07322578424444));
#40014=CARTESIAN_POINT('Ctrl Pts',(-2.55967421022036,7.88450458701924,-8.07571842548375));
#40015=CARTESIAN_POINT('Ctrl Pts',(-2.75863122288067,7.83661067021283,-8.07836144421808));
#40016=CARTESIAN_POINT('Ctrl Pts',(-2.95628598346539,7.78360035556706,-8.08106560032508));
#40017=CARTESIAN_POINT('Ctrl Pts',(-3.19878486586875,7.71856300448368,-8.0843832782391));
#40018=CARTESIAN_POINT('Ctrl Pts',(-3.43933039900217,7.64575489262882,-8.0877255164212));
#40019=CARTESIAN_POINT('Ctrl Pts',(-3.6775306242641,7.56543015431638,-8.09078481904143));
#40020=CARTESIAN_POINT('Ctrl Pts',(-3.96235759097273,7.46938216972677,-8.09444296791431));
#40021=CARTESIAN_POINT('Ctrl Pts',(-4.24383121655615,7.36258759907886,-8.09769624835467));
#40022=CARTESIAN_POINT('Ctrl Pts',(-4.52128137417785,7.24555633741688,-8.10002218723693));
#40023=CARTESIAN_POINT('Ctrl Pts',(-4.88829810139467,7.09074499758769,-8.1030989866289));
#40024=CARTESIAN_POINT('Ctrl Pts',(-5.24827434791527,6.91802662505855,-8.10455035959127));
#40025=CARTESIAN_POINT('Ctrl Pts',(-5.59965894280897,6.72865801645831,-8.10319481985575));
#40026=CARTESIAN_POINT('Ctrl Pts',(-5.64417482545532,6.70466746342937,-8.10302309050658));
#40027=CARTESIAN_POINT('Ctrl Pts',(-5.68855281542513,6.68040966675613,-8.10280638090245));
#40028=CARTESIAN_POINT('Ctrl Pts',(-5.7327897587563,6.65588714131628,-8.10254235865644));
#40029=CARTESIAN_POINT('Ctrl Pts',(5.8442109276592,6.60975781659273,-8.11489313945908));
#40030=CARTESIAN_POINT('Ctrl Pts',(5.39516759795808,6.86923202515899,-8.12241643595089));
#40031=CARTESIAN_POINT('Ctrl Pts',(4.36936999562943,7.380526520853,-8.12655400963949));
#40032=CARTESIAN_POINT('Ctrl Pts',(2.70735887873967,7.93435136477757,-8.10987588460702));
#40033=CARTESIAN_POINT('Ctrl Pts',(0.904594091570436,8.22878805472967,-8.09288686312857));
#40034=CARTESIAN_POINT('Ctrl Pts',(-0.901198823780471,8.22906308886219,
-8.09286831827879));
#40035=CARTESIAN_POINT('Ctrl Pts',(-2.70398663593974,7.93518345288968,-8.1098357600967));
#40036=CARTESIAN_POINT('Ctrl Pts',(-4.36726502917644,7.38148399620803,-8.12654684250591));
#40037=CARTESIAN_POINT('Ctrl Pts',(-5.39421917802381,6.8697862795005,-8.12243344312352));
#40038=CARTESIAN_POINT('Ctrl Pts',(-5.84432678346674,6.60969083810708,-8.11489124898177));
#40039=CARTESIAN_POINT('Ctrl Pts',(5.72537981142124,6.40696257187108,-7.90741414418503));
#40040=CARTESIAN_POINT('Ctrl Pts',(5.28537605413658,6.66000489116012,-7.91604649446402));
#40041=CARTESIAN_POINT('Ctrl Pts',(4.28025648075084,7.15876699709817,-7.92256998014448));
#40042=CARTESIAN_POINT('Ctrl Pts',(2.6519626539299,7.69915973752875,-7.90889401748803));
#40043=CARTESIAN_POINT('Ctrl Pts',(0.886045026031056,7.98647110079696,-7.89367199191233));
#40044=CARTESIAN_POINT('Ctrl Pts',(-0.882719338489682,7.98673947796939,
-7.89365515637576));
#40045=CARTESIAN_POINT('Ctrl Pts',(-2.64865910398843,7.69997168607342,-7.90885871599316));
#40046=CARTESIAN_POINT('Ctrl Pts',(-4.27819398429727,7.15970115468978,-7.92256756530623));
#40047=CARTESIAN_POINT('Ctrl Pts',(-5.28444672405522,6.66054540297074,-7.9160658522132));
#40048=CARTESIAN_POINT('Ctrl Pts',(-5.72549333439,6.4068972576017,-7.90741196554548));
#40049=CARTESIAN_POINT('Ctrl Pts',(5.71943373791309,6.40363111006797,-7.59396822918313));
#40050=CARTESIAN_POINT('Ctrl Pts',(5.28070658173558,6.65404878042135,-7.60260325901111));
#40051=CARTESIAN_POINT('Ctrl Pts',(4.27825102124085,7.14800517646924,-7.6092187454652));
#40052=CARTESIAN_POINT('Ctrl Pts',(2.6523390834295,7.68419247725851,-7.59572769065918));
#40053=CARTESIAN_POINT('Ctrl Pts',(0.886530195119529,7.96977217997496,-7.58059743549267));
#40054=CARTESIAN_POINT('Ctrl Pts',(-0.8832030571043,7.97003912961983,-7.58058067281829));
#40055=CARTESIAN_POINT('Ctrl Pts',(-2.64903784070115,7.68499899712703,-7.59569267513307));
#40056=CARTESIAN_POINT('Ctrl Pts',(-4.27619364792927,7.14893090541477,-7.60921659325103));
#40057=CARTESIAN_POINT('Ctrl Pts',(-5.27977997084161,6.6545836524422,-7.60262263134438));
#40058=CARTESIAN_POINT('Ctrl Pts',(-5.71954693670857,6.40356646873755,-7.59396605610153));
#40059=CARTESIAN_POINT('Ctrl Pts',(5.83023063406281,6.60192618672222,-7.3778700458245));
#40060=CARTESIAN_POINT('Ctrl Pts',(5.38418897415298,6.85522895262948,-7.38539963283444));
#40061=CARTESIAN_POINT('Ctrl Pts',(4.3646552438395,7.35522359613006,-7.38975351198828));
#40062=CARTESIAN_POINT('Ctrl Pts',(2.70824450483877,7.89916004901893,-7.37351014503725));
#40063=CARTESIAN_POINT('Ctrl Pts',(0.905735068707309,8.18952504203874,-7.35673689298432));
#40064=CARTESIAN_POINT('Ctrl Pts',(-0.902336389694713,8.18979671959776,
-7.35671851944764));
#40065=CARTESIAN_POINT('Ctrl Pts',(-2.70487768650738,7.8999793725258,-7.37347069289444));
#40066=CARTESIAN_POINT('Ctrl Pts',(-4.36256232336407,7.35616125289302,-7.38974696233364));
#40067=CARTESIAN_POINT('Ctrl Pts',(-5.38324694783943,6.85576994589504,-7.38541667426304));
#40068=CARTESIAN_POINT('Ctrl Pts',(-5.83034572764334,6.60186079054662,-7.3778681684244));
#40069=CARTESIAN_POINT('',(-5.72001815070041,6.64700889995603,-7.39409229753282));
#40070=CARTESIAN_POINT('Origin',(-5.89877671949853,6.95919955112704,-7.74135717571565));
#40071=CARTESIAN_POINT('Ctrl Pts',(5.72001488685505,6.64700976236097,-7.39409060170019));
#40072=CARTESIAN_POINT('Ctrl Pts',(5.54310206102047,6.74533606056453,-7.39676017670215));
#40073=CARTESIAN_POINT('Ctrl Pts',(5.36158785252199,6.84067954195826,-7.39860465582333));
#40074=CARTESIAN_POINT('Ctrl Pts',(5.1754616574481,6.93251781017533,-7.39975339332922));
#40075=CARTESIAN_POINT('Ctrl Pts',(4.99269419995749,7.02269881224069,-7.40088140130893));
#40076=CARTESIAN_POINT('Ctrl Pts',(4.80547960727636,7.10949997762252,-7.40133851378473));
#40077=CARTESIAN_POINT('Ctrl Pts',(4.6138337175032,7.19238904742863,-7.40126841792195));
#40078=CARTESIAN_POINT('Ctrl Pts',(4.55683580273732,7.21704130655834,-7.40124757052461));
#40079=CARTESIAN_POINT('Ctrl Pts',(4.49944610286399,7.24134726660044,-7.40118023619262));
#40080=CARTESIAN_POINT('Ctrl Pts',(4.44166550877915,7.26529226398299,-7.40107057479409));
#40081=CARTESIAN_POINT('Ctrl Pts',(4.42850790010658,7.27074494078937,-7.40104560305762));
#40082=CARTESIAN_POINT('Ctrl Pts',(4.41533002256282,7.27617889864318,-7.40101843718722));
#40083=CARTESIAN_POINT('Ctrl Pts',(4.40213190278768,7.28159396299967,-7.40098912934694));
#40084=CARTESIAN_POINT('Ctrl Pts',(4.21117034315222,7.35994369407183,-7.40056507872579));
#40085=CARTESIAN_POINT('Ctrl Pts',(4.01596862780368,7.43435233647871,-7.39968081201011));
#40086=CARTESIAN_POINT('Ctrl Pts',(3.8165986469795,7.50434439156106,-7.39843718528071));
#40087=CARTESIAN_POINT('Ctrl Pts',(3.77349781704224,7.51947563474317,-7.39816833164514));
#40088=CARTESIAN_POINT('Ctrl Pts',(3.73020224843773,7.53440030208692,-7.3978827611826));
#40089=CARTESIAN_POINT('Ctrl Pts',(3.68671278435282,7.54911331686161,-7.39758162520437));
#40090=CARTESIAN_POINT('Ctrl Pts',(3.56438421629974,7.59049855963255,-7.39673458020663));
#40091=CARTESIAN_POINT('Ctrl Pts',(3.44052193650649,7.63021118821232,-7.39576239974459));
#40092=CARTESIAN_POINT('Ctrl Pts',(3.31515060744115,7.66814403300511,-7.39468104272607));
#40093=CARTESIAN_POINT('Ctrl Pts',(3.25246494290849,7.68711045540151,-7.39414036421681));
#40094=CARTESIAN_POINT('Ctrl Pts',(3.18940201028333,7.70563191107659,-7.39357237190721));
#40095=CARTESIAN_POINT('Ctrl Pts',(3.1259655539031,7.72369515016552,-7.3929784612098));
#40096=CARTESIAN_POINT('Ctrl Pts',(3.09424732571298,7.73272676970999,-7.3926815058611));
#40097=CARTESIAN_POINT('Ctrl Pts',(3.06243571634816,7.74164383392144,-7.3923780698253));
#40098=CARTESIAN_POINT('Ctrl Pts',(3.03053121358297,7.75044469037029,-7.3920683036439));
#40099=CARTESIAN_POINT('Ctrl Pts',(3.01457896220038,7.75484511859471,-7.3919134205532));
#40100=CARTESIAN_POINT('Ctrl Pts',(2.99860348745703,7.75921649480437,-7.39175695485891));
#40101=CARTESIAN_POINT('Ctrl Pts',(2.98260485279153,7.76355861313257,-7.39159892310988));
#40102=CARTESIAN_POINT('Ctrl Pts',(2.96757448754333,7.76763793776173,-7.39145045575887));
#40103=CARTESIAN_POINT('Ctrl Pts',(2.9513816149432,7.77199691858728,-7.39128914173787));
#40104=CARTESIAN_POINT('Ctrl Pts',(2.93724511216979,7.77577436204495,-7.39114730518404));
#40105=CARTESIAN_POINT('Ctrl Pts',(2.93633442616335,7.77601770829204,-7.39113816794785));
#40106=CARTESIAN_POINT('Ctrl Pts',(2.93543227902122,7.77625865832359,-7.39112911177721));
#40107=CARTESIAN_POINT('Ctrl Pts',(2.93453953320978,7.77649698869763,-7.39112014540118));
#40108=CARTESIAN_POINT('Ctrl Pts',(2.84807339415212,7.79958027511503,-7.39025171464965));
#40109=CARTESIAN_POINT('Ctrl Pts',(2.76126214800757,7.8216862190474,-7.38937821303356));
#40110=CARTESIAN_POINT('Ctrl Pts',(2.67411779411,7.84279743750039,-7.38851198570502));
#40111=CARTESIAN_POINT('Ctrl Pts',(2.42339777807464,7.90353579623881,-7.38601979292385));
#40112=CARTESIAN_POINT('Ctrl Pts',(2.16992012160589,7.95604400160564,-7.38358730623505));
#40113=CARTESIAN_POINT('Ctrl Pts',(1.91409726142779,7.99999663393151,-7.38140756716427));
#40114=CARTESIAN_POINT('Ctrl Pts',(1.66581451969773,8.042653807151,-7.37929207368423));
#40115=CARTESIAN_POINT('Ctrl Pts',(1.41532240940271,8.07725234402325,-7.37741450777488));
#40116=CARTESIAN_POINT('Ctrl Pts',(1.16300478372367,8.10344682314147,-7.37595930986092));
#40117=CARTESIAN_POINT('Ctrl Pts',(1.07270633115421,8.11282120166089,-7.37543852927947));
#40118=CARTESIAN_POINT('Ctrl Pts',(0.982174166778356,8.12111876850057,-7.37497192963931));
#40119=CARTESIAN_POINT('Ctrl Pts',(0.891426247545732,8.1283221166188,-7.37456827777986));
#40120=CARTESIAN_POINT('Ctrl Pts',(0.634296538441118,8.14873244472201,-7.37342455034148));
#40121=CARTESIAN_POINT('Ctrl Pts',(0.37543293836073,8.16036115306758,-7.37278610170794));
#40122=CARTESIAN_POINT('Ctrl Pts',(0.115324552487338,8.16301820257557,-7.37263966809104));
#40123=CARTESIAN_POINT('Ctrl Pts',(0.0769167899751985,8.16341054412251,
-7.37261804561407));
#40124=CARTESIAN_POINT('Ctrl Pts',(0.0384819294165527,8.16360718853533,
-7.37260715563853));
#40125=CARTESIAN_POINT('Ctrl Pts',(2.15925475930276E-5,8.16360743803404,
-7.37260696056192));
#40126=CARTESIAN_POINT('Ctrl Pts',(-0.258129994921792,8.16360911270702,
-7.3726056511783));
#40127=CARTESIAN_POINT('Ctrl Pts',(-0.515109037614368,8.15480586118552,
-7.37304260681286));
#40128=CARTESIAN_POINT('Ctrl Pts',(-0.770460315820714,8.13735601892008,
-7.37396937370198));
#40129=CARTESIAN_POINT('Ctrl Pts',(-0.809708757097711,8.13467391325662,
-7.37411182122009));
#40130=CARTESIAN_POINT('Ctrl Pts',(-0.848918766915221,8.13178743638375,
-7.37426584593983));
#40131=CARTESIAN_POINT('Ctrl Pts',(-0.888088715740413,8.12869705861704,
-7.37443164063193));
#40132=CARTESIAN_POINT('Ctrl Pts',(-1.08981987124167,8.11278114612515,-7.3752855083498));
#40133=CARTESIAN_POINT('Ctrl Pts',(-1.29048836738904,8.09145876435622,-7.3764512185077));
#40134=CARTESIAN_POINT('Ctrl Pts',(-1.48990484646398,8.06489626046362,-7.37785293389087));
#40135=CARTESIAN_POINT('Ctrl Pts',(-1.73493161452673,8.03225841372874,-7.37957524787252));
#40136=CARTESIAN_POINT('Ctrl Pts',(-1.97805598588168,7.9916870343962,-7.38168071551812));
#40137=CARTESIAN_POINT('Ctrl Pts',(-2.21892777462716,7.94350514881498,-7.3839752327673));
#40138=CARTESIAN_POINT('Ctrl Pts',(-2.33936366899991,7.91941420602437,-7.38512249139189));
#40139=CARTESIAN_POINT('Ctrl Pts',(-2.45923687164102,7.89342169547882,-7.38631515545542));
#40140=CARTESIAN_POINT('Ctrl Pts',(-2.57850627791965,7.86557417008048,-7.38751823647971));
#40141=CARTESIAN_POINT('Ctrl Pts',(-2.60930159135434,7.8583839500586,-7.3878288715234));
#40142=CARTESIAN_POINT('Ctrl Pts',(-2.64005670289387,7.85107009617181,-7.38814014048465));
#40143=CARTESIAN_POINT('Ctrl Pts',(-2.67077082458501,7.84363339425458,-7.38845145415508));
#40144=CARTESIAN_POINT('Ctrl Pts',(-2.69953417933264,7.83666902465455,-7.38874299514819));
#40145=CARTESIAN_POINT('Ctrl Pts',(-2.72826158585112,7.82959691648446,-7.38903457532465));
#40146=CARTESIAN_POINT('Ctrl Pts',(-2.75695259273191,7.82241789298791,-7.38932555207471));
#40147=CARTESIAN_POINT('Ctrl Pts',(-2.78661652972273,7.81499542428396,-7.38962639602959));
#40148=CARTESIAN_POINT('Ctrl Pts',(-2.81624150333557,7.80745862641934,-7.38992665046021));
#40149=CARTESIAN_POINT('Ctrl Pts',(-2.8458269132347,7.79980834038875,-7.39022570062281));
#40150=CARTESIAN_POINT('Ctrl Pts',(-2.86061961818427,7.79598319737345,-7.3903752257041));
#40151=CARTESIAN_POINT('Ctrl Pts',(-2.87540243220805,7.79212968229107,-7.39052444969649));
#40152=CARTESIAN_POINT('Ctrl Pts',(-2.89017528111123,7.7882479020018,-7.39067329341478));
#40153=CARTESIAN_POINT('Ctrl Pts',(-2.90420328195651,7.78456184134173,-7.39081463242254));
#40154=CARTESIAN_POINT('Ctrl Pts',(-2.91705775282148,7.78116066606872,-7.39094394101347));
#40155=CARTESIAN_POINT('Ctrl Pts',(-2.93205612393056,7.77716033250627,-7.39109444591867));
#40156=CARTESIAN_POINT('Ctrl Pts',(-2.93285249596642,7.7769479258549,-7.391102437313));
#40157=CARTESIAN_POINT('Ctrl Pts',(-2.93365490901664,7.77673381813008,-7.39111048831088));
#40158=CARTESIAN_POINT('Ctrl Pts',(-2.93446385852311,7.77651787282764,-7.39111860382889));
#40159=CARTESIAN_POINT('Ctrl Pts',(-3.14099738938505,7.72138470885261,-7.39319058307616));
#40160=CARTESIAN_POINT('Ctrl Pts',(-3.34369757065512,7.66128569454362,-7.39509711240524));
#40161=CARTESIAN_POINT('Ctrl Pts',(-3.54245550567647,7.59674786722476,-7.3966933083795));
#40162=CARTESIAN_POINT('Ctrl Pts',(-3.74549187236312,7.53082080891001,-7.39832386381418));
#40163=CARTESIAN_POINT('Ctrl Pts',(-3.94441448021563,7.46026173758937,-7.39963065398707));
#40164=CARTESIAN_POINT('Ctrl Pts',(-4.13913195941006,7.38558994759841,-7.40048304455997));
#40165=CARTESIAN_POINT('Ctrl Pts',(-4.23997658616605,7.34691725718564,-7.40092449958255));
#40166=CARTESIAN_POINT('Ctrl Pts',(-4.33969369867562,7.30714075765009,-7.40124445291142));
#40167=CARTESIAN_POINT('Ctrl Pts',(-4.43827307181376,7.26632831536047,-7.40142708854303));
#40168=CARTESIAN_POINT('Ctrl Pts',(-4.63592436459349,7.18449951362183,-7.40179327233531));
#40169=CARTESIAN_POINT('Ctrl Pts',(-4.82900095119531,7.09850894800746,-7.4016060823059));
#40170=CARTESIAN_POINT('Ctrl Pts',(-5.01748502204055,7.00887300417893,-7.40076120591469));
#40171=CARTESIAN_POINT('Ctrl Pts',(-5.20992697392762,6.9173548408018,-7.3998985883943));
#40172=CARTESIAN_POINT('Ctrl Pts',(-5.39758156089646,6.82203653720136,-7.39835044074719));
#40173=CARTESIAN_POINT('Ctrl Pts',(-5.5804485117512,6.72342214887826,-7.39602844414171));
#40174=CARTESIAN_POINT('Ctrl Pts',(-5.62728543047245,6.69816447345334,-7.39543372122554));
#40175=CARTESIAN_POINT('Ctrl Pts',(-5.67380837004966,6.67269034805117,-7.39478834450131));
#40176=CARTESIAN_POINT('Ctrl Pts',(-5.72001751101611,6.64700778276234,-7.39409105480892));
#40177=CARTESIAN_POINT('Ctrl Pts',(-5.71200137201152,6.68631702029758,-8.11922551140502));
#40178=CARTESIAN_POINT('Ctrl Pts',(-5.71752593264098,6.68350451781287,-8.11887479851681));
#40179=CARTESIAN_POINT('Ctrl Pts',(-5.76529466296359,6.65838320673758,-8.11644404322045));
#40180=CARTESIAN_POINT('Ctrl Pts',(-5.85056684041905,6.60034318303366,-8.12199201673112));
#40181=CARTESIAN_POINT('Ctrl Pts',(-5.9485659051434,6.49937427859963,-8.15388804757165));
#40182=CARTESIAN_POINT('Ctrl Pts',(-6.01626018410924,6.3902222746575,-8.20520228410394));
#40183=CARTESIAN_POINT('Ctrl Pts',(-6.04733840082506,6.29406348953598,-8.26306349687466));
#40184=CARTESIAN_POINT('Ctrl Pts',(-6.0514193600241,6.23884558946966,-8.30253412448785));
#40185=CARTESIAN_POINT('Ctrl Pts',(-6.05072408266302,6.21774110434867,-8.31866918503377));
#40186=CARTESIAN_POINT('Ctrl Pts',(-5.59593758434029,6.47862795026978,-7.91168787081027));
#40187=CARTESIAN_POINT('Ctrl Pts',(-5.60109254679665,6.47602393259023,-7.91133523079966));
#40188=CARTESIAN_POINT('Ctrl Pts',(-5.64567310121454,6.45276591384098,-7.90883421003711));
#40189=CARTESIAN_POINT('Ctrl Pts',(-5.72536150005282,6.39904474865737,-7.91338893404229));
#40190=CARTESIAN_POINT('Ctrl Pts',(-5.81694503696564,6.30576471974002,-7.94197422327985));
#40191=CARTESIAN_POINT('Ctrl Pts',(-5.88005388554802,6.20535296458813,-7.98843005024452));
#40192=CARTESIAN_POINT('Ctrl Pts',(-5.90885936553763,6.11755368429137,-8.04085370327794));
#40193=CARTESIAN_POINT('Ctrl Pts',(-5.9126015749991,6.06763592744995,-8.076478249824));
#40194=CARTESIAN_POINT('Ctrl Pts',(-5.91196326125511,6.04865028217018,-8.09100475681771));
#40195=CARTESIAN_POINT('Ctrl Pts',(-5.57882413750114,6.48053453245818,-7.59643955907908));
#40196=CARTESIAN_POINT('Ctrl Pts',(-5.58615398423115,6.47687427905703,-7.59596288053133));
#40197=CARTESIAN_POINT('Ctrl Pts',(-5.64947523397066,6.44422885305795,-7.59263309125204));
#40198=CARTESIAN_POINT('Ctrl Pts',(-5.76170274087936,6.3695931524597,-7.59961231738624));
#40199=CARTESIAN_POINT('Ctrl Pts',(-5.89066796668504,6.24048464928553,-7.64046879782618));
#40200=CARTESIAN_POINT('Ctrl Pts',(-5.98090855899055,6.09972137569547,-7.70688735341896));
#40201=CARTESIAN_POINT('Ctrl Pts',(-6.0235971880795,5.97279316563431,-7.78342716853378));
#40202=CARTESIAN_POINT('Ctrl Pts',(-6.02950570161484,5.89741576079667,-7.83730334457995));
#40203=CARTESIAN_POINT('Ctrl Pts',(-6.02850469510944,5.86813423963277,-7.85968193391842));
#40204=CARTESIAN_POINT('Ctrl Pts',(-5.67187599726008,6.6907870813339,-7.38007458214567));
#40205=CARTESIAN_POINT('Ctrl Pts',(-5.68249992573452,6.68549806344202,-7.37943304082086));
#40206=CARTESIAN_POINT('Ctrl Pts',(-5.77420924649652,6.63836645847544,-7.37505910349267));
#40207=CARTESIAN_POINT('Ctrl Pts',(-5.93577462414858,6.53128892558299,-7.38629171363848));
#40208=CARTESIAN_POINT('Ctrl Pts',(-6.12142110281481,6.34631437177203,-7.44695953508515));
#40209=CARTESIAN_POINT('Ctrl Pts',(-6.25273014201225,6.14255171031536,-7.54507961510835));
#40210=CARTESIAN_POINT('Ctrl Pts',(-6.31635964671171,5.95464882433744,-7.65948506785012));
#40211=CARTESIAN_POINT('Ctrl Pts',(-6.32551985612253,5.839736663941,-7.74174959118279));
#40212=CARTESIAN_POINT('Ctrl Pts',(-6.32397418693164,5.79449183343361,-7.77629512811694));
#40213=CARTESIAN_POINT('',(-5.99998809173015,6.09546018036231,-8.13557732097441));
#40214=CARTESIAN_POINT('',(-5.99999999616315,6.4401456877457,-7.42970720374052));
#40215=CARTESIAN_POINT('Ctrl Pts',(-5.99998809173015,6.09546018036231,-8.13557732097441));
#40216=CARTESIAN_POINT('Ctrl Pts',(-5.99998614033837,6.09852832454662,-8.11172602130616));
#40217=CARTESIAN_POINT('Ctrl Pts',(-5.99998781129153,6.10206242548599,-8.08802362797946));
#40218=CARTESIAN_POINT('Ctrl Pts',(-6.00000062824682,6.10612629471922,-8.06456699740365));
#40219=CARTESIAN_POINT('Ctrl Pts',(-6.00000707142059,6.10816923042823,-8.05277518387173));
#40220=CARTESIAN_POINT('Ctrl Pts',(-6.00001566896851,6.11034552813368,-8.04104576003382));
#40221=CARTESIAN_POINT('Ctrl Pts',(-6.0000244752749,6.11265957726614,-8.02939240223511));
#40222=CARTESIAN_POINT('Ctrl Pts',(-6.00004292770159,6.11750835496144,-8.00497436349195));
#40223=CARTESIAN_POINT('Ctrl Pts',(-6.0000639885888,6.12296503416167,-7.98088990423614));
#40224=CARTESIAN_POINT('Ctrl Pts',(-6.00008526219676,6.12903222827216,-7.95725886271824));
#40225=CARTESIAN_POINT('Ctrl Pts',(-6.00009914086696,6.13299039965054,-7.94184222852553));
#40226=CARTESIAN_POINT('Ctrl Pts',(-6.00011245325555,6.13720738562287,-7.92661880791639));
#40227=CARTESIAN_POINT('Ctrl Pts',(-6.00012171175195,6.14167237067045,-7.91162211399328));
#40228=CARTESIAN_POINT('Ctrl Pts',(-6.00013624555423,6.14868141479889,-7.88808060414107));
#40229=CARTESIAN_POINT('Ctrl Pts',(-6.00013967179948,6.15630399211504,-7.86509883736143));
#40230=CARTESIAN_POINT('Ctrl Pts',(-6.00012396232579,6.16445611094957,-7.84279762684001));
#40231=CARTESIAN_POINT('Ctrl Pts',(-6.00011958298537,6.1667286825347,-7.83658070356233));
#40232=CARTESIAN_POINT('Ctrl Pts',(-6.00011380591016,6.16904212195121,-7.83041656999937));
#40233=CARTESIAN_POINT('Ctrl Pts',(-6.00010670568612,6.17139398746753,-7.82430758167122));
#40234=CARTESIAN_POINT('Ctrl Pts',(-6.00010098822625,6.17328782865677,-7.81938831496988));
#40235=CARTESIAN_POINT('Ctrl Pts',(-6.00009441688719,6.17520658170548,-7.81450480268433));
#40236=CARTESIAN_POINT('Ctrl Pts',(-6.00008719772562,6.17714893736528,-7.80965812022649));
#40237=CARTESIAN_POINT('Ctrl Pts',(-6.00006865390096,6.1821382567506,-7.79720847094657));
#40238=CARTESIAN_POINT('Ctrl Pts',(-6.00005102576016,6.18734715796721,-7.78482922322189));
#40239=CARTESIAN_POINT('Ctrl Pts',(-6.00003057015073,6.19268901813973,-7.77273754654777));
#40240=CARTESIAN_POINT('Ctrl Pts',(-6.00000992968195,6.19807915322845,-7.76053659620135));
#40241=CARTESIAN_POINT('Ctrl Pts',(-5.99998595813927,6.20360451483891,-7.7486289442589));
#40242=CARTESIAN_POINT('Ctrl Pts',(-5.9999679154756,6.20912493297519,-7.73722698573307));
#40243=CARTESIAN_POINT('Ctrl Pts',(-5.99995722328527,6.21239636575918,-7.73047011695934));
#40244=CARTESIAN_POINT('Ctrl Pts',(-5.99994890968132,6.21566508061159,-7.72389058671366));
#40245=CARTESIAN_POINT('Ctrl Pts',(-5.99994782973637,6.21889429253799,-7.71752989090999));
#40246=CARTESIAN_POINT('Ctrl Pts',(-5.99994380484488,6.23092937595653,-7.69382395077915));
#40247=CARTESIAN_POINT('Ctrl Pts',(-5.99996594985854,6.2438453349866,-7.67052094837828));
#40248=CARTESIAN_POINT('Ctrl Pts',(-5.99999369856138,6.2576313664447,-7.6478095149004));
#40249=CARTESIAN_POINT('Ctrl Pts',(-6.00002003739153,6.27071694897144,-7.62625201751771));
#40250=CARTESIAN_POINT('Ctrl Pts',(-6.0000506789523,6.28458595267117,-7.60522848329486));
#40251=CARTESIAN_POINT('Ctrl Pts',(-6.00007008721582,6.29917668151905,-7.58489634214688));
#40252=CARTESIAN_POINT('Ctrl Pts',(-6.00007112610709,6.2999576983678,-7.5838079972826));
#40253=CARTESIAN_POINT('Ctrl Pts',(-6.000072134762,6.30074077123508,-7.58272163050395));
#40254=CARTESIAN_POINT('Ctrl Pts',(-6.00007311154347,6.30152588665487,-7.58163726482764));
#40255=CARTESIAN_POINT('Ctrl Pts',(-6.00009137615595,6.31620657972263,-7.56136095988436));
#40256=CARTESIAN_POINT('Ctrl Pts',(-6.00009744663363,6.33160530345637,-7.54178609901824));
#40257=CARTESIAN_POINT('Ctrl Pts',(-6.00008943235725,6.34761295506631,-7.5230490340063));
#40258=CARTESIAN_POINT('Ctrl Pts',(-6.00008131870252,6.36381910421309,-7.50407962627832));
#40259=CARTESIAN_POINT('Ctrl Pts',(-6.00005836465068,6.38064866194837,-7.48596970036587));
#40260=CARTESIAN_POINT('Ctrl Pts',(-6.00003565608961,6.39794656555899,-7.46883145061165));
#40261=CARTESIAN_POINT('Ctrl Pts',(-6.00001753956961,6.41174655120251,-7.45515883421331));
#40262=CARTESIAN_POINT('Ctrl Pts',(-5.99999991840031,6.42584360010603,-7.4421041232633));
#40263=CARTESIAN_POINT('Ctrl Pts',(-5.99999992131821,6.44014555029568,-7.42970704517059));
#40264=CARTESIAN_POINT('Ctrl Pts',(-5.7200186792313,6.64700982300718,-7.39409332430001));
#40265=CARTESIAN_POINT('Ctrl Pts',(-5.77263456945053,6.61776016162055,-7.39330425574794));
#40266=CARTESIAN_POINT('Ctrl Pts',(-5.82217073198462,6.58571612012162,-7.39609700292507));
#40267=CARTESIAN_POINT('Ctrl Pts',(-5.868800030588,6.55119618956499,-7.40209721534042));
#40268=CARTESIAN_POINT('Ctrl Pts',(-5.91542932731003,6.51667626040112,-7.40809742751368));
#40269=CARTESIAN_POINT('Ctrl Pts',(-5.95915199503726,6.47968081216783,-7.41730553493613));
#40270=CARTESIAN_POINT('Ctrl Pts',(-6.00000008250492,6.44014582409289,-7.42970735400782));
#40271=CARTESIAN_POINT('Ctrl Pts',(-5.73278520173054,6.65587881687604,-8.10255227250958));
#40272=CARTESIAN_POINT('Ctrl Pts',(-5.74762629760419,6.64186178191593,-8.09760842313734));
#40273=CARTESIAN_POINT('Ctrl Pts',(-5.76162678132051,6.62763291182143,-8.0934228773982));
#40274=CARTESIAN_POINT('Ctrl Pts',(-5.77478496304676,6.61338734380077,-8.08987534016305));
#40275=CARTESIAN_POINT('Ctrl Pts',(-5.78881567284001,6.59819714238114,-8.08609256329747));
#40276=CARTESIAN_POINT('Ctrl Pts',(-5.80188881891289,6.58298772744398,-8.08303539958181));
#40277=CARTESIAN_POINT('Ctrl Pts',(-5.81403036341231,6.56794750122288,-8.08057762221901));
#40278=CARTESIAN_POINT('Ctrl Pts',(-5.81727080485107,6.56393343428951,-8.0799216691305));
#40279=CARTESIAN_POINT('Ctrl Pts',(-5.8204450272239,6.55993117890586,-8.07930850351914));
#40280=CARTESIAN_POINT('Ctrl Pts',(-5.82355381037148,6.55594381974502,-8.07873591648801));
#40281=CARTESIAN_POINT('Ctrl Pts',(-5.83603219891105,6.53993890254953,-8.07643760132479));
#40282=CARTESIAN_POINT('Ctrl Pts',(-5.84745527801701,6.52417836019587,-8.07479074156169));
#40283=CARTESIAN_POINT('Ctrl Pts',(-5.85790553240099,6.50885077338267,-8.0736434501055));
#40284=CARTESIAN_POINT('Ctrl Pts',(-5.86877308233067,6.49291113125786,-8.07245034544738));
#40285=CARTESIAN_POINT('Ctrl Pts',(-5.87858892580013,6.47743905626987,-8.07179789810214));
#40286=CARTESIAN_POINT('Ctrl Pts',(-5.88745828632321,6.46259199003365,-8.0715436304873));
#40287=CARTESIAN_POINT('Ctrl Pts',(-5.89162957320336,6.45560937021132,-8.07142404766472));
#40288=CARTESIAN_POINT('Ctrl Pts',(-5.8955916611711,6.44876428570152,-8.07139290003505));
#40289=CARTESIAN_POINT('Ctrl Pts',(-5.8993561323307,6.44206972988576,-8.07143712060889));
#40290=CARTESIAN_POINT('Ctrl Pts',(-5.90168368711965,6.43793051755335,-8.07146446198144));
#40291=CARTESIAN_POINT('Ctrl Pts',(-5.90393570203241,6.4338488111739,-8.07152063639131));
#40292=CARTESIAN_POINT('Ctrl Pts',(-5.90611496800989,6.42982732608125,-8.0716027422794));
#40293=CARTESIAN_POINT('Ctrl Pts',(-5.90944521738537,6.42368188612273,-8.0717282125457));
#40294=CARTESIAN_POINT('Ctrl Pts',(-5.91260560611597,6.41767715783716,-8.07191417930119));
#40295=CARTESIAN_POINT('Ctrl Pts',(-5.91560709582519,6.41182246680458,-8.07215001690292));
#40296=CARTESIAN_POINT('Ctrl Pts',(-5.91808990593493,6.4069795096422,-8.07234510002448));
#40297=CARTESIAN_POINT('Ctrl Pts',(-5.92046392144401,6.40223928765411,-8.07257430320933));
#40298=CARTESIAN_POINT('Ctrl Pts',(-5.92273529257371,6.39760620780249,-8.07283214767203));
#40299=CARTESIAN_POINT('Ctrl Pts',(-5.92387097813855,6.39528966787668,-8.07296106990338));
#40300=CARTESIAN_POINT('Ctrl Pts',(-5.9249809953795,6.39299991032722,-8.07309715638919));
#40301=CARTESIAN_POINT('Ctrl Pts',(-5.92606609131996,6.39073744462867,-8.07323976033666));
#40302=CARTESIAN_POINT('Ctrl Pts',(-5.926827454153,6.3891499745906,-8.07333981908851));
#40303=CARTESIAN_POINT('Ctrl Pts',(-5.92726381041733,6.38823388318992,-8.07339909990531));
#40304=CARTESIAN_POINT('Ctrl Pts',(-5.92803487088773,6.38660482663352,-8.07350917997331));
#40305=CARTESIAN_POINT('Ctrl Pts',(-5.92836272745133,6.38591214829637,-8.07355598625401));
#40306=CARTESIAN_POINT('Ctrl Pts',(-5.92875078185222,6.38509044622351,-8.07361219599087));
#40307=CARTESIAN_POINT('Ctrl Pts',(-5.92924734241237,6.3840324112441,-8.07368649483813));
#40308=CARTESIAN_POINT('Ctrl Pts',(-5.93919299879007,6.36284093293236,-8.07517463317085));
#40309=CARTESIAN_POINT('Ctrl Pts',(-5.94793107358897,6.3420071871622,-8.07733441703594));
#40310=CARTESIAN_POINT('Ctrl Pts',(-5.95553872020091,6.32169894627584,-8.08002898480051));
#40311=CARTESIAN_POINT('Ctrl Pts',(-5.95863181590775,6.31344207842914,-8.08112453463471));
#40312=CARTESIAN_POINT('Ctrl Pts',(-5.96153809863311,6.30527152009402,-8.08230877042614));
#40313=CARTESIAN_POINT('Ctrl Pts',(-5.96426303055246,6.29719641142837,-8.08357353496591));
#40314=CARTESIAN_POINT('Ctrl Pts',(-5.97109019756844,6.27696467090637,-8.0867423329412));
#40315=CARTESIAN_POINT('Ctrl Pts',(-5.97677989589696,6.25733527366989,-8.09041450330044));
#40316=CARTESIAN_POINT('Ctrl Pts',(-5.98146315778518,6.23843868552022,-8.09444883517228));
#40317=CARTESIAN_POINT('Ctrl Pts',(-5.98644690024909,6.21832968221606,-8.09874201192454));
#40318=CARTESIAN_POINT('Ctrl Pts',(-5.99029046242889,6.19905036821662,-8.10344555835054));
#40319=CARTESIAN_POINT('Ctrl Pts',(-5.99314481922394,6.18070836123524,-8.10841954843399));
#40320=CARTESIAN_POINT('Ctrl Pts',(-5.99383961628356,6.17624361718492,-8.10963029885263));
#40321=CARTESIAN_POINT('Ctrl Pts',(-5.99447578898681,6.17183419912674,-8.11085719687801));
#40322=CARTESIAN_POINT('Ctrl Pts',(-5.99505550273162,6.16748126860043,-8.11209845041418));
#40323=CARTESIAN_POINT('Ctrl Pts',(-5.99754124264647,6.14881644781163,-8.11742079008077));
#40324=CARTESIAN_POINT('Ctrl Pts',(-5.99899094575813,6.13119319818402,-8.12300451323803));
#40325=CARTESIAN_POINT('Ctrl Pts',(-5.9996181811312,6.11467246052096,-8.12870975260029));
#40326=CARTESIAN_POINT('Ctrl Pts',(-5.99986797364141,6.10809318149992,-8.13098182800101));
#40327=CARTESIAN_POINT('Ctrl Pts',(-5.99998707059393,6.10168833650056,-8.13327352536238));
#40328=CARTESIAN_POINT('Ctrl Pts',(-5.99998809173015,6.09546018036231,-8.13557732097441));
#40329=CARTESIAN_POINT('Ctrl Pts',(-5.72202397771648,10.2826310612706,-17.037335075537));
#40330=CARTESIAN_POINT('Ctrl Pts',(-5.72274491315933,10.3310956803065,-16.560067518738));
#40331=CARTESIAN_POINT('Ctrl Pts',(-5.72404046055613,10.3627269173045,-15.5563860123165));
#40332=CARTESIAN_POINT('Ctrl Pts',(-5.72530462330493,10.1890957103804,-14.0392334779456));
#40333=CARTESIAN_POINT('Ctrl Pts',(-5.72546453572454,9.77722809651949,-12.5261342131263));
#40334=CARTESIAN_POINT('Ctrl Pts',(-5.72471277436271,9.14170964943181,-11.0927040517244));
#40335=CARTESIAN_POINT('Ctrl Pts',(-5.72306496928055,8.29718534881308,-9.7712877786294));
#40336=CARTESIAN_POINT('Ctrl Pts',(-5.7203882568828,7.319416170681,-8.65807750094687));
#40337=CARTESIAN_POINT('Ctrl Pts',(-5.7182966466807,6.59327323403327,-8.03228802666557));
#40338=CARTESIAN_POINT('Ctrl Pts',(-5.71724105953304,6.24681320759565,-7.76998411580299));
#40339=CARTESIAN_POINT('Ctrl Pts',(-5.90002812422718,10.2259058223041,-17.0315448724223));
#40340=CARTESIAN_POINT('Ctrl Pts',(-5.90064109140466,10.273764758127,-16.5568923148414));
#40341=CARTESIAN_POINT('Ctrl Pts',(-5.901741328884,10.3046069941456,-15.5587623015314));
#40342=CARTESIAN_POINT('Ctrl Pts',(-5.90281088151832,10.1313725119932,-14.0503248888921));
#40343=CARTESIAN_POINT('Ctrl Pts',(-5.90294613974592,9.72176930505232,-12.5458334775211));
#40344=CARTESIAN_POINT('Ctrl Pts',(-5.90231016726573,9.09020456074211,-11.1204468081396));
#40345=CARTESIAN_POINT('Ctrl Pts',(-5.90091446861734,8.25108189201988,-9.80603023482109));
#40346=CARTESIAN_POINT('Ctrl Pts',(-5.89863677263844,7.27969287036672,-8.69816806086486));
#40347=CARTESIAN_POINT('Ctrl Pts',(-5.89685243426304,6.55808918076619,-8.07498723699972));
#40348=CARTESIAN_POINT('Ctrl Pts',(-5.89594596532901,6.2137775747096,-7.81368830926344));
#40349=CARTESIAN_POINT('Ctrl Pts',(-6.0072809883487,10.0734860462671,-17.0159867249596));
#40350=CARTESIAN_POINT('Ctrl Pts',(-6.00760395029268,10.1204165494032,-16.548432100775));
#40351=CARTESIAN_POINT('Ctrl Pts',(-6.00818201264186,10.1504140238049,-15.5651446473605));
#40352=CARTESIAN_POINT('Ctrl Pts',(-6.00873882863447,9.97943362493164,-14.0795567262227));
#40353=CARTESIAN_POINT('Ctrl Pts',(-6.0088091981725,9.57592251317866,-12.5976212484565));
#40354=CARTESIAN_POINT('Ctrl Pts',(-6.00847818312919,8.95410325942813,-11.1936935666068));
#40355=CARTESIAN_POINT('Ctrl Pts',(-6.00774957909008,8.12794887207174,-9.89868029665919));
#40356=CARTESIAN_POINT('Ctrl Pts',(-6.00654714904829,7.17173485299533,-8.80693139848031));
#40357=CARTESIAN_POINT('Ctrl Pts',(-6.00559943123166,6.46120738736004,-8.1924918516984));
#40358=CARTESIAN_POINT('Ctrl Pts',(-6.00511044224782,6.12220788075211,-7.9348294930684));
#40359=CARTESIAN_POINT('Ctrl Pts',(-5.99966790381059,9.88747851054264,-16.9970001412723));
#40360=CARTESIAN_POINT('Ctrl Pts',(-5.99963699265514,9.93353691820315,-16.5381342555582));
#40361=CARTESIAN_POINT('Ctrl Pts',(-5.99957878926884,9.96297950349812,-15.5729324201564));
#40362=CARTESIAN_POINT('Ctrl Pts',(-5.99951367917714,9.79519339046945,-14.1150172035289));
#40363=CARTESIAN_POINT('Ctrl Pts',(-5.9995053673528,9.39911971302706,-12.6603941934467));
#40364=CARTESIAN_POINT('Ctrl Pts',(-5.99954420986514,8.78886574866588,-11.2825968892181));
#40365=CARTESIAN_POINT('Ctrl Pts',(-5.99962585484118,7.97796036473452,-10.0114848862901));
#40366=CARTESIAN_POINT('Ctrl Pts',(-5.99973680304981,7.03953062065321,-8.94005066472971));
#40367=CARTESIAN_POINT('Ctrl Pts',(-5.99981416734842,6.34210186098044,-8.33692512051669));
#40368=CARTESIAN_POINT('Ctrl Pts',(-5.99984092736157,6.0094130898816,-8.08405015709546));
#40369=CARTESIAN_POINT('',(-5.99999988467789,9.9132994413493,-16.899370324403));
#40370=CARTESIAN_POINT('Origin',(-5.59998164335621,9.91328771266205,-16.8993697091815));
#40371=CARTESIAN_POINT('Ctrl Pts',(-6.,9.91329812083799,-16.8993691889257));
#40372=CARTESIAN_POINT('Ctrl Pts',(-6.,9.95683978041412,-16.4254094363205));
#40373=CARTESIAN_POINT('Ctrl Pts',(-6.,9.96638815220342,-15.9532839355417));
#40374=CARTESIAN_POINT('Ctrl Pts',(-6.,9.94189523357363,-15.4800412069182));
#40375=CARTESIAN_POINT('Ctrl Pts',(-6.,9.91740229762106,-15.0067981435907));
#40376=CARTESIAN_POINT('Ctrl Pts',(-6.,9.85886802309754,-14.5324378508381));
#40377=CARTESIAN_POINT('Ctrl Pts',(-6.,9.76681037528992,-14.0658326605446));
#40378=CARTESIAN_POINT('Ctrl Pts',(-6.,9.67475272748236,-13.5992274702515));
#40379=CARTESIAN_POINT('Ctrl Pts',(-6.,9.54917170639076,-13.1403773824174));
#40380=CARTESIAN_POINT('Ctrl Pts',(-6.,9.39100129395212,-12.691978875132));
#40381=CARTESIAN_POINT('Ctrl Pts',(-6.,9.23283088151338,-12.2435803678463));
#40382=CARTESIAN_POINT('Ctrl Pts',(-6.,9.04207107772757,-11.8056334411093));
#40383=CARTESIAN_POINT('Ctrl Pts',(-6.,8.82146087395316,-11.3843740208869));
#40384=CARTESIAN_POINT('Ctrl Pts',(-6.,8.60085067017891,-10.9631146006647));
#40385=CARTESIAN_POINT('Ctrl Pts',(-6.,8.35039006641611,-10.5585426869571));
#40386=CARTESIAN_POINT('Ctrl Pts',(-6.,8.07150645159638,-10.1733978041594));
#40387=CARTESIAN_POINT('Ctrl Pts',(-6.,7.79262283677646,-9.78825292136152));
#40388=CARTESIAN_POINT('Ctrl Pts',(-6.,7.48531621089955,-9.42253506947359));
#40389=CARTESIAN_POINT('Ctrl Pts',(-6.,7.15537147961372,-9.08219260210466));
#40390=CARTESIAN_POINT('Ctrl Pts',(-6.,6.82542674832812,-8.74185013473596));
#40391=CARTESIAN_POINT('Ctrl Pts',(-6.,6.47284391163362,-8.42688305188624));
#40392=CARTESIAN_POINT('Ctrl Pts',(-6.,6.09546018150529,-8.13557732045525));
#40393=CARTESIAN_POINT('Origin',(-5.599999999997,9.91330329093349,-16.899368849389));
#40394=CARTESIAN_POINT('Origin',(-5.6,9.91330329095944,-16.8993688494318));
#40395=CARTESIAN_POINT('Ctrl Pts',(-6.05069755286452,4.09530921457736,-9.54399861839001));
#40396=CARTESIAN_POINT('Ctrl Pts',(-6.05139439140886,4.07077799860572,-9.55420987696813));
#40397=CARTESIAN_POINT('Ctrl Pts',(-6.04731517240641,4.00898140897246,-9.58229613908414));
#40398=CARTESIAN_POINT('Ctrl Pts',(-6.01623683914788,3.9107894786984,-9.63664297345575));
#40399=CARTESIAN_POINT('Ctrl Pts',(-5.9485470217377,3.81177761901256,-9.70551105786188));
#40400=CARTESIAN_POINT('Ctrl Pts',(-5.85055617149809,3.73367302953022,-9.77700044850094));
#40401=CARTESIAN_POINT('Ctrl Pts',(-5.76530789870929,3.69985386375794,-9.82447901550751));
#40402=CARTESIAN_POINT('Ctrl Pts',(-5.71756150656501,3.68939776309269,-9.84744168818631));
#40403=CARTESIAN_POINT('Ctrl Pts',(-5.71205470319225,3.68829782904571,-9.85004476031037));
#40404=CARTESIAN_POINT('Ctrl Pts',(-5.91199537999528,3.98270422300683,-9.2837621698363));
#40405=CARTESIAN_POINT('Ctrl Pts',(-5.91263520020597,3.9606235181659,-9.29294359029123));
#40406=CARTESIAN_POINT('Ctrl Pts',(-5.90889416717406,3.90480218592893,-9.31836542063868));
#40407=CARTESIAN_POINT('Ctrl Pts',(-5.88008575414045,3.81549053213944,-9.36819605709431));
#40408=CARTESIAN_POINT('Ctrl Pts',(-5.81697549178688,3.72504770653924,-9.43192966962737));
#40409=CARTESIAN_POINT('Ctrl Pts',(-5.72539191842396,3.65364813821231,-9.49842128531275));
#40410=CARTESIAN_POINT('Ctrl Pts',(-5.64571912788174,3.62284523330527,-9.54266060677016));
#40411=CARTESIAN_POINT('Ctrl Pts',(-5.601155517203,3.61338071461377,-9.5640471330943));
#40412=CARTESIAN_POINT('Ctrl Pts',(-5.59601666916031,3.61238633551412,-9.56647137060792));
#40413=CARTESIAN_POINT('Ctrl Pts',(-6.02851531559025,3.87266147843904,-9.01181418246432));
#40414=CARTESIAN_POINT('Ctrl Pts',(-6.02951858501767,3.83863157203546,-9.02598629563478));
#40415=CARTESIAN_POINT('Ctrl Pts',(-6.02361237825883,3.75427593904666,-9.0643298376604));
#40416=CARTESIAN_POINT('Ctrl Pts',(-5.98092300637074,3.62451976792727,-9.13598611800144));
#40417=CARTESIAN_POINT('Ctrl Pts',(-5.89068726945848,3.49662036141256,-9.22467856542358));
#40418=CARTESIAN_POINT('Ctrl Pts',(-5.76173137337581,3.39668502760156,-9.31605732679907));
#40419=CARTESIAN_POINT('Ctrl Pts',(-5.64953417929655,3.35332938988757,-9.37718983283142));
#40420=CARTESIAN_POINT('Ctrl Pts',(-5.58624215424927,3.33988942963279,-9.40711563376416));
#40421=CARTESIAN_POINT('Ctrl Pts',(-5.57893584696836,3.3384754226433,-9.41051341605323));
#40422=CARTESIAN_POINT('Ctrl Pts',(-6.32391758555148,3.83727685773935,-8.90632479261494));
#40423=CARTESIAN_POINT('Ctrl Pts',(-6.32546665298515,3.78472672174695,-8.92823840796942));
#40424=CARTESIAN_POINT('Ctrl Pts',(-6.31631045619702,3.65602187178656,-8.98662396698808));
#40425=CARTESIAN_POINT('Ctrl Pts',(-6.25268354791552,3.46299417507872,-9.09214836051762));
#40426=CARTESIAN_POINT('Ctrl Pts',(-6.1213889355671,3.27615277066782,-9.21954082369584));
#40427=CARTESIAN_POINT('Ctrl Pts',(-5.93576610989893,3.1311364871012,-9.34938649381138));
#40428=CARTESIAN_POINT('Ctrl Pts',(-5.77425343810608,3.06788321990275,-9.43647681126404));
#40429=CARTESIAN_POINT('Ctrl Pts',(-5.68259198183112,3.04810536026742,-9.47946268409793));
#40430=CARTESIAN_POINT('Ctrl Pts',(-5.67200284155713,3.04602146758907,-9.48434855924641));
#40431=CARTESIAN_POINT('',(-5.7327876945012,3.68906971078177,-9.8154375057469));
#40432=CARTESIAN_POINT('',(-5.7200181592662,3.07996731899951,-9.45352474346443));
#40433=CARTESIAN_POINT('Origin',(-5.89876031575697,3.22462567369242,-9.89750035628898));
#40434=CARTESIAN_POINT('',(-5.99999999681367,3.21424228399819,-9.29218338999141));
#40435=CARTESIAN_POINT('Ctrl Pts',(-6.00000008328868,3.21424234556147,-9.29218358296574));
#40436=CARTESIAN_POINT('Ctrl Pts',(-5.9591513766782,3.1837340995611,-9.32022140189732));
#40437=CARTESIAN_POINT('Ctrl Pts',(-5.91542827662098,3.15726183429538,-9.34765654781793));
#40438=CARTESIAN_POINT('Ctrl Pts',(-5.86879893709601,3.13480561381036,-9.37455156189743));
#40439=CARTESIAN_POINT('Ctrl Pts',(-5.8221695955671,3.11234939236026,-9.40144657713277));
#40440=CARTESIAN_POINT('Ctrl Pts',(-5.77263377979091,3.09390902843134,-9.42780092518505));
#40441=CARTESIAN_POINT('Ctrl Pts',(-5.72001867762027,3.07996773844747,-9.45352603095761));
#40442=CARTESIAN_POINT('',(-5.99998808311064,3.99788652747824,-9.34661203061488));
#40443=CARTESIAN_POINT('Ctrl Pts',(-5.99998808311064,3.99788652747824,-9.34661203061488));
#40444=CARTESIAN_POINT('Ctrl Pts',(-5.99998579341305,3.97186927865861,-9.33574485652103));
#40445=CARTESIAN_POINT('Ctrl Pts',(-5.99998684304345,3.94595612801873,-9.32570975247612));
#40446=CARTESIAN_POINT('Ctrl Pts',(-5.99998299235381,3.92014869004665,-9.31654001952392));
#40447=CARTESIAN_POINT('Ctrl Pts',(-5.99998186343085,3.91258261440246,-9.31385169016598));
#40448=CARTESIAN_POINT('Ctrl Pts',(-5.9999801250393,3.90502573855629,-9.31123744936816));
#40449=CARTESIAN_POINT('Ctrl Pts',(-5.99997728605667,3.89747832269323,-9.30869745889218));
#40450=CARTESIAN_POINT('Ctrl Pts',(-5.99996366357526,3.8612630492276,-9.29650965165367));
#40451=CARTESIAN_POINT('Ctrl Pts',(-5.99992845379828,3.82526738685101,-9.28603455207253));
#40452=CARTESIAN_POINT('Ctrl Pts',(-5.99991579096825,3.78947379315245,-9.2772235887423));
#40453=CARTESIAN_POINT('Ctrl Pts',(-5.99991509405309,3.78750384661685,-9.27673866602585));
#40454=CARTESIAN_POINT('Ctrl Pts',(-5.99991445984403,3.78553450404061,-9.27625877781718));
#40455=CARTESIAN_POINT('Ctrl Pts',(-5.99991389460418,3.78356575918368,-9.2757839149007));
#40456=CARTESIAN_POINT('Ctrl Pts',(-5.99990496077822,3.75244901488712,-9.26827852998715));
#40457=CARTESIAN_POINT('Ctrl Pts',(-5.99990285316706,3.72148342877298,-9.26205336045457));
#40458=CARTESIAN_POINT('Ctrl Pts',(-5.99990386436181,3.6906829130877,-9.25710757884461));
#40459=CARTESIAN_POINT('Ctrl Pts',(-5.99990457445796,3.66905371924126,-9.25363447890509));
#40460=CARTESIAN_POINT('Ctrl Pts',(-5.99990726531124,3.64750534606039,-9.25079193579496));
#40461=CARTESIAN_POINT('Ctrl Pts',(-5.99991517820639,3.62603054452835,-9.24858550131508));
#40462=CARTESIAN_POINT('Ctrl Pts',(-5.99991811031894,3.61807308597285,-9.24776791001381));
#40463=CARTESIAN_POINT('Ctrl Pts',(-5.99992619871551,3.60985636020238,-9.24700745409626));
#40464=CARTESIAN_POINT('Ctrl Pts',(-5.99993158137481,3.60174918672314,-9.24635368447191));
#40465=CARTESIAN_POINT('Ctrl Pts',(-5.99993703257443,3.59353878021062,-9.24569159004464));
#40466=CARTESIAN_POINT('Ctrl Pts',(-5.99993943567107,3.5854410647341,-9.24513895522679));
#40467=CARTESIAN_POINT('Ctrl Pts',(-5.99994447713256,3.57785510414327,-9.24469688598806));
#40468=CARTESIAN_POINT('Ctrl Pts',(-5.99994531264981,3.5765978891561,-9.24462362221802));
#40469=CARTESIAN_POINT('Ctrl Pts',(-5.99994625522812,3.57535475773664,-9.24455328746695));
#40470=CARTESIAN_POINT('Ctrl Pts',(-5.9999473718635,3.57412755605516,-9.24448576306536));
#40471=CARTESIAN_POINT('Ctrl Pts',(-5.99997424819204,3.54459000396275,-9.24286051632755));
#40472=CARTESIAN_POINT('Ctrl Pts',(-5.9999604183843,3.51545932585125,-9.24253390810929));
#40473=CARTESIAN_POINT('Ctrl Pts',(-5.99993587232395,3.48674320219651,-9.24342539985017));
#40474=CARTESIAN_POINT('Ctrl Pts',(-5.99991530510076,3.46268186950695,-9.24417238365708));
#40475=CARTESIAN_POINT('Ctrl Pts',(-5.99988812252707,3.43891057700592,-9.2457750610003));
#40476=CARTESIAN_POINT('Ctrl Pts',(-5.99987117432901,3.41542447440808,-9.24821300048202));
#40477=CARTESIAN_POINT('Ctrl Pts',(-5.99985202935563,3.38889417263689,-9.25096693847068));
#40478=CARTESIAN_POINT('Ctrl Pts',(-5.99984750936127,3.36272649206113,-9.25478616413407));
#40479=CARTESIAN_POINT('Ctrl Pts',(-5.99986528824152,3.33691195950075,-9.25968264302251));
#40480=CARTESIAN_POINT('Ctrl Pts',(-5.9998825122732,3.31190305453613,-9.26442631114418));
#40481=CARTESIAN_POINT('Ctrl Pts',(-5.99992124729762,3.28722486563241,-9.27018190377966));
#40482=CARTESIAN_POINT('Ctrl Pts',(-5.9999558782658,3.26288698839438,-9.27699111499168));
#40483=CARTESIAN_POINT('Ctrl Pts',(-5.99997917531694,3.24651433696959,-9.28157182844347));
#40484=CARTESIAN_POINT('Ctrl Pts',(-5.99999991524942,3.23029611050298,-9.28663002149779));
#40485=CARTESIAN_POINT('Ctrl Pts',(-5.99999992273962,3.2142422154948,-9.29218319195217));
#40486=CARTESIAN_POINT('Ctrl Pts',(-5.99998808311064,3.99788652747824,-9.34661203061488));
#40487=CARTESIAN_POINT('Ctrl Pts',(-5.99998551891527,3.98506101158456,-9.35726021948571));
#40488=CARTESIAN_POINT('Ctrl Pts',(-5.99924019469057,3.97174114049352,-9.36891242702109));
#40489=CARTESIAN_POINT('Ctrl Pts',(-5.99754680958626,3.9580607789439,-9.3815924924929));
#40490=CARTESIAN_POINT('Ctrl Pts',(-5.99687196577081,3.95260891370579,-9.38664572211056));
#40491=CARTESIAN_POINT('Ctrl Pts',(-5.9960463470293,3.94710027549565,-9.39186201124298));
#40492=CARTESIAN_POINT('Ctrl Pts',(-5.99505598210094,3.94154535750297,-9.39724211738209));
#40493=CARTESIAN_POINT('Ctrl Pts',(-5.99264929769866,3.92804635919838,-9.41031630565024));
#40494=CARTESIAN_POINT('Ctrl Pts',(-5.98926946557905,3.9142709411533,-9.42435983375565));
#40495=CARTESIAN_POINT('Ctrl Pts',(-5.98476114128937,3.90038875329463,-9.43935506675853));
#40496=CARTESIAN_POINT('Ctrl Pts',(-5.98055933660131,3.88745041117965,-9.45333077841581));
#40497=CARTESIAN_POINT('Ctrl Pts',(-5.97537763920637,3.87441904409948,-9.46813319482114));
#40498=CARTESIAN_POINT('Ctrl Pts',(-5.96908598668068,3.86147236049078,-9.48372558770977));
#40499=CARTESIAN_POINT('Ctrl Pts',(-5.96754611687718,3.85830368468373,-9.48754179575297));
#40500=CARTESIAN_POINT('Ctrl Pts',(-5.96593972225518,3.85514029170247,-9.49140521264629));
#40501=CARTESIAN_POINT('Ctrl Pts',(-5.96426481102341,3.85198521734112,-9.49531507433625));
#40502=CARTESIAN_POINT('Ctrl Pts',(-5.96381007643915,3.85112862183875,-9.49637659287905));
#40503=CARTESIAN_POINT('Ctrl Pts',(-5.96335029114559,3.85027264058767,-9.49744153437959));
#40504=CARTESIAN_POINT('Ctrl Pts',(-5.96288542932361,3.84941732573222,-9.49850988238613));
#40505=CARTESIAN_POINT('Ctrl Pts',(-5.95829898380248,3.84097857081097,-9.50905047681218));
#40506=CARTESIAN_POINT('Ctrl Pts',(-5.95321825980051,3.83260404402286,-9.51992311623898));
#40507=CARTESIAN_POINT('Ctrl Pts',(-5.94761928869927,3.8243480581809,-9.53110902528923));
#40508=CARTESIAN_POINT('Ctrl Pts',(-5.94481980314865,3.82022006525991,-9.53670197981435));
#40509=CARTESIAN_POINT('Ctrl Pts',(-5.94189071380441,3.81612173192298,-9.54237324806219));
#40510=CARTESIAN_POINT('Ctrl Pts',(-5.93882920492322,3.81206076166437,-9.54811985199363));
#40511=CARTESIAN_POINT('Ctrl Pts',(-5.93729845048262,3.81003027653507,-9.55099315395935));
#40512=CARTESIAN_POINT('Ctrl Pts',(-5.93573458786337,3.80800913398943,-9.55388528957284));
#40513=CARTESIAN_POINT('Ctrl Pts',(-5.93413726119774,3.8059983378373,-9.5567958628498));
#40514=CARTESIAN_POINT('Ctrl Pts',(-5.93307815099486,3.80466507597769,-9.5587257234852));
#40515=CARTESIAN_POINT('Ctrl Pts',(-5.93173234157703,3.80300231282774,-9.56115325118467));
#40516=CARTESIAN_POINT('Ctrl Pts',(-5.93063879374801,3.80167632426087,-9.563104569513));
#40517=CARTESIAN_POINT('Ctrl Pts',(-5.93008307684265,3.80100248609542,-9.5640961864812));
#40518=CARTESIAN_POINT('Ctrl Pts',(-5.92959342566296,3.80041492290089,-9.56496479343206));
#40519=CARTESIAN_POINT('Ctrl Pts',(-5.92924452537267,3.79999801751792,-9.56558248670613));
#40520=CARTESIAN_POINT('Ctrl Pts',(-5.92334532745876,3.79294899109437,-9.57602643007663));
#40521=CARTESIAN_POINT('Ctrl Pts',(-5.91666160167339,3.78561043952302,-9.58734919508044));
#40522=CARTESIAN_POINT('Ctrl Pts',(-5.90905328822459,3.77814425919953,-9.59952402406024));
#40523=CARTESIAN_POINT('Ctrl Pts',(-5.9080903040565,3.7771992648199,-9.60106499206));
#40524=CARTESIAN_POINT('Ctrl Pts',(-5.90711249699386,3.7762522872061,-9.60261958067031));
#40525=CARTESIAN_POINT('Ctrl Pts',(-5.90611957387601,3.77530371017949,-9.60418770868075));
#40526=CARTESIAN_POINT('Ctrl Pts',(-5.89855598182255,3.76807792448518,-9.6161329241212));
#40527=CARTESIAN_POINT('Ctrl Pts',(-5.89011475648501,3.76075622121118,-9.62886574624393));
#40528=CARTESIAN_POINT('Ctrl Pts',(-5.88068114333654,3.75351428035395,-9.64233988204093));
#40529=CARTESIAN_POINT('Ctrl Pts',(-5.87365864584871,3.74812329063701,-9.65237019421252));
#40530=CARTESIAN_POINT('Ctrl Pts',(-5.8660862667034,3.74277711608668,-9.66281092509877));
#40531=CARTESIAN_POINT('Ctrl Pts',(-5.85791979596359,3.7375640109276,-9.67363288992283));
#40532=CARTESIAN_POINT('Ctrl Pts',(-5.84746904137633,3.73089272238804,-9.68748191995446));
#40533=CARTESIAN_POINT('Ctrl Pts',(-5.83604469511993,3.72443720624922,-9.70195661253992));
#40534=CARTESIAN_POINT('Ctrl Pts',(-5.82356408767723,3.71842356605161,-9.71696952444098));
#40535=CARTESIAN_POINT('Ctrl Pts',(-5.81185652587554,3.71278240919366,-9.7310525404089));
#40536=CARTESIAN_POINT('Ctrl Pts',(-5.79921851722962,3.7075311182103,-9.74560902264382));
#40537=CARTESIAN_POINT('Ctrl Pts',(-5.78561697672598,3.70286691787578,-9.76054504582999));
#40538=CARTESIAN_POINT('Ctrl Pts',(-5.77289240786099,3.69850344608074,-9.77451805539834));
#40539=CARTESIAN_POINT('Ctrl Pts',(-5.75932443077255,3.69465358063561,-9.78882332260751));
#40540=CARTESIAN_POINT('Ctrl Pts',(-5.74490786027132,3.69151076355338,-9.80335875951711));
#40541=CARTESIAN_POINT('Ctrl Pts',(-5.74093131861722,3.69064387617281,-9.80736808824939));
#40542=CARTESIAN_POINT('Ctrl Pts',(-5.73689035526843,3.68983099223883,-9.81139476874628));
#40543=CARTESIAN_POINT('Ctrl Pts',(-5.73278520331761,3.68907667806357,-9.81543627503468));
#40544=CARTESIAN_POINT('Ctrl Pts',(-5.71725897249954,3.60560105360399,-9.29487899241727));
#40545=CARTESIAN_POINT('Ctrl Pts',(-5.71831455425541,3.65953286909643,-9.72607755489095));
#40546=CARTESIAN_POINT('Ctrl Pts',(-5.72040614738814,3.838411285377,-10.6678342160512));
#40547=CARTESIAN_POINT('Ctrl Pts',(-5.72308282462462,4.31359609435923,-12.0712148773345));
#40548=CARTESIAN_POINT('Ctrl Pts',(-5.72473060493935,5.03571368099359,-13.4633017408292));
#40549=CARTESIAN_POINT('Ctrl Pts',(-5.72548235451857,5.95934088934631,-14.7303911815181));
#40550=CARTESIAN_POINT('Ctrl Pts',(-5.72532244465371,7.06378884116024,-15.8436279992245));
#40551=CARTESIAN_POINT('Ctrl Pts',(-5.72405830482639,8.29086173581263,-16.7525703081706));
#40552=CARTESIAN_POINT('Ctrl Pts',(-5.72276278486364,9.17588634241873,-17.2270158545483));
#40553=CARTESIAN_POINT('Ctrl Pts',(-5.7220418682695,9.61344013988758,-17.4236767878015));
#40554=CARTESIAN_POINT('Ctrl Pts',(-5.8959561156602,3.65997454462387,-9.28812061696448));
#40555=CARTESIAN_POINT('Ctrl Pts',(-5.89686256011918,3.71411017760644,-9.71695579985479));
#40556=CARTESIAN_POINT('Ctrl Pts',(-5.89864683886563,3.89299890606486,-10.6534764015069));
#40557=CARTESIAN_POINT('Ctrl Pts',(-5.90092445355812,4.36674183318056,-12.0486567166572));
#40558=CARTESIAN_POINT('Ctrl Pts',(-5.90232009808801,5.0854978237521,-13.4325649000885));
#40559=CARTESIAN_POINT('Ctrl Pts',(-5.90295604583695,6.00413540577092,-14.6922077788471));
#40560=CARTESIAN_POINT('Ctrl Pts',(-5.9028207928619,7.10226023811067,-15.799178922291));
#40561=CARTESIAN_POINT('Ctrl Pts',(-5.90175128485163,8.32198322005073,-16.7034195001779));
#40562=CARTESIAN_POINT('Ctrl Pts',(-5.90065109597932,9.20180506054372,-17.175772271617));
#40563=CARTESIAN_POINT('Ctrl Pts',(-5.90003815923874,9.63679110521912,-17.3716501036199));
#40564=CARTESIAN_POINT('Ctrl Pts',(-6.00511200699231,3.81066937852945,-9.26938986800578));
#40565=CARTESIAN_POINT('Ctrl Pts',(-6.0056009722777,3.86431168765211,-9.69180636116294));
#40566=CARTESIAN_POINT('Ctrl Pts',(-6.0065486299692,4.04116833572064,-10.6143641034697));
#40567=CARTESIAN_POINT('Ctrl Pts',(-6.00775098846849,4.50854425402217,-11.9883460169313));
#40568=CARTESIAN_POINT('Ctrl Pts',(-6.00847954447436,5.21698070534443,-13.3513219104762));
#40569=CARTESIAN_POINT('Ctrl Pts',(-6.00881053804551,6.12190713121469,-14.5917956565363));
#40570=CARTESIAN_POINT('Ctrl Pts',(-6.00874017300846,7.20354417012326,-15.6822130904412));
#40571=CARTESIAN_POINT('Ctrl Pts',(-6.00818339521858,8.40460620805652,-16.5730769807682));
#40572=CARTESIAN_POINT('Ctrl Pts',(-6.00760537290816,9.27115183997566,-17.0387401214206));
#40573=CARTESIAN_POINT('Ctrl Pts',(-6.00728243546019,9.69952680962233,-17.2318730621056));
#40574=CARTESIAN_POINT('Ctrl Pts',(-5.9998408175774,3.99628885031533,-9.24631810374516));
#40575=CARTESIAN_POINT('Ctrl Pts',(-5.99981404844536,4.04894055408171,-9.66087586636771));
#40576=CARTESIAN_POINT('Ctrl Pts',(-5.99973665412961,4.22254844296643,-10.5664333418028));
#40577=CARTESIAN_POINT('Ctrl Pts',(-5.99962568094289,4.68122376165327,-11.9148571729911));
#40578=CARTESIAN_POINT('Ctrl Pts',(-5.99954401753405,5.37658608631832,-13.2526773418967));
#40579=CARTESIAN_POINT('Ctrl Pts',(-5.9995051673635,6.26466620718276,-14.4700709223921));
#40580=CARTESIAN_POINT('Ctrl Pts',(-5.99951348071399,7.32636941191874,-15.540391859643));
#40581=CARTESIAN_POINT('Ctrl Pts',(-5.99957860435503,8.5050642212501,-16.4146537204691));
#40582=CARTESIAN_POINT('Ctrl Pts',(-5.99963682031295,9.35567047233198,-16.8717549394652));
#40583=CARTESIAN_POINT('Ctrl Pts',(-5.99966773898728,9.77608509663727,-17.0612989188918));
#40584=CARTESIAN_POINT('',(-5.99999997114735,9.67863337142275,-17.0348538902779));
#40585=CARTESIAN_POINT('Ctrl Pts',(-6.,3.99788652645587,-9.34661203134569));
#40586=CARTESIAN_POINT('Ctrl Pts',(-6.,4.06147282871,-9.81908885364613));
#40587=CARTESIAN_POINT('Ctrl Pts',(-6.,4.15795093339124,-10.2819181268309));
#40588=CARTESIAN_POINT('Ctrl Pts',(-6.,4.28772381294125,-10.7378299097621));
#40589=CARTESIAN_POINT('Ctrl Pts',(-6.,4.41749669249136,-11.1937416926937));
#40590=CARTESIAN_POINT('Ctrl Pts',(-6.,4.5805643469103,-11.6427359853717));
#40591=CARTESIAN_POINT('Ctrl Pts',(-6.,4.77466779593315,-12.0768287139941));
#40592=CARTESIAN_POINT('Ctrl Pts',(-6.,4.96877124495587,-12.5109214426161));
#40593=CARTESIAN_POINT('Ctrl Pts',(-6.,5.19391048858245,-12.9301126071823));
#40594=CARTESIAN_POINT('Ctrl Pts',(-6.,5.44842673883702,-13.3317963333689));
#40595=CARTESIAN_POINT('Ctrl Pts',(-6.,5.70294298909176,-13.7334800595558));
#40596=CARTESIAN_POINT('Ctrl Pts',(-6.,5.98683624597452,-14.1176563473629));
#40597=CARTESIAN_POINT('Ctrl Pts',(-6.,6.29607553925051,-14.4788351908868));
#40598=CARTESIAN_POINT('Ctrl Pts',(-6.,6.60531483252628,-14.8400140344105));
#40599=CARTESIAN_POINT('Ctrl Pts',(-6.,6.93990016219523,-15.1781954336509));
#40600=CARTESIAN_POINT('Ctrl Pts',(-6.,7.29796328415509,-15.49122228417));
#40601=CARTESIAN_POINT('Ctrl Pts',(-6.,7.6560264061152,-15.8042491346892));
#40602=CARTESIAN_POINT('Ctrl Pts',(-6.,8.03756732036623,-16.092121436487));
#40603=CARTESIAN_POINT('Ctrl Pts',(-6.,8.43516135621591,-16.3499544612483));
#40604=CARTESIAN_POINT('Ctrl Pts',(-6.,8.83275511078938,-16.6077873036066));
#40605=CARTESIAN_POINT('Ctrl Pts',(-6.,9.24640196424807,-16.8355809114308));
#40606=CARTESIAN_POINT('Ctrl Pts',(-6.,9.67863396563729,-17.0348526013916));
#40607=CARTESIAN_POINT('',(-5.736443569433,9.52121843706297,-17.3763278265689));
#40608=CARTESIAN_POINT('Origin',(-5.59998163814024,9.67863859077867,-17.0348433699263));
#40609=CARTESIAN_POINT('Ctrl Pts',(-5.73278790982,3.68906911002063,-9.81543761164561));
#40610=CARTESIAN_POINT('Ctrl Pts',(-5.73461480971437,3.83284536504953,-10.625338532278));
#40611=CARTESIAN_POINT('Ctrl Pts',(-5.73605973940222,4.07387518415476,-11.4195438253679));
#40612=CARTESIAN_POINT('Ctrl Pts',(-5.73818934991407,4.74008576935209,-12.9297554454633));
#40613=CARTESIAN_POINT('Ctrl Pts',(-5.73887403073807,5.16463847589479,-13.645990507428));
#40614=CARTESIAN_POINT('Ctrl Pts',(-5.73948314352221,6.17415914950061,-14.9577795832333));
#40615=CARTESIAN_POINT('Ctrl Pts',(-5.73940757548236,6.75884789279361,-15.5535353420817));
#40616=CARTESIAN_POINT('Ctrl Pts',(-5.7384961905792,8.05516229836731,-16.5887322234374));
#40617=CARTESIAN_POINT('Ctrl Pts',(-5.73766037378333,8.76684603319029,-17.0280903649815));
#40618=CARTESIAN_POINT('Ctrl Pts',(-5.73644356975675,9.52121823635002,-17.3763277339147));
#40619=CARTESIAN_POINT('Origin',(-5.599999999997,9.67863108576248,-17.0348569102134));
#40620=CARTESIAN_POINT('',(-5.593361696257,9.87744142979155,-17.381887715825));
#40621=CARTESIAN_POINT('Origin',(-5.599999999997,9.67863108576248,-17.0348569102134));
#40622=CARTESIAN_POINT('Origin',(-5.6,9.67863108578652,-17.0348569102573));
#40623=CARTESIAN_POINT('Ctrl Pts',(-5.59335880963397,9.87743876208659,-17.3818891889333));
#40624=CARTESIAN_POINT('Ctrl Pts',(-5.59335897597999,9.88085962292803,-17.3799294167645));
#40625=CARTESIAN_POINT('Ctrl Pts',(-5.59336249921671,9.95658496857357,-17.3365326542547));
#40626=CARTESIAN_POINT('Ctrl Pts',(-5.59336249921671,10.0355852075694,-17.2909218450052));
#40627=CARTESIAN_POINT('Ctrl Pts',(-5.59335897598,10.111030579166,-17.2470401532232));
#40628=CARTESIAN_POINT('Ctrl Pts',(-5.59335880963398,10.1144382220706,-17.2450574869161));
#40629=CARTESIAN_POINT('Ctrl Pts',(-5.83074004396025,9.87939819740572,-17.3853094563155));
#40630=CARTESIAN_POINT('Ctrl Pts',(-5.83074021194161,9.88281933951928,-17.3833494092223));
#40631=CARTESIAN_POINT('Ctrl Pts',(-5.83074376981389,9.95855095781735,-17.3399466417504));
#40632=CARTESIAN_POINT('Ctrl Pts',(-5.83074376981389,10.037558812847,-17.2943314353818));
#40633=CARTESIAN_POINT('Ctrl Pts',(-5.83074021194162,10.1130125212196,-17.2504473138044));
#40634=CARTESIAN_POINT('Ctrl Pts',(-5.83074004396027,10.1164205428518,-17.2484645413707));
#40635=CARTESIAN_POINT('Ctrl Pts',(-6.00000347484088,9.79664251978775,-17.2408563365192));
#40636=CARTESIAN_POINT('Ctrl Pts',(-6.00000357357708,9.800049674696,-17.2389042214154));
#40637=CARTESIAN_POINT('Ctrl Pts',(-6.00000566482435,9.87547170312966,-17.1956771557313));
#40638=CARTESIAN_POINT('Ctrl Pts',(-6.00000566482435,9.95415740030959,-17.1502479472839));
#40639=CARTESIAN_POINT('Ctrl Pts',(-6.00000357357708,10.0293041515383,-17.1065440874999));
#40640=CARTESIAN_POINT('Ctrl Pts',(-6.00000347484088,10.0326983102635,-17.1045694623467));
#40641=CARTESIAN_POINT('Ctrl Pts',(-5.9999999999769,9.67862555753756,-17.0348533301202));
#40642=CARTESIAN_POINT('Ctrl Pts',(-5.99999999996752,9.68201281535372,-17.0329126138548));
#40643=CARTESIAN_POINT('Ctrl Pts',(-5.99999999976693,9.75699439869606,-16.9899379593609));
#40644=CARTESIAN_POINT('Ctrl Pts',(-5.99999999976693,9.83522068191858,-16.9447739936855));
#40645=CARTESIAN_POINT('Ctrl Pts',(-5.99999999996752,9.90992861609885,-16.9013253649444));
#40646=CARTESIAN_POINT('Ctrl Pts',(-5.9999999999769,9.91330295459431,-16.8993622717592));
#40647=CARTESIAN_POINT('Origin',(-5.47625714583714,-8.61393265067164,14.9197686319482));
#40648=CARTESIAN_POINT('Ctrl Pts',(-6.00000000001697,9.67863488297892,-17.0348530243128));
#40649=CARTESIAN_POINT('Ctrl Pts',(-6.00000000001004,9.6820198209521,-17.0329138284621));
#40650=CARTESIAN_POINT('Ctrl Pts',(-6.00000000000346,9.68540450272322,-17.0309741411835));
#40651=CARTESIAN_POINT('Ctrl Pts',(-5.9999999999973,9.68878892526243,-17.0290339620093));
#40652=CARTESIAN_POINT('Ctrl Pts',(-5.99999999993208,9.72458345046399,-17.0085141269286));
#40653=CARTESIAN_POINT('Ctrl Pts',(-5.99999999990817,9.76034897938042,-16.9879392663609));
#40654=CARTESIAN_POINT('Ctrl Pts',(-5.99999999990817,9.79608195797508,-16.9673088199789));
#40655=CARTESIAN_POINT('Ctrl Pts',(-5.99999999990817,9.83181480046151,-16.9466784521789));
#40656=CARTESIAN_POINT('Ctrl Pts',(-5.99999999993208,9.86751509308548,-16.9259924988652));
#40657=CARTESIAN_POINT('Ctrl Pts',(-5.9999999999973,9.90318155031143,-16.9052543226814));
#40658=CARTESIAN_POINT('Ctrl Pts',(-6.00000000000346,9.90655401254468,-16.9032934125881));
#40659=CARTESIAN_POINT('Ctrl Pts',(-6.00000000001004,9.90992617229324,-16.9013320355928));
#40660=CARTESIAN_POINT('Ctrl Pts',(-6.00000000001697,9.91329802845247,-16.8993701945575));
#40661=CARTESIAN_POINT('Ctrl Pts',(-5.67770424700723,9.69013290714839,-17.4901834495681));
#40662=CARTESIAN_POINT('Ctrl Pts',(-3.78513616467149,8.87579171292761,-17.9133901356215));
#40663=CARTESIAN_POINT('Ctrl Pts',(-2.06853043374644E-10,8.0559151625809,
-18.3263289253002));
#40664=CARTESIAN_POINT('Ctrl Pts',(3.78513616425752,8.87579171283821,-17.913390135667));
#40665=CARTESIAN_POINT('Ctrl Pts',(5.67770424638677,9.69013290687893,-17.4901834497026));
#40666=CARTESIAN_POINT('Ctrl Pts',(-5.67770424700723,9.88675274008847,-17.3789457438659));
#40667=CARTESIAN_POINT('Ctrl Pts',(-3.78513616467149,9.58462619244214,-17.5169198758068));
#40668=CARTESIAN_POINT('Ctrl Pts',(-2.06853045109368E-10,9.35278546520724,
-17.7857301779258));
#40669=CARTESIAN_POINT('Ctrl Pts',(3.78513616425752,9.58462619241777,-17.5169198758378));
#40670=CARTESIAN_POINT('Ctrl Pts',(5.67770424638677,9.88675273998615,-17.3789457439054));
#40671=CARTESIAN_POINT('Ctrl Pts',(-5.67770424700723,10.0824918035142,-17.2660281226572));
#40672=CARTESIAN_POINT('Ctrl Pts',(-3.78513616467149,10.2888806489686,-17.1108358236266));
#40673=CARTESIAN_POINT('Ctrl Pts',(-2.06853409401297E-10,10.576208809251,
-17.0878170844136));
#40674=CARTESIAN_POINT('Ctrl Pts',(3.78513616425752,10.2888806489984,-17.1108358236215));
#40675=CARTESIAN_POINT('Ctrl Pts',(5.67770424638677,10.0824918035797,-17.2660281226026));
#40676=CARTESIAN_POINT('Ctrl Pts',(-5.67770424700723,10.2772218172614,-17.1515046485292));
#40677=CARTESIAN_POINT('Ctrl Pts',(-3.78513616467149,10.9871582910923,-16.6959444169702));
#40678=CARTESIAN_POINT('Ctrl Pts',(-2.0685344062632E-10,11.7011732380177,
-16.2470303047039));
#40679=CARTESIAN_POINT('Ctrl Pts',(3.78513616425752,10.9871582911679,-16.6959444169159));
#40680=CARTESIAN_POINT('Ctrl Pts',(5.67770424638677,10.2772218174911,-17.1515046483743));
#40681=CARTESIAN_POINT('Ctrl Pts',(-5.5933616962572,9.8774414297856,-17.3818877158146));
#40682=CARTESIAN_POINT('Ctrl Pts',(-5.58011194449613,9.87199617872778,-17.3847537905975));
#40683=CARTESIAN_POINT('Ctrl Pts',(-5.56077715143487,9.86405587308934,-17.3889346813685));
#40684=CARTESIAN_POINT('Ctrl Pts',(-5.53532113652999,9.85368788323714,-17.3943993484187));
#40685=CARTESIAN_POINT('Ctrl Pts',(-5.50995410366162,9.84335613491194,-17.3998449136101));
#40686=CARTESIAN_POINT('Ctrl Pts',(-5.47850841230432,9.83061363966293,-17.4065654390655));
#40687=CARTESIAN_POINT('Ctrl Pts',(-5.440927579018,9.81556929477701,-17.4145088993808));
#40688=CARTESIAN_POINT('Ctrl Pts',(-5.41351892178665,9.80459707154005,-17.420302266956));
#40689=CARTESIAN_POINT('Ctrl Pts',(-5.38284643787845,9.79240132902821,-17.4267457139548));
#40690=CARTESIAN_POINT('Ctrl Pts',(-5.34888208855784,9.77903861936218,-17.4338110542043));
#40691=CARTESIAN_POINT('Ctrl Pts',(-5.30328372218514,9.76109869873152,-17.4432965288177));
#40692=CARTESIAN_POINT('Ctrl Pts',(-5.25175264298193,9.74105373926007,-17.4539038384112));
#40693=CARTESIAN_POINT('Ctrl Pts',(-5.19420651583573,9.71907748007655,-17.465544925654));
#40694=CARTESIAN_POINT('Ctrl Pts',(-5.15775181712237,9.70515581502086,-17.4729193980846));
#40695=CARTESIAN_POINT('Ctrl Pts',(-5.11888293091578,9.69045994364656,-17.4807082620169));
#40696=CARTESIAN_POINT('Ctrl Pts',(-5.0775760599003,9.67504302649964,-17.4888837519901));
#40697=CARTESIAN_POINT('Ctrl Pts',(-5.01428285603189,9.65142017499784,-17.5014107950915));
#40698=CARTESIAN_POINT('Ctrl Pts',(-4.94526616581234,9.62610223170551,-17.5148467864822));
#40699=CARTESIAN_POINT('Ctrl Pts',(-4.87042972055464,9.59931641119694,-17.5290729156207));
#40700=CARTESIAN_POINT('Ctrl Pts',(-4.84061386073117,9.58864457521129,-17.5347407993739));
#40701=CARTESIAN_POINT('Ctrl Pts',(-4.80987409122418,9.57774022043901,-17.5405338235698));
#40702=CARTESIAN_POINT('Ctrl Pts',(-4.77820388113395,9.56661968261119,-17.5464433139158));
#40703=CARTESIAN_POINT('Ctrl Pts',(-4.70106691667843,9.53953414927539,-17.5608366553389));
#40704=CARTESIAN_POINT('Ctrl Pts',(-4.61841080073076,9.51116306793432,-17.5759226414519));
#40705=CARTESIAN_POINT('Ctrl Pts',(-4.53013500070397,9.48177397814663,-17.5915598828748));
#40706=CARTESIAN_POINT('Ctrl Pts',(-4.50293141539754,9.47271726485856,-17.5963787463784));
#40707=CARTESIAN_POINT('Ctrl Pts',(-4.47519409959358,9.46356419349808,-17.6012497792823));
#40708=CARTESIAN_POINT('Ctrl Pts',(-4.44691998668231,9.45432346338256,-17.6061683461136));
#40709=CARTESIAN_POINT('Ctrl Pts',(-4.35781348566433,9.4252010951573,-17.6216693198041));
#40710=CARTESIAN_POINT('Ctrl Pts',(-4.26337571436441,9.39520473748902,-17.6376442626533));
#40711=CARTESIAN_POINT('Ctrl Pts',(-4.16350853538153,9.36463621112325,-17.6539330750319));
#40712=CARTESIAN_POINT('Ctrl Pts',(-4.13544286586689,9.35604553932027,-17.6585107193557));
#40713=CARTESIAN_POINT('Ctrl Pts',(-4.10694837447457,9.3474099522417,-17.6631130001808));
#40714=CARTESIAN_POINT('Ctrl Pts',(-4.07802284616762,9.3387368036049,-17.6677359985849));
#40715=CARTESIAN_POINT('Ctrl Pts',(-3.98966527509743,9.31224330834538,-17.681857673588));
#40716=CARTESIAN_POINT('Ctrl Pts',(-3.89728568477082,9.28539730969706,-17.6961737677151));
#40717=CARTESIAN_POINT('Ctrl Pts',(-3.80082222259122,9.25842603150079,-17.7105635640497));
#40718=CARTESIAN_POINT('Ctrl Pts',(-3.75631511471526,9.24598180068934,-17.7172028469792));
#40719=CARTESIAN_POINT('Ctrl Pts',(-3.71093864267729,9.23351127863602,-17.7238576120777));
#40720=CARTESIAN_POINT('Ctrl Pts',(-3.66468681174934,9.22103880866935,-17.7305148894988));
#40721=CARTESIAN_POINT('Ctrl Pts',(-3.6291388814236,9.21145279911104,-17.7356314963266));
#40722=CARTESIAN_POINT('Ctrl Pts',(-3.59307387138023,9.20186566495838,-17.7407495726304));
#40723=CARTESIAN_POINT('Ctrl Pts',(-3.55648921837644,9.19228894191619,-17.7458629834574));
#40724=CARTESIAN_POINT('Ctrl Pts',(-3.51439653036569,9.18127038680953,-17.7517462484041));
#40725=CARTESIAN_POINT('Ctrl Pts',(-3.47161588281534,9.1702654167767,-17.7576234419693));
#40726=CARTESIAN_POINT('Ctrl Pts',(-3.42814354335167,9.1592925882825,-17.7634846849554));
#40727=CARTESIAN_POINT('Ctrl Pts',(-3.40640737361983,9.1538061740354,-17.7664153064484));
#40728=CARTESIAN_POINT('Ctrl Pts',(-3.38449828090911,9.1483277950983,-17.7693419401528));
#40729=CARTESIAN_POINT('Ctrl Pts',(-3.36241579598645,9.14285982146657,-17.7722633232205));
#40730=CARTESIAN_POINT('Ctrl Pts',(-3.35137455352512,9.1401258346507,-17.7737240147544));
#40731=CARTESIAN_POINT('Ctrl Pts',(-3.34028996301079,9.13739444915452,-17.7751833936165));
#40732=CARTESIAN_POINT('Ctrl Pts',(-3.32916196703421,9.13466596612807,-17.776641299268));
#40733=CARTESIAN_POINT('Ctrl Pts',(-3.32359796904591,9.13330172461484,-17.7773702520937));
#40734=CARTESIAN_POINT('Ctrl Pts',(-3.31802311969206,9.1319382087186,-17.778098836616));
#40735=CARTESIAN_POINT('Ctrl Pts',(-3.31243741184863,9.13057545642724,-17.7788270325796));
#40736=CARTESIAN_POINT('Ctrl Pts',(-3.3068517040052,9.12921270413588,-17.7795552285433));
#40737=CARTESIAN_POINT('Ctrl Pts',(-3.30243415517163,9.12813691830816,-17.7801300933024));
#40738=CARTESIAN_POINT('Ctrl Pts',(-3.29564770574228,9.12648952845955,-17.7810104344809));
#40739=CARTESIAN_POINT('Ctrl Pts',(-3.26393770760084,9.11879202336772,-17.7851238692638));
#40740=CARTESIAN_POINT('Ctrl Pts',(-3.23232942717988,9.11123014550933,-17.7891654603057));
#40741=CARTESIAN_POINT('Ctrl Pts',(-3.20082427869682,9.10380211593025,-17.7931361187594));
#40742=CARTESIAN_POINT('Ctrl Pts',(-3.02528951599938,9.06241594661338,-17.8152591247753));
#40743=CARTESIAN_POINT('Ctrl Pts',(-2.85295938427949,9.02518586220078,-17.8351795195926));
#40744=CARTESIAN_POINT('Ctrl Pts',(-2.68407158453179,8.99178486883743,-17.8530663542106));
#40745=CARTESIAN_POINT('Ctrl Pts',(-2.50184039212567,8.95574494850426,-17.8723663818364));
#40746=CARTESIAN_POINT('Ctrl Pts',(-2.32361766415623,8.9241624222754,-17.8892991455982));
#40747=CARTESIAN_POINT('Ctrl Pts',(-2.14966969634919,8.89659677674154,-17.9040935676009));
#40748=CARTESIAN_POINT('Ctrl Pts',(-2.13682621314835,8.89456146175742,-17.9051859167261));
#40749=CARTESIAN_POINT('Ctrl Pts',(-2.12400601123722,8.89254804288692,-17.9062666104474));
#40750=CARTESIAN_POINT('Ctrl Pts',(-2.11120918688827,8.89055634176565,-17.9073357418195));
#40751=CARTESIAN_POINT('Ctrl Pts',(-1.93623842500656,8.86332384617726,-17.9219539569042));
#40752=CARTESIAN_POINT('Ctrl Pts',(-1.76564250964608,8.84015095694756,-17.9344106798837));
#40753=CARTESIAN_POINT('Ctrl Pts',(-1.59965452899343,8.82056074414114,-17.9449536053094));
#40754=CARTESIAN_POINT('Ctrl Pts',(-1.55746334879606,8.81558126191978,-17.9476334286599));
#40755=CARTESIAN_POINT('Ctrl Pts',(-1.51556961880659,8.81083328673493,-17.95018959672));
#40756=CARTESIAN_POINT('Ctrl Pts',(-1.47397664556802,8.8063090668019,-17.9526261566541));
#40757=CARTESIAN_POINT('Ctrl Pts',(-1.30951026857606,8.78841945701537,-17.9622607692697));
#40758=CARTESIAN_POINT('Ctrl Pts',(-1.14975024394602,8.77402676598206,-17.9700258867514));
#40759=CARTESIAN_POINT('Ctrl Pts',(-0.994879319579393,8.76263737856074,
-17.9761785830586));
#40760=CARTESIAN_POINT('Ctrl Pts',(-0.923028843571489,8.75735341121175,
-17.9790330514503));
#40761=CARTESIAN_POINT('Ctrl Pts',(-0.852229999824751,8.75271615434218,
-17.9815403518941));
#40762=CARTESIAN_POINT('Ctrl Pts',(-0.782497653221542,8.74867785693833,
-17.9837255207404));
#40763=CARTESIAN_POINT('Ctrl Pts',(-0.633185211092702,8.74003096526203,
-17.988404452582));
#40764=CARTESIAN_POINT('Ctrl Pts',(-0.48876513848955,8.73412787932249,-17.9916073647212));
#40765=CARTESIAN_POINT('Ctrl Pts',(-0.349359262933425,8.73049489884206,
-17.9935789001746));
#40766=CARTESIAN_POINT('Ctrl Pts',(-0.262262031653481,8.72822510540704,
-17.9948106651822));
#40767=CARTESIAN_POINT('Ctrl Pts',(-0.177121215541505,8.72684207671218,
-17.9955615210256));
#40768=CARTESIAN_POINT('Ctrl Pts',(-0.0939590014244084,8.72623675497946,
-17.9958885074368));
#40769=CARTESIAN_POINT('Ctrl Pts',(0.0408293133112234,8.72525565680773,
-17.9964184830725));
#40770=CARTESIAN_POINT('Ctrl Pts',(0.170418217022037,8.72631579691311,-17.9958363492441));
#40771=CARTESIAN_POINT('Ctrl Pts',(0.294737354709391,8.72898124266637,-17.9943858101474));
#40772=CARTESIAN_POINT('Ctrl Pts',(0.343121177597331,8.730018608736,-17.9938212741632));
#40773=CARTESIAN_POINT('Ctrl Pts',(0.390707155839702,8.73129949621115,-17.9931249665939));
#40774=CARTESIAN_POINT('Ctrl Pts',(0.437492444106394,8.73279961278336,-17.9923103622705));
#40775=CARTESIAN_POINT('Ctrl Pts',(0.473998627888868,8.73397014166774,-17.991674733075));
#40776=CARTESIAN_POINT('Ctrl Pts',(0.510017321629045,8.73527416507888,-17.990967068312));
#40777=CARTESIAN_POINT('Ctrl Pts',(0.545547455340001,8.7367004771479,-17.9901935606565));
#40778=CARTESIAN_POINT('Ctrl Pts',(0.575306016459619,8.73789509676928,-17.9895457028402));
#40779=CARTESIAN_POINT('Ctrl Pts',(0.604721856468692,8.73917550597213,-17.988851653594));
#40780=CARTESIAN_POINT('Ctrl Pts',(0.633794572981875,8.74053515190824,-17.9881150240992));
#40781=CARTESIAN_POINT('Ctrl Pts',(0.665686567166257,8.74202664721683,-17.987306961201));
#40782=CARTESIAN_POINT('Ctrl Pts',(0.697165584262103,8.74361348041315,-17.9864476655722));
#40783=CARTESIAN_POINT('Ctrl Pts',(0.728231308503099,8.74528723796721,-17.985541761664));
#40784=CARTESIAN_POINT('Ctrl Pts',(0.743764170623598,8.74612411674424,-17.9850888097099));
#40785=CARTESIAN_POINT('Ctrl Pts',(0.759193709529455,8.74698272644005,-17.984624205335));
#40786=CARTESIAN_POINT('Ctrl Pts',(0.774519880040027,8.74786203977384,-17.9841485121783));
#40787=CARTESIAN_POINT('Ctrl Pts',(0.782182965295312,8.74830169644073,-17.9839106656));
#40788=CARTESIAN_POINT('Ctrl Pts',(0.789820208451713,8.74874652900686,-17.983670046805));
#40789=CARTESIAN_POINT('Ctrl Pts',(0.797431605159051,8.74919640992754,-17.9834267256678));
#40790=CARTESIAN_POINT('Ctrl Pts',(0.805043001866389,8.74964629084823,-17.9831834045305));
#40791=CARTESIAN_POINT('Ctrl Pts',(0.814391076480518,8.7502084329586,-17.9828794075472));
#40792=CARTESIAN_POINT('Ctrl Pts',(0.820188251806143,8.75056107063619,-17.982688724792));
#40793=CARTESIAN_POINT('Ctrl Pts',(0.913106248232728,8.75621320027285,-17.9796324329662));
#40794=CARTESIAN_POINT('Ctrl Pts',(1.01092014190408,8.76311877591221,-17.9759012853841));
#40795=CARTESIAN_POINT('Ctrl Pts',(1.11357262060553,8.77158708174356,-17.971331569502));
#40796=CARTESIAN_POINT('Ctrl Pts',(1.22621187672514,8.78087924576631,-17.9663172785259));
#40797=CARTESIAN_POINT('Ctrl Pts',(1.34467778636123,8.79205294515384,-17.9602933731797));
#40798=CARTESIAN_POINT('Ctrl Pts',(1.46886551454821,8.80554585695815,-17.9530280626319));
#40799=CARTESIAN_POINT('Ctrl Pts',(1.5153544234466,8.81059684514194,-17.9503083385085));
#40800=CARTESIAN_POINT('Ctrl Pts',(1.56264480959407,8.81597318478322,-17.9474144792473));
#40801=CARTESIAN_POINT('Ctrl Pts',(1.61072987577884,8.82169907113468,-17.9443337255254));
#40802=CARTESIAN_POINT('Ctrl Pts',(1.74016701018894,8.83711222079,-17.9360408403276));
#40803=CARTESIAN_POINT('Ctrl Pts',(1.87536541077607,8.8550562939364,-17.9263946075971));
#40804=CARTESIAN_POINT('Ctrl Pts',(2.01616865939584,8.87601506459434,-17.9151402743103));
#40805=CARTESIAN_POINT('Ctrl Pts',(2.02947228666054,8.87799532908038,-17.9140769220323));
#40806=CARTESIAN_POINT('Ctrl Pts',(2.04282591751082,8.88000252588665,-17.9129992048174));
#40807=CARTESIAN_POINT('Ctrl Pts',(2.05622939953854,8.88203707503234,-17.9119069022469));
#40808=CARTESIAN_POINT('Ctrl Pts',(2.18612622307218,8.90175444927892,-17.9013210982043));
#40809=CARTESIAN_POINT('Ctrl Pts',(2.32070785844954,8.92403976017556,-17.8893658762888));
#40810=CARTESIAN_POINT('Ctrl Pts',(2.45982125553463,8.94927553327455,-17.8758403317894));
#40811=CARTESIAN_POINT('Ctrl Pts',(2.57753274685146,8.97062890791897,-17.8643956251885));
#40812=CARTESIAN_POINT('Ctrl Pts',(2.69848834972096,8.99409519305475,-17.8518263861054));
#40813=CARTESIAN_POINT('Ctrl Pts',(2.82257920276446,9.01990720279287,-17.8380107025425));
#40814=CARTESIAN_POINT('Ctrl Pts',(2.92927450828348,9.04210078271857,-17.8261317562499));
#40815=CARTESIAN_POINT('Ctrl Pts',(3.0382873664991,9.06602868485195,-17.8133312539005));
#40816=CARTESIAN_POINT('Ctrl Pts',(3.149539801541,9.09183746377786,-17.7995327346023));
#40817=CARTESIAN_POINT('Ctrl Pts',(3.24642781372313,9.11431392720122,-17.787515819149));
#40818=CARTESIAN_POINT('Ctrl Pts',(3.34501424878886,9.13821698171628,-17.77474193929));
#40819=CARTESIAN_POINT('Ctrl Pts',(3.44524276091874,9.1636416709327,-17.7611617882135));
#40820=CARTESIAN_POINT('Ctrl Pts',(3.44871466880745,9.16452238019579,-17.7606913728332));
#40821=CARTESIAN_POINT('Ctrl Pts',(3.45218854645181,9.1654049152036,-17.7602199900659));
#40822=CARTESIAN_POINT('Ctrl Pts',(3.45566439144633,9.16628927984497,-17.7597476379063));
#40823=CARTESIAN_POINT('Ctrl Pts',(3.53373654223191,9.18615329844753,-17.7491379734686));
#40824=CARTESIAN_POINT('Ctrl Pts',(3.61280142985509,9.20694044006577,-17.7380392030405));
#40825=CARTESIAN_POINT('Ctrl Pts',(3.69283061359466,9.22869446064501,-17.7264288224018));
#40826=CARTESIAN_POINT('Ctrl Pts',(3.69949261699861,9.23050536702162,-17.725462320037));
#40827=CARTESIAN_POINT('Ctrl Pts',(3.70616130265311,9.23232297332201,-17.7244922725653));
#40828=CARTESIAN_POINT('Ctrl Pts',(3.71283665319058,9.23414730455173,-17.7235186671645));
#40829=CARTESIAN_POINT('Ctrl Pts',(3.74625606261466,9.24328061851759,-17.7186444186405));
#40830=CARTESIAN_POINT('Ctrl Pts',(3.77984252556761,9.25258248776584,-17.7136809929659));
#40831=CARTESIAN_POINT('Ctrl Pts',(3.81359387701825,9.26205601500284,-17.7086268127341));
#40832=CARTESIAN_POINT('Ctrl Pts',(3.83384037984567,9.26773892213829,-17.7055949497137));
#40833=CARTESIAN_POINT('Ctrl Pts',(3.85414621761188,9.27348360048981,-17.7025304286917));
#40834=CARTESIAN_POINT('Ctrl Pts',(3.8745109209936,9.27929071539973,-17.6994329122567));
#40835=CARTESIAN_POINT('Ctrl Pts',(3.88469327268447,9.2821942728547,-17.6978841540392));
#40836=CARTESIAN_POINT('Ctrl Pts',(3.89489034077921,9.28511343945291,-17.6963271469753));
#40837=CARTESIAN_POINT('Ctrl Pts',(3.90510206547525,9.2880482981763,-17.6947618490399));
#40838=CARTESIAN_POINT('Ctrl Pts',(3.91020792782327,9.289515727538,-17.6939792000721));
#40839=CARTESIAN_POINT('Ctrl Pts',(3.91531745432161,9.29098707993123,-17.6931944783869));
#40840=CARTESIAN_POINT('Ctrl Pts',(3.92043063744515,9.29246236570345,-17.6924076787479));
#40841=CARTESIAN_POINT('Ctrl Pts',(3.92554382056869,9.29393765147567,-17.6916208791089));
#40842=CARTESIAN_POINT('Ctrl Pts',(3.93242661853467,9.29592838500546,-17.6905592143405));
#40843=CARTESIAN_POINT('Ctrl Pts',(3.93578114914916,9.29690003349812,-17.6900410407387));
#40844=CARTESIAN_POINT('Ctrl Pts',(3.94207838550102,9.2987240443397,-17.6890683080328));
#40845=CARTESIAN_POINT('Ctrl Pts',(3.94835838647121,9.30054739878747,-17.6880959557532));
#40846=CARTESIAN_POINT('Ctrl Pts',(3.95462116944837,9.30237003113425,-17.6871240188475));
#40847=CARTESIAN_POINT('Ctrl Pts',(4.02983425200072,9.32425898971077,-17.6754515130318));
#40848=CARTESIAN_POINT('Ctrl Pts',(4.1025639945611,9.34604295765425,-17.6638393840448));
#40849=CARTESIAN_POINT('Ctrl Pts',(4.17284111891252,9.36761359660687,-17.6523453170107));
#40850=CARTESIAN_POINT('Ctrl Pts',(4.24076842735754,9.38846299047454,-17.6412355705048));
#40851=CARTESIAN_POINT('Ctrl Pts',(4.30640441838942,9.40911317057249,-17.6302360787778));
#40852=CARTESIAN_POINT('Ctrl Pts',(4.36977697048984,9.42947505700555,-17.6193942607279));
#40853=CARTESIAN_POINT('Ctrl Pts',(4.43122693487369,9.44921920734554,-17.6088813602538));
#40854=CARTESIAN_POINT('Ctrl Pts',(4.49054873063997,9.46869236090643,-17.5985166775392));
#40855=CARTESIAN_POINT('Ctrl Pts',(4.5477674454098,9.48782062019841,-17.5883395360635));
#40856=CARTESIAN_POINT('Ctrl Pts',(4.60352144780265,9.50645922504345,-17.578422913985));
#40857=CARTESIAN_POINT('Ctrl Pts',(4.65727867302525,9.52477042143705,-17.5686843289927));
#40858=CARTESIAN_POINT('Ctrl Pts',(4.70906171444353,9.54269206233632,-17.5591568289019));
#40859=CARTESIAN_POINT('Ctrl Pts',(4.75987978164253,9.56027973441181,-17.5498068732679));
#40860=CARTESIAN_POINT('Ctrl Pts',(4.8087965634695,9.57749227523871,-17.5406601907414));
#40861=CARTESIAN_POINT('Ctrl Pts',(4.85583261242937,9.59427637097178,-17.5317450928251));
#40862=CARTESIAN_POINT('Ctrl Pts',(4.90207267825761,9.61077643228066,-17.5229808636088));
#40863=CARTESIAN_POINT('Ctrl Pts',(4.94649513038224,9.6268624611947,-17.5144404326597));
#40864=CARTESIAN_POINT('Ctrl Pts',(4.98911858191001,9.6424885761226,-17.5061481039024));
#40865=CARTESIAN_POINT('Ctrl Pts',(4.98947832141365,9.64262045964274,-17.5060781171199));
#40866=CARTESIAN_POINT('Ctrl Pts',(4.98983793276467,9.64275231042812,-17.5060081479946));
#40867=CARTESIAN_POINT('Ctrl Pts',(4.99019741597397,9.64288412845248,-17.5059381965404));
#40868=CARTESIAN_POINT('Ctrl Pts',(5.03326309494624,9.65867577761138,-17.4975580920137));
#40869=CARTESIAN_POINT('Ctrl Pts',(5.07448979202937,9.67399688545065,-17.4894318230365));
#40870=CARTESIAN_POINT('Ctrl Pts',(5.1138956704581,9.68880469390431,-17.4815819379706));
#40871=CARTESIAN_POINT('Ctrl Pts',(5.15370025521237,9.70376232687992,-17.4736526282362));
#40872=CARTESIAN_POINT('Ctrl Pts',(5.19164699321678,9.71819623298685,-17.4660053223283));
#40873=CARTESIAN_POINT('Ctrl Pts',(5.22775340220523,9.73206688375502,-17.4586607148637));
#40874=CARTESIAN_POINT('Ctrl Pts',(5.26453906456748,9.74619847673802,-17.4511779366548));
#40875=CARTESIAN_POINT('Ctrl Pts',(5.29941451023093,9.75974542755134,-17.444009355409));
#40876=CARTESIAN_POINT('Ctrl Pts',(5.33239691037664,9.77267052382948,-17.4371742321374));
#40877=CARTESIAN_POINT('Ctrl Pts',(5.3664114649273,9.78600009931467,-17.4301252098602));
#40878=CARTESIAN_POINT('Ctrl Pts',(5.3984126497053,9.79866828470103,-17.4234308497413));
#40879=CARTESIAN_POINT('Ctrl Pts',(5.42841772935895,9.81063913570891,-17.4171094389117));
#40880=CARTESIAN_POINT('Ctrl Pts',(5.45996541482443,9.82322542598741,-17.410463034941));
#40881=CARTESIAN_POINT('Ctrl Pts',(5.48930650010712,9.83504080994725,-17.4042289291992));
#40882=CARTESIAN_POINT('Ctrl Pts',(5.51645909150323,9.84604910464715,-17.3984250783859));
#40883=CARTESIAN_POINT('Ctrl Pts',(5.54440583240798,9.8573793661052,-17.3924514785713));
#40884=CARTESIAN_POINT('Ctrl Pts',(5.57003422426587,9.86785462335406,-17.3869336679418));
#40885=CARTESIAN_POINT('Ctrl Pts',(5.59336166006701,9.87744149966146,-17.3818876748619));
#40886=CARTESIAN_POINT('Ctrl Pts',(-5.84637331455752,9.55547474172696,-17.3476041564549));
#40887=CARTESIAN_POINT('Ctrl Pts',(-5.81071185191775,9.54063160033165,-17.3552733651954));
#40888=CARTESIAN_POINT('Ctrl Pts',(-5.69191847149354,9.49167373167442,-17.3806024305499));
#40889=CARTESIAN_POINT('Ctrl Pts',(-5.48049361555364,9.40739237367748,-17.4243722057435));
#40890=CARTESIAN_POINT('Ctrl Pts',(-5.2021495036308,9.30184459029148,-17.479369066501));
#40891=CARTESIAN_POINT('Ctrl Pts',(-4.89414309097487,9.19156149103333,-17.536962878198));
#40892=CARTESIAN_POINT('Ctrl Pts',(-4.55276432929974,9.07723438519874,-17.5967675196366));
#40893=CARTESIAN_POINT('Ctrl Pts',(-4.17238112667691,8.95957671976703,-17.6583984118004));
#40894=CARTESIAN_POINT('Ctrl Pts',(-3.74657532026531,8.84000882077894,-17.721111142741));
#40895=CARTESIAN_POINT('Ctrl Pts',(-3.27004047448275,8.72141187442827,-17.7834030530746));
#40896=CARTESIAN_POINT('Ctrl Pts',(-2.73870586769555,8.60813163533864,-17.8430067909733));
#40897=CARTESIAN_POINT('Ctrl Pts',(-2.14779200690435,8.50556187107943,-17.897101921995));
#40898=CARTESIAN_POINT('Ctrl Pts',(-1.49669793916356,8.42117401415249,-17.9417588875659));
#40899=CARTESIAN_POINT('Ctrl Pts',(-0.805489886452122,8.36490960362597,
-17.971684220105));
#40900=CARTESIAN_POINT('Ctrl Pts',(-0.11337925692961,8.34312729743292,-17.9833787418543));
#40901=CARTESIAN_POINT('Ctrl Pts',(0.536146508488068,8.35364625772937,-17.977717202363));
#40902=CARTESIAN_POINT('Ctrl Pts',(1.11983353235545,8.38851236910003,-17.9591191164996));
#40903=CARTESIAN_POINT('Ctrl Pts',(1.63691904071335,8.4393404653141,-17.9321437229463));
#40904=CARTESIAN_POINT('Ctrl Pts',(2.09764269443844,8.50038183956579,-17.8998528831987));
#40905=CARTESIAN_POINT('Ctrl Pts',(2.51227845886102,8.56810417229776,-17.8641129073894));
#40906=CARTESIAN_POINT('Ctrl Pts',(2.88626565936715,8.63960400139166,-17.8264469425659));
#40907=CARTESIAN_POINT('Ctrl Pts',(3.2232840470072,8.71248864803032,-17.7881049412844));
#40908=CARTESIAN_POINT('Ctrl Pts',(3.52770199605896,8.78521869171782,-17.7498872415768));
#40909=CARTESIAN_POINT('Ctrl Pts',(3.80294640697365,8.85662163053349,-17.7124022350257));
#40910=CARTESIAN_POINT('Ctrl Pts',(4.05165902840887,8.92575523409715,-17.6761384257067));
#40911=CARTESIAN_POINT('Ctrl Pts',(4.27618401348504,8.99192944160887,-17.6414529589729));
#40912=CARTESIAN_POINT('Ctrl Pts',(4.47887700846266,9.05473894280456,-17.6085545575236));
#40913=CARTESIAN_POINT('Ctrl Pts',(4.66209438678431,9.11402294515649,-17.577524623232));
#40914=CARTESIAN_POINT('Ctrl Pts',(4.82815454959788,9.16981751996399,-17.5483421923328));
#40915=CARTESIAN_POINT('Ctrl Pts',(4.97929846125148,9.22230881982344,-17.5209084312054));
#40916=CARTESIAN_POINT('Ctrl Pts',(5.11759084189312,9.27176794816472,-17.4950807348835));
#40917=CARTESIAN_POINT('Ctrl Pts',(5.24463362120297,9.31841543321117,-17.4707435021366));
#40918=CARTESIAN_POINT('Ctrl Pts',(5.36151919418637,9.36236488162901,-17.4478372925747));
#40919=CARTESIAN_POINT('Ctrl Pts',(5.46894871897953,9.40363638206334,-17.4263514514219));
#40920=CARTESIAN_POINT('Ctrl Pts',(5.56756023616595,9.44226580283917,-17.406266900768));
#40921=CARTESIAN_POINT('Ctrl Pts',(5.6579973458819,9.47832606039999,-17.3875449759112));
#40922=CARTESIAN_POINT('Ctrl Pts',(5.74090606562001,9.51192223555312,-17.3701299000524));
#40923=CARTESIAN_POINT('Ctrl Pts',(5.80283958810511,9.53739134960786,-17.3569501787337));
#40924=CARTESIAN_POINT('Ctrl Pts',(5.83721149049653,9.55166218125863,-17.3495747889199));
#40925=CARTESIAN_POINT('Ctrl Pts',(5.8463475925958,9.55546502788484,-17.3476101108887));
#40926=CARTESIAN_POINT('Ctrl Pts',(-5.81214069693568,9.6776290300071,-17.4225528946938));
#40927=CARTESIAN_POINT('Ctrl Pts',(-5.77669403943401,9.66284974879393,-17.4302160824804));
#40928=CARTESIAN_POINT('Ctrl Pts',(-5.65860780706729,9.6140989355557,-17.4555273035572));
#40929=CARTESIAN_POINT('Ctrl Pts',(-5.44840103507682,9.53015694427974,-17.4992760054666));
#40930=CARTESIAN_POINT('Ctrl Pts',(-5.1716235662445,9.42501829450879,-17.5542570073678));
#40931=CARTESIAN_POINT('Ctrl Pts',(-4.86534001924691,9.31515643154803,-17.6118405916567));
#40932=CARTESIAN_POINT('Ctrl Pts',(-4.52587676502638,9.20126515974296,-17.6716387378284));
#40933=CARTESIAN_POINT('Ctrl Pts',(-4.14764618194598,9.08405852203899,-17.7332657288787));
#40934=CARTESIAN_POINT('Ctrl Pts',(-3.72427796798699,8.96495349815562,-17.7959764462078));
#40935=CARTESIAN_POINT('Ctrl Pts',(-3.25050693887968,8.8468213189703,-17.8582676328334));
#40936=CARTESIAN_POINT('Ctrl Pts',(-2.72229502793864,8.7339908807422,-17.9178712771889));
#40937=CARTESIAN_POINT('Ctrl Pts',(-2.13489630729917,8.63183353884197,-17.9719662105889));
#40938=CARTESIAN_POINT('Ctrl Pts',(-1.48771081717117,8.54778848442007,-18.0166222406388));
#40939=CARTESIAN_POINT('Ctrl Pts',(-0.800671855351995,8.49175380188948,
-18.0465458816406));
#40940=CARTESIAN_POINT('Ctrl Pts',(-0.112708541201747,8.47005970746182,
-18.0582390465695));
#40941=CARTESIAN_POINT('Ctrl Pts',(0.532949978621521,8.48053622101904,-18.0525782429442));
#40942=CARTESIAN_POINT('Ctrl Pts',(1.11311776538049,8.51526017793769,-18.0339815736975));
#40943=CARTESIAN_POINT('Ctrl Pts',(1.62709018905108,8.56588107546072,-18.0070072842141));
#40944=CARTESIAN_POINT('Ctrl Pts',(2.08504975370832,8.62667479118321,-17.9747170663004));
#40945=CARTESIAN_POINT('Ctrl Pts',(2.49721344229027,8.69412423447536,-17.9389773342653));
#40946=CARTESIAN_POINT('Ctrl Pts',(2.86898749461564,8.76533823308763,-17.9013114427223));
#40947=CARTESIAN_POINT('Ctrl Pts',(3.20402760911694,8.83793391897526,-17.8629695570604));
#40948=CARTESIAN_POINT('Ctrl Pts',(3.50667332561844,8.91037796332439,-17.8247521929843));
#40949=CARTESIAN_POINT('Ctrl Pts',(3.78032819766911,8.98150228244581,-17.7872678757862));
#40950=CARTESIAN_POINT('Ctrl Pts',(4.02761533238891,9.05036799932828,-17.7510052017049));
#40951=CARTESIAN_POINT('Ctrl Pts',(4.25086223368234,9.11628731866267,-17.7163213743395));
#40952=CARTESIAN_POINT('Ctrl Pts',(4.45240821357209,9.17885604156746,-17.6834251529964));
#40953=CARTESIAN_POINT('Ctrl Pts',(4.63459373937968,9.23791353477718,-17.6523979671745));
#40954=CARTESIAN_POINT('Ctrl Pts',(4.79972194542439,9.29349528775297,-17.6232188834924));
#40955=CARTESIAN_POINT('Ctrl Pts',(4.95001934007057,9.34578631988376,-17.5957891117641));
#40956=CARTESIAN_POINT('Ctrl Pts',(5.08753747324296,9.39505629485978,-17.5699661113688));
#40957=CARTESIAN_POINT('Ctrl Pts',(5.21386790054559,9.4415244999522,-17.5456343620477));
#40958=CARTESIAN_POINT('Ctrl Pts',(5.33009563895032,9.48530371309719,-17.5227345087097));
#40959=CARTESIAN_POINT('Ctrl Pts',(5.43691681896545,9.52641357738842,-17.5012559687883));
#40960=CARTESIAN_POINT('Ctrl Pts',(5.53496502099396,9.5648895099918,-17.4811797200827));
#40961=CARTESIAN_POINT('Ctrl Pts',(5.62487964845031,9.600803928118,-17.4624671215404));
#40962=CARTESIAN_POINT('Ctrl Pts',(5.70730293164213,9.63426144409487,-17.4450623578241));
#40963=CARTESIAN_POINT('Ctrl Pts',(5.76886861607727,9.65962318953327,-17.4318917174653));
#40964=CARTESIAN_POINT('Ctrl Pts',(5.80303452985547,9.67383305507474,-17.4245218566629));
#40965=CARTESIAN_POINT('Ctrl Pts',(5.81211577346237,9.67761960876587,-17.422558677682));
#40966=CARTESIAN_POINT('Ctrl Pts',(-5.75637685509934,9.8140410329922,-17.4252871788604));
#40967=CARTESIAN_POINT('Ctrl Pts',(-5.72124236127017,9.7993897878127,-17.4329279894493));
#40968=CARTESIAN_POINT('Ctrl Pts',(-5.60419107359204,9.75105931185798,-17.4581666988706));
#40969=CARTESIAN_POINT('Ctrl Pts',(-5.39580527606125,9.66783272587568,-17.5017964291619));
#40970=CARTESIAN_POINT('Ctrl Pts',(-5.12142095100228,9.56358874197378,-17.5566334095007));
#40971=CARTESIAN_POINT('Ctrl Pts',(-4.81781048341173,9.45467084686905,-17.6140674917309));
#40972=CARTESIAN_POINT('Ctrl Pts',(-4.48135661765004,9.34177398380753,-17.6737092386581));
#40973=CARTESIAN_POINT('Ctrl Pts',(-4.10654539124082,9.22561137506256,-17.7351721601088));
#40974=CARTESIAN_POINT('Ctrl Pts',(-3.68708984653772,9.10759142874642,-17.7977117189014));
#40975=CARTESIAN_POINT('Ctrl Pts',(-3.2178010218237,8.99056153156208,-17.8598276396926));
#40976=CARTESIAN_POINT('Ctrl Pts',(-2.69470548472169,8.87880960914205,-17.9192576327495));
#40977=CARTESIAN_POINT('Ctrl Pts',(-2.11312431732625,8.77765127324428,-17.9731888284785));
#40978=CARTESIAN_POINT('Ctrl Pts',(-1.47247131244265,8.69444440361395,-18.0177040810838));
#40979=CARTESIAN_POINT('Ctrl Pts',(-0.79246216940496,8.63897622205117,-18.0475294251907));
#40980=CARTESIAN_POINT('Ctrl Pts',(-0.111558320839529,8.61750183103525,
-18.059182549587));
#40981=CARTESIAN_POINT('Ctrl Pts',(0.52749191852145,8.6278723666929,-18.0535412908526));
#40982=CARTESIAN_POINT('Ctrl Pts',(1.10170577775085,8.66224461984375,-18.0350066389497));
#40983=CARTESIAN_POINT('Ctrl Pts',(1.61044334327689,8.71235628289372,-18.0081195170544));
#40984=CARTESIAN_POINT('Ctrl Pts',(2.06378679093631,8.77254508682486,-17.9759306394822));
#40985=CARTESIAN_POINT('Ctrl Pts',(2.4718495657996,8.83933224481332,-17.9402999855696));
#40986=CARTESIAN_POINT('Ctrl Pts',(2.83997682955784,8.90985712180265,-17.9027460783165));
#40987=CARTESIAN_POINT('Ctrl Pts',(3.17177856607899,8.98176081272291,-17.8645154707668));
#40988=CARTESIAN_POINT('Ctrl Pts',(3.47154177309266,9.05352460016479,-17.8264066164218));
#40989=CARTESIAN_POINT('Ctrl Pts',(3.74262739560875,9.12399074783355,-17.7890266501162));
#40990=CARTESIAN_POINT('Ctrl Pts',(3.98762439282825,9.19222800962803,-17.7528631841345));
#40991=CARTESIAN_POINT('Ctrl Pts',(4.20883005547312,9.25755353604305,-17.7182728316013));
#40992=CARTESIAN_POINT('Ctrl Pts',(4.40855467300355,9.3195653228394,-17.6854641626409));
#40993=CARTESIAN_POINT('Ctrl Pts',(4.58911102375203,9.37810272990502,-17.6545187345435));
#40994=CARTESIAN_POINT('Ctrl Pts',(4.7527761669793,9.43319958665139,-17.6254159783337));
#40995=CARTESIAN_POINT('Ctrl Pts',(4.90175235812833,9.48503807969688,-17.598057636747));
#40996=CARTESIAN_POINT('Ctrl Pts',(5.03806939881879,9.53388445863904,-17.5723017856496));
#40997=CARTESIAN_POINT('Ctrl Pts',(5.16330186304976,9.57995516360071,-17.5480334301608));
#40998=CARTESIAN_POINT('Ctrl Pts',(5.27852271290777,9.62336113040067,-17.5251935807664));
#40999=CARTESIAN_POINT('Ctrl Pts',(5.38441979560827,9.66412103109555,-17.5037718754277));
#41000=CARTESIAN_POINT('Ctrl Pts',(5.48161934164266,9.70226927265982,-17.4837495046991));
#41001=CARTESIAN_POINT('Ctrl Pts',(5.57075379922798,9.73787708217004,-17.4650880447167));
#41002=CARTESIAN_POINT('Ctrl Pts',(5.65245896154948,9.7710477993865,-17.4477318689615));
#41003=CARTESIAN_POINT('Ctrl Pts',(5.71348552357779,9.796191046643,-17.434598822889));
#41004=CARTESIAN_POINT('Ctrl Pts',(5.74735130046084,9.81027810305254,-17.4272502808467));
#41005=CARTESIAN_POINT('Ctrl Pts',(5.75635272233611,9.8140319128402,-17.4252927958575));
#41006=CARTESIAN_POINT('Ctrl Pts',(-5.69417743957803,9.92771327144431,-17.3549336348315));
#41007=CARTESIAN_POINT('Ctrl Pts',(-5.65936792101113,9.91321960471387,-17.3625417556048));
#41008=CARTESIAN_POINT('Ctrl Pts',(-5.54339907756701,9.86540905243201,-17.3876728669242));
#41009=CARTESIAN_POINT('Ctrl Pts',(-5.33694401269858,9.78308042667019,-17.4311178392296));
#41010=CARTESIAN_POINT('Ctrl Pts',(-5.06513131455385,9.67997470341483,-17.4857214910404));
#41011=CARTESIAN_POINT('Ctrl Pts',(-4.76442037050557,9.57226825687109,-17.5429071195401));
#41012=CARTESIAN_POINT('Ctrl Pts',(-4.43125498855782,9.46065550148003,-17.6022847388691));
#41013=CARTESIAN_POINT('Ctrl Pts',(-4.06020411559034,9.34584764235814,-17.663467660997));
#41014=CARTESIAN_POINT('Ctrl Pts',(-3.64507706599585,9.22924160764453,-17.7257130627828));
#41015=CARTESIAN_POINT('Ctrl Pts',(-3.18077544795952,9.11365349726097,-17.7875264269979));
#41016=CARTESIAN_POINT('Ctrl Pts',(-2.66340495859278,9.00331722991946,-17.8466560259837));
#41017=CARTESIAN_POINT('Ctrl Pts',(-2.08836900848276,8.90347441105333,-17.9003040865354));
#41018=CARTESIAN_POINT('Ctrl Pts',(-1.45510419309184,8.82137451837695,-17.9445766737933));
#41019=CARTESIAN_POINT('Ctrl Pts',(-0.783082843198929,8.76665646966238,
-17.9742336186812));
#41020=CARTESIAN_POINT('Ctrl Pts',(-0.110239903977575,8.7454738833116,-17.9858188158545));
#41021=CARTESIAN_POINT('Ctrl Pts',(0.521249582007313,8.75570355774493,-17.9802106405749));
#41022=CARTESIAN_POINT('Ctrl Pts',(1.08868634505104,8.78960963235603,-17.9617818848648));
#41023=CARTESIAN_POINT('Ctrl Pts',(1.59148420789597,8.83904768676422,-17.935044492473));
#41024=CARTESIAN_POINT('Ctrl Pts',(2.03960899817982,8.89843785453517,-17.9030303521735));
#41025=CARTESIAN_POINT('Ctrl Pts',(2.44305208407453,8.96435237350228,-17.8675882038322));
#41026=CARTESIAN_POINT('Ctrl Pts',(2.80708608283326,9.03397113821115,-17.8302280017904));
#41027=CARTESIAN_POINT('Ctrl Pts',(3.13526596976642,9.10496688075775,-17.7921898350716));
#41028=CARTESIAN_POINT('Ctrl Pts',(3.43181671015123,9.1758400646716,-17.7542684107075));
#41029=CARTESIAN_POINT('Ctrl Pts',(3.70004890813467,9.24544643262587,-17.7170683235269));
#41030=CARTESIAN_POINT('Ctrl Pts',(3.94251110847289,9.31286458365095,-17.6810753908391));
#41031=CARTESIAN_POINT('Ctrl Pts',(4.16146500019945,9.37741795690274,-17.646645145667));
#41032=CARTESIAN_POINT('Ctrl Pts',(4.35918701579828,9.43870723235016,-17.6139857940658));
#41033=CARTESIAN_POINT('Ctrl Pts',(4.53795795535941,9.49657159849751,-17.5831790868076));
#41034=CARTESIAN_POINT('Ctrl Pts',(4.70002505220228,9.55104259508925,-17.554205055054));
#41035=CARTESIAN_POINT('Ctrl Pts',(4.84756307655687,9.60229864215115,-17.5269663201844));
#41036=CARTESIAN_POINT('Ctrl Pts',(4.98257739074038,9.65060152385877,-17.501321960375));
#41037=CARTESIAN_POINT('Ctrl Pts',(5.10662357656201,9.69616399681796,-17.4771578087562));
#41038=CARTESIAN_POINT('Ctrl Pts',(5.22076112767138,9.7390946394701,-17.4544154229623));
#41039=CARTESIAN_POINT('Ctrl Pts',(5.32566859456254,9.77941088992731,-17.4330847501919));
#41040=CARTESIAN_POINT('Ctrl Pts',(5.42196395766287,9.81714585911028,-17.413147293363));
#41041=CARTESIAN_POINT('Ctrl Pts',(5.51027183420198,9.85236921482051,-17.3945649807498));
#41042=CARTESIAN_POINT('Ctrl Pts',(5.59122067258088,9.88518256407872,-17.3772825511604));
#41043=CARTESIAN_POINT('Ctrl Pts',(5.65168283897655,9.91005528387838,-17.3642054611152));
#41044=CARTESIAN_POINT('Ctrl Pts',(5.68523561929143,9.92399090717374,-17.3568882701779));
#41045=CARTESIAN_POINT('Ctrl Pts',(5.69415387512849,9.92770437916783,-17.3549391363549));
#41046=CARTESIAN_POINT('',(5.73644274980887,9.52121898128059,-17.3763264188351));
#41047=CARTESIAN_POINT('Origin',(5.599999999773,9.67863108544398,-17.0348569101664));
#41048=CARTESIAN_POINT('Ctrl Pts',(-5.73644387793582,9.52121721533315,-17.3763301032669));
#41049=CARTESIAN_POINT('Ctrl Pts',(-5.66411038342567,9.49169730160193,-17.3916242104899));
#41050=CARTESIAN_POINT('Ctrl Pts',(-5.58548129177106,9.46019526663674,-17.4079767022565));
#41051=CARTESIAN_POINT('Ctrl Pts',(-5.50055660135251,9.42702545331558,-17.4252224540635));
#41052=CARTESIAN_POINT('Ctrl Pts',(-5.41741954877212,9.39455385406014,-17.4421051882566));
#41053=CARTESIAN_POINT('Ctrl Pts',(-5.32824914863658,9.36048411499632,-17.4598438857157));
#41054=CARTESIAN_POINT('Ctrl Pts',(-5.23304539942654,9.32515773129678,-17.4782590784543));
#41055=CARTESIAN_POINT('Ctrl Pts',(-5.1347710008645,9.28869194985171,-17.4972682246886));
#41056=CARTESIAN_POINT('Ctrl Pts',(-5.03006778418147,9.25088688316903,-17.516998351475));
#41057=CARTESIAN_POINT('Ctrl Pts',(-4.91893574770631,9.21216969728679,-17.5372248895517));
#41058=CARTESIAN_POINT('Ctrl Pts',(-4.80780371123115,9.17345251140456,-17.5574514276284));
#41059=CARTESIAN_POINT('Ctrl Pts',(-4.69024285496385,9.13382320291011,-17.5781743787171));
#41060=CARTESIAN_POINT('Ctrl Pts',(-4.56625317723326,9.09376135229856,-17.5991415486935));
#41061=CARTESIAN_POINT('Ctrl Pts',(-4.44622761409869,9.05498033223404,-17.6194383704113));
#41062=CARTESIAN_POINT('Ctrl Pts',(-4.32017773615893,9.01579424100516,-17.6399639103149));
#41063=CARTESIAN_POINT('Ctrl Pts',(-4.18810354341397,8.97668495174031,-17.6604647153228));
#41064=CARTESIAN_POINT('Ctrl Pts',(-4.05161767055035,8.93626929315137,-17.6816503096298));
#41065=CARTESIAN_POINT('Ctrl Pts',(-3.90869830026241,8.89593536972225,-17.7028096379926));
#41066=CARTESIAN_POINT('Ctrl Pts',(-3.75934543255017,8.85626673446492,-17.7236357165823));
#41067=CARTESIAN_POINT('Ctrl Pts',(-3.60999256483792,8.81659809920759,-17.7444617951721));
#41068=CARTESIAN_POINT('Ctrl Pts',(-3.45420619970136,8.77759474677075,-17.7649546263512));
#41069=CARTESIAN_POINT('Ctrl Pts',(-3.29198633714049,8.73989291609286,-17.7847794700339));
#41070=CARTESIAN_POINT('Ctrl Pts',(-3.21175032065614,8.72124510897475,-17.7945850909943));
#41071=CARTESIAN_POINT('Ctrl Pts',(-3.1299404019154,8.70291652036431,-17.8042268665942));
#41072=CARTESIAN_POINT('Ctrl Pts',(-3.04655658560425,8.68498892402543,-17.8136617872421));
#41073=CARTESIAN_POINT('Ctrl Pts',(-3.00486467744867,8.67602512585599,-17.8183792475661));
#41074=CARTESIAN_POINT('Ctrl Pts',(-2.96277928617363,8.66716159628124,-17.8230449549843));
#41075=CARTESIAN_POINT('Ctrl Pts',(-2.92030042303628,8.65840888808932,-17.8276533930247));
#41076=CARTESIAN_POINT('Ctrl Pts',(-2.89906099146761,8.65403253399335,-17.8299576120449));
#41077=CARTESIAN_POINT('Ctrl Pts',(-2.87772319136642,8.64968388651658,-17.8322475112797));
#41078=CARTESIAN_POINT('Ctrl Pts',(-2.85628702258498,8.64536427823138,-17.8345223891241));
#41079=CARTESIAN_POINT('Ctrl Pts',(-2.84556893819426,8.64320447408879,-17.8356598280463));
#41080=CARTESIAN_POINT('Ctrl Pts',(-2.83482626160102,8.64105192982512,-17.836793511467));
#41081=CARTESIAN_POINT('Ctrl Pts',(-2.82405899279638,8.63890681319801,-17.8379233510875));
#41082=CARTESIAN_POINT('Ctrl Pts',(-2.81867535839406,8.63783425488446,-17.8384882708978));
#41083=CARTESIAN_POINT('Ctrl Pts',(-2.81328557593688,8.63676355348512,-17.8390522297484));
#41084=CARTESIAN_POINT('Ctrl Pts',(-2.80788964542488,8.63569473004595,-17.8396152165656));
#41085=CARTESIAN_POINT('Ctrl Pts',(-2.80249371491288,8.63462590660678,-17.8401782033829));
#41086=CARTESIAN_POINT('Ctrl Pts',(-2.79531868547233,8.63320981247684,-17.8409241382583));
#41087=CARTESIAN_POINT('Ctrl Pts',(-2.79168340972041,8.63249391468896,-17.8413012498115));
#41088=CARTESIAN_POINT('Ctrl Pts',(-2.04588093613951,8.48562243162411,-17.9186683461067));
#41089=CARTESIAN_POINT('Ctrl Pts',(-1.30009078784875,8.39776408503863,-17.9651455234455));
#41090=CARTESIAN_POINT('Ctrl Pts',(-0.554283333978138,8.36894043965146,
-17.9807044955084));
#41091=CARTESIAN_POINT('Ctrl Pts',(-0.369523434874257,8.36179991861496,
-17.9845589409065));
#41092=CARTESIAN_POINT('Ctrl Pts',(-0.184762473712586,8.35828264718359,
-17.986515842323));
#41093=CARTESIAN_POINT('Ctrl Pts',(-7.99360577730113E-13,8.35838942830133,
-17.9865746369497));
#41094=CARTESIAN_POINT('Ctrl Pts',(6.94550121454233E-5,8.35838946844197,
-17.9865746590515));
#41095=CARTESIAN_POINT('Ctrl Pts',(0.000138910025304622,8.35838950909474,
-17.9865746808851));
#41096=CARTESIAN_POINT('Ctrl Pts',(0.000208365038677248,8.35838955025963,
-17.9865747024504));
#41097=CARTESIAN_POINT('Ctrl Pts',(0.465533255570969,8.35866534097634,-17.9867191828595));
#41098=CARTESIAN_POINT('Ctrl Pts',(0.930858145081447,8.38166463295442,-17.9746778676881));
#41099=CARTESIAN_POINT('Ctrl Pts',(1.39618303357009,8.42737850509597,-17.9504583227467));
#41100=CARTESIAN_POINT('Ctrl Pts',(1.62884547781441,8.45023544116675,-17.9383485502759));
#41101=CARTESIAN_POINT('Ctrl Pts',(1.86150792191003,8.47877067136745,-17.9231942685957));
#41102=CARTESIAN_POINT('Ctrl Pts',(2.09417036449486,8.51298095415368,-17.9049967252316));
#41103=CARTESIAN_POINT('Ctrl Pts',(2.21050158578728,8.5300860955468,-17.8958979535495));
#41104=CARTESIAN_POINT('Ctrl Pts',(2.32683280861868,8.5486099938875,-17.8860383780086));
#41105=CARTESIAN_POINT('Ctrl Pts',(2.44316403066954,8.56855209163748,-17.8754181650244));
#41106=CARTESIAN_POINT('Ctrl Pts',(2.50132964169498,8.57852314051247,-17.8701080585323));
#41107=CARTESIAN_POINT('Ctrl Pts',(2.55949525262821,8.58884873884022,-17.8646077934184));
#41108=CARTESIAN_POINT('Ctrl Pts',(2.61766086348722,8.5995288113506,-17.8589173932483));
#41109=CARTESIAN_POINT('Ctrl Pts',(2.64674366891673,8.60486884760579,-17.8560721931632));
#41110=CARTESIAN_POINT('Ctrl Pts',(2.67582647433671,8.61029750238258,-17.8531794593596));
#41111=CARTESIAN_POINT('Ctrl Pts',(2.7049092797489,8.61581476573433,-17.8502391948578));
#41112=CARTESIAN_POINT('Ctrl Pts',(2.73217440982283,8.62098720012659,-17.8474826968874));
#41113=CARTESIAN_POINT('Ctrl Pts',(2.75943953989021,8.62623751314833,-17.8446844238911));
#41114=CARTESIAN_POINT('Ctrl Pts',(2.78670466995733,8.63156569635524,-17.8418443784168));
#41115=CARTESIAN_POINT('Ctrl Pts',(2.78852234529513,8.63192090856904,-17.8416550420518));
#41116=CARTESIAN_POINT('Ctrl Pts',(2.79172234575743,8.63254712883725,-17.8413212491149));
#41117=CARTESIAN_POINT('Ctrl Pts',(2.7921576959705,8.63263237126126,-17.8412758123555));
#41118=CARTESIAN_POINT('Ctrl Pts',(2.80635105401264,8.63541145855232,-17.839794475779));
#41119=CARTESIAN_POINT('Ctrl Pts',(2.82656971290414,8.63939945105124,-17.8376812591674));
#41120=CARTESIAN_POINT('Ctrl Pts',(2.85281367264499,8.64467374260481,-17.8348954844623));
#41121=CARTESIAN_POINT('Ctrl Pts',(2.87905792637246,8.64994809324134,-17.8321096785508));
#41122=CARTESIAN_POINT('Ctrl Pts',(2.9113276159417,8.65650877173247,-17.8286512992758));
#41123=CARTESIAN_POINT('Ctrl Pts',(2.9496227413527,8.66447932329167,-17.8244554218755));
#41124=CARTESIAN_POINT('Ctrl Pts',(2.9879183200816,8.67244996920214,-17.8202594948066));
#41125=CARTESIAN_POINT('Ctrl Pts',(3.03223947730509,8.68183052149572,-17.8153260518509));
#41126=CARTESIAN_POINT('Ctrl Pts',(3.08258621302318,8.69279067999899,-17.8095659239372));
#41127=CARTESIAN_POINT('Ctrl Pts',(3.13293393523487,8.70375105325554,-17.8038056831596));
#41128=CARTESIAN_POINT('Ctrl Pts',(3.18930747207375,8.7162910944596,-17.7972187246566));
#41129=CARTESIAN_POINT('Ctrl Pts',(3.25170682353982,8.7306266669751,-17.7896916363006));
#41130=CARTESIAN_POINT('Ctrl Pts',(3.31410687991243,8.7449624014352,-17.7821644629133));
#41131=CARTESIAN_POINT('Ctrl Pts',(3.3825328870566,8.76109370763203,-17.7736971379277));
#41132=CARTESIAN_POINT('Ctrl Pts',(3.45698484497233,8.77928261259938,-17.7641520138671));
#41133=CARTESIAN_POINT('Ctrl Pts',(3.53143822129211,8.79747186408838,-17.7546067079598));
#41134=CARTESIAN_POINT('Ctrl Pts',(3.61191777798963,8.81771879250422,-17.7439835613382));
#41135=CARTESIAN_POINT('Ctrl Pts',(3.69842351506488,8.84033160069405,-17.7321206943966));
#41136=CARTESIAN_POINT('Ctrl Pts',(3.77372180500989,8.86001475518896,-17.7217947481097));
#41137=CARTESIAN_POINT('Ctrl Pts',(3.85358595433381,8.88149117333469,-17.7105291312976));
#41138=CARTESIAN_POINT('Ctrl Pts',(3.93801596303663,8.90499259034002,-17.6982021477661));
#41139=CARTESIAN_POINT('Ctrl Pts',(3.98561503901163,8.91824197584575,-17.6912525686452));
#41140=CARTESIAN_POINT('Ctrl Pts',(4.0346653103836,8.93213545810003,-17.683965397655));
#41141=CARTESIAN_POINT('Ctrl Pts',(4.08516678273887,8.94671828866847,-17.6763168873926));
#41142=CARTESIAN_POINT('Ctrl Pts',(4.11041751891651,8.95400970395269,-17.6724926322615));
#41143=CARTESIAN_POINT('Ctrl Pts',(4.13603104579127,8.96147347239214,-17.6685780102973));
#41144=CARTESIAN_POINT('Ctrl Pts',(4.16200737546585,8.96911553234021,-17.6645699336875));
#41145=CARTESIAN_POINT('Ctrl Pts',(4.17499554030314,8.97293656231424,-17.6625658953826));
#41146=CARTESIAN_POINT('Ctrl Pts',(4.18807440525279,8.97680216617658,-17.6605384914099));
#41147=CARTESIAN_POINT('Ctrl Pts',(4.20124397016567,8.98071309740182,-17.6584873257955));
#41148=CARTESIAN_POINT('Ctrl Pts',(4.2078287526221,8.98266856301444,-17.6574617429884));
#41149=CARTESIAN_POINT('Ctrl Pts',(4.21443621003134,8.98463536053006,-17.6564302196462));
#41150=CARTESIAN_POINT('Ctrl Pts',(4.22106634239483,8.98661358516831,-17.6553927057802));
#41151=CARTESIAN_POINT('Ctrl Pts',(4.22769647475832,8.98859180980657,-17.6543551919142));
#41152=CARTESIAN_POINT('Ctrl Pts',(4.23593799439455,8.99105772534333,-17.65306190396));
#41153=CARTESIAN_POINT('Ctrl Pts',(4.24102476427196,8.99258263611854,-17.6522621422006));
#41154=CARTESIAN_POINT('Ctrl Pts',(4.37039571957259,9.03136543315713,-17.6319219370575));
#41155=CARTESIAN_POINT('Ctrl Pts',(4.49374081874749,9.070127787373,-17.6116087574268));
#41156=CARTESIAN_POINT('Ctrl Pts',(4.61106006309524,9.1083980751459,-17.5915706671761));
#41157=CARTESIAN_POINT('Ctrl Pts',(4.72934316492,9.14698277939176,-17.5713679503697));
#41158=CARTESIAN_POINT('Ctrl Pts',(4.84150099218696,9.185067237906,-17.5514448938586));
#41159=CARTESIAN_POINT('Ctrl Pts',(4.94753354622695,9.22221554440591,-17.5320307290879));
#41160=CARTESIAN_POINT('Ctrl Pts',(5.05275887907135,9.25908104247346,-17.5127643635043));
#41161=CARTESIAN_POINT('Ctrl Pts',(5.15195184655995,9.2950246503136,-17.4939991381214));
#41162=CARTESIAN_POINT('Ctrl Pts',(5.24511244999343,9.32966666640695,-17.4759346754223));
#41163=CARTESIAN_POINT('Ctrl Pts',(5.33934505593314,9.3647073094596,-17.4576623442834));
#41164=CARTESIAN_POINT('Ctrl Pts',(5.42740566978876,9.39841614503533,-17.4401070426611));
#41165=CARTESIAN_POINT('Ctrl Pts',(5.50929429290636,9.4304482037099,-17.4234500711274));
#41166=CARTESIAN_POINT('Ctrl Pts',(5.59118291602396,9.46248026238448,-17.4067930995937));
#41167=CARTESIAN_POINT('Ctrl Pts',(5.66689954840355,9.49283554612634,-17.3910344570249));
#41168=CARTESIAN_POINT('Ctrl Pts',(5.73644419139122,9.5212173172705,-17.3763300250116));
#41169=CARTESIAN_POINT('Origin',(5.6,9.67863108576213,-17.0348569102136));
#41170=CARTESIAN_POINT('Origin',(5.599974278086,9.67865015409865,-17.0348418886545));
#41171=CARTESIAN_POINT('Ctrl Pts',(5.71192057974457,3.68828900101138,-9.85023514350112));
#41172=CARTESIAN_POINT('Ctrl Pts',(5.71687909013046,3.68927746603566,-9.84789209427039));
#41173=CARTESIAN_POINT('Ctrl Pts',(5.76414655581842,3.69951923241957,-9.82520668560991));
#41174=CARTESIAN_POINT('Ctrl Pts',(5.84911010038005,3.73283091286591,-9.77805626709572));
#41175=CARTESIAN_POINT('Ctrl Pts',(5.94752938889343,3.81065413233525,-9.7065237214035));
#41176=CARTESIAN_POINT('Ctrl Pts',(6.01566971792523,3.90954242904105,-9.63753575219431));
#41177=CARTESIAN_POINT('Ctrl Pts',(6.04716489751294,4.00788517584066,-9.58296136794285));
#41178=CARTESIAN_POINT('Ctrl Pts',(6.05142143229536,4.0698892375096,-9.55471543074864));
#41179=CARTESIAN_POINT('Ctrl Pts',(6.0507700358332,4.09458285042653,-9.54441628184707));
#41180=CARTESIAN_POINT('Ctrl Pts',(5.59583289853465,3.61242448643793,-9.5665423944353));
#41181=CARTESIAN_POINT('Ctrl Pts',(5.60045925819736,3.61331789904416,-9.56436069032235));
#41182=CARTESIAN_POINT('Ctrl Pts',(5.64456722873301,3.62258540256811,-9.54323612999687));
#41183=CARTESIAN_POINT('Ctrl Pts',(5.7239592089636,3.65291740087055,-9.49930946581784));
#41184=CARTESIAN_POINT('Ctrl Pts',(5.81592915863889,3.72404613777338,-9.43278546471175));
#41185=CARTESIAN_POINT('Ctrl Pts',(5.87945135471979,3.81436258040131,-9.36894609262212));
#41186=CARTESIAN_POINT('Ctrl Pts',(5.90864330625533,3.90380035745063,-9.31890905716097));
#41187=CARTESIAN_POINT('Ctrl Pts',(5.91254704364485,3.95980194151539,-9.29334384463089));
#41188=CARTESIAN_POINT('Ctrl Pts',(5.91194908378594,3.98202534295877,-9.28408410725217));
#41189=CARTESIAN_POINT('Ctrl Pts',(5.5786770225829,3.33840156455887,-9.41055857489166));
#41190=CARTESIAN_POINT('Ctrl Pts',(5.58525591743157,3.33967221246092,-9.40750014613255));
#41191=CARTESIAN_POINT('Ctrl Pts',(5.64791910753711,3.35283604660006,-9.3779306843833));
#41192=CARTESIAN_POINT('Ctrl Pts',(5.75974886295832,3.39554420108066,-9.3172095505129));
#41193=CARTESIAN_POINT('Ctrl Pts',(5.88925468160274,3.49511101909614,-9.22577859145062));
#41194=CARTESIAN_POINT('Ctrl Pts',(5.98006530410807,3.6228200472589,-9.13695179587132));
#41195=CARTESIAN_POINT('Ctrl Pts',(6.02330455844228,3.75272356690769,-9.06502589944593));
#41196=CARTESIAN_POINT('Ctrl Pts',(6.02945981529473,3.83732356858628,-9.02648321068592));
#41197=CARTESIAN_POINT('Ctrl Pts',(6.02852200235225,3.871565851545,-9.01219518727837));
#41198=CARTESIAN_POINT('Ctrl Pts',(5.67169867046695,3.04584531044098,-9.48453249266367));
#41199=CARTESIAN_POINT('Ctrl Pts',(5.68123487669659,3.04771819915123,-9.48013397279952));
#41200=CARTESIAN_POINT('Ctrl Pts',(5.77200483704837,3.06709486655197,-9.43764959196145));
#41201=CARTESIAN_POINT('Ctrl Pts',(5.9330183650432,3.12942229883713,-9.35112473670729));
#41202=CARTESIAN_POINT('Ctrl Pts',(6.11944005804963,3.27391826346144,-9.22119812121329));
#41203=CARTESIAN_POINT('Ctrl Pts',(6.2515577828283,3.46047303546363,-9.09362743190567));
#41204=CARTESIAN_POINT('Ctrl Pts',(6.31598669919579,3.65368723849839,-8.98773487091865));
#41205=CARTESIAN_POINT('Ctrl Pts',(6.32552189499299,3.78273995333454,-8.92906339352892));
#41206=CARTESIAN_POINT('Ctrl Pts',(6.32407371695654,3.83561169243889,-8.90697548725414));
#41207=CARTESIAN_POINT('',(5.99998739574839,3.99788653423051,-9.34660672477245));
#41208=CARTESIAN_POINT('',(5.99999998791461,3.21424323425742,-9.29218306971572));
#41209=CARTESIAN_POINT('Ctrl Pts',(5.9999873957484,3.99788653423051,-9.34660672477246));
#41210=CARTESIAN_POINT('Ctrl Pts',(5.9999852507043,3.97568044757288,-9.33733089968698));
#41211=CARTESIAN_POINT('Ctrl Pts',(5.99998676083559,3.95337029535213,-9.328534099322));
#41212=CARTESIAN_POINT('Ctrl Pts',(5.99999979818264,3.93100830776541,-9.32032006028138));
#41213=CARTESIAN_POINT('Ctrl Pts',(6.00000674470619,3.91909345477917,-9.31594347849442));
#41214=CARTESIAN_POINT('Ctrl Pts',(6.00001622835211,3.90716442776862,-9.31173201822555));
#41215=CARTESIAN_POINT('Ctrl Pts',(6.00002591441227,3.89523282137244,-9.30769827794002));
#41216=CARTESIAN_POINT('Ctrl Pts',(6.00004505393926,3.87165612468503,-9.29972766039951));
#41217=CARTESIAN_POINT('Ctrl Pts',(6.00006657100939,3.84806757203079,-9.29245336782808));
#41218=CARTESIAN_POINT('Ctrl Pts',(6.00008776123526,3.82457051194069,-9.28593625304491));
#41219=CARTESIAN_POINT('Ctrl Pts',(6.00010095762279,3.8099375244107,-9.28187766618392));
#41220=CARTESIAN_POINT('Ctrl Pts',(6.00011344209019,3.79534069376842,-9.27811196626277));
#41221=CARTESIAN_POINT('Ctrl Pts',(6.00012222415269,3.78081005016456,-9.2746453820103));
#41222=CARTESIAN_POINT('Ctrl Pts',(6.0001366712745,3.75690610068274,-9.26894260262181));
#41223=CARTESIAN_POINT('Ctrl Pts',(6.00013999171371,3.73318089327534,-9.26405207526274));
#41224=CARTESIAN_POINT('Ctrl Pts',(6.00012429846304,3.70978124469432,-9.25996126528744));
#41225=CARTESIAN_POINT('Ctrl Pts',(6.00011929433188,3.70231976249024,-9.25865682237133));
#41226=CARTESIAN_POINT('Ctrl Pts',(6.0001124687567,3.69489145750722,-9.25743331593505));
#41227=CARTESIAN_POINT('Ctrl Pts',(6.00010395164358,3.68750121638747,-9.25628930568157));
#41228=CARTESIAN_POINT('Ctrl Pts',(6.00009904587385,3.68324451336532,-9.25563036751914));
#41229=CARTESIAN_POINT('Ctrl Pts',(6.00009358391438,3.6790004383084,-9.25499779435146));
#41230=CARTESIAN_POINT('Ctrl Pts',(6.00008768224772,3.67476986072246,-9.25439125254406));
#41231=CARTESIAN_POINT('Ctrl Pts',(6.00006914321531,3.66148025634672,-9.252485909717));
#41232=CARTESIAN_POINT('Ctrl Pts',(6.00005143457785,3.64814284857007,-9.25080653782235));
#41233=CARTESIAN_POINT('Ctrl Pts',(6.00003088539827,3.63498884507945,-9.24938653464367));
#41234=CARTESIAN_POINT('Ctrl Pts',(6.00001015026417,3.62171580780848,-9.24795368151047));
#41235=CARTESIAN_POINT('Ctrl Pts',(5.99998607093735,3.60863002122327,-9.24678503799945));
#41236=CARTESIAN_POINT('Ctrl Pts',(5.99996799233405,3.59598531542618,-9.24586523586959));
#41237=CARTESIAN_POINT('Ctrl Pts',(5.99995732843904,3.58852667423793,-9.24532267883735));
#41238=CARTESIAN_POINT('Ctrl Pts',(5.99994904811738,3.58122177219781,-9.24486573182062));
#41239=CARTESIAN_POINT('Ctrl Pts',(5.99994795245078,3.57412414233203,-9.24448341761151));
#41240=CARTESIAN_POINT('Ctrl Pts',(5.99994403955748,3.54877677088038,-9.24311808010406));
#41241=CARTESIAN_POINT('Ctrl Pts',(5.99996395296392,3.52334629616488,-9.24263149392783));
#41242=CARTESIAN_POINT('Ctrl Pts',(5.99998991135032,3.4979788568905,-9.24309866573729));
#41243=CARTESIAN_POINT('Ctrl Pts',(6.00001572107996,3.47275669017528,-9.2435631621784));
#41244=CARTESIAN_POINT('Ctrl Pts',(6.0000467896797,3.44759768203729,-9.24497095300123));
#41245=CARTESIAN_POINT('Ctrl Pts',(6.00006724836824,3.42266827285967,-9.2473496812447));
#41246=CARTESIAN_POINT('Ctrl Pts',(6.00007042323265,3.41879962341389,-9.24771882219126));
#41247=CARTESIAN_POINT('Ctrl Pts',(6.00007335753721,3.41493653288833,-9.24811124861399));
#41248=CARTESIAN_POINT('Ctrl Pts',(6.00007601149692,3.41107965124373,-9.24852695617774));
#41249=CARTESIAN_POINT('Ctrl Pts',(6.00009313069709,3.38620107876555,-9.25120845167268));
#41250=CARTESIAN_POINT('Ctrl Pts',(6.00009752492617,3.36158052757525,-9.25486277091957));
#41251=CARTESIAN_POINT('Ctrl Pts',(6.00008809909509,3.33739081585142,-9.2594608407126));
#41252=CARTESIAN_POINT('Ctrl Pts',(6.00007855584451,3.31289976799455,-9.26411618959132));
#41253=CARTESIAN_POINT('Ctrl Pts',(6.00005445404436,3.28885138994719,-9.26973869991398));
#41254=CARTESIAN_POINT('Ctrl Pts',(6.00003199288285,3.26541979533693,-9.27624752567763));
#41255=CARTESIAN_POINT('Ctrl Pts',(6.00001529299223,3.24799838696856,-9.28108684257062));
#41256=CARTESIAN_POINT('Ctrl Pts',(5.99999988409146,3.23091786654435,-9.28641496667356));
#41257=CARTESIAN_POINT('Ctrl Pts',(5.99999988834965,3.21424316874114,-9.29218288031211));
#41258=CARTESIAN_POINT('',(5.72001531699897,3.07996588268296,-9.45352634319216));
#41259=CARTESIAN_POINT('Ctrl Pts',(5.72001583933073,3.07996630535118,-9.4535276405668));
#41260=CARTESIAN_POINT('Ctrl Pts',(5.77262443154598,3.09390593168778,-9.42780571397045));
#41261=CARTESIAN_POINT('Ctrl Pts',(5.82215801010858,3.11234353252729,-9.40145328697083));
#41262=CARTESIAN_POINT('Ctrl Pts',(5.86878812167787,3.13479953409958,-9.37455809133654));
#41263=CARTESIAN_POINT('Ctrl Pts',(5.91541823324956,3.15725553567303,-9.34766289570087));
#41264=CARTESIAN_POINT('Ctrl Pts',(5.9591451108491,3.18373012441069,-9.32022546296157));
#41265=CARTESIAN_POINT('Ctrl Pts',(6.00000005306072,3.21424330184847,-9.2921832651174));
#41266=CARTESIAN_POINT('',(5.732785011186,3.68906787169418,-9.8154400921193));
#41267=CARTESIAN_POINT('Origin',(5.89877268707396,3.22461201072033,-9.89752207294649));
#41268=CARTESIAN_POINT('Ctrl Pts',(5.73278241140467,3.68907514109833,-9.81543880829859));
#41269=CARTESIAN_POINT('Ctrl Pts',(5.74767869655519,3.69181193174699,-9.80076990118021));
#41270=CARTESIAN_POINT('Ctrl Pts',(5.76173623909103,3.6953181596331,-9.78629106413066));
#41271=CARTESIAN_POINT('Ctrl Pts',(5.77495188027913,3.69939287286273,-9.77211145501697));
#41272=CARTESIAN_POINT('Ctrl Pts',(5.78903149098141,3.70373396953599,-9.75700485720687));
#41273=CARTESIAN_POINT('Ctrl Pts',(5.8021556712026,3.70872059120982,-9.7422377839714));
#41274=CARTESIAN_POINT('Ctrl Pts',(5.81434871324948,3.71415040708076,-9.72791047994506));
#41275=CARTESIAN_POINT('Ctrl Pts',(5.81704649346132,3.71535178486279,-9.7247404820772));
#41276=CARTESIAN_POINT('Ctrl Pts',(5.81969878836263,3.71657499800083,-9.72159190038994));
#41277=CARTESIAN_POINT('Ctrl Pts',(5.82230601989191,3.71781808030776,-9.7184656370051));
#41278=CARTESIAN_POINT('Ctrl Pts',(5.83435659809276,3.72356358483297,-9.70401610271081));
#41279=CARTESIAN_POINT('Ctrl Pts',(5.84544360969293,3.72972998718172,-9.69004559213706));
#41280=CARTESIAN_POINT('Ctrl Pts',(5.85563655093317,3.73611851920504,-9.67663236834336));
#41281=CARTESIAN_POINT('Ctrl Pts',(5.85625534830033,3.73650635689613,-9.67581807270749));
#41282=CARTESIAN_POINT('Ctrl Pts',(5.85687085394639,3.73689502613249,-9.675005822708));
#41283=CARTESIAN_POINT('Ctrl Pts',(5.8574830846827,3.73728448728698,-9.67419563274415));
#41284=CARTESIAN_POINT('Ctrl Pts',(5.86845368369367,3.7442632648995,-9.65967779054991));
#41285=CARTESIAN_POINT('Ctrl Pts',(5.87837190542306,3.75149250611659,-9.6458239201788));
#41286=CARTESIAN_POINT('Ctrl Pts',(5.88734074550242,3.75876990355745,-9.63270027080071));
#41287=CARTESIAN_POINT('Ctrl Pts',(5.89145114766236,3.76210512080907,-9.62668572752949));
#41288=CARTESIAN_POINT('Ctrl Pts',(5.89536229525458,3.76545109053723,-9.62082414314524));
#41289=CARTESIAN_POINT('Ctrl Pts',(5.89908473362999,3.7687912671586,-9.61511999917659));
#41290=CARTESIAN_POINT('Ctrl Pts',(5.90118652018917,3.77067721868286,-9.61189928954601));
#41291=CARTESIAN_POINT('Ctrl Pts',(5.90322815175333,3.77256135393962,-9.60872875266206));
#41292=CARTESIAN_POINT('Ctrl Pts',(5.90521156720407,3.77444091972493,-9.60560905069248));
#41293=CARTESIAN_POINT('Ctrl Pts',(5.90881698138608,3.77785755799699,-9.59993811688959));
#41294=CARTESIAN_POINT('Ctrl Pts',(5.91223005913712,3.78125896334876,-9.59443521989477));
#41295=CARTESIAN_POINT('Ctrl Pts',(5.91546371809077,3.78462845364829,-9.58910380772825));
#41296=CARTESIAN_POINT('Ctrl Pts',(5.91797000004203,3.78724001313668,-9.58497163971697));
#41297=CARTESIAN_POINT('Ctrl Pts',(5.92036843045022,3.78983237029622,-9.58094254052739));
#41298=CARTESIAN_POINT('Ctrl Pts',(5.92266498720102,3.79239866553362,-9.57701761862196));
#41299=CARTESIAN_POINT('Ctrl Pts',(5.92381326557642,3.79368181315232,-9.57505515766924));
#41300=CARTESIAN_POINT('Ctrl Pts',(5.92493606868236,3.79495845008678,-9.57311874029835));
#41301=CARTESIAN_POINT('Ctrl Pts',(5.92603412320337,3.79622776990128,-9.57120848851216));
#41302=CARTESIAN_POINT('Ctrl Pts',(5.92680721247964,3.79712143912988,-9.5698635687995));
#41303=CARTESIAN_POINT('Ctrl Pts',(5.9272598572055,3.79764976715791,-9.5690714496196));
#41304=CARTESIAN_POINT('Ctrl Pts',(5.92804436577352,3.79857558745796,-9.56769193863759));
#41305=CARTESIAN_POINT('Ctrl Pts',(5.92837413107571,3.79896475262896,-9.56711206625073));
#41306=CARTESIAN_POINT('Ctrl Pts',(5.92876221561471,3.79942440361365,-9.56642841113834));
#41307=CARTESIAN_POINT('Ctrl Pts',(5.92925474945964,3.80001299631371,-9.56555634204678));
#41308=CARTESIAN_POINT('Ctrl Pts',(5.93919911428426,3.81189681019301,-9.5479490785299));
#41309=CARTESIAN_POINT('Ctrl Pts',(5.94793617624666,3.82418303306961,-9.53098761711083));
#41310=CARTESIAN_POINT('Ctrl Pts',(5.95554257333252,3.8366698253501,-9.51474872794075));
#41311=CARTESIAN_POINT('Ctrl Pts',(5.95842928936594,3.84140870803993,-9.50858588090515));
#41312=CARTESIAN_POINT('Ctrl Pts',(5.96115320676407,3.84617694320634,-9.50252680046662));
#41313=CARTESIAN_POINT('Ctrl Pts',(5.96371874238293,3.85096506477631,-9.49657462218512));
#41314=CARTESIAN_POINT('Ctrl Pts',(5.97059811524388,3.86380420578894,-9.48061411341949));
#41315=CARTESIAN_POINT('Ctrl Pts',(5.97633958264131,3.87678283276641,-9.46542399863919));
#41316=CARTESIAN_POINT('Ctrl Pts',(5.98107332916792,3.88971313303436,-9.45104725786613));
#41317=CARTESIAN_POINT('Ctrl Pts',(5.98611100902723,3.90347363179968,-9.43574744892454));
#41318=CARTESIAN_POINT('Ctrl Pts',(5.99000695882383,3.91717969774421,-9.42136878702499));
#41319=CARTESIAN_POINT('Ctrl Pts',(5.99291129001556,3.93065595429813,-9.40793516398228));
#41320=CARTESIAN_POINT('Ctrl Pts',(5.9936189823796,3.93393968581135,-9.40466182088841));
#41321=CARTESIAN_POINT('Ctrl Pts',(5.99426778641181,3.93720998520123,-9.40144446713658));
#41322=CARTESIAN_POINT('Ctrl Pts',(5.99485986278615,3.94046470722935,-9.39828322180869));
#41323=CARTESIAN_POINT('Ctrl Pts',(5.99739682065465,3.95441069970065,-9.38473776288417));
#41324=CARTESIAN_POINT('Ctrl Pts',(5.99889426464765,3.9680669647464,-9.37222378271122));
#41325=CARTESIAN_POINT('Ctrl Pts',(5.99956526189633,3.98128094884042,-9.36072483287852));
#41326=CARTESIAN_POINT('Ctrl Pts',(5.99985052308264,3.9868986123791,-9.35583628217733));
#41327=CARTESIAN_POINT('Ctrl Pts',(5.99998613323582,3.99243691442869,-9.35113096953797));
#41328=CARTESIAN_POINT('Ctrl Pts',(5.9999873957484,3.99788653423051,-9.34660672477246));
#41329=CARTESIAN_POINT('Ctrl Pts',(5.99970218889552,4.00041486715457,-9.24574070815));
#41330=CARTESIAN_POINT('Ctrl Pts',(5.99970218889552,4.05365232671755,-9.67397475390689));
#41331=CARTESIAN_POINT('Ctrl Pts',(5.99970218889552,4.23216237618003,-10.6067286561567));
#41332=CARTESIAN_POINT('Ctrl Pts',(5.99970218889552,4.71033964600048,-11.9928024105301));
#41333=CARTESIAN_POINT('Ctrl Pts',(5.99970218889552,5.43783896865657,-13.3613500312052));
#41334=CARTESIAN_POINT('Ctrl Pts',(5.99970218889552,6.36842720326896,-14.5997817842042));
#41335=CARTESIAN_POINT('Ctrl Pts',(5.99970218889552,7.4806322410857,-15.6796607105075));
#41336=CARTESIAN_POINT('Ctrl Pts',(5.99970218889552,8.6355046825311,-16.4940256800099));
#41337=CARTESIAN_POINT('Ctrl Pts',(5.99970218889552,9.43064114619334,-16.9071647489066));
#41338=CARTESIAN_POINT('Ctrl Pts',(5.99970218889552,9.77579624644421,-17.0620851371039));
#41339=CARTESIAN_POINT('Ctrl Pts',(6.00690077768462,3.81539387032592,-9.26873651609987));
#41340=CARTESIAN_POINT('Ctrl Pts',(6.00690077768462,3.86963575160847,-9.70506457286073));
#41341=CARTESIAN_POINT('Ctrl Pts',(6.00690077768462,4.05148520857158,-10.6552730337179));
#41342=CARTESIAN_POINT('Ctrl Pts',(6.00690077768462,4.53871003918023,-12.0675567208086));
#41343=CARTESIAN_POINT('Ctrl Pts',(6.00690077768462,5.27984031821352,-13.4617523186532));
#41344=CARTESIAN_POINT('Ctrl Pts',(6.00690077768462,6.22801756506338,-14.7235948399977));
#41345=CARTESIAN_POINT('Ctrl Pts',(6.00690077768462,7.36107910569074,-15.823715865998));
#41346=CARTESIAN_POINT('Ctrl Pts',(6.00690077768462,8.53776162516752,-16.653466849808));
#41347=CARTESIAN_POINT('Ctrl Pts',(6.00690077768462,9.34778507995447,-17.0743424403229));
#41348=CARTESIAN_POINT('Ctrl Pts',(6.00690077768462,9.69945326722534,-17.2321839331678));
#41349=CARTESIAN_POINT('Ctrl Pts',(5.89988018238953,3.66357392134844,-9.28760584687473));
#41350=CARTESIAN_POINT('Ctrl Pts',(5.89988018238953,3.71863998614226,-9.73057548680401));
#41351=CARTESIAN_POINT('Ctrl Pts',(5.89988018238953,3.90322961143632,-10.6951063772361));
#41352=CARTESIAN_POINT('Ctrl Pts',(5.89988018238953,4.39787846548393,-12.12889676203));
#41353=CARTESIAN_POINT('Ctrl Pts',(5.89988018238953,5.15019369723824,-13.5441379420103));
#41354=CARTESIAN_POINT('Ctrl Pts',(5.89988018238953,6.11280370029348,-14.8251902920569));
#41355=CARTESIAN_POINT('Ctrl Pts',(5.89988018238953,7.2629791536517,-15.9419210790931));
#41356=CARTESIAN_POINT('Ctrl Pts',(5.89988018238953,8.45755804700211,-16.7842971376075));
#41357=CARTESIAN_POINT('Ctrl Pts',(5.89988018238953,9.27979710040495,-17.2115209714956));
#41358=CARTESIAN_POINT('Ctrl Pts',(5.89988018238953,9.63680963537774,-17.3717593920753));
#41359=CARTESIAN_POINT('Ctrl Pts',(5.72194802639809,3.60705103823582,-9.29463093801039));
#41360=CARTESIAN_POINT('Ctrl Pts',(5.72194802639809,3.6624239482688,-9.74007325318647));
#41361=CARTESIAN_POINT('Ctrl Pts',(5.72194802639809,3.84803374393823,-10.7099364139704));
#41362=CARTESIAN_POINT('Ctrl Pts',(5.72194802639809,4.34544657736628,-12.1517337870921));
#41363=CARTESIAN_POINT('Ctrl Pts',(5.72194802639809,5.10192599030869,-13.5748102811249));
#41364=CARTESIAN_POINT('Ctrl Pts',(5.72194802639809,6.06990933854909,-14.8630144903926));
#41365=CARTESIAN_POINT('Ctrl Pts',(5.72194802639809,7.22645633724943,-15.9859291260432));
#41366=CARTESIAN_POINT('Ctrl Pts',(5.72194802639809,8.42769808785784,-16.8330055261617));
#41367=CARTESIAN_POINT('Ctrl Pts',(5.72194802639809,9.25448503406041,-17.2625928242768));
#41368=CARTESIAN_POINT('Ctrl Pts',(5.72194802639809,9.61348728080861,-17.42372362604));
#41369=CARTESIAN_POINT('Ctrl Pts',(5.7327834389226,3.6890722712595,-9.81543931491054));
#41370=CARTESIAN_POINT('Ctrl Pts',(5.73338951170027,3.73677170904278,-10.084157914535));
#41371=CARTESIAN_POINT('Ctrl Pts',(5.73395354707033,3.79517197547473,-10.3512385133618));
#41372=CARTESIAN_POINT('Ctrl Pts',(5.7344755542285,3.86412906900604,-10.6157496455956));
#41373=CARTESIAN_POINT('Ctrl Pts',(5.73532470372123,3.97630163230417,-11.046030131679));
#41374=CARTESIAN_POINT('Ctrl Pts',(5.73606263992312,4.11640986609988,-11.4695137403519));
#41375=CARTESIAN_POINT('Ctrl Pts',(5.73668942140747,4.28354912573053,-11.8826273916816));
#41376=CARTESIAN_POINT('Ctrl Pts',(5.73681690169486,4.31754336675963,-11.9666500507909));
#41377=CARTESIAN_POINT('Ctrl Pts',(5.73693978387871,4.35265576367259,-12.050243567833));
#41378=CARTESIAN_POINT('Ctrl Pts',(5.73705806847412,4.38887864994803,-12.1333776205571));
#41379=CARTESIAN_POINT('Ctrl Pts',(5.737074784282,4.39399761582651,-12.1451260046035));
#41380=CARTESIAN_POINT('Ctrl Pts',(5.73709140827173,4.39913875918398,-12.156865212573));
#41381=CARTESIAN_POINT('Ctrl Pts',(5.73710794044476,4.4043020414885,-12.1685951647897));
#41382=CARTESIAN_POINT('Ctrl Pts',(5.73767502817134,4.58141330323435,-12.5709567857097));
#41383=CARTESIAN_POINT('Ctrl Pts',(5.73813408881124,4.78457573118237,-12.9624318471077));
#41384=CARTESIAN_POINT('Ctrl Pts',(5.73848518367753,5.01222354854569,-13.3397802562608));
#41385=CARTESIAN_POINT('Ctrl Pts',(5.73855071710513,5.05471503215729,-13.4102140250933));
#41386=CARTESIAN_POINT('Ctrl Pts',(5.7386124889663,5.0980595256941,-13.4801554890252));
#41387=CARTESIAN_POINT('Ctrl Pts',(5.73867049957996,5.14224676627578,-13.5495833927193));
#41388=CARTESIAN_POINT('Ctrl Pts',(5.73897977937872,5.37782815409092,-13.9197337277492));
#41389=CARTESIAN_POINT('Ctrl Pts',(5.73918215116736,5.63736614834506,-14.2752900546389));
#41390=CARTESIAN_POINT('Ctrl Pts',(5.73927764632016,5.91884386064799,-14.6132513264352));
#41391=CARTESIAN_POINT('Ctrl Pts',(5.73929840882404,5.98004259088702,-14.6867306812824));
#41392=CARTESIAN_POINT('Ctrl Pts',(5.73931411902131,6.04227833582952,-14.7593781301047));
#41393=CARTESIAN_POINT('Ctrl Pts',(5.73932477703137,6.10553019429181,-14.8311625497617));
#41394=CARTESIAN_POINT('Ctrl Pts',(5.73937358627051,6.39519731501835,-15.1599052406577));
#41395=CARTESIAN_POINT('Ctrl Pts',(5.73931644079047,6.7061775767551,-15.4705511644378));
#41396=CARTESIAN_POINT('Ctrl Pts',(5.73915333151696,7.03610866911516,-15.7604158973285));
#41397=CARTESIAN_POINT('Ctrl Pts',(5.73911747414971,7.10863955650045,-15.8241387375975));
#41398=CARTESIAN_POINT('Ctrl Pts',(5.73907649562849,7.18208617501254,-15.8868571080663));
#41399=CARTESIAN_POINT('Ctrl Pts',(5.7390303956456,7.25642321283939,-15.9485422260026));
#41400=CARTESIAN_POINT('Ctrl Pts',(5.73900084443127,7.30407506865231,-15.9880838923325));
#41401=CARTESIAN_POINT('Ctrl Pts',(5.73896918874389,7.35209280736278,-16.0272009802856));
#41402=CARTESIAN_POINT('Ctrl Pts',(5.73893542848712,7.40046852655848,-16.0658876523886));
#41403=CARTESIAN_POINT('Ctrl Pts',(5.73869640194024,7.74297424835245,-16.3397937931704));
#41404=CARTESIAN_POINT('Ctrl Pts',(5.7383518708658,8.10342832194923,-16.5921267927799));
#41405=CARTESIAN_POINT('Ctrl Pts',(5.7379017997706,8.47900281544137,-16.8207962970312));
#41406=CARTESIAN_POINT('Ctrl Pts',(5.73786596841235,8.5089033008736,-16.8390012851205));
#41407=CARTESIAN_POINT('Ctrl Pts',(5.7378294681113,8.53889960067031,-16.8570562728187));
#41408=CARTESIAN_POINT('Ctrl Pts',(5.73779229884403,8.56899027663243,-16.8749601964822));
#41409=CARTESIAN_POINT('Ctrl Pts',(5.7374116956997,8.87711057941036,-17.0582914844555));
#41410=CARTESIAN_POINT('Ctrl Pts',(5.73696095042956,9.19512814699331,-17.2257845440857));
#41411=CARTESIAN_POINT('Ctrl Pts',(5.73644003522278,9.52122270927801,-17.3763183336487));
#41412=CARTESIAN_POINT('Ctrl Pts',(5.99999999930592,3.99788653280082,-9.34660672570642));
#41413=CARTESIAN_POINT('Ctrl Pts',(5.99999999931562,4.01825013013249,-9.49792584808906));
#41414=CARTESIAN_POINT('Ctrl Pts',(5.99999999835918,4.04202369835754,-9.64825763309733));
#41415=CARTESIAN_POINT('Ctrl Pts',(5.99999999609537,4.06917084562767,-9.79770306355383));
#41416=CARTESIAN_POINT('Ctrl Pts',(5.99999999382034,4.09645246929592,-9.94788878848784));
#41417=CARTESIAN_POINT('Ctrl Pts',(5.99999999024012,4.12714128448646,-10.0971798054401));
#41418=CARTESIAN_POINT('Ctrl Pts',(5.99999999039158,4.1612523170038,-10.2456708113104));
#41419=CARTESIAN_POINT('Ctrl Pts',(5.9999999904855,4.18240376014979,-10.3377465661783));
#41420=CARTESIAN_POINT('Ctrl Pts',(5.99999999231395,4.20487204400595,-10.4295145418709));
#41421=CARTESIAN_POINT('Ctrl Pts',(5.99999999505291,4.22867045872271,-10.5209946588892));
#41422=CARTESIAN_POINT('Ctrl Pts',(5.99999999721692,4.24747323717649,-10.5932717577503));
#41423=CARTESIAN_POINT('Ctrl Pts',(5.99999999999964,4.26710647649524,-10.6653691270461));
#41424=CARTESIAN_POINT('Ctrl Pts',(5.99999999999964,4.28757893858364,-10.7372995788032));
#41425=CARTESIAN_POINT('Ctrl Pts',(5.99999999999964,4.33786650361673,-10.9139860591577));
#41426=CARTESIAN_POINT('Ctrl Pts',(5.99999998462025,4.39314036643884,-11.0896695597218));
#41427=CARTESIAN_POINT('Ctrl Pts',(5.99999998025196,4.45330086234597,-11.2638532657156));
#41428=CARTESIAN_POINT('Ctrl Pts',(5.99999997588671,4.51341961085679,-11.4379160997636));
#41429=CARTESIAN_POINT('Ctrl Pts',(5.99999998175306,4.57841809273495,-11.6104807782189));
#41430=CARTESIAN_POINT('Ctrl Pts',(5.99999999007196,4.6481466218464,-11.7810648390995));
#41431=CARTESIAN_POINT('Ctrl Pts',(5.99999999337622,4.67584266136247,-11.8488205045518));
#41432=CARTESIAN_POINT('Ctrl Pts',(5.99999999675167,4.70428439666252,-11.9162638791355));
#41433=CARTESIAN_POINT('Ctrl Pts',(5.99999999861009,4.73346031539168,-11.9833655503387));
#41434=CARTESIAN_POINT('Ctrl Pts',(5.99999999947165,4.74698625511949,-12.0144738478616));
#41435=CARTESIAN_POINT('Ctrl Pts',(5.99999999999964,4.76066997194886,-12.0455087123589));
#41436=CARTESIAN_POINT('Ctrl Pts',(5.99999999999964,4.77450985443936,-12.0764672813386));
#41437=CARTESIAN_POINT('Ctrl Pts',(5.99999999999964,4.86135087722856,-12.270722817549));
#41438=CARTESIAN_POINT('Ctrl Pts',(5.99999998564323,4.95440536705064,-12.4619541304201));
#41439=CARTESIAN_POINT('Ctrl Pts',(5.9999999850471,5.05350689336951,-12.6499608882332));
#41440=CARTESIAN_POINT('Ctrl Pts',(5.99999998445025,5.15272837313359,-12.8381952112428));
#41441=CARTESIAN_POINT('Ctrl Pts',(5.99999999412997,5.25801178107184,-13.0231976929862));
#41442=CARTESIAN_POINT('Ctrl Pts',(5.99999999838051,5.36923781847837,-13.2047465952675));
#41443=CARTESIAN_POINT('Ctrl Pts',(5.99999999937177,5.3951765530956,-13.2470851421233));
#41444=CARTESIAN_POINT('Ctrl Pts',(5.99999999999964,5.42143867719124,-13.2892357558119));
#41445=CARTESIAN_POINT('Ctrl Pts',(5.99999999999964,5.44802302870523,-13.3311954148891));
#41446=CARTESIAN_POINT('Ctrl Pts',(5.99999999999964,5.45163175457307,-13.3368912810094));
#41447=CARTESIAN_POINT('Ctrl Pts',(5.9999999999881,5.45524638131076,-13.3425836503172));
#41448=CARTESIAN_POINT('Ctrl Pts',(5.99999999996605,5.45886690005094,-13.3482725046921));
#41449=CARTESIAN_POINT('Ctrl Pts',(5.99999999925239,5.57604743761589,-13.5323961238789));
#41450=CARTESIAN_POINT('Ctrl Pts',(5.9999999904792,5.6994038552837,-13.7128355868706));
#41451=CARTESIAN_POINT('Ctrl Pts',(5.99999999007258,5.82856569873213,-13.8890427222146));
#41452=CARTESIAN_POINT('Ctrl Pts',(5.99999998966571,5.95780733724832,-14.0653587168001));
#41453=CARTESIAN_POINT('Ctrl Pts',(5.99999999693157,6.09286125024825,-14.2374366970401));
#41454=CARTESIAN_POINT('Ctrl Pts',(5.99999999941398,6.23331363007942,-14.4047572445278));
#41455=CARTESIAN_POINT('Ctrl Pts',(5.9999999997784,6.25393228767317,-14.4293201966202));
#41456=CARTESIAN_POINT('Ctrl Pts',(5.99999999999964,6.27466721652169,-14.4537806817704));
#41457=CARTESIAN_POINT('Ctrl Pts',(5.99999999999964,6.2955170368321,-14.4781371198393));
#41458=CARTESIAN_POINT('Ctrl Pts',(5.99999999999964,6.32570182820854,-14.5133985269324));
#41459=CARTESIAN_POINT('Ctrl Pts',(5.99999999953038,6.35612835002207,-14.5484407605217));
#41460=CARTESIAN_POINT('Ctrl Pts',(5.9999999987273,6.38679509714238,-14.5832618902974));
#41461=CARTESIAN_POINT('Ctrl Pts',(5.99999999501563,6.5285310601452,-14.7441986320471));
#41462=CARTESIAN_POINT('Ctrl Pts',(5.99999998445148,6.67539562223214,-14.9004153354487));
#41463=CARTESIAN_POINT('Ctrl Pts',(5.99999998419194,6.82720685789883,-15.0517239487321));
#41464=CARTESIAN_POINT('Ctrl Pts',(5.99999998393239,6.97901809356552,-15.2030325620155));
#41465=CARTESIAN_POINT('Ctrl Pts',(5.99999999999964,7.13577644841082,-15.3494334645929));
#41466=CARTESIAN_POINT('Ctrl Pts',(5.99999999999964,7.29733248735904,-15.4906976622844));
#41467=CARTESIAN_POINT('Ctrl Pts',(5.99999999999964,7.36277783087636,-15.5479229074984));
#41468=CARTESIAN_POINT('Ctrl Pts',(5.99999999597129,7.4290034226837,-15.6043166838342));
#41469=CARTESIAN_POINT('Ctrl Pts',(5.99999999157416,7.49596991329926,-15.6598390584008));
#41470=CARTESIAN_POINT('Ctrl Pts',(5.99999998233606,7.63666220114164,-15.776487994793));
#41471=CARTESIAN_POINT('Ctrl Pts',(5.99999997355904,7.78062676030411,-15.8892879071132));
#41472=CARTESIAN_POINT('Ctrl Pts',(5.99999997660567,7.92745072947075,-15.9979560613712));
#41473=CARTESIAN_POINT('Ctrl Pts',(5.99999997965611,8.07445806097555,-16.1067599267598));
#41474=CARTESIAN_POINT('Ctrl Pts',(5.99999999487372,8.22433156184451,-16.211421464211));
#41475=CARTESIAN_POINT('Ctrl Pts',(5.99999999914232,8.37662831455504,-16.3117005488194));
#41476=CARTESIAN_POINT('Ctrl Pts',(5.9999999996836,8.39594054927499,-16.3244165994573));
#41477=CARTESIAN_POINT('Ctrl Pts',(5.99999999999964,8.41529171670325,-16.3370622409303));
#41478=CARTESIAN_POINT('Ctrl Pts',(5.99999999999964,8.43468088597692,-16.349637036712));
#41479=CARTESIAN_POINT('Ctrl Pts',(5.99999999999964,8.5422003635077,-16.419368516871));
#41480=CARTESIAN_POINT('Ctrl Pts',(5.99999999306094,8.65090074866789,-16.4868827931156));
#41481=CARTESIAN_POINT('Ctrl Pts',(5.99999999145038,8.76083030931053,-16.5522396053082));
#41482=CARTESIAN_POINT('Ctrl Pts',(5.99999998952809,8.89203703813673,-16.630246407884));
#41483=CARTESIAN_POINT('Ctrl Pts',(5.9999999927489,9.02499432575621,-16.7051809905324));
#41484=CARTESIAN_POINT('Ctrl Pts',(5.99999999547941,9.15977750377954,-16.7771012992923));
#41485=CARTESIAN_POINT('Ctrl Pts',(5.99999999819766,9.2939557808812,-16.8486988328981));
#41486=CARTESIAN_POINT('Ctrl Pts',(5.99999999961509,9.42994399508163,-16.917309315494));
#41487=CARTESIAN_POINT('Ctrl Pts',(5.99999999985075,9.56784100775507,-16.9829446186675));
#41488=CARTESIAN_POINT('Ctrl Pts',(5.99999999991364,9.60463633082665,-17.0004582118799));
#41489=CARTESIAN_POINT('Ctrl Pts',(5.99999999993319,9.64156767640953,-17.0177597130991));
#41490=CARTESIAN_POINT('Ctrl Pts',(5.99999999993288,9.67863716454227,-17.0348487658772));
#41491=CARTESIAN_POINT('Ctrl Pts',(-5.843530343918,3.68097998125157,-9.5215919621966));
#41492=CARTESIAN_POINT('Ctrl Pts',(-3.895686895945,3.12097286918903,-10.4634459889947));
#41493=CARTESIAN_POINT('Ctrl Pts',(0.0001666015266437,2.56014793946572,
-11.405543724591));
#41494=CARTESIAN_POINT('Ctrl Pts',(3.896020098999,3.1210208372572,-10.4633654101759));
#41495=CARTESIAN_POINT('Ctrl Pts',(5.844030148498,3.68112368174947,-9.52135027794804));
#41496=CARTESIAN_POINT('Ctrl Pts',(-5.843530343918,3.79656867134517,-10.3003500893644));
#41497=CARTESIAN_POINT('Ctrl Pts',(-3.895686895945,3.28180629096974,-11.180108871291));
#41498=CARTESIAN_POINT('Ctrl Pts',(0.0001666015266437,2.76478792290348,
-12.0604741630417));
#41499=CARTESIAN_POINT('Ctrl Pts',(3.896020098999,3.28185051220906,-11.1800335725302));
#41500=CARTESIAN_POINT('Ctrl Pts',(5.844030148498,3.79670076181209,-10.3001243390543));
#41501=CARTESIAN_POINT('Ctrl Pts',(-5.843530343918,4.23580747360814,-11.9384157807471));
#41502=CARTESIAN_POINT('Ctrl Pts',(-3.895686895945,3.77920767318315,-12.6803385188317));
#41503=CARTESIAN_POINT('Ctrl Pts',(0.0001666015266437,3.32382461832179,
-13.4219179025983));
#41504=CARTESIAN_POINT('Ctrl Pts',(3.896020098999,3.77924662267507,-12.6802750906046));
#41505=CARTESIAN_POINT('Ctrl Pts',(5.844030148498,4.23592463931539,-11.938225399815));
#41506=CARTESIAN_POINT('Ctrl Pts',(-5.843530343918,5.5035950710752,-14.2139339843063));
#41507=CARTESIAN_POINT('Ctrl Pts',(-3.895686895945,5.02273055892627,-14.7660279845512));
#41508=CARTESIAN_POINT('Ctrl Pts',(0.0001666015266437,4.54131537343804,
-15.3185232177601));
#41509=CARTESIAN_POINT('Ctrl Pts',(3.896020098999,5.02277173497978,-14.7659807289319));
#41510=CARTESIAN_POINT('Ctrl Pts',(5.844030148498,5.50371846320554,-14.2137923143453));
#41511=CARTESIAN_POINT('Ctrl Pts',(-5.843530343918,7.3885050858399,-16.156062941913));
#41512=CARTESIAN_POINT('Ctrl Pts',(-3.895686895945,6.77499147815254,-16.5818456382825));
#41513=CARTESIAN_POINT('Ctrl Pts',(0.0001666015266437,6.16225586059323,
-17.0065483907037));
#41514=CARTESIAN_POINT('Ctrl Pts',(3.896020098999,6.7750438862104,-16.5818093129175));
#41515=CARTESIAN_POINT('Ctrl Pts',(5.844030148498,7.38866251637734,-16.1559536840225));
#41516=CARTESIAN_POINT('Ctrl Pts',(-5.843530343918,8.93341756257242,-17.0810053340763));
#41517=CARTESIAN_POINT('Ctrl Pts',(-3.895686895945,8.18554666399747,-17.491591968287));
#41518=CARTESIAN_POINT('Ctrl Pts',(0.0001666015266437,7.43613425203332,
-17.9044829814061));
#41519=CARTESIAN_POINT('Ctrl Pts',(3.896020098999,8.18561076219368,-17.4915566531935));
#41520=CARTESIAN_POINT('Ctrl Pts',(5.844030148498,8.93360946981109,-17.0808999756088));
#41521=CARTESIAN_POINT('Ctrl Pts',(-5.843530343918,9.74782183257114,-17.434906675706));
#41522=CARTESIAN_POINT('Ctrl Pts',(-3.895686895945,8.92798459116701,-17.8601636149315));
#41523=CARTESIAN_POINT('Ctrl Pts',(0.0001666015266437,8.1080647953231,-18.2855106697697));
#41524=CARTESIAN_POINT('Ctrl Pts',(3.896020098999,8.92805471995194,-17.86012723446));
#41525=CARTESIAN_POINT('Ctrl Pts',(5.844030148498,9.74803220673196,-17.4347975527403));
#41526=CARTESIAN_POINT('Ctrl Pts',(-5.73278975501784,3.68906394501494,-9.81543852467968));
#41527=CARTESIAN_POINT('Ctrl Pts',(-5.37901312686398,3.59283532062234,-9.98633382004624));
#41528=CARTESIAN_POINT('Ctrl Pts',(-5.01621706148927,3.50244639616453,-10.1410528069802));
#41529=CARTESIAN_POINT('Ctrl Pts',(-4.64601453417756,3.41960856061868,-10.2790753857095));
#41530=CARTESIAN_POINT('Ctrl Pts',(-4.37165623574712,3.35821717096216,-10.3813643682297));
#41531=CARTESIAN_POINT('Ctrl Pts',(-4.09323005633235,3.30097639447212,-10.4744809579979));
#41532=CARTESIAN_POINT('Ctrl Pts',(-3.81139253999388,3.24858254091202,-10.5582409695191));
#41533=CARTESIAN_POINT('Ctrl Pts',(-3.57235399153529,3.20414505485315,-10.629281446433));
#41534=CARTESIAN_POINT('Ctrl Pts',(-3.33086150898132,3.16319478165567,-10.6935907748667));
#41535=CARTESIAN_POINT('Ctrl Pts',(-3.08731565576137,3.12613831654997,-10.7510928452597));
#41536=CARTESIAN_POINT('Ctrl Pts',(-3.04370967163684,3.11950349354746,-10.7613883782591));
#41537=CARTESIAN_POINT('Ctrl Pts',(-3.00003786142227,3.11299343151016,-10.7714658046476));
#41538=CARTESIAN_POINT('Ctrl Pts',(-2.95630252426794,3.10661037140673,-10.7813248529935));
#41539=CARTESIAN_POINT('Ctrl Pts',(-2.75784317738745,3.07764573956327,-10.8260625964956));
#41540=CARTESIAN_POINT('Ctrl Pts',(-2.55807094835414,3.05131357907767,-10.866364096742));
#41541=CARTESIAN_POINT('Ctrl Pts',(-2.35725261120207,3.02779065953336,-10.9021038314712));
#41542=CARTESIAN_POINT('Ctrl Pts',(-2.16327810578139,3.00506939438713,-10.9366255662206));
#41543=CARTESIAN_POINT('Ctrl Pts',(-1.9683275793972,2.98496919543223,-10.9668911187537));
#41544=CARTESIAN_POINT('Ctrl Pts',(-1.77264145029077,2.96762488254539,-10.9928288224598));
#41545=CARTESIAN_POINT('Ctrl Pts',(-1.58004668869298,2.95055456784925,-11.0183567731862));
#41546=CARTESIAN_POINT('Ctrl Pts',(-1.38673938228074,2.93615384392036,-11.0396923982212));
#41547=CARTESIAN_POINT('Ctrl Pts',(-1.19294873426629,2.92452605748633,-11.0568097509667));
#41548=CARTESIAN_POINT('Ctrl Pts',(-0.99481114965818,2.91263744706069,-11.0743110646918));
#41549=CARTESIAN_POINT('Ctrl Pts',(-0.796168296488997,2.9036478299414,-11.0874023173225));
#41550=CARTESIAN_POINT('Ctrl Pts',(-0.597265150369091,2.89763823993256,
-11.0961050744984));
#41551=CARTESIAN_POINT('Ctrl Pts',(-0.408473574731138,2.89193415737359,
-11.1043654126162));
#41552=CARTESIAN_POINT('Ctrl Pts',(-0.219447498295875,2.88891469255251,
-11.1086723131217));
#41553=CARTESIAN_POINT('Ctrl Pts',(-0.030396402586863,2.88862252261748,
-11.1090887091539));
#41554=CARTESIAN_POINT('Ctrl Pts',(-0.0202709323560394,2.88860687416028,
-11.1091110110909));
#41555=CARTESIAN_POINT('Ctrl Pts',(-0.010145390354594,2.88859904285181,
-11.1091221633804));
#41556=CARTESIAN_POINT('Ctrl Pts',(-1.98087675444825E-5,2.88859903306065,
-11.1091221793492));
#41557=CARTESIAN_POINT('Ctrl Pts',(-1.32058452790807E-5,2.88859903305426,
-11.1091221793596));
#41558=CARTESIAN_POINT('Ctrl Pts',(-6.60292303140436E-6,2.88859903305121,
-11.1091221793653));
#41559=CARTESIAN_POINT('Ctrl Pts',(-7.99360577730113E-13,2.88859903305147,
-11.1091221793662));
#41560=CARTESIAN_POINT('Ctrl Pts',(0.189405503646998,2.88859904071486,-11.1091222063918));
#41561=CARTESIAN_POINT('Ctrl Pts',(0.378797279580155,2.8913380614621,-11.1052218521454));
#41562=CARTESIAN_POINT('Ctrl Pts',(0.567964667945599,2.89677460616661,-11.097355447509));
#41563=CARTESIAN_POINT('Ctrl Pts',(0.769363593162857,2.90256267709069,-11.0889804022499));
#41564=CARTESIAN_POINT('Ctrl Pts',(0.970508174933544,2.91140858960037,-11.0761095047332));
#41565=CARTESIAN_POINT('Ctrl Pts',(1.171144190504,2.92322964262542,-11.0587180531935));
#41566=CARTESIAN_POINT('Ctrl Pts',(1.36695866628512,2.93476662064355,-11.0417445404538));
#41567=CARTESIAN_POINT('Ctrl Pts',(1.56228872515895,2.94913719244932,-11.0204655771592));
#41568=CARTESIAN_POINT('Ctrl Pts',(1.75689803534998,2.96623568336572,-10.9949064346219));
#41569=CARTESIAN_POINT('Ctrl Pts',(1.95869514303697,2.9839656984886,-10.9684032779439));
#41570=CARTESIAN_POINT('Ctrl Pts',(2.15971727784271,3.00462885550607,-10.9372979254205));
#41571=CARTESIAN_POINT('Ctrl Pts',(2.35970094251548,3.0280777242204,-10.9016683699337));
#41572=CARTESIAN_POINT('Ctrl Pts',(2.55968460718826,3.05152659293472,-10.8660388144469));
#41573=CARTESIAN_POINT('Ctrl Pts',(2.75862980172807,3.07776097135519,-10.825885376108));
#41574=CARTESIAN_POINT('Ctrl Pts',(2.95627302888323,3.10660622105748,-10.7813321095109));
#41575=CARTESIAN_POINT('Ctrl Pts',(3.19877084584174,3.14199782128135,-10.7266676009231));
#41576=CARTESIAN_POINT('Ctrl Pts',(3.43931583985532,3.18129608636574,-10.6652855428938));
#41577=CARTESIAN_POINT('Ctrl Pts',(3.67751607631245,3.2241077234401,-10.5972522151377));
#41578=CARTESIAN_POINT('Ctrl Pts',(3.96233417229581,3.27529797051463,-10.51590417299));
#41579=CARTESIAN_POINT('Ctrl Pts',(4.2437999231366,3.33151069708892,-10.4250471694021));
#41580=CARTESIAN_POINT('Ctrl Pts',(4.52124330571427,3.39203867129015,-10.3248614333745));
#41581=CARTESIAN_POINT('Ctrl Pts',(4.88827658264392,3.47211187581421,-10.192324486001));
#41582=CARTESIAN_POINT('Ctrl Pts',(5.24827032461013,3.55973199273167,-10.0434649111247));
#41583=CARTESIAN_POINT('Ctrl Pts',(5.59967327730505,3.6532475106715,-9.8787802312009));
#41584=CARTESIAN_POINT('Ctrl Pts',(5.6441832833375,3.66509253427107,-9.85792065662804));
#41585=CARTESIAN_POINT('Ctrl Pts',(5.6885554613365,3.6770322090519,-9.83680721171413));
#41586=CARTESIAN_POINT('Ctrl Pts',(5.7327866589135,3.68906325963484,-9.81544090738039));
#41587=CARTESIAN_POINT('Ctrl Pts',(-5.84422094409324,3.72283000523856,-9.78167408162266));
#41588=CARTESIAN_POINT('Ctrl Pts',(-5.38507933576137,3.59683815761584,-10.0152843826947));
#41589=CARTESIAN_POINT('Ctrl Pts',(-4.35131200003916,3.34345413932339,-10.4619161435517));
#41590=CARTESIAN_POINT('Ctrl Pts',(-2.68512122938073,3.05355923238929,-10.9303254787283));
#41591=CARTESIAN_POINT('Ctrl Pts',(-0.894430115197969,2.89419166045093,
-11.1728831745123));
#41592=CARTESIAN_POINT('Ctrl Pts',(0.897577000464036,2.89433296944046,-11.1726725040321));
#41593=CARTESIAN_POINT('Ctrl Pts',(2.68825409632356,3.05397482372149,-10.9296798875333));
#41594=CARTESIAN_POINT('Ctrl Pts',(4.35334874826658,3.34391794571683,-10.4611286604278));
#41595=CARTESIAN_POINT('Ctrl Pts',(5.38611390228171,3.59711968962454,-10.014763833926));
#41596=CARTESIAN_POINT('Ctrl Pts',(5.84433011088186,3.72285991154443,-9.78161853339931));
#41597=CARTESIAN_POINT('Ctrl Pts',(-5.7253823284647,3.64455025382003,-9.50229674233198));
#41598=CARTESIAN_POINT('Ctrl Pts',(-5.27548411908097,3.52282891856501,-9.73077840355672));
#41599=CARTESIAN_POINT('Ctrl Pts',(-4.26255740633406,3.27781652768212,-10.1677131448542));
#41600=CARTESIAN_POINT('Ctrl Pts',(-2.63017516266764,2.99718831488208,-10.6260529752425));
#41601=CARTESIAN_POINT('Ctrl Pts',(-0.876088458604595,2.84283318581267,
-10.8634076236384));
#41602=CARTESIAN_POINT('Ctrl Pts',(0.879170849863336,2.8429700697441,-10.8632014724712));
#41603=CARTESIAN_POINT('Ctrl Pts',(2.63324420333494,2.99759077241429,-10.6254212356259));
#41604=CARTESIAN_POINT('Ctrl Pts',(4.26455304776783,3.27826526122104,-10.1669426530745));
#41605=CARTESIAN_POINT('Ctrl Pts',(5.27649785620924,3.52310092714498,-9.73026926825663));
#41606=CARTESIAN_POINT('Ctrl Pts',(5.72548929810404,3.6445791484027,-9.5022424109029));
#41607=CARTESIAN_POINT('Ctrl Pts',(-5.71943584543031,3.37475341540664,-9.34268206148292));
#41608=CARTESIAN_POINT('Ctrl Pts',(-5.27084297399291,3.25437642499162,-9.56884092463208));
#41609=CARTESIAN_POINT('Ctrl Pts',(-4.26059460930962,3.01185372124479,-10.0016516746214));
#41610=CARTESIAN_POINT('Ctrl Pts',(-2.6305607665523,2.73346781021963,-10.4564761199075));
#41611=CARTESIAN_POINT('Ctrl Pts',(-0.876566641464214,2.58004209268039,
-10.6924012836617));
#41612=CARTESIAN_POINT('Ctrl Pts',(0.879650375344035,2.58017826058766,-10.6921962381974));
#41613=CARTESIAN_POINT('Ctrl Pts',(2.63362771378936,2.73386754327752,-10.4558485735717));
#41614=CARTESIAN_POINT('Ctrl Pts',(4.26258539034863,3.01229823853514,-10.0008879757299));
#41615=CARTESIAN_POINT('Ctrl Pts',(5.27185378417918,3.25464542811177,-9.56833693988253));
#41616=CARTESIAN_POINT('Ctrl Pts',(5.71954249942017,3.37478198354303,-9.34262828327426));
#41617=CARTESIAN_POINT('Ctrl Pts',(-5.83023996337941,3.08845069594387,-9.4063707542719));
#41618=CARTESIAN_POINT('Ctrl Pts',(-5.37416754064385,2.96561979924004,-9.63451945103832));
#41619=CARTESIAN_POINT('Ctrl Pts',(-4.34669767293009,2.71808976474014,-10.0714544604592));
#41620=CARTESIAN_POINT('Ctrl Pts',(-2.68602843357863,2.4334671496755,-10.5315980787564));
#41621=CARTESIAN_POINT('Ctrl Pts',(-0.895554653482513,2.27628487850067,
-10.7707946411655));
#41622=CARTESIAN_POINT('Ctrl Pts',(0.898704696302249,2.27642450392807,-10.7705865705077));
#41623=CARTESIAN_POINT('Ctrl Pts',(2.68915637879637,2.43387633501067,-10.5309623471982));
#41624=CARTESIAN_POINT('Ctrl Pts',(4.3487229931822,2.71854365750337,-10.0706829494537));
#41625=CARTESIAN_POINT('Ctrl Pts',(5.37519522517315,2.96589426453183,-9.63401101278662));
#41626=CARTESIAN_POINT('Ctrl Pts',(5.83034838799569,3.08847983468315,-9.40631650684342));
#41627=CARTESIAN_POINT('Ctrl Pts',(-5.72001753233616,3.07996681168233,-9.45352318625267));
#41628=CARTESIAN_POINT('Ctrl Pts',(-5.54305534100265,3.03310276487157,-9.54003493482035));
#41629=CARTESIAN_POINT('Ctrl Pts',(-5.3615059653871,2.98701684693875,-9.62354209665977));
#41630=CARTESIAN_POINT('Ctrl Pts',(-5.1753597899198,2.94208361578591,-9.70365867399441));
#41631=CARTESIAN_POINT('Ctrl Pts',(-4.99261523307681,2.89797149049547,-9.78231120813346));
#41632=CARTESIAN_POINT('Ctrl Pts',(-4.80544024685734,2.85497027317297,-9.85769593441277));
#41633=CARTESIAN_POINT('Ctrl Pts',(-4.6138516950545,2.81347141986786,-9.9294257276793));
#41634=CARTESIAN_POINT('Ctrl Pts',(-4.54633624105595,2.79884730013341,-9.95470317516789));
#41635=CARTESIAN_POINT('Ctrl Pts',(-4.47827293657318,2.78441009408221,-9.97952653607247));
#41636=CARTESIAN_POINT('Ctrl Pts',(-4.40966334609503,2.77017807323515,-10.0038782076587));
#41637=CARTESIAN_POINT('Ctrl Pts',(-4.40581152306788,2.76937907086188,-10.0052453391152));
#41638=CARTESIAN_POINT('Ctrl Pts',(-4.40195797835678,2.76858071535721,-10.0066109837952));
#41639=CARTESIAN_POINT('Ctrl Pts',(-4.39810271264232,2.76778301002835,-10.0079751385947));
#41640=CARTESIAN_POINT('Ctrl Pts',(-4.20696612240203,2.72823432833767,-10.0756072854423));
#41641=CARTESIAN_POINT('Ctrl Pts',(-4.01159851371404,2.69026623838527,-10.1395832951787));
#41642=CARTESIAN_POINT('Ctrl Pts',(-3.81207290579326,2.65420530166328,-10.1995431025816));
#41643=CARTESIAN_POINT('Ctrl Pts',(-3.76843043495447,2.64631765057073,-10.2126581817604));
#41644=CARTESIAN_POINT('Ctrl Pts',(-3.72458910374073,2.63852139568591,-10.2255810089721));
#41645=CARTESIAN_POINT('Ctrl Pts',(-3.6805497995005,2.63082021387585,-10.2383076400666));
#41646=CARTESIAN_POINT('Ctrl Pts',(-3.55786021758428,2.60936540679298,-10.2737629015682));
#41647=CARTESIAN_POINT('Ctrl Pts',(-3.43363449003342,2.5886457533485,-10.3076961673479));
#41648=CARTESIAN_POINT('Ctrl Pts',(-3.30789770372184,2.56872932468178,-10.340022384266));
#41649=CARTESIAN_POINT('Ctrl Pts',(-3.24502931056605,2.55877111034841,-10.356185492725));
#41650=CARTESIAN_POINT('Ctrl Pts',(-3.18178314679223,2.54901369546737,-10.3719468108874));
#41651=CARTESIAN_POINT('Ctrl Pts',(-3.11816301394347,2.53946498461077,-10.3872955340494));
#41652=CARTESIAN_POINT('Ctrl Pts',(-3.08635294751909,2.53469062918247,-10.3949698956304));
#41653=CARTESIAN_POINT('Ctrl Pts',(-3.05444938858022,2.52996844940208,-10.4025411068631));
#41654=CARTESIAN_POINT('Ctrl Pts',(-3.02245283213984,2.52529941032688,-10.4100078084096));
#41655=CARTESIAN_POINT('Ctrl Pts',(-3.00645455391965,2.52296489078928,-10.4137411591829));
#41656=CARTESIAN_POINT('Ctrl Pts',(-2.99043302631282,2.52064365640634,-10.4174483824348));
#41657=CARTESIAN_POINT('Ctrl Pts',(-2.97438831367734,2.51833582545579,-10.4211293077042));
#41658=CARTESIAN_POINT('Ctrl Pts',(-2.95955595302759,2.51620237615352,-10.4245320991634));
#41659=CARTESIAN_POINT('Ctrl Pts',(-2.94352577511445,2.5139130275725,-10.4281786877099));
#41660=CARTESIAN_POINT('Ctrl Pts',(-2.92956478792253,2.51193203497011,-10.4313304172836));
#41661=CARTESIAN_POINT('Ctrl Pts',(-2.92842365934937,2.51177011466815,-10.4315880300599));
#41662=CARTESIAN_POINT('Ctrl Pts',(-2.9272963626467,2.51161024093396,-10.4318423609015));
#41663=CARTESIAN_POINT('Ctrl Pts',(-2.92618468578872,2.51145266038476,-10.4320930187536));
#41664=CARTESIAN_POINT('Ctrl Pts',(-2.83482829520798,2.49850286288042,-10.4526918074003));
#41665=CARTESIAN_POINT('Ctrl Pts',(-2.74308865013777,2.48609382009464,-10.4723429839348));
#41666=CARTESIAN_POINT('Ctrl Pts',(-2.65097987157538,2.47424830538277,-10.491036159891));
#41667=CARTESIAN_POINT('Ctrl Pts',(-2.40077663237707,2.44207128385301,-10.541814090596));
#41668=CARTESIAN_POINT('Ctrl Pts',(-2.14784930868952,2.41405016388818,-10.585526059997));
#41669=CARTESIAN_POINT('Ctrl Pts',(-1.89260573277423,2.39051010363169,-10.6219891796602));
#41670=CARTESIAN_POINT('Ctrl Pts',(-1.64481354069086,2.36765725371446,-10.6573878231682));
#41671=CARTESIAN_POINT('Ctrl Pts',(-1.3948379837133,2.34902750915391,-10.6859546344191));
#41672=CARTESIAN_POINT('Ctrl Pts',(-1.14305895590474,2.33494920718288,-10.7074846403153));
#41673=CARTESIAN_POINT('Ctrl Pts',(-1.05633093452868,2.33009978312676,-10.7149008847415));
#41674=CARTESIAN_POINT('Ctrl Pts',(-0.969389011244006,2.32579068746956,
-10.7214818557861));
#41675=CARTESIAN_POINT('Ctrl Pts',(-0.882249031691758,2.32203627246146,
-10.727218107575));
#41676=CARTESIAN_POINT('Ctrl Pts',(-0.625764048147959,2.31098564935461,
-10.7441020046476));
#41677=CARTESIAN_POINT('Ctrl Pts',(-0.367561507220804,2.30473871258826,
-10.7536705579575));
#41678=CARTESIAN_POINT('Ctrl Pts',(-0.108124721210384,2.30337804384068,
-10.7557538378253));
#41679=CARTESIAN_POINT('Ctrl Pts',(-0.0721012726907265,2.30318911157192,
-10.7560431064607));
#41680=CARTESIAN_POINT('Ctrl Pts',(-0.0360540656339076,2.30309442682546,
-10.7561879977457));
#41681=CARTESIAN_POINT('Ctrl Pts',(1.55675634620075E-5,2.30309424985344,
-10.7561879973148));
#41682=CARTESIAN_POINT('Ctrl Pts',(0.258123167549015,2.3030929834745,-10.7561879942312));
#41683=CARTESIAN_POINT('Ctrl Pts',(0.515061792059015,2.3078718503129,-10.7487843545561));
#41684=CARTESIAN_POINT('Ctrl Pts',(0.77037644122687,2.31739613540424,-10.7341395381072));
#41685=CARTESIAN_POINT('Ctrl Pts',(0.808742208416225,2.31882733610365,-10.7319388824838));
#41686=CARTESIAN_POINT('Ctrl Pts',(0.84707132814878,2.32036574238111,-10.7295746387273));
#41687=CARTESIAN_POINT('Ctrl Pts',(0.885362278207682,2.32201128975929,-10.7270472762613));
#41688=CARTESIAN_POINT('Ctrl Pts',(1.08656404905455,2.33065790328005,-10.7137671199067));
#41689=CARTESIAN_POINT('Ctrl Pts',(1.2867118663148,2.34226152640888,-10.6959845869193));
#41690=CARTESIAN_POINT('Ctrl Pts',(1.48561773745142,2.35667529156902,-10.6738045705339));
#41691=CARTESIAN_POINT('Ctrl Pts',(1.72995221186358,2.3743810521611,-10.6465588054139));
#41692=CARTESIAN_POINT('Ctrl Pts',(1.97240063589042,2.39636085514469,-10.6126717426014));
#41693=CARTESIAN_POINT('Ctrl Pts',(2.21261554862799,2.42228886661666,-10.5723239222172));
#41694=CARTESIAN_POINT('Ctrl Pts',(2.33272300499677,2.43525287235264,-10.5521500120251));
#41695=CARTESIAN_POINT('Ctrl Pts',(2.45227253079915,2.44920181630043,-10.5303609011959));
#41696=CARTESIAN_POINT('Ctrl Pts',(2.57122332400129,2.46408272756912,-10.5069791448595));
#41697=CARTESIAN_POINT('Ctrl Pts',(2.59887870385466,2.46754245442442,-10.5015430200913));
#41698=CARTESIAN_POINT('Ctrl Pts',(2.62650176530099,2.47105249563266,-10.4960208074496));
#41699=CARTESIAN_POINT('Ctrl Pts',(2.65409192553637,2.47461221620557,-10.4904127836425));
#41700=CARTESIAN_POINT('Ctrl Pts',(2.68583690121256,2.47870799680405,-10.4839602448451));
#41701=CARTESIAN_POINT('Ctrl Pts',(2.71753832026729,2.48286954562529,-10.4773941044017));
#41702=CARTESIAN_POINT('Ctrl Pts',(2.74919555557085,2.48709559038792,-10.4707148841878));
#41703=CARTESIAN_POINT('Ctrl Pts',(2.77878112492963,2.49104508058311,-10.4644727556189));
#41704=CARTESIAN_POINT('Ctrl Pts',(2.80832805715831,2.49505096219467,-10.4581318569174));
#41705=CARTESIAN_POINT('Ctrl Pts',(2.83783575611512,2.49911229294227,-10.4516926038457));
#41706=CARTESIAN_POINT('Ctrl Pts',(2.85258960559352,2.50114295831608,-10.4484729773099));
#41707=CARTESIAN_POINT('Ctrl Pts',(2.86733364675631,2.50318748596766,-10.4452287621483));
#41708=CARTESIAN_POINT('Ctrl Pts',(2.88206780592029,2.50524575524457,-10.441960010658));
#41709=CARTESIAN_POINT('Ctrl Pts',(2.89584461574247,2.50717028884539,-10.4389036457079));
#41710=CARTESIAN_POINT('Ctrl Pts',(2.90840992863005,2.5089366641677,-10.436096477744));
#41711=CARTESIAN_POINT('Ctrl Pts',(2.923137806357,2.51102209973565,-10.4327794102906));
#41712=CARTESIAN_POINT('Ctrl Pts',(2.92416124532654,2.51116701647575,-10.4325489075556));
#41713=CARTESIAN_POINT('Ctrl Pts',(2.92519512135964,2.51131348378967,-10.4323159249662));
#41714=CARTESIAN_POINT('Ctrl Pts',(2.92624056398715,2.51146166644494,-10.4320801995225));
#41715=CARTESIAN_POINT('Ctrl Pts',(3.13297121031788,2.54076398805763,-10.3854667632059));
#41716=CARTESIAN_POINT('Ctrl Pts',(3.33587866711728,2.57241886503027,-10.3344575226723));
#41717=CARTESIAN_POINT('Ctrl Pts',(3.53485207388181,2.60603621417604,-10.2794357398157));
#41718=CARTESIAN_POINT('Ctrl Pts',(3.73806256971372,2.64036943638673,-10.2232422818173));
#41719=CARTESIAN_POINT('Ctrl Pts',(3.93716971927397,2.67674968545062,-10.1628635658874));
#41720=CARTESIAN_POINT('Ctrl Pts',(4.13208039840941,2.71480311244308,-10.098683050252));
#41721=CARTESIAN_POINT('Ctrl Pts',(4.22656654105684,2.73325013416083,-10.0675704945808));
#41722=CARTESIAN_POINT('Ctrl Pts',(4.32006688591088,2.75209095923471,-10.0355641548993));
#41723=CARTESIAN_POINT('Ctrl Pts',(4.41257282447384,2.77128632053656,-10.0027056903117));
#41724=CARTESIAN_POINT('Ctrl Pts',(4.61058268702672,2.81237417837655,-9.93237182680255));
#41725=CARTESIAN_POINT('Ctrl Pts',(4.804035331853,2.85508378576198,-9.85813547086469));
#41726=CARTESIAN_POINT('Ctrl Pts',(4.9929108501,2.8990635906378,-9.78039118652011));
#41727=CARTESIAN_POINT('Ctrl Pts',(5.1857817011965,2.94397371173864,-9.70100235715463));
#41728=CARTESIAN_POINT('Ctrl Pts',(5.37387978343848,2.99020842254106,-9.61795560508356));
#41729=CARTESIAN_POINT('Ctrl Pts',(5.55720283873327,3.03743585162211,-9.53164303677593));
#41730=CARTESIAN_POINT('Ctrl Pts',(5.61189830411155,3.05152642090732,-9.50589119621235));
#41731=CARTESIAN_POINT('Ctrl Pts',(5.66616883817662,3.06570563505726,-9.47984846050826));
#41732=CARTESIAN_POINT('Ctrl Pts',(5.72001468712874,3.0799653729863,-9.45352477868309));
#41733=CARTESIAN_POINT('Ctrl Pts',(6.05078165618827,-4.09458887238873,-9.54443970746419));
#41734=CARTESIAN_POINT('Ctrl Pts',(6.0514309326576,-4.06997623068921,-9.55470507407486));
#41735=CARTESIAN_POINT('Ctrl Pts',(6.04719970398084,-4.00805739104224,-9.58290432047297));
#41736=CARTESIAN_POINT('Ctrl Pts',(6.01579032749343,-3.90976504771429,-9.63742351885017));
#41737=CARTESIAN_POINT('Ctrl Pts',(5.94768463712015,-3.81080368340423,-9.70642972249064));
#41738=CARTESIAN_POINT('Ctrl Pts',(5.84925760035456,-3.7329089217144,-9.77799616062866));
#41739=CARTESIAN_POINT('Ctrl Pts',(5.76422183048588,-3.69954275308194,-9.82519790048264));
#41740=CARTESIAN_POINT('Ctrl Pts',(5.71689747708232,-3.6892852770504,-9.84791207876869));
#41741=CARTESIAN_POINT('Ctrl Pts',(5.71188842785141,-3.68828725659104,-9.85027878928298));
#41742=CARTESIAN_POINT('Ctrl Pts',(5.9119338424872,-3.98202445464115,-9.28409234374272));
#41743=CARTESIAN_POINT('Ctrl Pts',(5.91252983174185,-3.959875089295,-9.29332121776031));
#41744=CARTESIAN_POINT('Ctrl Pts',(5.90864954675052,-3.90395398774346,-9.31884235613713));
#41745=CARTESIAN_POINT('Ctrl Pts',(5.87953897617286,-3.81456732430523,-9.36882529662082));
#41746=CARTESIAN_POINT('Ctrl Pts',(5.81605214418774,-3.72418838849228,-9.43267821318822));
#41747=CARTESIAN_POINT('Ctrl Pts',(5.72407864663328,-3.652997061284,-9.49923100425177));
#41748=CARTESIAN_POINT('Ctrl Pts',(5.64462215644559,-3.6226165199218,-9.54320383514445));
#41749=CARTESIAN_POINT('Ctrl Pts',(5.60046280975658,-3.61333517226186,-9.56435438307519));
#41750=CARTESIAN_POINT('Ctrl Pts',(5.59578948546033,-3.61243316965986,-9.5665580338794));
#41751=CARTESIAN_POINT('Ctrl Pts',(6.02851721676376,-3.8715554395682,-9.01218059937768));
#41752=CARTESIAN_POINT('Ctrl Pts',(6.02945192459048,-3.83742568340882,-9.02642167041017));
#41753=CARTESIAN_POINT('Ctrl Pts',(6.02333299803029,-3.7529376633562,-9.06490257042747));
#41754=CARTESIAN_POINT('Ctrl Pts',(5.98020755072705,-3.62309265216294,-9.13676063368903));
#41755=CARTESIAN_POINT('Ctrl Pts',(5.88943948424395,-3.4952859482716,-9.22561325181903));
#41756=CARTESIAN_POINT('Ctrl Pts',(5.75992263904637,-3.39562764242272,-9.31708718700472));
#41757=CARTESIAN_POINT('Ctrl Pts',(5.64799870728207,-3.35285012688804,-9.37787341286657));
#41758=CARTESIAN_POINT('Ctrl Pts',(5.58526054501384,-3.33966614696647,-9.40748009093418));
#41759=CARTESIAN_POINT('Ctrl Pts',(5.57861458744835,-3.33838322120361,-9.41056941987632));
#41760=CARTESIAN_POINT('Ctrl Pts',(6.32410045353725,-3.83560443861232,-8.90696767285684));
#41761=CARTESIAN_POINT('Ctrl Pts',(6.32554382421795,-3.78290488455112,-8.92898366934629));
#41762=CARTESIAN_POINT('Ctrl Pts',(6.31606430844593,-3.65401356063343,-8.98756587194144));
#41763=CARTESIAN_POINT('Ctrl Pts',(6.25179835610878,-3.46087038311676,-9.09336926176179));
#41764=CARTESIAN_POINT('Ctrl Pts',(6.11973434725635,-3.27416309711438,-9.22098494131091));
#41765=CARTESIAN_POINT('Ctrl Pts',(5.93329042167987,-3.1295301513967,-9.35097668483132));
#41766=CARTESIAN_POINT('Ctrl Pts',(5.77213775295316,-3.0671004297697,-9.4375958660983));
#41767=CARTESIAN_POINT('Ctrl Pts',(5.68125709334696,-3.0476935953827,-9.48013465539532));
#41768=CARTESIAN_POINT('Ctrl Pts',(5.67162338877499,-3.04580253600233,-9.48457775597017));
#41769=CARTESIAN_POINT('',(5.73278595301787,-3.68906554369663,-9.815438227342));
#41770=CARTESIAN_POINT('',(5.7200159288464,-3.07996626094983,-9.45352720243893));
#41771=CARTESIAN_POINT('Origin',(5.89875613670428,-3.22462513219392,-9.8974987073781));
#41772=CARTESIAN_POINT('',(5.99999998876135,-3.2142420670336,-9.29218347180064));
#41773=CARTESIAN_POINT('Ctrl Pts',(6.00000005573716,-3.21424213478534,-9.29218366766699));
#41774=CARTESIAN_POINT('Ctrl Pts',(5.95912832913167,-3.18371657550664,-9.32023732779621));
#41775=CARTESIAN_POINT('Ctrl Pts',(5.91539006756828,-3.15723896628417,-9.34768031862321));
#41776=CARTESIAN_POINT('Ctrl Pts',(5.86875892973,-3.13478493225045,-9.37457511033737));
#41777=CARTESIAN_POINT('Ctrl Pts',(5.82212779189173,-3.11233089821673,-9.40146990205153));
#41778=CARTESIAN_POINT('Ctrl Pts',(5.77260355260912,-3.09390025876082,-9.42781596698812));
#41779=CARTESIAN_POINT('Ctrl Pts',(5.72001606108407,-3.07996636795448,-9.45352753089058));
#41780=CARTESIAN_POINT('',(5.99998733812332,-3.99788407449396,-9.34660788725514));
#41781=CARTESIAN_POINT('Ctrl Pts',(5.99998733812332,-3.99788407449396,-9.34660788725514));
#41782=CARTESIAN_POINT('Ctrl Pts',(5.99998488596604,-3.97180407808845,-9.3357140563781));
#41783=CARTESIAN_POINT('Ctrl Pts',(5.9999858305139,-3.94582833044417,-9.3256565521199));
#41784=CARTESIAN_POINT('Ctrl Pts',(5.99998224149706,-3.91995848301427,-9.31646864591698));
#41785=CARTESIAN_POINT('Ctrl Pts',(5.99998112254582,-3.91189301572182,-9.3136041235356));
#41786=CARTESIAN_POINT('Ctrl Pts',(5.99997934669105,-3.90383796951955,-9.310823799426));
#41787=CARTESIAN_POINT('Ctrl Pts',(5.99997632633964,-3.89579365835037,-9.30812785308905));
#41788=CARTESIAN_POINT('Ctrl Pts',(5.99996219472167,-3.85815594109312,-9.29551406132529));
#41789=CARTESIAN_POINT('Ctrl Pts',(5.99992491129164,-3.82075549376394,-9.28475071122847));
#41790=CARTESIAN_POINT('Ctrl Pts',(5.99991412123476,-3.78357059890767,-9.27578193406091));
#41791=CARTESIAN_POINT('Ctrl Pts',(5.99990486207759,-3.75166151908597,-9.26808565234089));
#41792=CARTESIAN_POINT('Ctrl Pts',(5.99990277981739,-3.71991114528791,-9.26173564795763));
#41793=CARTESIAN_POINT('Ctrl Pts',(5.99990414412111,-3.68833374065537,-9.25673100183795));
#41794=CARTESIAN_POINT('Ctrl Pts',(5.99990504451532,-3.6674937238673,-9.25342810502404));
#41795=CARTESIAN_POINT('Ctrl Pts',(5.99990781486193,-3.64672846175442,-9.250710922078));
#41796=CARTESIAN_POINT('Ctrl Pts',(5.99991537550728,-3.6260312685207,-9.24858454831112));
#41797=CARTESIAN_POINT('Ctrl Pts',(5.99991828174551,-3.61807546957057,-9.24776719100131));
#41798=CARTESIAN_POINT('Ctrl Pts',(5.99992634338063,-3.60986023920379,-9.24700690180229));
#41799=CARTESIAN_POINT('Ctrl Pts',(5.99993169908744,-3.60175447189294,-9.2463532514576));
#41800=CARTESIAN_POINT('Ctrl Pts',(5.99993712301145,-3.59354545904762,-9.24569127537686));
#41801=CARTESIAN_POINT('Ctrl Pts',(5.99993949878579,-3.58544904623269,-9.24513871128581));
#41802=CARTESIAN_POINT('Ctrl Pts',(5.99994451384018,-3.57786438072415,-9.24469668443833));
#41803=CARTESIAN_POINT('Ctrl Pts',(5.99994534777804,-3.57660315019569,-9.24462318116336));
#41804=CARTESIAN_POINT('Ctrl Pts',(5.99994628951504,-3.57535609798006,-9.24455262588208));
#41805=CARTESIAN_POINT('Ctrl Pts',(5.99994740674549,-3.57412508935423,-9.24448489874969));
#41806=CARTESIAN_POINT('Ctrl Pts',(5.9999742135278,-3.54458831805716,-9.24285985666782));
#41807=CARTESIAN_POINT('Ctrl Pts',(5.99996031027524,-3.51545847374159,-9.24253337306945));
#41808=CARTESIAN_POINT('Ctrl Pts',(5.99993575361401,-3.48674310711012,-9.24342493463139));
#41809=CARTESIAN_POINT('Ctrl Pts',(5.99991415256481,-3.46148388960773,-9.24420918884966));
#41810=CARTESIAN_POINT('Ctrl Pts',(5.99988537901417,-3.43654429589967,-9.24593621729577));
#41811=CARTESIAN_POINT('Ctrl Pts',(5.99986870330864,-3.41191858348489,-9.2485831616114));
#41812=CARTESIAN_POINT('Ctrl Pts',(5.99985078225209,-3.38545380908684,-9.25142778120972));
#41813=CARTESIAN_POINT('Ctrl Pts',(5.99984832471424,-3.35935020724328,-9.25533463258301));
#41814=CARTESIAN_POINT('Ctrl Pts',(5.99986773243008,-3.33359881707214,-9.26031735681989));
#41815=CARTESIAN_POINT('Ctrl Pts',(5.99988654285589,-3.30863994925345,-9.26514673320612));
#41816=CARTESIAN_POINT('Ctrl Pts',(5.99992646290735,-3.28401122807348,-9.2709876518158));
#41817=CARTESIAN_POINT('Ctrl Pts',(5.99996032824771,-3.25972320748426,-9.27788278843555));
#41818=CARTESIAN_POINT('Ctrl Pts',(5.99998165966428,-3.24442444245233,-9.28222596142575));
#41819=CARTESIAN_POINT('Ctrl Pts',(5.99999988603535,-3.22926128485911,-9.28698799135304));
#41820=CARTESIAN_POINT('Ctrl Pts',(5.99999989033238,-3.21424200111748,-9.29218328124107));
#41821=CARTESIAN_POINT('Ctrl Pts',(5.99998733812332,-3.99788407449396,-9.34660788725514));
#41822=CARTESIAN_POINT('Ctrl Pts',(5.99998442648227,-3.98506455951682,-9.35725069887637));
#41823=CARTESIAN_POINT('Ctrl Pts',(5.99923934431779,-3.97175114978455,-9.36889665012024));
#41824=CARTESIAN_POINT('Ctrl Pts',(5.99754757095219,-3.9580775449888,-9.38156938257316));
#41825=CARTESIAN_POINT('Ctrl Pts',(5.99683713707804,-3.95233552763226,-9.38689109917871));
#41826=CARTESIAN_POINT('Ctrl Pts',(5.99595953918619,-3.94653051018614,-9.392393686159));
#41827=CARTESIAN_POINT('Ctrl Pts',(5.99489848361549,-3.94067479526504,-9.39807799691719));
#41828=CARTESIAN_POINT('Ctrl Pts',(5.99250382409841,-3.92745923535258,-9.41090672071916));
#41829=CARTESIAN_POINT('Ctrl Pts',(5.98917443765327,-3.91398268590984,-9.42466279085472));
#41830=CARTESIAN_POINT('Ctrl Pts',(5.98476532291861,-3.90040413868406,-9.4393294105634));
#41831=CARTESIAN_POINT('Ctrl Pts',(5.98056462641809,-3.88746744747819,-9.45330274121877));
#41832=CARTESIAN_POINT('Ctrl Pts',(5.97538423138413,-3.87443775181405,-9.46810266737493));
#41833=CARTESIAN_POINT('Ctrl Pts',(5.96909466645958,-3.86149238497048,-9.48369242079305));
#41834=CARTESIAN_POINT('Ctrl Pts',(5.96741551873607,-3.85803631391848,-9.48785447322056));
#41835=CARTESIAN_POINT('Ctrl Pts',(5.96565727348637,-3.85458649918978,-9.49207268886684));
#41836=CARTESIAN_POINT('Ctrl Pts',(5.96381735718526,-3.85114688309128,-9.49634606941855));
#41837=CARTESIAN_POINT('Ctrl Pts',(5.96351328401592,-3.850578436055,-9.49705230826613));
#41838=CARTESIAN_POINT('Ctrl Pts',(5.96320698007237,-3.85001026815408,-9.49776005350371));
#41839=CARTESIAN_POINT('Ctrl Pts',(5.96289843783564,-3.84944239465364,-9.49846930029565));
#41840=CARTESIAN_POINT('Ctrl Pts',(5.95831416539658,-3.84100501873863,-9.50900717853002));
#41841=CARTESIAN_POINT('Ctrl Pts',(5.95323565980044,-3.83263199254864,-9.51987698043347));
#41842=CARTESIAN_POINT('Ctrl Pts',(5.94763907818266,-3.82437747432279,-9.53105996212404));
#41843=CARTESIAN_POINT('Ctrl Pts',(5.94484078737377,-3.82025021520986,-9.53665145296933));
#41844=CARTESIAN_POINT('Ctrl Pts',(5.94191293623144,-3.81615260702795,-9.5423212351393));
#41845=CARTESIAN_POINT('Ctrl Pts',(5.93885272790819,-3.81209232950736,-9.54806633546841));
#41846=CARTESIAN_POINT('Ctrl Pts',(5.93732262374657,-3.81006219074706,-9.55093888563297));
#41847=CARTESIAN_POINT('Ctrl Pts',(5.93575942704362,-3.8080413864398,-9.55383026506808));
#41848=CARTESIAN_POINT('Ctrl Pts',(5.93416278454396,-3.80603091718481,-9.55674007844489));
#41849=CARTESIAN_POINT('Ctrl Pts',(5.9330991746773,-3.8046916349493,-9.55867846240898));
#41850=CARTESIAN_POINT('Ctrl Pts',(5.93175171859144,-3.80302652765125,-9.56110924344933));
#41851=CARTESIAN_POINT('Ctrl Pts',(5.93065599743354,-3.80169767257101,-9.56306466655013));
#41852=CARTESIAN_POINT('Ctrl Pts',(5.93010687208962,-3.80103171116496,-9.56404463519907));
#41853=CARTESIAN_POINT('Ctrl Pts',(5.92962186463968,-3.80044952661347,-9.56490518456632));
#41854=CARTESIAN_POINT('Ctrl Pts',(5.92927215875649,-3.80003154015743,-9.56552441212107));
#41855=CARTESIAN_POINT('Ctrl Pts',(5.92326911397194,-3.79285639231029,-9.57615406098208));
#41856=CARTESIAN_POINT('Ctrl Pts',(5.91647655577503,-3.78540876595849,-9.58765163498892));
#41857=CARTESIAN_POINT('Ctrl Pts',(5.90875553078948,-3.77785188769607,-9.59998916486729));
#41858=CARTESIAN_POINT('Ctrl Pts',(5.90763524385544,-3.77675541773316,-9.60177928645697));
#41859=CARTESIAN_POINT('Ctrl Pts',(5.9064953972911,-3.77565672763503,-9.60358705241849));
#41860=CARTESIAN_POINT('Ctrl Pts',(5.90533555419657,-3.77455640091975,-9.60541233540429));
#41861=CARTESIAN_POINT('Ctrl Pts',(5.89751903312143,-3.76714097809225,-9.61771345009286));
#41862=CARTESIAN_POINT('Ctrl Pts',(5.88879369601463,-3.75964795878791,-9.63081225330071));
#41863=CARTESIAN_POINT('Ctrl Pts',(5.87904237408387,-3.75226213629508,-9.64465846120265));
#41864=CARTESIAN_POINT('Ctrl Pts',(5.87007096184807,-3.74546703110276,-9.65739725086347));
#41865=CARTESIAN_POINT('Ctrl Pts',(5.86023095512446,-3.73876252446447,-9.67076877328719));
#41866=CARTESIAN_POINT('Ctrl Pts',(5.8494388689441,-3.73232780646497,-9.68471105146388));
#41867=CARTESIAN_POINT('Ctrl Pts',(5.84101794142072,-3.72730687788807,-9.6955900337176));
#41868=CARTESIAN_POINT('Ctrl Pts',(5.83201744822162,-3.72245074407605,-9.70681616103984));
#41869=CARTESIAN_POINT('Ctrl Pts',(5.82240240038839,-3.71786284377927,-9.71834822089586));
#41870=CARTESIAN_POINT('Ctrl Pts',(5.8105783876476,-3.71222091744633,-9.73252966076286));
#41871=CARTESIAN_POINT('Ctrl Pts',(5.79782361947076,-3.70698410220008,-9.74717460361531));
#41872=CARTESIAN_POINT('Ctrl Pts',(5.78410757713597,-3.70234957630206,-9.76218794847119));
#41873=CARTESIAN_POINT('Ctrl Pts',(5.77126455919935,-3.69801003740423,-9.77624569578389));
#41874=CARTESIAN_POINT('Ctrl Pts',(5.75757862353476,-3.69419833069783,-9.79062652340357));
#41875=CARTESIAN_POINT('Ctrl Pts',(5.74304692965124,-3.69110834401341,-9.80522706601143));
#41876=CARTESIAN_POINT('Ctrl Pts',(5.73967098514949,-3.69039049077199,-9.80861900517109));
#41877=CARTESIAN_POINT('Ctrl Pts',(5.73624949911788,-3.6897117421629,-9.81202268530853));
#41878=CARTESIAN_POINT('Ctrl Pts',(5.73278263502695,-3.68907482142868,-9.81543658880499));
#41879=CARTESIAN_POINT('Ctrl Pts',(5.99928507671105,-9.77920217853695,-17.0543525004093));
#41880=CARTESIAN_POINT('Ctrl Pts',(5.99928507671105,-9.74894839965409,-17.0407709830188));
#41881=CARTESIAN_POINT('Ctrl Pts',(5.99928507671105,-9.27203920734991,-16.8237867818301));
#41882=CARTESIAN_POINT('Ctrl Pts',(5.99928507671105,-8.38193522942945,-16.3303542912131));
#41883=CARTESIAN_POINT('Ctrl Pts',(5.99928507671105,-7.21246426312353,-15.4323267873847));
#41884=CARTESIAN_POINT('Ctrl Pts',(5.99928507671105,-6.18849730658614,-14.3709116157454));
#41885=CARTESIAN_POINT('Ctrl Pts',(5.99928507671105,-5.33271053138996,-13.1688951809494));
#41886=CARTESIAN_POINT('Ctrl Pts',(5.99928507671105,-4.66383020185381,-11.8527237226987));
#41887=CARTESIAN_POINT('Ctrl Pts',(5.99928507671105,-4.22479091101948,-10.5321726316834));
#41888=CARTESIAN_POINT('Ctrl Pts',(5.99928507671105,-4.05899861709883,-9.64833292798501));
#41889=CARTESIAN_POINT('Ctrl Pts',(5.99928507671105,-4.00882230477428,-9.24471639752991));
#41890=CARTESIAN_POINT('Ctrl Pts',(6.01063076682066,-9.70160365670749,-17.2272481798314));
#41891=CARTESIAN_POINT('Ctrl Pts',(6.01063076682066,-9.67076859172804,-17.2134055071903));
#41892=CARTESIAN_POINT('Ctrl Pts',(6.01063076682066,-9.18470271755529,-16.9922531320754));
#41893=CARTESIAN_POINT('Ctrl Pts',(6.01063076682066,-8.27768704363521,-16.4894545190853));
#41894=CARTESIAN_POINT('Ctrl Pts',(6.01063076682066,-7.08568152473405,-15.5741206058228));
#41895=CARTESIAN_POINT('Ctrl Pts',(6.01063076682066,-6.04222139176158,-14.4924942432127));
#41896=CARTESIAN_POINT('Ctrl Pts',(6.01063076682066,-5.16996888347368,-13.2673642990713));
#41897=CARTESIAN_POINT('Ctrl Pts',(6.01063076682066,-4.48832934805044,-11.9260686457922));
#41898=CARTESIAN_POINT('Ctrl Pts',(6.01063076682066,-4.04084801205732,-10.5801430309673));
#41899=CARTESIAN_POINT('Ctrl Pts',(6.01063076682066,-3.87189820410474,-9.67946904936188));
#41900=CARTESIAN_POINT('Ctrl Pts',(6.01063076682066,-3.82075861600654,-9.26809120543838));
#41901=CARTESIAN_POINT('Ctrl Pts',(5.90351705923382,-9.63722444731814,-17.3706901795732));
#41902=CARTESIAN_POINT('Ctrl Pts',(5.90351705923382,-9.60590712136365,-17.3566308408348));
#41903=CARTESIAN_POINT('Ctrl Pts',(5.90351705923382,-9.11224445377126,-17.1320203619313));
#41904=CARTESIAN_POINT('Ctrl Pts',(5.90351705923382,-8.19119807937274,-16.6214511943171));
#41905=CARTESIAN_POINT('Ctrl Pts',(5.90351705923382,-6.98049688630115,-15.6917591086185));
#41906=CARTESIAN_POINT('Ctrl Pts',(5.90351705923382,-5.92086434104531,-14.5933646367085));
#41907=CARTESIAN_POINT('Ctrl Pts',(5.90351705923382,-5.03495112308005,-13.3490586899501));
#41908=CARTESIAN_POINT('Ctrl Pts',(5.90351705923382,-4.34272597895849,-11.9869188791486));
#41909=CARTESIAN_POINT('Ctrl Pts',(5.90351705923382,-3.88824074417813,-10.6199414228328));
#41910=CARTESIAN_POINT('Ctrl Pts',(5.90351705923382,-3.71667132115728,-9.70530097025956));
#41911=CARTESIAN_POINT('Ctrl Pts',(5.90351705923382,-3.66473255633256,-9.28748399304876));
#41912=CARTESIAN_POINT('Ctrl Pts',(5.7219541158257,-9.61342486666327,-17.4237175384707));
#41913=CARTESIAN_POINT('Ctrl Pts',(5.7219541158257,-9.58192925940845,-17.4095781030297));
#41914=CARTESIAN_POINT('Ctrl Pts',(5.7219541158257,-9.08545822403752,-17.1836892390603));
#41915=CARTESIAN_POINT('Ctrl Pts',(5.7219541158257,-8.1592250076253,-16.670247467953));
#41916=CARTESIAN_POINT('Ctrl Pts',(5.7219541158257,-6.94161243417266,-15.7352474810556));
#41917=CARTESIAN_POINT('Ctrl Pts',(5.7219541158257,-5.87600130305989,-14.6306542071787));
#41918=CARTESIAN_POINT('Ctrl Pts',(5.7219541158257,-4.98503802057335,-13.3792593131512));
#41919=CARTESIAN_POINT('Ctrl Pts',(5.7219541158257,-4.28889960925415,-12.0094138748187));
#41920=CARTESIAN_POINT('Ctrl Pts',(5.7219541158257,-3.83182518682086,-10.6346540147708));
#41921=CARTESIAN_POINT('Ctrl Pts',(5.7219541158257,-3.6592873496071,-9.71485046443014));
#41922=CARTESIAN_POINT('Ctrl Pts',(5.7219541158257,-3.60705314668704,-9.29465308097585));
#41923=CARTESIAN_POINT('',(6.,-9.67863108609234,-17.0348569101268));
#41924=CARTESIAN_POINT('Ctrl Pts',(5.99999999999975,-9.67863108609234,-17.0348569101268));
#41925=CARTESIAN_POINT('Ctrl Pts',(5.99999999999975,-9.53996482698304,-16.9709229523293));
#41926=CARTESIAN_POINT('Ctrl Pts',(6.00000000003748,-9.40322990798227,-16.9040238345894));
#41927=CARTESIAN_POINT('Ctrl Pts',(5.99999999795225,-9.26832001841028,-16.8341585314232));
#41928=CARTESIAN_POINT('Ctrl Pts',(5.9999999958601,-9.13296247356695,-16.7640614026188));
#41929=CARTESIAN_POINT('Ctrl Pts',(5.99999999148619,-8.99944169515712,-16.6909781287944));
#41930=CARTESIAN_POINT('Ctrl Pts',(5.9999999908736,-8.86767321980464,-16.6148604837069));
#41931=CARTESIAN_POINT('Ctrl Pts',(5.999999990262,-8.73611954092696,-16.5388669183872));
#41932=CARTESIAN_POINT('Ctrl Pts',(5.99999999695627,-8.60631206866638,-16.4598486138675));
#41933=CARTESIAN_POINT('Ctrl Pts',(5.99999999953315,-8.47819538354683,-16.3777143843573));
#41934=CARTESIAN_POINT('Ctrl Pts',(5.99999999982105,-8.46388161375179,-16.368537980422));
#41935=CARTESIAN_POINT('Ctrl Pts',(5.99999999999975,-8.44958898201702,-16.3593226402141));
#41936=CARTESIAN_POINT('Ctrl Pts',(5.99999999999975,-8.43531743665977,-16.3500682051006));
#41937=CARTESIAN_POINT('Ctrl Pts',(5.99999999999975,-8.41951507644074,-16.3398211075631));
#41938=CARTESIAN_POINT('Ctrl Pts',(5.99999999977976,-8.40373799579059,-16.3295268932043));
#41939=CARTESIAN_POINT('Ctrl Pts',(5.99999999940213,-8.38798676299647,-16.3191857879626));
#41940=CARTESIAN_POINT('Ctrl Pts',(5.99999999572735,-8.23470703684241,-16.218553551725));
#41941=CARTESIAN_POINT('Ctrl Pts',(5.99999998184258,-8.08387696921227,-16.1134769902152));
#41942=CARTESIAN_POINT('Ctrl Pts',(5.99999998033336,-7.93593246474559,-16.0042029928214));
#41943=CARTESIAN_POINT('Ctrl Pts',(5.99999997882273,-7.78785045817077,-15.8948274343386));
#41944=CARTESIAN_POINT('Ctrl Pts',(5.99999998731005,-7.64265976297581,-15.7812468735922));
#41945=CARTESIAN_POINT('Ctrl Pts',(5.99999999411987,-7.50077077039805,-15.6637536647744));
#41946=CARTESIAN_POINT('Ctrl Pts',(5.99999999739303,-7.43257160183055,-15.6072803682337));
#41947=CARTESIAN_POINT('Ctrl Pts',(5.99999999999975,-7.36513478079692,-15.5499037886234));
#41948=CARTESIAN_POINT('Ctrl Pts',(5.99999999999975,-7.2985032883994,-15.4916598064485));
#41949=CARTESIAN_POINT('Ctrl Pts',(5.99999999999975,-7.27238327152466,-15.4688277529776));
#41950=CARTESIAN_POINT('Ctrl Pts',(5.99999999960415,-7.24638785264023,-15.4458614503158));
#41951=CARTESIAN_POINT('Ctrl Pts',(5.99999999898866,-7.22051776537586,-15.4227616312456));
#41952=CARTESIAN_POINT('Ctrl Pts',(5.99999999507861,-7.05617055376858,-15.2760133495707));
#41953=CARTESIAN_POINT('Ctrl Pts',(5.99999998615656,-6.89687872218188,-15.1238800776715));
#41954=CARTESIAN_POINT('Ctrl Pts',(5.99999998771985,-6.74283048209707,-14.9666009211883));
#41955=CARTESIAN_POINT('Ctrl Pts',(5.99999998928315,-6.58878224201225,-14.8093217647052));
#41956=CARTESIAN_POINT('Ctrl Pts',(5.99999999999975,-6.43997714680681,-14.6468962856083));
#41957=CARTESIAN_POINT('Ctrl Pts',(5.99999999999975,-6.29664110038409,-14.4795249794017));
#41958=CARTESIAN_POINT('Ctrl Pts',(5.99999999999975,-6.26385436913173,-14.4412404154493));
#41959=CARTESIAN_POINT('Ctrl Pts',(5.9999999993467,-6.23135170199723,-14.4026986427207));
#41960=CARTESIAN_POINT('Ctrl Pts',(5.99999999845574,-6.19913907434213,-14.3639052805569));
#41961=CARTESIAN_POINT('Ctrl Pts',(5.99999999449763,-6.05603309707375,-14.1915641085351));
#41962=CARTESIAN_POINT('Ctrl Pts',(5.99999998895133,-5.91865446098742,-14.0142547234861));
#41963=CARTESIAN_POINT('Ctrl Pts',(5.99999999115154,-5.78742187725139,-13.8325315580029));
#41964=CARTESIAN_POINT('Ctrl Pts',(5.99999999312721,-5.6695821336787,-13.6693540100791));
#41965=CARTESIAN_POINT('Ctrl Pts',(5.99999999999975,-5.55669768554855,-13.5026183338488));
#41966=CARTESIAN_POINT('Ctrl Pts',(5.99999999999975,-5.44904317682204,-13.3327476292645));
#41967=CARTESIAN_POINT('Ctrl Pts',(5.99999999999975,-5.41325256682299,-13.2762727429828));
#41968=CARTESIAN_POINT('Ctrl Pts',(5.99999999913628,-5.3780422672377,-13.219450528623));
#41969=CARTESIAN_POINT('Ctrl Pts',(5.99999999780775,-5.34341678808511,-13.1622879102247));
#41970=CARTESIAN_POINT('Ctrl Pts',(5.99999999336883,-5.22772507034453,-12.9712944084768));
#41971=CARTESIAN_POINT('Ctrl Pts',(5.99999998477715,-5.11855861803619,-12.7765024093267));
#41972=CARTESIAN_POINT('Ctrl Pts',(5.99999998688354,-5.01608477796987,-12.5781968539945));
#41973=CARTESIAN_POINT('Ctrl Pts',(5.99999998863009,-4.93111681469402,-12.4137683605179));
#41974=CARTESIAN_POINT('Ctrl Pts',(5.99999999999975,-4.85075089132226,-12.2469236105177));
#41975=CARTESIAN_POINT('Ctrl Pts',(5.99999999999975,-4.77510784589638,-12.0778154581411));
#41976=CARTESIAN_POINT('Ctrl Pts',(5.99999999999975,-4.74092204835261,-12.001389436058));
#41977=CARTESIAN_POINT('Ctrl Pts',(5.99999999683355,-4.70768988233596,-11.9245038096418));
#41978=CARTESIAN_POINT('Ctrl Pts',(5.99999999319076,-4.67543337998466,-11.8471991538661));
#41979=CARTESIAN_POINT('Ctrl Pts',(5.99999998466668,-4.59995360841341,-11.6663073232581));
#41980=CARTESIAN_POINT('Ctrl Pts',(5.99999997595979,-4.52981981238297,-11.483119818371));
#41981=CARTESIAN_POINT('Ctrl Pts',(5.99999997954455,-4.46519569756246,-11.298180586888));
#41982=CARTESIAN_POINT('Ctrl Pts',(5.9999999831293,-4.40057158274195,-11.1132413554049));
#41983=CARTESIAN_POINT('Ctrl Pts',(5.99999999999975,-4.34145727180482,-10.9265509189464));
#41984=CARTESIAN_POINT('Ctrl Pts',(5.99999999999975,-4.28796151252698,-10.7386680750688));
#41985=CARTESIAN_POINT('Ctrl Pts',(5.99999999999975,-4.26062856773402,-10.6426718415621));
#41986=CARTESIAN_POINT('Ctrl Pts',(5.99999999545169,-4.23478514967344,-10.5463642320482));
#41987=CARTESIAN_POINT('Ctrl Pts',(5.99999999307294,-4.21041230415808,-10.4497165385558));
#41988=CARTESIAN_POINT('Ctrl Pts',(5.9999999894094,-4.17287556932914,-10.3008689680017));
#41989=CARTESIAN_POINT('Ctrl Pts',(5.99999999031163,-4.13882446525617,-10.1512153093438));
#41990=CARTESIAN_POINT('Ctrl Pts',(5.99999999276244,-4.10822755624092,-10.0006714392445));
#41991=CARTESIAN_POINT('Ctrl Pts',(5.99999999520029,-4.07779233417733,-9.85092310634911));
#41992=CARTESIAN_POINT('Ctrl Pts',(5.99999999786784,-4.05077479923683,-9.70029349478971));
#41993=CARTESIAN_POINT('Ctrl Pts',(5.99999999875695,-4.02719432983824,-9.54868945835378));
#41994=CARTESIAN_POINT('Ctrl Pts',(5.99999999915085,-4.01674728362348,-9.48152309502914));
#41995=CARTESIAN_POINT('Ctrl Pts',(5.99999999931877,-4.00697554670158,-9.41416537293925));
#41996=CARTESIAN_POINT('Ctrl Pts',(5.99999999931449,-3.99788407308631,-9.34660788817994));
#41997=CARTESIAN_POINT('',(5.73644276520394,-9.5212169767595,-17.3763304373435));
#41998=CARTESIAN_POINT('Origin',(5.6,-9.67863108603356,-17.0348569100686));
#41999=CARTESIAN_POINT('Ctrl Pts',(5.73644276397727,-9.52121697613054,-17.3763304378314));
#42000=CARTESIAN_POINT('Ctrl Pts',(5.7370879225765,-9.11866915060707,-17.190470746701));
#42001=CARTESIAN_POINT('Ctrl Pts',(5.73762563119994,-8.7282103260932,-16.9787094510485));
#42002=CARTESIAN_POINT('Ctrl Pts',(5.73805595553824,-8.35333654529934,-16.7430677114181));
#42003=CARTESIAN_POINT('Ctrl Pts',(5.73812189681658,-8.29589230121891,-16.7069588601183));
#42004=CARTESIAN_POINT('Ctrl Pts',(5.73818531654628,-8.23881393095504,-16.6702892103096));
#42005=CARTESIAN_POINT('Ctrl Pts',(5.73824621493434,-8.18211392296719,-16.6330659762319));
#42006=CARTESIAN_POINT('Ctrl Pts',(5.73865147315426,-7.80479450550312,-16.3853579159207));
#42007=CARTESIAN_POINT('Ctrl Pts',(5.73894507726364,-7.44423378224291,-16.1131375843732));
#42008=CARTESIAN_POINT('Ctrl Pts',(5.73912707307373,-7.10336499304846,-15.8189084157108));
#42009=CARTESIAN_POINT('Ctrl Pts',(5.73915087281185,-7.05878930797042,-15.7804318312336));
#42010=CARTESIAN_POINT('Ctrl Pts',(5.7391727638931,-7.01455032175002,-15.7415788234522));
#42011=CARTESIAN_POINT('Ctrl Pts',(5.73919274637924,-6.97065454662951,-15.7023549458821));
#42012=CARTESIAN_POINT('Ctrl Pts',(5.73934700322017,-6.631796631049,-15.3995622202062));
#42013=CARTESIAN_POINT('Ctrl Pts',(5.73938752573454,-6.31339406649295,-15.0746719077206));
#42014=CARTESIAN_POINT('Ctrl Pts',(5.73931432084042,-6.01802942968551,-14.730631055353));
#42015=CARTESIAN_POINT('Ctrl Pts',(5.73930537005946,-5.98191512067613,-14.688565093129));
#42016=CARTESIAN_POINT('Ctrl Pts',(5.7392947190043,-5.94614518966932,-14.6462127796561));
#42017=CARTESIAN_POINT('Ctrl Pts',(5.73928236764773,-5.91072432463659,-14.6035794599369));
#42018=CARTESIAN_POINT('Ctrl Pts',(5.73918135756739,-5.62105052227199,-14.2549218023928));
#42019=CARTESIAN_POINT('Ctrl Pts',(5.73896663323084,-5.35472450905668,-13.887474076343));
#42020=CARTESIAN_POINT('Ctrl Pts',(5.73863815928527,-5.11384103203013,-13.5046257092083));
#42021=CARTESIAN_POINT('Ctrl Pts',(5.73859603612378,-5.08295038228288,-13.4555296277275));
#42022=CARTESIAN_POINT('Ctrl Pts',(5.73855204227779,-5.05247810754861,-13.4061802174161));
#42023=CARTESIAN_POINT('Ctrl Pts',(5.73850617763449,-5.02242859617607,-13.3565845722254));
#42024=CARTESIAN_POINT('Ctrl Pts',(5.73815298350166,-4.79102352361814,-12.9746587654586));
#42025=CARTESIAN_POINT('Ctrl Pts',(5.73768884852362,-4.58469079413331,-12.5781343505374));
#42026=CARTESIAN_POINT('Ctrl Pts',(5.73711370889819,-4.40507707959883,-12.170380536125));
#42027=CARTESIAN_POINT('Ctrl Pts',(5.7370302059657,-4.37899946085101,-12.1111798868718));
#42028=CARTESIAN_POINT('Ctrl Pts',(5.73694436290758,-4.35348502742357,-12.0517424499186));
#42029=CARTESIAN_POINT('Ctrl Pts',(5.73685617955183,-4.32853878640423,-11.992078459459));
#42030=CARTESIAN_POINT('Ctrl Pts',(5.73622835025684,-4.15093179040852,-11.5672953385699));
#42031=CARTESIAN_POINT('Ctrl Pts',(5.73548189400739,-4.0021263642364,-11.1310327750241));
#42032=CARTESIAN_POINT('Ctrl Pts',(5.73461675057501,-3.8830427836656,-10.6872506417479));
#42033=CARTESIAN_POINT('Ctrl Pts',(5.73452239358223,-3.87005491583734,-10.6388494796069));
#42034=CARTESIAN_POINT('Ctrl Pts',(5.73442662479487,-3.85742058667043,-10.5903588204422));
#42035=CARTESIAN_POINT('Ctrl Pts',(5.73432944414849,-3.84514098364243,-10.5417837649701));
#42036=CARTESIAN_POINT('Ctrl Pts',(5.73384873086919,-3.78439876325035,-10.3015026485271));
#42037=CARTESIAN_POINT('Ctrl Pts',(5.73333347080855,-3.73233631768364,-10.0591568647339));
#42038=CARTESIAN_POINT('Ctrl Pts',(5.73278365810998,-3.68907196542854,-9.81543709296658));
#42039=CARTESIAN_POINT('Ctrl Pts',(5.99999999997498,-9.91330135657868,-16.8993650110575));
#42040=CARTESIAN_POINT('Ctrl Pts',(5.99999999997498,-9.8352288888744,-16.9447895967214));
#42041=CARTESIAN_POINT('Ctrl Pts',(5.99999999997498,-9.75700380943188,-16.9899528783353));
#42042=CARTESIAN_POINT('Ctrl Pts',(5.99999999997498,-9.67862816205492,-17.0348534691251));
#42043=CARTESIAN_POINT('Ctrl Pts',(6.00000263486244,-10.0326958051699,-17.1045706743814));
#42044=CARTESIAN_POINT('Ctrl Pts',(6.00000263486244,-9.95416474484388,-17.150262077563));
#42045=CARTESIAN_POINT('Ctrl Pts',(6.00000263486244,-9.87548026973954,-17.195690591635));
#42046=CARTESIAN_POINT('Ctrl Pts',(6.00000263486244,-9.79664425061344,-17.2408549245712));
#42047=CARTESIAN_POINT('Ctrl Pts',(5.83074066841652,-10.116417534179,-17.2484649101534));
#42048=CARTESIAN_POINT('Ctrl Pts',(5.83074066841652,-10.0375648997125,-17.2943434110118));
#42049=CARTESIAN_POINT('Ctrl Pts',(5.83074066841652,-9.95855828736023,-17.3399579112862));
#42050=CARTESIAN_POINT('Ctrl Pts',(5.83074066841652,-9.87939944653079,-17.3853071853881));
#42051=CARTESIAN_POINT('Ctrl Pts',(5.59336110044025,-10.1144359114731,-17.2450590549679));
#42052=CARTESIAN_POINT('Ctrl Pts',(5.59336110044025,-10.0355908883964,-17.2909331273821));
#42053=CARTESIAN_POINT('Ctrl Pts',(5.59336110044025,-9.95659190076218,-17.3365432255193));
#42054=CARTESIAN_POINT('Ctrl Pts',(5.59336110044025,-9.87744070085091,-17.381888122219));
#42055=CARTESIAN_POINT('',(5.99999999995606,-9.91329603789449,-16.8993703023574));
#42056=CARTESIAN_POINT('',(5.59336167790258,-10.1144355809267,-17.2450590897518));
#42057=CARTESIAN_POINT('Origin',(5.6,-9.91330329119712,-16.8993688492374));
#42058=CARTESIAN_POINT('',(5.5933616956255,-9.87744142956214,-17.381887715675));
#42059=CARTESIAN_POINT('Origin',(5.59336169592161,-7.49315402656696,-13.0994163770562));
#42060=CARTESIAN_POINT('Origin',(5.6,-9.67863108611231,-17.0348569102122));
#42061=CARTESIAN_POINT('Ctrl Pts',(5.99999999999155,-9.91329301289976,-16.8993720623907));
#42062=CARTESIAN_POINT('Ctrl Pts',(5.9999999999916,-9.88722393977981,-16.9145397247211));
#42063=CARTESIAN_POINT('Ctrl Pts',(5.99999999999962,-9.86114407693648,-16.9296767195906));
#42064=CARTESIAN_POINT('Ctrl Pts',(5.99999999999962,-9.83508082013908,-16.9447638792498));
#42065=CARTESIAN_POINT('Ctrl Pts',(5.99999999999962,-9.80901756334168,-16.959851038909));
#42066=CARTESIAN_POINT('Ctrl Pts',(5.99999999999962,-9.78297091259021,-16.974888363358));
#42067=CARTESIAN_POINT('Ctrl Pts',(5.99999999999962,-9.75690044718562,-16.9899010654911));
#42068=CARTESIAN_POINT('Ctrl Pts',(5.99999999999962,-9.73082998178102,-17.0049137676242));
#42069=CARTESIAN_POINT('Ctrl Pts',(5.99999999999962,-9.7047357017233,-17.0199018474415));
#42070=CARTESIAN_POINT('Ctrl Pts',(5.99999999999962,-9.67863108609234,-17.0348569101268));
#42071=CARTESIAN_POINT('Origin',(5.6,-9.67863108603356,-17.0348569100686));
#42072=CARTESIAN_POINT('Origin',(5.600000004205,-9.67863108710757,-17.0348569087084));
#42073=CARTESIAN_POINT('Ctrl Pts',(-5.69266360645557,-9.93047718662622,
-17.3532040955763));
#42074=CARTESIAN_POINT('Ctrl Pts',(-5.65789955297649,-9.91591746177382,
-17.3608556206644));
#42075=CARTESIAN_POINT('Ctrl Pts',(-5.54372467191845,-9.86855446001491,
-17.3857806485202));
#42076=CARTESIAN_POINT('Ctrl Pts',(-5.34116840845335,-9.78714565169692,
-17.4287927186182));
#42077=CARTESIAN_POINT('Ctrl Pts',(-5.07576710977349,-9.68537184202562,
-17.4827626121575));
#42078=CARTESIAN_POINT('Ctrl Pts',(-4.78281267363776,-9.57897699504215,
-17.5393275023324));
#42079=CARTESIAN_POINT('Ctrl Pts',(-4.45929925449841,-9.46872737380591,
-17.5980532014339));
#42080=CARTESIAN_POINT('Ctrl Pts',(-4.10061014601583,-9.35538870497184,
-17.6585174226153));
#42081=CARTESIAN_POINT('Ctrl Pts',(-3.70134367778252,-9.24025425662571,
-17.7200257080785));
#42082=CARTESIAN_POINT('Ctrl Pts',(-3.2566726167652,-9.12574041664841,-17.7812901303106));
#42083=CARTESIAN_POINT('Ctrl Pts',(-2.76260093164982,-9.01549190881541,
-17.8403691196296));
#42084=CARTESIAN_POINT('Ctrl Pts',(-2.21454168295961,-8.91411127568825,
-17.8948066609545));
#42085=CARTESIAN_POINT('Ctrl Pts',(-1.60546929120789,-8.82723526419404,
-17.9415848779543));
#42086=CARTESIAN_POINT('Ctrl Pts',(-0.938933076209208,-8.76363029294198,
-17.9759675605449));
#42087=CARTESIAN_POINT('Ctrl Pts',(-0.236645353180689,-8.73273868672654,
-17.9927933052039));
#42088=CARTESIAN_POINT('Ctrl Pts',(0.464246679174975,-8.7390529531475,-17.989337089631));
#42089=CARTESIAN_POINT('Ctrl Pts',(1.1288813795409,-8.77907936488918,-17.9676027521604));
#42090=CARTESIAN_POINT('Ctrl Pts',(1.73416986111007,-8.84413326189491,-17.9324777156547));
#42091=CARTESIAN_POINT('Ctrl Pts',(2.2738216203696,-8.92486775034786,-17.8890293563113));
#42092=CARTESIAN_POINT('Ctrl Pts',(2.75209716612224,-9.01417698631136,-17.8410792541175));
#42093=CARTESIAN_POINT('Ctrl Pts',(3.17956622796434,-9.10813982684136,-17.7907195797015));
#42094=CARTESIAN_POINT('Ctrl Pts',(3.56235593967422,-9.20363013326605,-17.7396142074167));
#42095=CARTESIAN_POINT('Ctrl Pts',(3.90389825968162,-9.29788912705087,-17.6892297131137));
#42096=CARTESIAN_POINT('Ctrl Pts',(4.20699235675401,-9.388673083866,-17.6407574720575));
#42097=CARTESIAN_POINT('Ctrl Pts',(4.47553242575446,-9.47469414069719,-17.5948792514844));
#42098=CARTESIAN_POINT('Ctrl Pts',(4.71438132197511,-9.55560416869257,-17.5517772747069));
#42099=CARTESIAN_POINT('Ctrl Pts',(4.9283498408451,-9.63159810677658,-17.5113467756739));
#42100=CARTESIAN_POINT('Ctrl Pts',(5.12118003505284,-9.70292908305465,-17.4734546182196));
#42101=CARTESIAN_POINT('Ctrl Pts',(5.29544654742088,-9.76971701115713,-17.4380406162804));
#42102=CARTESIAN_POINT('Ctrl Pts',(5.45302073831863,-9.83201159502866,-17.4050827994527));
#42103=CARTESIAN_POINT('Ctrl Pts',(5.58355273454169,-9.88505636891086,-17.3770948527372));
#42104=CARTESIAN_POINT('Ctrl Pts',(5.66171486335273,-9.91751652281573,-17.3600153922565));
#42105=CARTESIAN_POINT('Ctrl Pts',(5.69263724707086,-9.93047273566079,-17.3532067220467));
#42106=CARTESIAN_POINT('Ctrl Pts',(-5.75649789768048,-9.81445032353156,
-17.4266145045828));
#42107=CARTESIAN_POINT('Ctrl Pts',(-5.72140176441163,-9.79971069472685,
-17.434270380524));
#42108=CARTESIAN_POINT('Ctrl Pts',(-5.60613635739674,-9.75175915352497,
-17.4592038938664));
#42109=CARTESIAN_POINT('Ctrl Pts',(-5.40164108893205,-9.66931698875883,
-17.5021963817961));
#42110=CARTESIAN_POINT('Ctrl Pts',(-5.13366937863353,-9.5661987286677,-17.5560725731441));
#42111=CARTESIAN_POINT('Ctrl Pts',(-4.83782308793672,-9.45834379568037,
-17.6124815425991));
#42112=CARTESIAN_POINT('Ctrl Pts',(-4.51104023762664,-9.34652661601802,
-17.6709975695962));
#42113=CARTESIAN_POINT('Ctrl Pts',(-4.14862925029359,-9.231521531333,-17.7312048309269));
#42114=CARTESIAN_POINT('Ctrl Pts',(-3.74510102845225,-9.11463774454148,
-17.7924129625212));
#42115=CARTESIAN_POINT('Ctrl Pts',(-3.29554242556852,-8.9983253434469,-17.8533379230091));
#42116=CARTESIAN_POINT('Ctrl Pts',(-2.79587913883895,-8.8862850261194,-17.9120433222388));
#42117=CARTESIAN_POINT('Ctrl Pts',(-2.24144276794023,-8.78319658437654,
-17.9660813301617));
#42118=CARTESIAN_POINT('Ctrl Pts',(-1.62510688401195,-8.69479920344606,
-18.0124491340476));
#42119=CARTESIAN_POINT('Ctrl Pts',(-0.950466599383164,-8.63003115288642,
-18.0464583229771));
#42120=CARTESIAN_POINT('Ctrl Pts',(-0.239549742883197,-8.59853868486254,
-18.0630341805028));
#42121=CARTESIAN_POINT('Ctrl Pts',(0.469949066202627,-8.60498016144591,
-18.0596381272223));
#42122=CARTESIAN_POINT('Ctrl Pts',(1.14273524876982,-8.64576713166439,-18.0381916489064));
#42123=CARTESIAN_POINT('Ctrl Pts',(1.75535098855907,-8.71199656223821,-18.0034263284059));
#42124=CARTESIAN_POINT('Ctrl Pts',(2.30141447271848,-8.79413512241296,-17.9603471611883));
#42125=CARTESIAN_POINT('Ctrl Pts',(2.7852478206494,-8.88494571507752,-17.9127462179189));
#42126=CARTESIAN_POINT('Ctrl Pts',(3.21756682194094,-8.98043993881617,-17.8627088342849));
#42127=CARTESIAN_POINT('Ctrl Pts',(3.60459389084317,-9.07744184548594,-17.8118953887759));
#42128=CARTESIAN_POINT('Ctrl Pts',(3.94982589630254,-9.17315216444604,-17.7617698453573));
#42129=CARTESIAN_POINT('Ctrl Pts',(4.25611894261082,-9.26529734916467,-17.7135218257619));
#42130=CARTESIAN_POINT('Ctrl Pts',(4.52743270504629,-9.35257560708462,-17.6678330416736));
#42131=CARTESIAN_POINT('Ctrl Pts',(4.76870079198005,-9.43463882557911,-17.6248868897531));
#42132=CARTESIAN_POINT('Ctrl Pts',(4.98479925044384,-9.51168909397294,-17.5845799209091));
#42133=CARTESIAN_POINT('Ctrl Pts',(5.17952065868517,-9.58398673758781,-17.546779662838));
#42134=CARTESIAN_POINT('Ctrl Pts',(5.35547601555703,-9.65165676751619,-17.5114262531364));
#42135=CARTESIAN_POINT('Ctrl Pts',(5.51456435186126,-9.71475354863065,-17.4784990017821));
#42136=CARTESIAN_POINT('Ctrl Pts',(5.64634486800574,-9.76846611527046,-17.4505151131804));
#42137=CARTESIAN_POINT('Ctrl Pts',(5.72525346100058,-9.80132967332423,-17.4334299861987));
#42138=CARTESIAN_POINT('Ctrl Pts',(5.75647083561349,-9.81444682222214,-17.4266191679546));
#42139=CARTESIAN_POINT('Ctrl Pts',(-5.81361929048237,-9.67439453857855,
-17.423197744291));
#42140=CARTESIAN_POINT('Ctrl Pts',(-5.77819666227631,-9.6595220433756,-17.4308427766472));
#42141=CARTESIAN_POINT('Ctrl Pts',(-5.66186327707103,-9.61114035601224,
-17.4557334262191));
#42142=CARTESIAN_POINT('Ctrl Pts',(-5.45549017818957,-9.52796766887907,
-17.4986076291796));
#42143=CARTESIAN_POINT('Ctrl Pts',(-5.18505475617177,-9.42393970967208,
-17.5522493851993));
#42144=CARTESIAN_POINT('Ctrl Pts',(-4.88646290757818,-9.31512956626903,
-17.6083407394487));
#42145=CARTESIAN_POINT('Ctrl Pts',(-4.55660702638627,-9.2023142636938,-17.6664668945342));
#42146=CARTESIAN_POINT('Ctrl Pts',(-4.1907357518231,-9.08627253772922,-17.7262204199607));
#42147=CARTESIAN_POINT('Ctrl Pts',(-3.78329193485985,-8.96832424820001,
-17.7869172956422));
#42148=CARTESIAN_POINT('Ctrl Pts',(-3.32929912805831,-8.85094208595135,
-17.8472814113126));
#42149=CARTESIAN_POINT('Ctrl Pts',(-2.82462928256113,-8.73786294953229,
-17.9053881650923));
#42150=CARTESIAN_POINT('Ctrl Pts',(-2.2645589068602,-8.63381421728722,-17.9588072543659));
#42151=CARTESIAN_POINT('Ctrl Pts',(-1.64189026832239,-8.54459435107722,
-18.0045638218666));
#42152=CARTESIAN_POINT('Ctrl Pts',(-0.96027229994903,-8.47922974920371,
-18.0380406721874));
#42153=CARTESIAN_POINT('Ctrl Pts',(-0.2420055177134,-8.44745609604986,-18.0542798623764));
#42154=CARTESIAN_POINT('Ctrl Pts',(0.474779168863501,-8.45395382657934,
-18.0509629399101));
#42155=CARTESIAN_POINT('Ctrl Pts',(1.15453262834516,-8.49510983520315,-18.0299118250766));
#42156=CARTESIAN_POINT('Ctrl Pts',(1.77347554169151,-8.56195149369413,-17.9956652267154));
#42157=CARTESIAN_POINT('Ctrl Pts',(2.32514101750424,-8.64485473380872,-17.9531396728781));
#42158=CARTESIAN_POINT('Ctrl Pts',(2.81388750093076,-8.73651098679611,-17.9060805154817));
#42159=CARTESIAN_POINT('Ctrl Pts',(3.25054379785076,-8.832890960607,-17.8565581084493));
#42160=CARTESIAN_POINT('Ctrl Pts',(3.64140302964256,-8.93078680616275,-17.8062235176184));
#42161=CARTESIAN_POINT('Ctrl Pts',(3.99000761178859,-9.02737231548921,-17.7565334831738));
#42162=CARTESIAN_POINT('Ctrl Pts',(4.29925370227988,-9.12035320253652,-17.7086725687123));
#42163=CARTESIAN_POINT('Ctrl Pts',(4.57315108197472,-9.20841675799382,-17.6633210002052));
#42164=CARTESIAN_POINT('Ctrl Pts',(4.81669094399185,-9.29121306576743,-17.6206634780497));
#42165=CARTESIAN_POINT('Ctrl Pts',(5.03480427213376,-9.36894754326617,-17.5805987012757));
#42166=CARTESIAN_POINT('Ctrl Pts',(5.23132679673705,-9.44188448240512,-17.5429955607112));
#42167=CARTESIAN_POINT('Ctrl Pts',(5.40890088264024,-9.51015186167537,-17.5077948859787));
#42168=CARTESIAN_POINT('Ctrl Pts',(5.56945003289077,-9.57380659447015,-17.4749776200002));
#42169=CARTESIAN_POINT('Ctrl Pts',(5.70244415125805,-9.62799710805693,-17.447059588863));
#42170=CARTESIAN_POINT('Ctrl Pts',(5.78208417666968,-9.6611555957235,-17.4300039376));
#42171=CARTESIAN_POINT('Ctrl Pts',(5.81359177729411,-9.67439082761106,-17.4232047915309));
#42172=CARTESIAN_POINT('Ctrl Pts',(-5.84786851508959,-9.55010334349577,
-17.3442496989582));
#42173=CARTESIAN_POINT('Ctrl Pts',(-5.812217479884,-9.5351824724971,-17.3518718310924));
#42174=CARTESIAN_POINT('Ctrl Pts',(-5.69514122735358,-9.4866502579589,-17.3766806339459));
#42175=CARTESIAN_POINT('Ctrl Pts',(-5.48748337876904,-9.4032556173417,-17.4193717913408));
#42176=CARTESIAN_POINT('Ctrl Pts',(-5.21538869253598,-9.29900866034276,
-17.4727054166742));
#42177=CARTESIAN_POINT('Ctrl Pts',(-4.9149750351536,-9.1900167307662,-17.5284081611456));
#42178=CARTESIAN_POINT('Ctrl Pts',(-4.5831125662408,-9.0770531753415,-17.5860755004643));
#42179=CARTESIAN_POINT('Ctrl Pts',(-4.21502210731758,-8.9608956758337,-17.6453079392981));
#42180=CARTESIAN_POINT('Ctrl Pts',(-3.80511703616835,-8.8428664734407,-17.7054282443237));
#42181=CARTESIAN_POINT('Ctrl Pts',(-3.34839805975775,-8.72544340689495,
-17.765170016477));
#42182=CARTESIAN_POINT('Ctrl Pts',(-2.8407230353756,-8.61236962673605,-17.8226236819756));
#42183=CARTESIAN_POINT('Ctrl Pts',(-2.27735525009385,-8.50837707579534,
-17.8753808010097));
#42184=CARTESIAN_POINT('Ctrl Pts',(-1.65107529422485,-8.41926371628257,
-17.9204993862399));
#42185=CARTESIAN_POINT('Ctrl Pts',(-0.965578662885549,-8.3540357348161,
-17.9534365922209));
#42186=CARTESIAN_POINT('Ctrl Pts',(-0.243318637273114,-8.3223788964438,
-17.9693481145899));
#42187=CARTESIAN_POINT('Ctrl Pts',(0.47737188163246,-8.32884628519568,-17.966106785336));
#42188=CARTESIAN_POINT('Ctrl Pts',(1.16093897363205,-8.3698768981194,-17.945446036046));
#42189=CARTESIAN_POINT('Ctrl Pts',(1.78342015349724,-8.43659637874813,-17.9117294849112));
#42190=CARTESIAN_POINT('Ctrl Pts',(2.33829376630727,-8.51941092724095,-17.869784288292));
#42191=CARTESIAN_POINT('Ctrl Pts',(2.82991911139756,-8.61102028452467,-17.8233051831625));
#42192=CARTESIAN_POINT('Ctrl Pts',(3.26917307993139,-8.70739211148768,-17.7743436753537));
#42193=CARTESIAN_POINT('Ctrl Pts',(3.66237499383399,-8.80531353084573,-17.724538365214));
#42194=CARTESIAN_POINT('Ctrl Pts',(4.01308062607134,-8.90195252815353,-17.6753362240971));
#42195=CARTESIAN_POINT('Ctrl Pts',(4.32419802749158,-8.99500899930038,-17.6279149003961));
#42196=CARTESIAN_POINT('Ctrl Pts',(4.59975757560383,-9.08316541187363,-17.5829521313571));
#42197=CARTESIAN_POINT('Ctrl Pts',(4.84477861688869,-9.16606874549135,-17.5406336814741));
#42198=CARTESIAN_POINT('Ctrl Pts',(5.06422123228634,-9.24392299646874,-17.5008606167677));
#42199=CARTESIAN_POINT('Ctrl Pts',(5.26194473312297,-9.31699208235458,-17.4635035011414));
#42200=CARTESIAN_POINT('Ctrl Pts',(5.44060899250946,-9.38540398708525,-17.4285040269477));
#42201=CARTESIAN_POINT('Ctrl Pts',(5.6021518658813,-9.44921534699241,-17.3958446583246));
#42202=CARTESIAN_POINT('Ctrl Pts',(5.73598088935879,-9.50355932364197,-17.3680353568609));
#42203=CARTESIAN_POINT('Ctrl Pts',(5.8161300955248,-9.53682114745297,-17.3510358204143));
#42204=CARTESIAN_POINT('Ctrl Pts',(5.84784092911347,-9.55009832792046,-17.344258799978));
#42205=CARTESIAN_POINT('',(-5.593361696257,-9.87744143006053,-17.3818877156668));
#42206=CARTESIAN_POINT('Ctrl Pts',(-5.593361696257,-9.87744143006053,-17.3818877156668));
#42207=CARTESIAN_POINT('Ctrl Pts',(-5.53987020059952,-9.85545802832816,
-17.3934585468391));
#42208=CARTESIAN_POINT('Ctrl Pts',(-5.4793497262585,-9.83099911672932,-17.4063497946954));
#42209=CARTESIAN_POINT('Ctrl Pts',(-5.37802554672181,-9.79072213244693,
-17.4276237192178));
#42210=CARTESIAN_POINT('Ctrl Pts',(-5.34249357553872,-9.77670562256007,
-17.4350336172399));
#42211=CARTESIAN_POINT('Ctrl Pts',(-5.28655975175779,-9.75487376400626,
-17.4465840985766));
#42212=CARTESIAN_POINT('Ctrl Pts',(-5.25793387311575,-9.74375670971193,
-17.4524678767338));
#42213=CARTESIAN_POINT('Ctrl Pts',(-5.22831954434635,-9.73235856535911,
-17.4585032833399));
#42214=CARTESIAN_POINT('Ctrl Pts',(-5.20835700291623,-9.72470001466014,
-17.4625591244086));
#42215=CARTESIAN_POINT('Ctrl Pts',(-5.19631311250797,-9.72009659507744,
-17.4649974123646));
#42216=CARTESIAN_POINT('Ctrl Pts',(-5.1220799029291,-9.69180540538195,-17.4799839844333));
#42217=CARTESIAN_POINT('Ctrl Pts',(-5.04939710272276,-9.66462085844997,
-17.4943969591114));
#42218=CARTESIAN_POINT('Ctrl Pts',(-4.93032631487558,-9.62113982432037,
-17.5174745985252));
#42219=CARTESIAN_POINT('Ctrl Pts',(-4.86827927406758,-9.59872847149976,
-17.5293749740773));
#42220=CARTESIAN_POINT('Ctrl Pts',(-4.79149567774383,-9.57153828977163,
-17.5438220492272));
#42221=CARTESIAN_POINT('Ctrl Pts',(-4.75200503407002,-9.55770243449621,
-17.5511756151097));
#42222=CARTESIAN_POINT('Ctrl Pts',(-4.73484500560012,-9.55172343097645,
-17.5543538058097));
#42223=CARTESIAN_POINT('Ctrl Pts',(-4.72335266064343,-9.54772672077564,
-17.556478385714));
#42224=CARTESIAN_POINT('Ctrl Pts',(-4.71643686245652,-9.54532685037244,
-17.5577541794684));
#42225=CARTESIAN_POINT('Ctrl Pts',(-4.56282068320413,-9.49210542227198,
-17.5860482166363));
#42226=CARTESIAN_POINT('Ctrl Pts',(-4.386889093463,-9.43374884345433,-17.6171019560031));
#42227=CARTESIAN_POINT('Ctrl Pts',(-4.08253603951581,-9.34005104916093,
-17.6670294778133));
#42228=CARTESIAN_POINT('Ctrl Pts',(-3.97434240997751,-9.30782386068614,
-17.6842115349644));
#42229=CARTESIAN_POINT('Ctrl Pts',(-3.80193804833617,-9.25876183240516,
-17.7103833193709));
#42230=CARTESIAN_POINT('Ctrl Pts',(-3.71320738818203,-9.23405323476083,
-17.7235674303112));
#42231=CARTESIAN_POINT('Ctrl Pts',(-3.6052634458353,-9.20511170082965,-17.7390166073284));
#42232=CARTESIAN_POINT('Ctrl Pts',(-3.55018526495355,-9.1906386182531,-17.7467441290376));
#42233=CARTESIAN_POINT('Ctrl Pts',(-3.52634328535243,-9.18443823905463,
-17.7500550341078));
#42234=CARTESIAN_POINT('Ctrl Pts',(-3.51039595563223,-9.18030550310546,
-17.7522619351916));
#42235=CARTESIAN_POINT('Ctrl Pts',(-3.50119799341605,-9.17793129863342,
-17.7535298272406));
#42236=CARTESIAN_POINT('Ctrl Pts',(-3.27586137147083,-9.11994720365643,
-17.7844960252267));
#42237=CARTESIAN_POINT('Ctrl Pts',(-3.02941181880873,-9.06174272207816,
-17.8156123473834));
#42238=CARTESIAN_POINT('Ctrl Pts',(-2.61782552001545,-8.97815820474398,
-17.860360920498));
#42239=CARTESIAN_POINT('Ctrl Pts',(-2.47364475878434,-8.95093882646814,
-17.8749443867086));
#42240=CARTESIAN_POINT('Ctrl Pts',(-2.24689562448764,-8.91208544364912,
-17.8957798174269));
#42241=CARTESIAN_POINT('Ctrl Pts',(-2.16956624764707,-8.89946471526788,
-17.9025510545595));
#42242=CARTESIAN_POINT('Ctrl Pts',(-2.01141482981592,-8.87506515653167,
-17.915648697891));
#42243=CARTESIAN_POINT('Ctrl Pts',(-1.93261264225071,-8.86356189842033,
-17.9218270113));
#42244=CARTESIAN_POINT('Ctrl Pts',(-1.50967150979595,-8.80586566263095,
-17.9528342587281));
#42245=CARTESIAN_POINT('Ctrl Pts',(-1.1550619741231,-8.76998362984971,-17.9721822696362));
#42246=CARTESIAN_POINT('Ctrl Pts',(-0.598762726050275,-8.73779219664723,
-17.9896029650133));
#42247=CARTESIAN_POINT('Ctrl Pts',(-0.409265485932076,-8.73066302435934,
-17.9934771411258));
#42248=CARTESIAN_POINT('Ctrl Pts',(-0.118923389613889,-8.72608300745925,
-17.9959714712881));
#42249=CARTESIAN_POINT('Ctrl Pts',(-0.0211266514843454,-8.72557448984061,
-17.9962498255603));
#42250=CARTESIAN_POINT('Ctrl Pts',(0.127092514745191,-8.72642220893752,
-17.9957877679624));
#42251=CARTESIAN_POINT('Ctrl Pts',(0.201583112618764,-8.72724880515296,
-17.9953371969745));
#42252=CARTESIAN_POINT('Ctrl Pts',(0.276645232630548,-8.72869526217384,
-17.9945496438171));
#42253=CARTESIAN_POINT('Ctrl Pts',(0.326813650891338,-8.72979901612804,
-17.9939488896616));
#42254=CARTESIAN_POINT('Ctrl Pts',(0.353716444626081,-8.73046880560203,
-17.9935844415831));
#42255=CARTESIAN_POINT('Ctrl Pts',(0.752470687018729,-8.74141659322514,
-17.9876293438515));
#42256=CARTESIAN_POINT('Ctrl Pts',(1.10888528675477,-8.76680638628075,-17.9738803725204));
#42257=CARTESIAN_POINT('Ctrl Pts',(1.61518192023207,-8.82097298245935,-17.9447112956001));
#42258=CARTESIAN_POINT('Ctrl Pts',(1.86124892043903,-8.85206972094614,-17.9279894068043));
#42259=CARTESIAN_POINT('Ctrl Pts',(2.13593478341671,-8.89391687546287,-17.9055257982567));
#42260=CARTESIAN_POINT('Ctrl Pts',(2.25100180242205,-8.91289053503451,-17.8953477722513));
#42261=CARTESIAN_POINT('Ctrl Pts',(2.32712303871463,-8.92575366186556,-17.8884490984369));
#42262=CARTESIAN_POINT('Ctrl Pts',(2.36664298290315,-8.93260298069073,-17.8847765119233));
#42263=CARTESIAN_POINT('Ctrl Pts',(2.68808813074154,-8.98954074940645,-17.8542525016971));
#42264=CARTESIAN_POINT('Ctrl Pts',(2.94934760460972,-9.04481782758675,-17.8246684230021));
#42265=CARTESIAN_POINT('Ctrl Pts',(3.30453249576307,-9.12819298700539,-17.7800978521836));
#42266=CARTESIAN_POINT('Ctrl Pts',(3.4168100728727,-9.15607565928406,-17.76520089681));
#42267=CARTESIAN_POINT('Ctrl Pts',(3.57605035862492,-9.19736314467759,-17.743153243358));
#42268=CARTESIAN_POINT('Ctrl Pts',(3.65337648152297,-9.21787438116161,-17.7322029881789));
#42269=CARTESIAN_POINT('Ctrl Pts',(3.7395757566091,-9.2414428236852,-17.7196251323142));
#42270=CARTESIAN_POINT('Ctrl Pts',(3.77565804558281,-9.25145346321499,-17.7142836508181));
#42271=CARTESIAN_POINT('Ctrl Pts',(3.79952173656711,-9.25810581892405,-17.7107342865122));
#42272=CARTESIAN_POINT('Ctrl Pts',(3.80961452997646,-9.26093063959662,-17.7092271754704));
#42273=CARTESIAN_POINT('Ctrl Pts',(4.03884499629718,-9.32544138467622,-17.6748113705168));
#42274=CARTESIAN_POINT('Ctrl Pts',(4.2328456349755,-9.38529250399132,-17.6429130577065));
#42275=CARTESIAN_POINT('Ctrl Pts',(4.49122806914593,-9.46901622821037,-17.5983382779601));
#42276=CARTESIAN_POINT('Ctrl Pts',(4.57191912656156,-9.4959353918958,-17.5840150142378));
#42277=CARTESIAN_POINT('Ctrl Pts',(4.68480108172324,-9.53443167111024,-17.5635439200051));
#42278=CARTESIAN_POINT('Ctrl Pts',(4.73920340156364,-9.55321133941474,-17.553560636219));
#42279=CARTESIAN_POINT('Ctrl Pts',(4.799105123665,-9.5742369214802,-17.5423882028615));
#42280=CARTESIAN_POINT('Ctrl Pts',(4.82401279362721,-9.58305308212916,-17.5377044547403));
#42281=CARTESIAN_POINT('Ctrl Pts',(4.8404480187903,-9.58888667848674,-17.5346054413657));
#42282=CARTESIAN_POINT('Ctrl Pts',(4.84692845456482,-9.59119177450282,-17.5333809517617));
#42283=CARTESIAN_POINT('Ctrl Pts',(4.93422806910404,-9.62235399167718,-17.5168284776004));
#42284=CARTESIAN_POINT('Ctrl Pts',(5.00665608387182,-9.64889059416907,-17.5027432111989));
#42285=CARTESIAN_POINT('Ctrl Pts',(5.10754064212285,-9.68649972701724,-17.4827987196256));
#42286=CARTESIAN_POINT('Ctrl Pts',(5.15604355527322,-9.70475862742077,-17.4731205210468));
#42287=CARTESIAN_POINT('Ctrl Pts',(5.20923639682545,-9.72504279169127,-17.4623766520456));
#42288=CARTESIAN_POINT('Ctrl Pts',(5.23130606667859,-9.73351349340259,-17.4578915977158));
#42289=CARTESIAN_POINT('Ctrl Pts',(5.24585756608274,-9.73911075894413,-17.4549283108024));
#42290=CARTESIAN_POINT('Ctrl Pts',(5.25198965447703,-9.74147381272326,-17.4536773941826));
#42291=CARTESIAN_POINT('Ctrl Pts',(5.39099848894759,-9.79518047740564,-17.4252507494902));
#42292=CARTESIAN_POINT('Ctrl Pts',(5.50206350613277,-9.83992060849029,-17.4016365743076));
#42293=CARTESIAN_POINT('Ctrl Pts',(5.593361696298,-9.877441429835,-17.3818877156174));
#42294=CARTESIAN_POINT('',(-5.73644346265596,-9.5212176560943,-17.3763289909634));
#42295=CARTESIAN_POINT('Origin',(-5.599999999997,-9.6786310860259,-17.0348569100619));
#42296=CARTESIAN_POINT('Ctrl Pts',(-5.73644387762363,-9.52121721553821,
-17.3763301032151));
#42297=CARTESIAN_POINT('Ctrl Pts',(-5.73644352459376,-9.52121707146375,
-17.3763301778592));
#42298=CARTESIAN_POINT('Ctrl Pts',(-5.73644317156365,-9.5212169273892,-17.3763302525035));
#42299=CARTESIAN_POINT('Ctrl Pts',(-5.73644281853329,-9.52121678331457,
-17.3763303271477));
#42300=CARTESIAN_POINT('Ctrl Pts',(-5.67992322178403,-9.49815066425739,
-17.3882807538312));
#42301=CARTESIAN_POINT('Ctrl Pts',(-5.61717095064414,-9.47290942008161,
-17.4013891368914));
#42302=CARTESIAN_POINT('Ctrl Pts',(-5.54808342727774,-9.44569918314702,
-17.4155436022901));
#42303=CARTESIAN_POINT('Ctrl Pts',(-5.52951990676316,-9.43838790946215,
-17.4193468462913));
#42304=CARTESIAN_POINT('Ctrl Pts',(-5.51049890446277,-9.43093469419091,
-17.4232254429296));
#42305=CARTESIAN_POINT('Ctrl Pts',(-5.49101823035263,-9.42334400648704,
-17.4271768288267));
#42306=CARTESIAN_POINT('Ctrl Pts',(-5.42195695327852,-9.39643412730443,
-17.4411849557898));
#42307=CARTESIAN_POINT('Ctrl Pts',(-5.34711974638812,-9.36779313739751,
-17.4561096755892));
#42308=CARTESIAN_POINT('Ctrl Pts',(-5.26639706158773,-9.33765672401009,
-17.4718271439572));
#42309=CARTESIAN_POINT('Ctrl Pts',(-5.2508485049638,-9.33185194024757,-17.4748545946361));
#42310=CARTESIAN_POINT('Ctrl Pts',(-5.2350815454412,-9.32599180437578,-17.4779113854455));
#42311=CARTESIAN_POINT('Ctrl Pts',(-5.21909533755791,-9.32007818972099,
-17.4809965265211));
#42312=CARTESIAN_POINT('Ctrl Pts',(-5.19132317678243,-9.30980471785349,
-17.4863562112312));
#42313=CARTESIAN_POINT('Ctrl Pts',(-5.16288931838467,-9.29936980768925,
-17.4918014763877));
#42314=CARTESIAN_POINT('Ctrl Pts',(-5.1337892851941,-9.2887838855698,-17.4973269203456));
#42315=CARTESIAN_POINT('Ctrl Pts',(-5.06602551715808,-9.26413298684911,
-17.5101937408131));
#42316=CARTESIAN_POINT('Ctrl Pts',(-4.99464963484642,-9.2386618869589,-17.5234960128167));
#42317=CARTESIAN_POINT('Ctrl Pts',(-4.91960196681596,-9.21251576379739,
-17.5371586424099));
#42318=CARTESIAN_POINT('Ctrl Pts',(-4.82891093158763,-9.18091959247115,
-17.5536691890301));
#42319=CARTESIAN_POINT('Ctrl Pts',(-4.73285787026604,-9.14833624523932,
-17.5707066532315));
#42320=CARTESIAN_POINT('Ctrl Pts',(-4.63133262667696,-9.11506274518776,
-17.588118684881));
#42321=CARTESIAN_POINT('Ctrl Pts',(-4.61738479820793,-9.11049153654174,
-17.5905107996119));
#42322=CARTESIAN_POINT('Ctrl Pts',(-4.6033336778579,-9.10590737359808,-17.5929099483661));
#42323=CARTESIAN_POINT('Ctrl Pts',(-4.58917897115216,-9.10131109609215,
-17.5953157015978));
#42324=CARTESIAN_POINT('Ctrl Pts',(-4.5569989063018,-9.09086167377023,-17.6007850692521));
#42325=CARTESIAN_POINT('Ctrl Pts',(-4.52428344765957,-9.08034960451572,
-17.6062885885683));
#42326=CARTESIAN_POINT('Ctrl Pts',(-4.49102921165013,-9.06978507926774,
-17.6118210417931));
#42327=CARTESIAN_POINT('Ctrl Pts',(-4.45061973879662,-9.05694740962175,
-17.6185439001483));
#42328=CARTESIAN_POINT('Ctrl Pts',(-4.40941469034533,-9.04403225153753,
-17.6253094982539));
#42329=CARTESIAN_POINT('Ctrl Pts',(-4.36740794739292,-9.03105885241992,
-17.6321080004935));
#42330=CARTESIAN_POINT('Ctrl Pts',(-4.34640457591672,-9.02457215286112,
-17.6355072516133));
#42331=CARTESIAN_POINT('Ctrl Pts',(-4.32520077691195,-9.01807089922343,
-17.6389147163269));
#42332=CARTESIAN_POINT('Ctrl Pts',(-4.30379578562449,-9.01155761129438,
-17.6423291198216));
#42333=CARTESIAN_POINT('Ctrl Pts',(-4.29309328998076,-9.00830096732986,
-17.644036321569));
#42334=CARTESIAN_POINT('Ctrl Pts',(-4.28234049601323,-9.00504131518672,
-17.6457452572156));
#42335=CARTESIAN_POINT('Ctrl Pts',(-4.2715373074274,-9.00177897451451,-17.6474557634699));
#42336=CARTESIAN_POINT('Ctrl Pts',(-4.26343491598802,-8.99933221901035,
-17.6487386431606));
#42337=CARTESIAN_POINT('Ctrl Pts',(-4.25530417755542,-8.9968839512415,-17.650022406252));
#42338=CARTESIAN_POINT('Ctrl Pts',(-4.24714505143305,-8.99443430757621,
-17.6513069830186));
#42339=CARTESIAN_POINT('Ctrl Pts',(-4.2444253427256,-8.99361775968778,-17.6517351752741));
#42340=CARTESIAN_POINT('Ctrl Pts',(-4.24040571702055,-8.99241248537787,
-17.6523672331073));
#42341=CARTESIAN_POINT('Ctrl Pts',(-4.23897646125202,-8.99198421043807,
-17.6525918284096));
#42342=CARTESIAN_POINT('Ctrl Pts',(-4.23363824301308,-8.99038461913656,
-17.6534306836833));
#42343=CARTESIAN_POINT('Ctrl Pts',(-4.22827574141105,-8.98878076076398,
-17.6542717650764));
#42344=CARTESIAN_POINT('Ctrl Pts',(-4.22288893012927,-8.98717271128015,
-17.6551150336142));
#42345=CARTESIAN_POINT('Ctrl Pts',(-4.1421074038801,-8.96305813128221,-17.6677608301641));
#42346=CARTESIAN_POINT('Ctrl Pts',(-4.05585939228501,-8.93799731004626,
-17.6809003637884));
#42347=CARTESIAN_POINT('Ctrl Pts',(-3.96405498682432,-8.91226963547649,
-17.6943903142864));
#42348=CARTESIAN_POINT('Ctrl Pts',(-3.91582486924293,-8.89875341298838,
-17.7014773586981));
#42349=CARTESIAN_POINT('Ctrl Pts',(-3.86606110337935,-8.88505388292564,
-17.7086607422642));
#42350=CARTESIAN_POINT('Ctrl Pts',(-3.81475024026647,-8.87121673240609,
-17.7159170732943));
#42351=CARTESIAN_POINT('Ctrl Pts',(-3.71991894440022,-8.84564329950596,
-17.7293280204715));
#42352=CARTESIAN_POINT('Ctrl Pts',(-3.61980302978308,-8.81959708984185,
-17.7429895018292));
#42353=CARTESIAN_POINT('Ctrl Pts',(-3.51432006484776,-8.79339955531239,
-17.7567370276897));
#42354=CARTESIAN_POINT('Ctrl Pts',(-3.46379569220283,-8.78085142493175,
-17.7633218361462));
#42355=CARTESIAN_POINT('Ctrl Pts',(-3.41204000915956,-8.76826924284194,
-17.7699260492204));
#42356=CARTESIAN_POINT('Ctrl Pts',(-3.35904414021376,-8.7556921475468,-17.7765296682036));
#42357=CARTESIAN_POINT('Ctrl Pts',(-3.24837094384221,-8.72942694301161,
-17.7903202453758));
#42358=CARTESIAN_POINT('Ctrl Pts',(-3.13228850732444,-8.70318068816256,
-17.8041098612256));
#42359=CARTESIAN_POINT('Ctrl Pts',(-3.01072520053139,-8.67734385271493,
-17.8176991668407));
#42360=CARTESIAN_POINT('Ctrl Pts',(-2.96856983178144,-8.66838423032262,
-17.8224116265818));
#42361=CARTESIAN_POINT('Ctrl Pts',(-2.92501766724462,-8.65932141386993,
-17.8271801970784));
#42362=CARTESIAN_POINT('Ctrl Pts',(-2.88136984601049,-8.65044680338113,
-17.8318519114778));
#42363=CARTESIAN_POINT('Ctrl Pts',(-2.87181233466587,-8.64850354050964,
-17.8328748712066));
#42364=CARTESIAN_POINT('Ctrl Pts',(-2.8622502854179,-8.64656913044084,-17.8338932746767));
#42365=CARTESIAN_POINT('Ctrl Pts',(-2.85269744002281,-8.64464634075612,
-17.8349056654296));
#42366=CARTESIAN_POINT('Ctrl Pts',(-2.83187074814701,-8.64045435955582,
-17.837112835063));
#42367=CARTESIAN_POINT('Ctrl Pts',(-2.81108776255884,-8.63631776879051,
-17.8392913449678));
#42368=CARTESIAN_POINT('Ctrl Pts',(-2.79049137152155,-8.63226346828058,
-17.84142701391));
#42369=CARTESIAN_POINT('Ctrl Pts',(-2.61969812019133,-8.59864363824783,
-17.8591368079095));
#42370=CARTESIAN_POINT('Ctrl Pts',(-2.45356650983542,-8.56904343577165,
-17.874747333849));
#42371=CARTESIAN_POINT('Ctrl Pts',(-2.29233862838001,-8.54299950336389,
-17.8884979961909));
#42372=CARTESIAN_POINT('Ctrl Pts',(-2.12998975602917,-8.51677449178518,
-17.9023442646225));
#42373=CARTESIAN_POINT('Ctrl Pts',(-1.97261304668375,-8.49415449375703,
-17.914305181698));
#42374=CARTESIAN_POINT('Ctrl Pts',(-1.82041653590442,-8.47465675411815,
-17.9246298556848));
#42375=CARTESIAN_POINT('Ctrl Pts',(-1.76985269925734,-8.46817907261915,
-17.9280599943012));
#42376=CARTESIAN_POINT('Ctrl Pts',(-1.71986020669752,-8.46204609989298,
-17.9313094777006));
#42377=CARTESIAN_POINT('Ctrl Pts',(-1.67044548275205,-8.45624043232021,
-17.9343872621625));
#42378=CARTESIAN_POINT('Ctrl Pts',(-1.52120350532392,-8.43870619880296,
-17.9436827636348));
#42379=CARTESIAN_POINT('Ctrl Pts',(-1.37723518824579,-8.4241556847917,-17.9514131060398));
#42380=CARTESIAN_POINT('Ctrl Pts',(-1.23869615121725,-8.4121078471322,-17.957825540084));
#42381=CARTESIAN_POINT('Ctrl Pts',(-1.14905169330374,-8.40431205253755,
-17.9619748339301));
#42382=CARTESIAN_POINT('Ctrl Pts',(-1.0616794722232,-8.39756458386839,-17.965572065017));
#42383=CARTESIAN_POINT('Ctrl Pts',(-0.976611993948442,-8.39174067995234,
-17.9686811741687));
#42384=CARTESIAN_POINT('Ctrl Pts',(-0.844717368027886,-8.38271088802736,
-17.9735017565679));
#42385=CARTESIAN_POINT('Ctrl Pts',(-0.718364973239535,-8.37589936903327,
-17.9771500149081));
#42386=CARTESIAN_POINT('Ctrl Pts',(-0.59764893798114,-8.37085523792009,
-17.9798579747241));
#42387=CARTESIAN_POINT('Ctrl Pts',(-0.480950252688124,-8.36597897216058,
-17.982475815425));
#42388=CARTESIAN_POINT('Ctrl Pts',(-0.369518419027349,-8.36275450372224,
-17.9842148255809));
#42389=CARTESIAN_POINT('Ctrl Pts',(-0.263409254252512,-8.36080591599256,
-17.9852673126018));
#42390=CARTESIAN_POINT('Ctrl Pts',(-0.255798643619334,-8.36066615480862,
-17.9853428015469));
#42391=CARTESIAN_POINT('Ctrl Pts',(-0.248215404147646,-8.36053297076181,
-17.9854147514066));
#42392=CARTESIAN_POINT('Ctrl Pts',(-0.24065955159746,-8.36040623146302,
-17.9854832297331));
#42393=CARTESIAN_POINT('Ctrl Pts',(-0.202148468472625,-8.35976025966322,
-17.9858322538181));
#42394=CARTESIAN_POINT('Ctrl Pts',(-0.164348870767216,-8.35928165386147,
-17.9860911216831));
#42395=CARTESIAN_POINT('Ctrl Pts',(-0.127262571736914,-8.3589527956832,
-17.9862686945712));
#42396=CARTESIAN_POINT('Ctrl Pts',(-0.10508126686014,-8.35875610570053,
-17.9863749008649));
#42397=CARTESIAN_POINT('Ctrl Pts',(-0.0831551306878216,-8.35861298799412,
-17.9864520145469));
#42398=CARTESIAN_POINT('Ctrl Pts',(-0.0614844712836392,-8.35851980347556,
-17.9865018816466));
#42399=CARTESIAN_POINT('Ctrl Pts',(-0.0416881557408339,-8.35843467869469,
-17.9865474356291));
#42400=CARTESIAN_POINT('Ctrl Pts',(-0.0231003214238363,-8.35839184303637,
-17.9865699936198));
#42401=CARTESIAN_POINT('Ctrl Pts',(-0.00299359736550399,-8.35838676981635,
-17.9865716737415));
#42402=CARTESIAN_POINT('Ctrl Pts',(-0.00108986357576685,-8.35838628947652,
-17.9865718328179));
#42403=CARTESIAN_POINT('Ctrl Pts',(0.000827486450446617,-8.35838618200386,
-17.9865717873868));
#42404=CARTESIAN_POINT('Ctrl Pts',(0.00276076763039516,-8.35838646560832,
-17.9865715281069));
#42405=CARTESIAN_POINT('Ctrl Pts',(0.115380446224821,-8.35840298645552,
-17.9865564242466));
#42406=CARTESIAN_POINT('Ctrl Pts',(0.233554097747699,-8.35974063747125,
-17.9858249645334));
#42407=CARTESIAN_POINT('Ctrl Pts',(0.357227596823177,-8.36282142206872,
-17.9841629399821));
#42408=CARTESIAN_POINT('Ctrl Pts',(0.400683622266197,-8.36390393897698,
-17.9835789427497));
#42409=CARTESIAN_POINT('Ctrl Pts',(0.444818436323151,-8.3652020196244,-17.9828798738739));
#42410=CARTESIAN_POINT('Ctrl Pts',(0.489628808808967,-8.36673509448657,
-17.9820558604452));
#42411=CARTESIAN_POINT('Ctrl Pts',(0.616894594461688,-8.37108917515977,
-17.9797155827246));
#42412=CARTESIAN_POINT('Ctrl Pts',(0.749612285280078,-8.37733668062018,
-17.9763686556394));
#42413=CARTESIAN_POINT('Ctrl Pts',(0.887682926937973,-8.38593002473395,
-17.9717825956685));
#42414=CARTESIAN_POINT('Ctrl Pts',(0.982201843108898,-8.39181276390401,
-17.968643120015));
#42415=CARTESIAN_POINT('Ctrl Pts',(1.0792286356825,-8.3987954762465,-17.9649225955862));
#42416=CARTESIAN_POINT('Ctrl Pts',(1.17872050964713,-8.40703101254687,-17.9605420742837));
#42417=CARTESIAN_POINT('Ctrl Pts',(1.32351032771627,-8.41901613007574,-17.9541671327216));
#42418=CARTESIAN_POINT('Ctrl Pts',(1.47352296203192,-8.43365408126441,-17.9463946600187));
#42419=CARTESIAN_POINT('Ctrl Pts',(1.62859653155586,-8.45142072464075,-17.9369799815677));
#42420=CARTESIAN_POINT('Ctrl Pts',(1.68654895885756,-8.45806028360508,-17.9334616291485));
#42421=CARTESIAN_POINT('Ctrl Pts',(1.74520772260452,-8.46513697481412,-17.9297138252413));
#42422=CARTESIAN_POINT('Ctrl Pts',(1.80456261858381,-8.47267625227983,-17.9257234471777));
#42423=CARTESIAN_POINT('Ctrl Pts',(1.96229923096924,-8.49271200615751,-17.9151189518365));
#42424=CARTESIAN_POINT('Ctrl Pts',(2.1249558097838,-8.51601437137955,-17.9028015591113));
#42425=CARTESIAN_POINT('Ctrl Pts',(2.29231728498669,-8.54305160629487,-17.8885294728786));
#42426=CARTESIAN_POINT('Ctrl Pts',(2.31269526918793,-8.54634366825407,-17.8867916993114));
#42427=CARTESIAN_POINT('Ctrl Pts',(2.33314294299478,-8.54969110847641,-17.885024941533));
#42428=CARTESIAN_POINT('Ctrl Pts',(2.35365986452972,-8.55309477709375,-17.8832287594278));
#42429=CARTESIAN_POINT('Ctrl Pts',(2.36243866304189,-8.55455114182873,-17.8824602074417));
#42430=CARTESIAN_POINT('Ctrl Pts',(2.37123013941515,-8.55601780098565,-17.8816862683799));
#42431=CARTESIAN_POINT('Ctrl Pts',(2.38003426028352,-8.5574948191759,-17.8809069088695));
#42432=CARTESIAN_POINT('Ctrl Pts',(2.44797134508464,-8.56889224448885,-17.8748929735834));
#42433=CARTESIAN_POINT('Ctrl Pts',(2.51666145215479,-8.58090650166341,-17.8685562781695));
#42434=CARTESIAN_POINT('Ctrl Pts',(2.58608847376924,-8.59356722554678,-17.8618815018982));
#42435=CARTESIAN_POINT('Ctrl Pts',(2.62080198457646,-8.59989758748846,-17.8585441137625));
#42436=CARTESIAN_POINT('Ctrl Pts',(2.6556997235816,-8.60638956729783,-17.8551222031688));
#42437=CARTESIAN_POINT('Ctrl Pts',(2.69077952127531,-8.61304685414928,-17.851613861692));
#42438=CARTESIAN_POINT('Ctrl Pts',(2.70831942012216,-8.61637549757501,-17.8498596909536));
#42439=CARTESIAN_POINT('Ctrl Pts',(2.72590483362213,-8.61974546781656,-17.8480839123907));
#42440=CARTESIAN_POINT('Ctrl Pts',(2.74353548531567,-8.62315722542768,-17.8462862873725));
#42441=CARTESIAN_POINT('Ctrl Pts',(2.75886023088542,-8.62612276057889,-17.844723773036));
#42442=CARTESIAN_POINT('Ctrl Pts',(2.77563789148753,-8.62939846974932,-17.8429979696744));
#42443=CARTESIAN_POINT('Ctrl Pts',(2.79016868445501,-8.63225838463787,-17.8414913638725));
#42444=CARTESIAN_POINT('Ctrl Pts',(2.79235512496293,-8.63268871447435,-17.8412646657176));
#42445=CARTESIAN_POINT('Ctrl Pts',(2.79449071610734,-8.63310954567438,-17.8410429737587));
#42446=CARTESIAN_POINT('Ctrl Pts',(2.79656287567783,-8.63351832069494,-17.8408276342317));
#42447=CARTESIAN_POINT('Ctrl Pts',(2.81155194711914,-8.63647521555661,-17.8392699648313));
#42448=CARTESIAN_POINT('Ctrl Pts',(2.82653495592412,-8.6394549709341,-17.8377005599592));
#42449=CARTESIAN_POINT('Ctrl Pts',(2.84151182039781,-8.64245751452065,-17.8361194547485));
#42450=CARTESIAN_POINT('Ctrl Pts',(2.98776197925397,-8.67177756861319,-17.8206798486395));
#42451=CARTESIAN_POINT('Ctrl Pts',(3.13342623719005,-8.70327062452146,-17.8041245447627));
#42452=CARTESIAN_POINT('Ctrl Pts',(3.27843755206495,-8.73686228895337,-17.7864898983305));
#42453=CARTESIAN_POINT('Ctrl Pts',(3.40982752547695,-8.76729858904749,-17.7705117263661));
#42454=CARTESIAN_POINT('Ctrl Pts',(3.54068146009692,-8.7994577580664,-17.7536474595275));
#42455=CARTESIAN_POINT('Ctrl Pts',(3.67095575806953,-8.83328068790664,-17.7359259293636));
#42456=CARTESIAN_POINT('Ctrl Pts',(3.7881302786502,-8.86370254126023,-17.7199863938356));
#42457=CARTESIAN_POINT('Ctrl Pts',(3.90483587259101,-8.89547037835598,-17.7033533317629));
#42458=CARTESIAN_POINT('Ctrl Pts',(4.02104510452003,-8.92853923906793,-17.6860484800191));
#42459=CARTESIAN_POINT('Ctrl Pts',(4.12468783508762,-8.95803213704215,-17.6706149205934));
#42460=CARTESIAN_POINT('Ctrl Pts',(4.22793574925146,-8.9885598949597,-17.6546470065895));
#42461=CARTESIAN_POINT('Ctrl Pts',(4.33077217729926,-9.0200896656201,-17.6381603930781));
#42462=CARTESIAN_POINT('Ctrl Pts',(4.42240217237626,-9.04818353065642,-17.6234703815367));
#42463=CARTESIAN_POINT('Ctrl Pts',(4.51370547671078,-9.07707292191899,-17.6083685600615));
#42464=CARTESIAN_POINT('Ctrl Pts',(4.60467210495441,-9.1067341689929,-17.5928660142161));
#42465=CARTESIAN_POINT('Ctrl Pts',(4.68609298329243,-9.13328285872658,-17.5789902564401));
#42466=CARTESIAN_POINT('Ctrl Pts',(4.76724413733699,-9.16044991128749,-17.5647934634993));
#42467=CARTESIAN_POINT('Ctrl Pts',(4.84811962989529,-9.18821823686332,-17.550283531101));
#42468=CARTESIAN_POINT('Ctrl Pts',(4.92104264857972,-9.213256107555,-17.5372003579677));
#42469=CARTESIAN_POINT('Ctrl Pts',(4.99374155163286,-9.23878281838882,-17.5238625999774));
#42470=CARTESIAN_POINT('Ctrl Pts',(5.06621286141821,-9.26478600954632,-17.510276029362));
#42471=CARTESIAN_POINT('Ctrl Pts',(5.13211260416723,-9.28843127845354,-17.497921464348));
#42472=CARTESIAN_POINT('Ctrl Pts',(5.19782415727064,-9.31247053252497,-17.4853611648872));
#42473=CARTESIAN_POINT('Ctrl Pts',(5.26334554178665,-9.33689503275619,-17.4725995993014));
#42474=CARTESIAN_POINT('Ctrl Pts',(5.32292696859615,-9.35910528645634,-17.4609949561526));
#42475=CARTESIAN_POINT('Ctrl Pts',(5.38235114343648,-9.38163410200066,-17.4492238850272));
#42476=CARTESIAN_POINT('Ctrl Pts',(5.44161694958957,-9.40447611389181,-17.4372902012635));
#42477=CARTESIAN_POINT('Ctrl Pts',(5.49538378457564,-9.42519873227531,-17.4264637830074));
#42478=CARTESIAN_POINT('Ctrl Pts',(5.54902027517795,-9.44617912364355,-17.4155035276484));
#42479=CARTESIAN_POINT('Ctrl Pts',(5.60252556054591,-9.46741559848347,-17.4044133515384));
#42480=CARTESIAN_POINT('Ctrl Pts',(5.64725681504284,-9.48516962323354,-17.3951417910453));
#42481=CARTESIAN_POINT('Ctrl Pts',(5.69189636725116,-9.50310263122264,-17.3857794246311));
#42482=CARTESIAN_POINT('Ctrl Pts',(5.736442763711,-9.52121697643775,-17.3763304371651));
#42483=CARTESIAN_POINT('Ctrl Pts',(-5.843530256076,-9.74782193877526,-17.4349067568258));
#42484=CARTESIAN_POINT('Ctrl Pts',(-3.895686837384,-8.92798470939806,-17.8601636858557));
#42485=CARTESIAN_POINT('Ctrl Pts',(0.0001633689307963,-8.10806560616921,
-18.2855103771765));
#42486=CARTESIAN_POINT('Ctrl Pts',(3.896013575246,-8.92805347740346,-17.8601280113164));
#42487=CARTESIAN_POINT('Ctrl Pts',(5.844020362869,-9.74802823084197,-17.4347997512851));
#42488=CARTESIAN_POINT('Ctrl Pts',(-5.843530256076,-8.93341761899431,-17.0810054062716));
#42489=CARTESIAN_POINT('Ctrl Pts',(-3.895686837384,-8.18554673507222,-17.4915920272974));
#42490=CARTESIAN_POINT('Ctrl Pts',(0.0001633689307963,-7.43613495951606,
-17.9044826847225));
#42491=CARTESIAN_POINT('Ctrl Pts',(3.896013575246,-8.1856095895101,-17.4915573974575));
#42492=CARTESIAN_POINT('Ctrl Pts',(5.844020362869,-8.93360580246804,-17.0809020921739));
#42493=CARTESIAN_POINT('Ctrl Pts',(-5.843530256076,-7.38850509491984,-16.1560629985976));
#42494=CARTESIAN_POINT('Ctrl Pts',(-3.895686837384,-6.77499150312524,-16.5818456797104));
#42495=CARTESIAN_POINT('Ctrl Pts',(0.0001633689307963,-6.16225640987013,
-17.0065480644992));
#42496=CARTESIAN_POINT('Ctrl Pts',(3.896013575246,-6.77504289425523,-16.5818100592022));
#42497=CARTESIAN_POINT('Ctrl Pts',(5.844020362869,-7.38865947067571,-16.1559558607449));
#42498=CARTESIAN_POINT('Ctrl Pts',(-5.843530256076,-5.5035950496103,-14.2139340091191));
#42499=CARTESIAN_POINT('Ctrl Pts',(-3.895686837384,-5.02273055192306,-14.7660279927807));
#42500=CARTESIAN_POINT('Ctrl Pts',(0.0001633689307963,-4.54131578037147,
-15.3185227509534));
#42501=CARTESIAN_POINT('Ctrl Pts',(3.896013575246,-5.02277092898996,-14.7659816541094));
#42502=CARTESIAN_POINT('Ctrl Pts',(5.844020362869,-5.50371604744393,-14.2137950881237));
#42503=CARTESIAN_POINT('Ctrl Pts',(-5.843530256076,-4.23580607983558,-11.9384133491196));
#42504=CARTESIAN_POINT('Ctrl Pts',(-3.895686837384,-3.77920631945423,-12.6803362705394));
#42505=CARTESIAN_POINT('Ctrl Pts',(0.000163368930796,-3.32382368434964,
-13.4219152215187));
#42506=CARTESIAN_POINT('Ctrl Pts',(3.896013575246,-3.77924451316813,-12.6802740730544));
#42507=CARTESIAN_POINT('Ctrl Pts',(5.844020362869,-4.23592097205499,-11.9382266622861));
#42508=CARTESIAN_POINT('Ctrl Pts',(-5.843530256076,-3.79656718977774,-10.3003446896952));
#42509=CARTESIAN_POINT('Ctrl Pts',(-3.895686837384,-3.28180463172425,-11.1801039028799));
#42510=CARTESIAN_POINT('Ctrl Pts',(0.0001633689307967,-2.7647865035497,
-12.0604688985302));
#42511=CARTESIAN_POINT('Ctrl Pts',(3.896013575246,-3.28184799491133,-11.1800300651747));
#42512=CARTESIAN_POINT('Ctrl Pts',(5.844020362869,-3.79669671721236,-10.3001233197275));
#42513=CARTESIAN_POINT('Ctrl Pts',(-5.843530256076,-3.68097872426921,-9.52158370504134));
#42514=CARTESIAN_POINT('Ctrl Pts',(-3.895686837384,-3.1209711468501,-10.4634383653078));
#42515=CARTESIAN_POINT('Ctrl Pts',(0.0001633689307967,-2.56014623248247,
-11.4055359487921));
#42516=CARTESIAN_POINT('Ctrl Pts',(3.896013575246,-3.12101818418698,-10.4633593499865));
#42517=CARTESIAN_POINT('Ctrl Pts',(5.844020362869,-3.6811196365252,-9.52134671026255));
#42518=CARTESIAN_POINT('',(-5.732788638925,-3.68906708236562,-9.81543797412044));
#42519=CARTESIAN_POINT('Ctrl Pts',(-5.73644356954166,-9.5212182362576,-17.3763277345531));
#42520=CARTESIAN_POINT('Ctrl Pts',(-5.73766037024463,-8.76684683173291,
-17.028090734259));
#42521=CARTESIAN_POINT('Ctrl Pts',(-5.73849618482518,-8.05516360140243,
-16.5887330605515));
#42522=CARTESIAN_POINT('Ctrl Pts',(-5.73940756700657,-6.75884968378645,
-15.5535369808515));
#42523=CARTESIAN_POINT('Ctrl Pts',(-5.73948313454001,-6.17416092819343,
-14.9577815504229));
#42524=CARTESIAN_POINT('Ctrl Pts',(-5.73887402245194,-5.16463991732877,
-13.6459927354831));
#42525=CARTESIAN_POINT('Ctrl Pts',(-5.73818934283044,-4.74008689118233,
-12.9297576020434));
#42526=CARTESIAN_POINT('Ctrl Pts',(-5.73605973643251,-4.07387566043888,
-11.4195453042489));
#42527=CARTESIAN_POINT('Ctrl Pts',(-5.73461480965608,-3.83284551954944,
-10.6253394036378));
#42528=CARTESIAN_POINT('Ctrl Pts',(-5.732788638925,-3.68906708236562,-9.81543797412044));
#42529=CARTESIAN_POINT('Ctrl Pts',(5.73278688036066,-3.68906294648598,-9.81543868668658));
#42530=CARTESIAN_POINT('Ctrl Pts',(5.37903378703979,-3.59284163073062,-9.98632746914467));
#42531=CARTESIAN_POINT('Ctrl Pts',(5.01625588585428,-3.50245734812832,-10.1410436198638));
#42532=CARTESIAN_POINT('Ctrl Pts',(4.64606584067004,-3.4196218239831,-10.2790646475806));
#42533=CARTESIAN_POINT('Ctrl Pts',(4.3717064383795,-3.35822983036102,-10.3813563411593));
#42534=CARTESIAN_POINT('Ctrl Pts',(4.0932757270239,-3.30098748245638,-10.4744756568886));
#42535=CARTESIAN_POINT('Ctrl Pts',(3.8114301982303,-3.24859133006159,-10.5582373815854));
#42536=CARTESIAN_POINT('Ctrl Pts',(3.57233893573706,-3.204143357871,-10.6292929579932));
#42537=CARTESIAN_POINT('Ctrl Pts',(3.33079029164474,-3.16318341588268,-10.6936140694128));
#42538=CARTESIAN_POINT('Ctrl Pts',(3.08718502825172,-3.12611849781819,-10.7511239095404));
#42539=CARTESIAN_POINT('Ctrl Pts',(3.04362356893838,-3.1194905543258,-10.7614078111522));
#42540=CARTESIAN_POINT('Ctrl Pts',(2.99999634605026,-3.11298709530054,-10.7714740291743));
#42541=CARTESIAN_POINT('Ctrl Pts',(2.95630565116257,-3.10661035551622,-10.7813222892007));
#42542=CARTESIAN_POINT('Ctrl Pts',(2.75783727944364,-3.07764352024104,-10.8260587745489));
#42543=CARTESIAN_POINT('Ctrl Pts',(2.55805789464781,-3.05130996919154,-10.8663594316571));
#42544=CARTESIAN_POINT('Ctrl Pts',(2.35723405313087,-3.02778623237469,-10.9020986226108));
#42545=CARTESIAN_POINT('Ctrl Pts',(2.16323819137806,-3.00506229899627,-10.9366226865617));
#42546=CARTESIAN_POINT('Ctrl Pts',(1.96826768825925,-2.98496040015708,-10.9668901438503));
#42547=CARTESIAN_POINT('Ctrl Pts',(1.77256282543726,-2.96761517395057,-10.9928292031195));
#42548=CARTESIAN_POINT('Ctrl Pts',(1.57994261266313,-2.95054333876805,-11.0183594175635));
#42549=CARTESIAN_POINT('Ctrl Pts',(1.38661100732697,-2.93614205053063,-11.0396964692977));
#42550=CARTESIAN_POINT('Ctrl Pts',(1.1927971074576,-2.92451449290185,-11.0568142909632));
#42551=CARTESIAN_POINT('Ctrl Pts',(0.994683243107288,-2.91262896572167,
-11.0743118894415));
#42552=CARTESIAN_POINT('Ctrl Pts',(0.796065446409081,-2.90364186949685,
-11.0874005424206));
#42553=CARTESIAN_POINT('Ctrl Pts',(0.597188404533596,-2.89763401017108,
-11.0961016630333));
#42554=CARTESIAN_POINT('Ctrl Pts',(0.408362354537037,-2.89192978038809,
-11.1043630401151));
#42555=CARTESIAN_POINT('Ctrl Pts',(0.219302601049658,-2.88891114283554,
-11.1086693634381));
#42556=CARTESIAN_POINT('Ctrl Pts',(0.0302185760373398,-2.8886206466935,
-11.1090834497124));
#42557=CARTESIAN_POINT('Ctrl Pts',(0.0201538524472,-2.88860518392041,-11.109105491045));
#42558=CARTESIAN_POINT('Ctrl Pts',(0.0100890600883165,-2.88859744448944,
-11.1091165150391));
#42559=CARTESIAN_POINT('Ctrl Pts',(2.42305459169099E-5,-2.88859743267018,
-11.1091165347574));
#42560=CARTESIAN_POINT('Ctrl Pts',(1.61536968630372E-5,-2.88859743266069,
-11.1091165347732));
#42561=CARTESIAN_POINT('Ctrl Pts',(8.07684783334205E-6,-2.88859743265618,
-11.1091165347819));
#42562=CARTESIAN_POINT('Ctrl Pts',(-1.17328610291081E-12,-2.88859743265665,
-11.1091165347836));
#42563=CARTESIAN_POINT('Ctrl Pts',(-0.189437344854955,-2.88859744363441,
-11.1091165734976));
#42564=CARTESIAN_POINT('Ctrl Pts',(-0.378861690437173,-2.89133726996081,
-11.1052144979462));
#42565=CARTESIAN_POINT('Ctrl Pts',(-0.568062428807369,-2.89677554744192,
-11.097344766198));
#42566=CARTESIAN_POINT('Ctrl Pts',(-0.769447710209329,-2.90256405043779,
-11.0889682230813));
#42567=CARTESIAN_POINT('Ctrl Pts',(-0.970579656371806,-2.91140995242851,
-11.0760962038057));
#42568=CARTESIAN_POINT('Ctrl Pts',(-1.17120429318957,-2.92323076595731,
-11.0587041736618));
#42569=CARTESIAN_POINT('Ctrl Pts',(-1.36703736658995,-2.93476926033246,
-11.0417275212937));
#42570=CARTESIAN_POINT('Ctrl Pts',(-1.56238707363891,-2.94914199135374,
-11.0204446274376));
#42571=CARTESIAN_POINT('Ctrl Pts',(-1.75701720624661,-2.96624345460967,
-10.994880896949));
#42572=CARTESIAN_POINT('Ctrl Pts',(-1.95879053438656,-2.98397256526165,
-10.9683789421321));
#42573=CARTESIAN_POINT('Ctrl Pts',(-2.15979050006648,-3.00463437240796,
-10.9372761550918));
#42574=CARTESIAN_POINT('Ctrl Pts',(-2.35975392151571,-3.02808173670664,
-10.9016506212175));
#42575=CARTESIAN_POINT('Ctrl Pts',(-2.55971734296493,-3.05152910100532,
-10.8660250873432));
#42576=CARTESIAN_POINT('Ctrl Pts',(-2.75864422018347,-3.07776182110568,
-10.825877125748));
#42577=CARTESIAN_POINT('Ctrl Pts',(-2.95627137140066,-3.10660556548852,
-10.7813308547632));
#42578=CARTESIAN_POINT('Ctrl Pts',(-3.19883119754988,-3.14200724779738,
-10.7266565062279));
#42579=CARTESIAN_POINT('Ctrl Pts',(-3.43943497053319,-3.18131687623534,
-10.665260368241));
#42580=CARTESIAN_POINT('Ctrl Pts',(-3.67769055117286,-3.22414075633116,
-10.5972094009893));
#42581=CARTESIAN_POINT('Ctrl Pts',(-3.96259738974965,-3.27534969868177,
-10.5158338214973));
#42582=CARTESIAN_POINT('Ctrl Pts',(-4.24414644049201,-3.33158317306783,
-10.4249426846565));
#42583=CARTESIAN_POINT('Ctrl Pts',(-4.52166717124462,-3.3921331042644,-10.3247174210247));
#42584=CARTESIAN_POINT('Ctrl Pts',(-4.88864236905086,-3.47220035876374,
-10.1921861112134));
#42585=CARTESIAN_POINT('Ctrl Pts',(-5.24857377478926,-3.5598100414616,-10.0433370079679));
#42586=CARTESIAN_POINT('Ctrl Pts',(-5.59991098953761,-3.65331093395734,
-9.87866971603991));
#42587=CARTESIAN_POINT('Ctrl Pts',(-5.64434240534598,-3.66513540588499,
-9.85784527555776));
#42588=CARTESIAN_POINT('Ctrl Pts',(-5.68863637360616,-3.67705416337425,
-9.8367678762802));
#42589=CARTESIAN_POINT('Ctrl Pts',(-5.73278975856799,-3.68906394712505,
-9.81543852851373));
#42590=CARTESIAN_POINT('Ctrl Pts',(5.84421883180474,-3.72282215870307,-9.78170207264411));
#42591=CARTESIAN_POINT('Ctrl Pts',(5.60210555070136,-3.65638716931675,-9.90489110085523));
#42592=CARTESIAN_POINT('Ctrl Pts',(4.82411485412597,-3.45517207621565,-10.2687173462891));
#42593=CARTESIAN_POINT('Ctrl Pts',(3.45674861901373,-3.1717867894043,-10.7434846212514));
#42594=CARTESIAN_POINT('Ctrl Pts',(1.73637252749493,-2.95116599793079,-11.0872359518019));
#42595=CARTESIAN_POINT('Ctrl Pts',(0.00178708571280825,-2.87580440265437,
-11.2002490127008));
#42596=CARTESIAN_POINT('Ctrl Pts',(-1.73280014723785,-2.95085735941276,
-11.0877033118007));
#42597=CARTESIAN_POINT('Ctrl Pts',(-3.45327880384202,-3.1711983285024,-10.7444278554086));
#42598=CARTESIAN_POINT('Ctrl Pts',(-4.82196103408831,-3.45464798710974,
-10.269637251114));
#42599=CARTESIAN_POINT('Ctrl Pts',(-5.60114390651019,-3.6561220066129,-9.90538363300166));
#42600=CARTESIAN_POINT('Ctrl Pts',(-5.8443346108831,-3.72285393964802,-9.78164313446629));
#42601=CARTESIAN_POINT('Ctrl Pts',(5.7253702758327,-3.64455037473193,-9.50230796587388));
#42602=CARTESIAN_POINT('Ctrl Pts',(5.4881314994798,-3.58036715962835,-9.62279259868668));
#42603=CARTESIAN_POINT('Ctrl Pts',(4.72581564301797,-3.38588375667695,-9.97867779049632));
#42604=CARTESIAN_POINT('Ctrl Pts',(3.38610693741535,-3.11167079843839,-10.4432062423216));
#42605=CARTESIAN_POINT('Ctrl Pts',(1.70079220243387,-2.89802964660707,-10.7795799094507));
#42606=CARTESIAN_POINT('Ctrl Pts',(0.00175042691972879,-2.82503096864176,
-10.8901685400845));
#42607=CARTESIAN_POINT('Ctrl Pts',(-1.69729287672102,-2.89773070464145,
-10.7800372441397));
#42608=CARTESIAN_POINT('Ctrl Pts',(-3.3827075656956,-3.11110109891825,-10.4441292117391));
#42609=CARTESIAN_POINT('Ctrl Pts',(-4.72370524846715,-3.38537694518877,
-9.97957774413633));
#42610=CARTESIAN_POINT('Ctrl Pts',(-5.48718921578431,-3.58011099558317,
-9.62327431064613));
#42611=CARTESIAN_POINT('Ctrl Pts',(-5.72548372426805,-3.64458107905496,
-9.50225032158714));
#42612=CARTESIAN_POINT('Ctrl Pts',(5.71942246157996,-3.37473909219602,-9.34268285703912));
#42613=CARTESIAN_POINT('Ctrl Pts',(5.48287285233699,-3.3112654349926,-9.46194227133996));
#42614=CARTESIAN_POINT('Ctrl Pts',(4.72266850715085,-3.11884881435695,-9.81433425125829));
#42615=CARTESIAN_POINT('Ctrl Pts',(3.38569730696337,-2.84709739195396,-10.2749197644463));
#42616=CARTESIAN_POINT('Ctrl Pts',(1.70145185496075,-2.63491822139972,-10.6090358172226));
#42617=CARTESIAN_POINT('Ctrl Pts',(0.00175145994779487,-2.56231815139111,
-10.7190101985091));
#42618=CARTESIAN_POINT('Ctrl Pts',(-1.69795250354239,-2.63462102463518,
-10.6094904682724));
#42619=CARTESIAN_POINT('Ctrl Pts',(-3.38230253911364,-2.84653212429915,
-10.2758358266937));
#42620=CARTESIAN_POINT('Ctrl Pts',(-4.72056368204768,-3.11834712228491,
-9.81522575608262));
#42621=CARTESIAN_POINT('Ctrl Pts',(-5.48193330987248,-3.311012103631,-9.4624190734827));
#42622=CARTESIAN_POINT('Ctrl Pts',(-5.71953557724954,-3.37476945656438,
-9.34262580081448));
#42623=CARTESIAN_POINT('Ctrl Pts',(5.83023580926565,-3.08842202064092,-9.40638358569627));
#42624=CARTESIAN_POINT('Ctrl Pts',(5.58974287210655,-3.02365536252599,-9.52669182842707));
#42625=CARTESIAN_POINT('Ctrl Pts',(4.81671666980029,-2.8272997397519,-9.88230469038235));
#42626=CARTESIAN_POINT('Ctrl Pts',(3.45578661938464,-2.54970205873507,-10.3478011867109));
#42627=CARTESIAN_POINT('Ctrl Pts',(1.73792413620994,-2.33251867796578,-10.6862443582688));
#42628=CARTESIAN_POINT('Ctrl Pts',(0.00178951524897414,-2.25809428228155,
-10.7978131876545));
#42629=CARTESIAN_POINT('Ctrl Pts',(-1.73435169431629,-2.33221414274175,
-10.6867054084471));
#42630=CARTESIAN_POINT('Ctrl Pts',(-3.45232762804018,-2.54912401807523,
-10.3487281805197));
#42631=CARTESIAN_POINT('Ctrl Pts',(-4.81457594437186,-2.82678768753553,
-9.8832047300166));
#42632=CARTESIAN_POINT('Ctrl Pts',(-5.58878767299468,-3.02339686010146,
-9.52717281640476));
#42633=CARTESIAN_POINT('Ctrl Pts',(-5.83035080595657,-3.08845300227363,
-9.4063260301971));
#42634=CARTESIAN_POINT('',(-5.7200185442403,-3.0799676360579,-9.45352569283355));
#42635=CARTESIAN_POINT('Origin',(-5.89878573791871,-3.22460261179308,-9.89753636536867));
#42636=CARTESIAN_POINT('Ctrl Pts',(5.72001578658213,-3.07996614583804,-9.45352684908776));
#42637=CARTESIAN_POINT('Ctrl Pts',(5.51356681596581,-3.02529977540968,-9.55445522100768));
#42638=CARTESIAN_POINT('Ctrl Pts',(5.30316956267147,-2.97232139279663,-9.65016641036658));
#42639=CARTESIAN_POINT('Ctrl Pts',(5.08894867055704,-2.92143297802579,-9.74045681632173));
#42640=CARTESIAN_POINT('Ctrl Pts',(4.85594668814816,-2.8660830940522,-9.8386631274448));
#42641=CARTESIAN_POINT('Ctrl Pts',(4.61842051735488,-2.81320484592507,-9.93045706148136));
#42642=CARTESIAN_POINT('Ctrl Pts',(4.3766008775274,-2.76339299495987,-10.0155394511694));
#42643=CARTESIAN_POINT('Ctrl Pts',(4.14452715583251,-2.71558868243068,-10.0971928141457));
#42644=CARTESIAN_POINT('Ctrl Pts',(3.90849626788228,-2.67057763096145,-10.1726744199736));
#42645=CARTESIAN_POINT('Ctrl Pts',(3.66875283939545,-2.62875548050569,-10.2417200197346));
#42646=CARTESIAN_POINT('Ctrl Pts',(3.58862574672169,-2.61477767370391,-10.26479645276));
#42647=CARTESIAN_POINT('Ctrl Pts',(3.50808466559867,-2.6011553063792,-10.2871537896843));
#42648=CARTESIAN_POINT('Ctrl Pts',(3.42713923261638,-2.58790184224115,-10.3087818015856));
#42649=CARTESIAN_POINT('Ctrl Pts',(3.3869886980803,-2.58132786209191,-10.3195097229371));
#42650=CARTESIAN_POINT('Ctrl Pts',(3.34673867487783,-2.57484465155967,-10.3300581989155));
#42651=CARTESIAN_POINT('Ctrl Pts',(3.30639080102876,-2.56845356021827,-10.3404260905222));
#42652=CARTESIAN_POINT('Ctrl Pts',(3.24554522478032,-2.55881563885026,-10.3560611235267));
#42653=CARTESIAN_POINT('Ctrl Pts',(3.1844766843321,-2.54938754043835,-10.3712855031509));
#42654=CARTESIAN_POINT('Ctrl Pts',(3.12319004734369,-2.54017420676512,-10.3860953093476));
#42655=CARTESIAN_POINT('Ctrl Pts',(3.08513329993774,-2.53445306542668,-10.3952916542811));
#42656=CARTESIAN_POINT('Ctrl Pts',(3.04632095066816,-2.52871572983249,-10.4044864855534));
#42657=CARTESIAN_POINT('Ctrl Pts',(3.00800426616806,-2.52314921706523,-10.4133813072128));
#42658=CARTESIAN_POINT('Ctrl Pts',(2.98461571063522,-2.51975141021738,-10.4188107182656));
#42659=CARTESIAN_POINT('Ctrl Pts',(2.96141213571219,-2.51641677170785,-10.4241292288973));
#42660=CARTESIAN_POINT('Ctrl Pts',(2.93868070631794,-2.51318337406863,-10.4292769885392));
#42661=CARTESIAN_POINT('Ctrl Pts',(2.67982640696756,-2.47636303752467,-10.4878971347796));
#42662=CARTESIAN_POINT('Ctrl Pts',(2.41895243086841,-2.44400427296749,-10.5386806582089));
#42663=CARTESIAN_POINT('Ctrl Pts',(2.15650358185332,-2.41645036367251,-10.5815940612891));
#42664=CARTESIAN_POINT('Ctrl Pts',(2.00946578054502,-2.40101319846723,-10.6056364316757));
#42665=CARTESIAN_POINT('Ctrl Pts',(1.86193310803913,-2.38708447197652,-10.6272077902081));
#42666=CARTESIAN_POINT('Ctrl Pts',(1.71398017126471,-2.37472713185341,-10.6462966328573));
#42667=CARTESIAN_POINT('Ctrl Pts',(1.4531427413368,-2.35294144169592,-10.6799497982858));
#42668=CARTESIAN_POINT('Ctrl Pts',(1.19099999568001,-2.33603818365922,-10.705889511206));
#42669=CARTESIAN_POINT('Ctrl Pts',(0.928059192655602,-2.32412814711591,
-10.7241021511244));
#42670=CARTESIAN_POINT('Ctrl Pts',(0.66629372200498,-2.31227134784639,-10.7422333814439));
#42671=CARTESIAN_POINT('Ctrl Pts',(0.40373671189424,-2.30536303813329,-10.7527065306979));
#42672=CARTESIAN_POINT('Ctrl Pts',(0.14087630804359,-2.30353950361934,-10.7554660904619));
#42673=CARTESIAN_POINT('Ctrl Pts',(0.0945133613883472,-2.3032178711781,
-10.7559528177143));
#42674=CARTESIAN_POINT('Ctrl Pts',(0.0481409586041718,-2.30305449545756,
-10.7561994721505));
#42675=CARTESIAN_POINT('Ctrl Pts',(0.00176176044996187,-2.30305021913014,
-10.7562056100611));
#42676=CARTESIAN_POINT('Ctrl Pts',(0.00117444596505243,-2.30305016497765,
-10.7562056877874));
#42677=CARTESIAN_POINT('Ctrl Pts',(0.000587130390413492,-2.30305013633867,
-10.756205726944));
#42678=CARTESIAN_POINT('Ctrl Pts',(-1.86268554556318E-7,-2.30305013321116,
-10.7562057275312));
#42679=CARTESIAN_POINT('Ctrl Pts',(-0.255000491349255,-2.30304877531682,
-10.7562059824751));
#42680=CARTESIAN_POINT('Ctrl Pts',(-0.509774434758715,-2.30783485820167,
-10.7489431787096));
#42681=CARTESIAN_POINT('Ctrl Pts',(-0.763898932404416,-2.31730701398244,
-10.7344707880309));
#42682=CARTESIAN_POINT('Ctrl Pts',(-1.00372079461643,-2.32624605787451,
-10.7208129324705));
#42683=CARTESIAN_POINT('Ctrl Pts',(-1.24296459205544,-2.33935895111826,
-10.700733749856));
#42684=CARTESIAN_POINT('Ctrl Pts',(-1.48126244510556,-2.356582676509,-10.6742439838085));
#42685=CARTESIAN_POINT('Ctrl Pts',(-1.5577578438524,-2.36211162158679,-10.665740570158));
#42686=CARTESIAN_POINT('Ctrl Pts',(-1.63415741723896,-2.36805837750173,
-10.6565774625737));
#42687=CARTESIAN_POINT('Ctrl Pts',(-1.71044775245404,-2.37442125867848,
-10.6467543951761));
#42688=CARTESIAN_POINT('Ctrl Pts',(-1.87890328193537,-2.38847103988123,
-10.6250642293781));
#42689=CARTESIAN_POINT('Ctrl Pts',(-2.04682653109725,-2.40454952041417,
-10.6001567271322));
#42690=CARTESIAN_POINT('Ctrl Pts',(-2.21410026640134,-2.42257268343704,
-10.572046645807));
#42691=CARTESIAN_POINT('Ctrl Pts',(-2.33561469550333,-2.43566544041622,
-10.5516263420574));
#42692=CARTESIAN_POINT('Ctrl Pts',(-2.45678531457589,-2.44978651145652,
-10.5295155390599));
#42693=CARTESIAN_POINT('Ctrl Pts',(-2.57756645267151,-2.46490128099779,
-10.5057186054411));
#42694=CARTESIAN_POINT('Ctrl Pts',(-2.63795702171931,-2.47245866576843,
-10.4938201386317));
#42695=CARTESIAN_POINT('Ctrl Pts',(-2.69825021746175,-2.48026446967665,
-10.4815001146347));
#42696=CARTESIAN_POINT('Ctrl Pts',(-2.75844045211332,-2.48831371733907,
-10.4687590489619));
#42697=CARTESIAN_POINT('Ctrl Pts',(-2.795972562294,-2.49333289116164,-10.4608142538731));
#42698=CARTESIAN_POINT('Ctrl Pts',(-2.83278783471037,-2.49835393714893,
-10.4528528804943));
#42699=CARTESIAN_POINT('Ctrl Pts',(-2.87015176601266,-2.50354781733663,
-10.4446022649074));
#42700=CARTESIAN_POINT('Ctrl Pts',(-2.89270836094146,-2.5066833613605,-10.4396213705737));
#42701=CARTESIAN_POINT('Ctrl Pts',(-2.9154646728921,-2.50988236193164,-10.4345342417536));
#42702=CARTESIAN_POINT('Ctrl Pts',(-2.93869667983939,-2.5131867540875,-10.4292731465582));
#42703=CARTESIAN_POINT('Ctrl Pts',(-3.10185557320944,-2.5363935725356,-10.3923243598291));
#42704=CARTESIAN_POINT('Ctrl Pts',(-3.26352239546762,-2.56118034873841,
-10.3524399770393));
#42705=CARTESIAN_POINT('Ctrl Pts',(-3.42360171637816,-2.58742510026999,
-10.309700957847));
#42706=CARTESIAN_POINT('Ctrl Pts',(-3.67169453244662,-2.62809952515793,
-10.2434635227612));
#42707=CARTESIAN_POINT('Ctrl Pts',(-3.91597451893442,-2.67227397445666,
-10.1703712528922));
#42708=CARTESIAN_POINT('Ctrl Pts',(-4.15620380046542,-2.71944877115637,
-10.0907290824044));
#42709=CARTESIAN_POINT('Ctrl Pts',(-4.40438535371314,-2.76818518765174,
-10.0084505298079));
#42710=CARTESIAN_POINT('Ctrl Pts',(-4.64824377246369,-2.8201241159297,-9.91918128445061));
#42711=CARTESIAN_POINT('Ctrl Pts',(-4.88751685622871,-2.87475428965369,
-9.82321881397021));
#42712=CARTESIAN_POINT('Ctrl Pts',(-4.95392625599963,-2.88991670152762,
-9.79658476903352));
#42713=CARTESIAN_POINT('Ctrl Pts',(-5.01998242881333,-2.90528664210822,
-9.76943490709447));
#42714=CARTESIAN_POINT('Ctrl Pts',(-5.08567973802691,-2.92085365990828,
-9.74177507982081));
#42715=CARTESIAN_POINT('Ctrl Pts',(-5.30103361184729,-2.97188189268074,
-9.65110696838838));
#42716=CARTESIAN_POINT('Ctrl Pts',(-5.5125318672241,-3.02502631681574,-9.55496102222212));
#42717=CARTESIAN_POINT('Ctrl Pts',(-5.72001839641912,-3.07996751644906,
-9.45352532568119));
#42718=CARTESIAN_POINT('Ctrl Pts',(-5.71197198844382,-3.68829479791916,
-9.8501703687033));
#42719=CARTESIAN_POINT('Ctrl Pts',(-5.71754580782435,-3.68940667657091,
-9.84753623637226));
#42720=CARTESIAN_POINT('Ctrl Pts',(-5.76536778611043,-3.69987796915319,
-9.8245378123085));
#42721=CARTESIAN_POINT('Ctrl Pts',(-5.85070495630983,-3.73375492021359,
-9.77700012003639));
#42722=CARTESIAN_POINT('Ctrl Pts',(-5.94870719254402,-3.81192663887559,
-9.70547744306355));
#42723=CARTESIAN_POINT('Ctrl Pts',(-6.01636824229405,-3.91100725665301,
-9.6365907833745));
#42724=CARTESIAN_POINT('Ctrl Pts',(-6.04738225412035,-4.00919272256942,
-9.58227189268685));
#42725=CARTESIAN_POINT('Ctrl Pts',(-6.05143261400087,-4.07095169026726,
-9.55421326848555));
#42726=CARTESIAN_POINT('Ctrl Pts',(-6.05072985177984,-4.09544619788918,
-9.5440201179351));
#42727=CARTESIAN_POINT('Ctrl Pts',(-5.59589935073135,-3.61241520274072,
-9.56651528941115));
#42728=CARTESIAN_POINT('Ctrl Pts',(-5.60110010589582,-3.61342022961924,
-9.56406241085858));
#42729=CARTESIAN_POINT('Ctrl Pts',(-5.64572896520279,-3.62289723996144,
-9.5426450484337));
#42730=CARTESIAN_POINT('Ctrl Pts',(-5.72547570812964,-3.6537490789919,-9.49835555934878));
#42731=CARTESIAN_POINT('Ctrl Pts',(-5.81705924964759,-3.72520141233989,
-9.43184052695804));
#42732=CARTESIAN_POINT('Ctrl Pts',(-5.88013461718338,-3.81569531693298,
-9.3680978453068));
#42733=CARTESIAN_POINT('Ctrl Pts',(-5.90887905532575,-3.90498789181401,
-9.31830046586544));
#42734=CARTESIAN_POINT('Ctrl Pts',(-5.91259286860787,-3.96076595326123,
-9.29290817691202));
#42735=CARTESIAN_POINT('Ctrl Pts',(-5.91194771160934,-3.98280987749108,
-9.28374470677804));
#42736=CARTESIAN_POINT('Ctrl Pts',(-5.57877004579782,-3.33842765893124,
-9.41053844742967));
#42737=CARTESIAN_POINT('Ctrl Pts',(-5.58616524518609,-3.33985698600003,
-9.40710010435303));
#42738=CARTESIAN_POINT('Ctrl Pts',(-5.6495565331106,-3.35331617480298,-9.37712813939376));
#42739=CARTESIAN_POINT('Ctrl Pts',(-5.76186844825849,-3.39674464954052,
-9.31592123793131));
#42740=CARTESIAN_POINT('Ctrl Pts',(-5.89083814572667,-3.49676380958585,
-9.22450171582332));
#42741=CARTESIAN_POINT('Ctrl Pts',(-5.98103739468164,-3.62475240735847,
-9.13578477922984));
#42742=CARTESIAN_POINT('Ctrl Pts',(-6.0236413123101,-3.75450472600272,-9.0641622319954));
#42743=CARTESIAN_POINT('Ctrl Pts',(-6.02950682140399,-3.83881283105142,
-9.02585447175553));
#42744=CARTESIAN_POINT('Ctrl Pts',(-6.02849503592009,-3.87279257907653,
-9.01170707669297));
#42745=CARTESIAN_POINT('Ctrl Pts',(-5.67181053456004,-3.04590420482865,
-9.48446714171748));
#42746=CARTESIAN_POINT('Ctrl Pts',(-5.68252944195994,-3.04801089652616,
-9.4795224919317));
#42747=CARTESIAN_POINT('Ctrl Pts',(-5.77434175986858,-3.06781879365414,
-9.43646696993557));
#42748=CARTESIAN_POINT('Ctrl Pts',(-5.93603114512472,-3.13118288995348,
-9.34926475855966));
#42749=CARTESIAN_POINT('Ctrl Pts',(-6.12168886188134,-3.27633231152322,
-9.2193510829));
#42750=CARTESIAN_POINT('Ctrl Pts',(-6.25294449101188,-3.46332288353974,
-9.09190985330162));
#42751=CARTESIAN_POINT('Ctrl Pts',(-6.31645340122605,-3.6563701535287,-8.98641973386077));
#42752=CARTESIAN_POINT('Ctrl Pts',(-6.32554862134644,-3.78502058339552,
-8.92807953097214));
#42753=CARTESIAN_POINT('Ctrl Pts',(-6.32398626296098,-3.83749979088896,
-8.90620108365363));
#42754=CARTESIAN_POINT('',(-5.99998805436274,-3.9978865442048,-9.34661202445984));
#42755=CARTESIAN_POINT('',(-5.99999999729861,-3.21424235897937,-9.29218336212829));
#42756=CARTESIAN_POINT('Ctrl Pts',(-5.99998805436274,-3.9978865442048,-9.34661202445984));
#42757=CARTESIAN_POINT('Ctrl Pts',(-5.99998615757755,-3.97569967948952,
-9.33734483768274));
#42758=CARTESIAN_POINT('Ctrl Pts',(-5.99998787688148,-3.95340882073654,
-9.32855545295178));
#42759=CARTESIAN_POINT('Ctrl Pts',(-6.00000067043316,-3.9310658935729,-9.32034755058032));
#42760=CARTESIAN_POINT('Ctrl Pts',(-6.00000703302803,-3.91995412434894,
-9.31626552872632));
#42761=CARTESIAN_POINT('Ctrl Pts',(-6.00001548520134,-3.908829972833,-9.31232702313013));
#42762=CARTESIAN_POINT('Ctrl Pts',(-6.00002414590328,-3.89770276645304,
-9.30854234483346));
#42763=CARTESIAN_POINT('Ctrl Pts',(-6.00004249128253,-3.87413275763661,
-9.30052551673));
#42764=CARTESIAN_POINT('Ctrl Pts',(-6.00006348281536,-3.85054713585633,
-9.29320139494933));
#42765=CARTESIAN_POINT('Ctrl Pts',(-6.00008478134917,-3.82704822256206,
-9.28663239331664));
#42766=CARTESIAN_POINT('Ctrl Pts',(-6.00009878952125,-3.81159284783559,
-9.28231192195949));
#42767=CARTESIAN_POINT('Ctrl Pts',(-6.00011226036874,-3.79617570477161,
-9.27831732549394));
#42768=CARTESIAN_POINT('Ctrl Pts',(-6.00012161146963,-3.78083205625065,
-9.27465621621041));
#42769=CARTESIAN_POINT('Ctrl Pts',(-6.00013617109966,-3.75694205139138,
-9.26895588239122));
#42770=CARTESIAN_POINT('Ctrl Pts',(-6.00013962298854,-3.73322992383675,
-9.26406658182334));
#42771=CARTESIAN_POINT('Ctrl Pts',(-6.00012391442244,-3.70984226421294,
-9.25997601119208));
#42772=CARTESIAN_POINT('Ctrl Pts',(-6.00011963924351,-3.70347717468189,
-9.2588627382644));
#42773=CARTESIAN_POINT('Ctrl Pts',(-6.00011403061838,-3.69713617242992,
-9.25780834367095));
#42774=CARTESIAN_POINT('Ctrl Pts',(-6.00010715608015,-3.69082229089165,
-9.25681195952613));
#42775=CARTESIAN_POINT('Ctrl Pts',(-6.00010131553909,-3.68545807832469,
-9.25596544121266));
#42776=CARTESIAN_POINT('Ctrl Pts',(-6.00009456501949,-3.68011344099444,
-9.25516079029681));
#42777=CARTESIAN_POINT('Ctrl Pts',(-6.00008712855673,-3.67479011176827,
-9.25439735758586));
#42778=CARTESIAN_POINT('Ctrl Pts',(-6.00006858490899,-3.66151579774108,
-9.25249365313454));
#42779=CARTESIAN_POINT('Ctrl Pts',(-6.00005096959346,-3.64819250826683,
-9.25081521949727));
#42780=CARTESIAN_POINT('Ctrl Pts',(-6.00003052847771,-3.63505165735234,
-9.24939564882071));
#42781=CARTESIAN_POINT('Ctrl Pts',(-6.00000990265753,-3.62179206667071,
-9.2479632510074));
#42782=CARTESIAN_POINT('Ctrl Pts',(-5.99998594742847,-3.60871873802229,
-9.24679454187284));
#42783=CARTESIAN_POINT('Ctrl Pts',(-5.99996790995349,-3.5960857271278,-9.24587435399025));
#42784=CARTESIAN_POINT('Ctrl Pts',(-5.99995721318206,-3.58859396732476,
-9.24532865458038));
#42785=CARTESIAN_POINT('Ctrl Pts',(-5.99994889418915,-3.58125733395095,
-9.24486937940367));
#42786=CARTESIAN_POINT('Ctrl Pts',(-5.99994781651967,-3.57413028014663,
-9.24448539899825));
#42787=CARTESIAN_POINT('Ctrl Pts',(-5.99994381541193,-3.54766937478428,
-9.24305977917727));
#42788=CARTESIAN_POINT('Ctrl Pts',(-5.99996581464687,-3.52111758167283,
-9.24259217744035));
#42789=CARTESIAN_POINT('Ctrl Pts',(-5.99999344291283,-3.49464197784248,
-9.2431668105431));
#42790=CARTESIAN_POINT('Ctrl Pts',(-6.00002107117879,-3.46816637401214,
-9.24374144364584));
#42791=CARTESIAN_POINT('Ctrl Pts',(-6.00005342999203,-3.4417680087858,-9.24535888815406));
#42792=CARTESIAN_POINT('Ctrl Pts',(-6.00007273963438,-3.4156408295774,-9.24804717908462));
#42793=CARTESIAN_POINT('Ctrl Pts',(-6.0000911444452,-3.39073794520572,-9.25060949925195));
#42794=CARTESIAN_POINT('Ctrl Pts',(-6.00009742310507,-3.36608229990409,
-9.25414433396963));
#42795=CARTESIAN_POINT('Ctrl Pts',(-6.00008958768821,-3.34184650386147,
-9.25862572524751));
#42796=CARTESIAN_POINT('Ctrl Pts',(-6.00008165516822,-3.31731035726507,
-9.26316265372952));
#42797=CARTESIAN_POINT('Ctrl Pts',(-6.000058850835,-3.29320556340356,-9.26866951866689));
#42798=CARTESIAN_POINT('Ctrl Pts',(-6.00003612101861,-3.26970688957186,
-9.27506846759169));
#42799=CARTESIAN_POINT('Ctrl Pts',(-6.00001783142877,-3.25079863713838,
-9.28021739397136));
#42800=CARTESIAN_POINT('Ctrl Pts',(-5.99999992125698,-3.23228289786736,
-9.28594277002995));
#42801=CARTESIAN_POINT('Ctrl Pts',(-5.99999992406984,-3.21424228989424,
-9.29218316240729));
#42802=CARTESIAN_POINT('Ctrl Pts',(-5.72001867921778,-3.07996774527742,
-9.45352602808894));
#42803=CARTESIAN_POINT('Ctrl Pts',(-5.77261523598685,-3.09390413589055,
-9.42780998495483));
#42804=CARTESIAN_POINT('Ctrl Pts',(-5.82214285829514,-3.11233855179879,
-9.40146116709804));
#42805=CARTESIAN_POINT('Ctrl Pts',(-5.86877313173194,-3.13479324096957,
-9.37456642764042));
#42806=CARTESIAN_POINT('Ctrl Pts',(-5.91540340287037,-3.15724792903357,
-9.34767168950842));
#42807=CARTESIAN_POINT('Ctrl Pts',(-5.95913655250815,-3.18372307206963,
-9.32023156202287));
#42808=CARTESIAN_POINT('Ctrl Pts',(-6.00000008491191,-3.21424242024491,
-9.29218355643704));
#42809=CARTESIAN_POINT('Ctrl Pts',(-5.73278520692685,-3.68907667907205,
-9.8154362792223));
#42810=CARTESIAN_POINT('Ctrl Pts',(-5.74762382962131,-3.69180325511032,
-9.80082774594881));
#42811=CARTESIAN_POINT('Ctrl Pts',(-5.76162171238064,-3.69529215425996,
-9.78641524403596));
#42812=CARTESIAN_POINT('Ctrl Pts',(-5.77477721800093,-3.69934156434397,
-9.77230761864449));
#42813=CARTESIAN_POINT('Ctrl Pts',(-5.78880577316832,-3.70365970873147,
-9.75726375740514));
#42814=CARTESIAN_POINT('Ctrl Pts',(-5.80187658368747,-3.70861550222048,
-9.74256647678676));
#42815=CARTESIAN_POINT('Ctrl Pts',(-5.81401568052954,-3.71400533038411,
-9.72831583026195));
#42816=CARTESIAN_POINT('Ctrl Pts',(-5.81729336960867,-3.71546064301076,
-9.7244679996455));
#42817=CARTESIAN_POINT('Ctrl Pts',(-5.8205032728521,-3.71694780460071,-9.72065256683664));
#42818=CARTESIAN_POINT('Ctrl Pts',(-5.82364619983945,-3.71846323640865,
-9.71687115362401));
#42819=CARTESIAN_POINT('Ctrl Pts',(-5.83610465210455,-3.7244703549056,-9.70188176437192));
#42820=CARTESIAN_POINT('Ctrl Pts',(-5.84750972960467,-3.73091750184809,
-9.6874295362641));
#42821=CARTESIAN_POINT('Ctrl Pts',(-5.85794382570231,-3.73757946624391,
-9.67360152486396));
#42822=CARTESIAN_POINT('Ctrl Pts',(-5.8688044299202,-3.74451374765551,-9.65920827435793));
#42823=CARTESIAN_POINT('Ctrl Pts',(-5.878613435895,-3.75168144867336,-9.64549094512086));
#42824=CARTESIAN_POINT('Ctrl Pts',(-5.88747619597288,-3.75888048322723,
-9.6325145729761));
#42825=CARTESIAN_POINT('Ctrl Pts',(-5.89165259807077,-3.76227288725818,
-9.6263997117622));
#42826=CARTESIAN_POINT('Ctrl Pts',(-5.89561902734608,-3.76567292020307,
-9.62044895431379));
#42827=CARTESIAN_POINT('Ctrl Pts',(-5.89938714503697,-3.76906266936731,
-9.61466703946109));
#42828=CARTESIAN_POINT('Ctrl Pts',(-5.90174440457449,-3.7711832290745,-9.61104998844258));
#42829=CARTESIAN_POINT('Ctrl Pts',(-5.90402406175946,-3.77329980253791,
-9.6074989896858));
#42830=CARTESIAN_POINT('Ctrl Pts',(-5.9062290268245,-3.77540836081767,-9.60401497849346));
#42831=CARTESIAN_POINT('Ctrl Pts',(-5.90952625901899,-3.77856142947814,
-9.59880510281265));
#42832=CARTESIAN_POINT('Ctrl Pts',(-5.91265649617662,-3.78169648827022,
-9.59374505629813));
#42833=CARTESIAN_POINT('Ctrl Pts',(-5.91563044428714,-3.78480001737202,
-9.58883752575352));
#42834=CARTESIAN_POINT('Ctrl Pts',(-5.91811180565001,-3.78738949671584,
-9.58474284883651));
#42835=CARTESIAN_POINT('Ctrl Pts',(-5.920484295981,-3.78995698533474,-9.58075441007369));
#42836=CARTESIAN_POINT('Ctrl Pts',(-5.92275407850264,-3.79249552701193,
-9.57687328474074));
#42837=CARTESIAN_POINT('Ctrl Pts',(-5.92388896976347,-3.79376479785053,
-9.57493272207426));
#42838=CARTESIAN_POINT('Ctrl Pts',(-5.92499817681059,-3.79502683695038,
-9.57301898699673));
#42839=CARTESIAN_POINT('Ctrl Pts',(-5.92608244824651,-3.79628082871286,
-9.571132197062));
#42840=CARTESIAN_POINT('Ctrl Pts',(-5.92684317282743,-3.79716062903442,
-9.56980842569366));
#42841=CARTESIAN_POINT('Ctrl Pts',(-5.92727871378404,-3.79766914381903,
-9.56904606582659));
#42842=CARTESIAN_POINT('Ctrl Pts',(-5.928049092874,-3.79857833855905,-9.56769139022369));
#42843=CARTESIAN_POINT('Ctrl Pts',(-5.92837674592737,-3.79896503185922,
-9.56711522765203));
#42844=CARTESIAN_POINT('Ctrl Pts',(-5.92876465306642,-3.79942445551461,
-9.56643192389701));
#42845=CARTESIAN_POINT('Ctrl Pts',(-5.92926118432832,-3.80001787185852,
-9.56555277030981));
#42846=CARTESIAN_POINT('Ctrl Pts',(-5.9392063852684,-3.81190361850559,-9.54794389096479));
#42847=CARTESIAN_POINT('Ctrl Pts',(-5.94794390660985,-3.82419219851774,
-9.5309806794631));
#42848=CARTESIAN_POINT('Ctrl Pts',(-5.95555097031253,-3.83668111574082,
-9.51474001570556));
#42849=CARTESIAN_POINT('Ctrl Pts',(-5.95867322267065,-3.84180708191834,
-9.50807417817662));
#42850=CARTESIAN_POINT('Ctrl Pts',(-5.96160508865422,-3.84696733110998,
-9.50152971460728));
#42851=CARTESIAN_POINT('Ctrl Pts',(-5.96435219187444,-3.85214989453163,
-9.49511056986388));
#42852=CARTESIAN_POINT('Ctrl Pts',(-5.97117112933457,-3.86501420031934,
-9.4791767868773));
#42853=CARTESIAN_POINT('Ctrl Pts',(-5.9768525793462,-3.87801257167857,-9.46401683414202));
#42854=CARTESIAN_POINT('Ctrl Pts',(-5.98152771173936,-3.89095751760361,
-9.44967300324281));
#42855=CARTESIAN_POINT('Ctrl Pts',(-5.98650278304255,-3.90473296257011,
-9.43440892610375));
#42856=CARTESIAN_POINT('Ctrl Pts',(-5.99033781740992,-3.91844820403234,
-9.4200690225312));
#42857=CARTESIAN_POINT('Ctrl Pts',(-5.99318392794507,-3.93192830023576,
-9.40667643182402));
#42858=CARTESIAN_POINT('Ctrl Pts',(-5.99387721931419,-3.93521195146339,
-9.40341409628478));
#42859=CARTESIAN_POINT('Ctrl Pts',(-5.99451181801508,-3.9384818624222,-9.40020785074143));
#42860=CARTESIAN_POINT('Ctrl Pts',(-5.99508989597192,-3.94173589648596,
-9.39705780395256));
#42861=CARTESIAN_POINT('Ctrl Pts',(-5.99756671015925,-3.95567802598549,
-9.38356121498038));
#42862=CARTESIAN_POINT('Ctrl Pts',(-5.99900795538788,-3.96932498629971,
-9.37109761283901));
#42863=CARTESIAN_POINT('Ctrl Pts',(-5.99962729227282,-3.98252532525775,
-9.35964972360189));
#42864=CARTESIAN_POINT('Ctrl Pts',(-5.99987086536048,-3.9877167604788,-9.35514749259242));
#42865=CARTESIAN_POINT('Ctrl Pts',(-5.99998706574566,-3.99283961991828,
-9.35080217488171));
#42866=CARTESIAN_POINT('Ctrl Pts',(-5.99998805436274,-3.99788654420479,
-9.34661202445984));
#42867=CARTESIAN_POINT('Ctrl Pts',(-5.72202476730477,-9.61344956113702,
-17.4236870238206));
#42868=CARTESIAN_POINT('Ctrl Pts',(-5.72274570226849,-9.17589143465609,
-17.2270248402683));
#42869=CARTESIAN_POINT('Ctrl Pts',(-5.72404124879816,-8.29086215801847,
-16.7525775515301));
#42870=CARTESIAN_POINT('Ctrl Pts',(-5.72530541068372,-7.06378515805125,
-15.8436322695082));
#42871=CARTESIAN_POINT('Ctrl Pts',(-5.72546532299495,-5.95933659063332,
-14.7303948480276));
#42872=CARTESIAN_POINT('Ctrl Pts',(-5.72471356214735,-5.03570890150477,
-13.4633046799478));
#42873=CARTESIAN_POINT('Ctrl Pts',(-5.72306575818266,-4.31359100517564,
-12.0712170809002));
#42874=CARTESIAN_POINT('Ctrl Pts',(-5.72038904755586,-3.83840722052135,
-10.6678390314501));
#42875=CARTESIAN_POINT('Ctrl Pts',(-5.71829743871595,-3.65952910665459,
-9.72608608764783));
#42876=CARTESIAN_POINT('Ctrl Pts',(-5.71724185222974,-3.60559726864913,
-9.29489095839975));
#42877=CARTESIAN_POINT('Ctrl Pts',(-5.90002717726106,-9.63679765643431,
-17.3716665606242));
#42878=CARTESIAN_POINT('Ctrl Pts',(-5.90064014424208,-9.20180701959731,
-17.1757873397771));
#42879=CARTESIAN_POINT('Ctrl Pts',(-5.90174038137585,-8.32197996147983,
-16.7034325008754));
#42880=CARTESIAN_POINT('Ctrl Pts',(-5.90280993369199,-7.10225209295494,
-15.7991883436704));
#42881=CARTESIAN_POINT('Ctrl Pts',(-5.90294519188033,-6.00412592355956,
-14.6922158654566));
#42882=CARTESIAN_POINT('Ctrl Pts',(-5.90230921958852,-5.08548723943647,
-13.4325714280488));
#42883=CARTESIAN_POINT('Ctrl Pts',(-5.9009135213621,-4.36673044058498,-12.048661604341));
#42884=CARTESIAN_POINT('Ctrl Pts',(-5.89863582611894,-3.89298817613705,
-10.6534829599988));
#42885=CARTESIAN_POINT('Ctrl Pts',(-5.89685148833867,-3.71409960335627,
-9.71696543058244));
#42886=CARTESIAN_POINT('Ctrl Pts',(-5.89594501973261,-3.65996390017634,
-9.2881333735693));
#42887=CARTESIAN_POINT('Ctrl Pts',(-6.00727960514337,-9.69953310260925,
-17.2318896281666));
#42888=CARTESIAN_POINT('Ctrl Pts',(-6.00760257008453,-9.27115360051871,
-17.0387552962051));
#42889=CARTESIAN_POINT('Ctrl Pts',(-6.00818063783358,-8.40460281232898,
-16.573090076404));
#42890=CARTESIAN_POINT('Ctrl Pts',(-6.00873745913476,-7.20353593893208,
-15.6822226095155));
#42891=CARTESIAN_POINT('Ctrl Pts',(-6.00880782934474,-6.12189755288578,
-14.5918038255627));
#42892=CARTESIAN_POINT('Ctrl Pts',(-6.00847681114424,-5.2169700002139,-13.3513285148959));
#42893=CARTESIAN_POINT('Ctrl Pts',(-6.00774820020079,-4.50853269808651,
-11.9883509755523));
#42894=CARTESIAN_POINT('Ctrl Pts',(-6.00654575904665,-4.04115736338279,
-10.6143706750423));
#42895=CARTESIAN_POINT('Ctrl Pts',(-6.00559803258962,-3.86430082012095,
-9.691815921938));
#42896=CARTESIAN_POINT('Ctrl Pts',(-6.00510903930179,-3.81065842092309,
-9.26940249172137));
#42897=CARTESIAN_POINT('Ctrl Pts',(-5.99966802959142,-9.77609339016483,
-17.0613104586777));
#42898=CARTESIAN_POINT('Ctrl Pts',(-5.99963712428367,-9.35567454107366,
-16.8717652077172));
#42899=CARTESIAN_POINT('Ctrl Pts',(-5.99957893141052,-8.50506367644026,
-16.4146621757356));
#42900=CARTESIAN_POINT('Ctrl Pts',(-5.99951383159447,-7.3263647493401,-15.5403972571897));
#42901=CARTESIAN_POINT('Ctrl Pts',(-5.99950552107023,-6.2646607784291,-14.4700755533922));
#42902=CARTESIAN_POINT('Ctrl Pts',(-5.9995443574713,-5.37658001505559,-13.2526810833737));
#42903=CARTESIAN_POINT('Ctrl Pts',(-5.99962598905998,-4.68121720532413,
-11.9148600033795));
#42904=CARTESIAN_POINT('Ctrl Pts',(-5.99973691556681,-4.22254267934907,
-10.5664384725443));
#42905=CARTESIAN_POINT('Ctrl Pts',(-5.99981426292777,-4.04893496254998,
-9.66088439635348));
#42906=CARTESIAN_POINT('Ctrl Pts',(-5.99984101441889,-3.9962831894273,-9.24632985745589));
#42907=CARTESIAN_POINT('',(-5.99999988467789,-9.67863428828651,-17.0348543136794));
#42908=CARTESIAN_POINT('Origin',(-5.59998164336546,-9.67863961984266,-17.0348438488183));
#42909=CARTESIAN_POINT('Ctrl Pts',(-6.,-9.67863396518321,-17.0348526023082));
#42910=CARTESIAN_POINT('Ctrl Pts',(-6.,-9.24640194919319,-16.8355809092864));
#42911=CARTESIAN_POINT('Ctrl Pts',(-6.,-8.83275508583899,-16.6077872915085));
#42912=CARTESIAN_POINT('Ctrl Pts',(-6.,-8.43516132001025,-16.3499544374811));
#42913=CARTESIAN_POINT('Ctrl Pts',(-6.,-8.03756727297484,-16.092121401096));
#42914=CARTESIAN_POINT('Ctrl Pts',(-6.,-7.65602634617269,-15.8042490859695));
#42915=CARTESIAN_POINT('Ctrl Pts',(-6.,-7.29796322174819,-15.4912222292012));
#42916=CARTESIAN_POINT('Ctrl Pts',(-6.,-6.93990009732394,-15.1781953724331));
#42917=CARTESIAN_POINT('Ctrl Pts',(-6.,-6.6053147752773,-14.8400139740232));
#42918=CARTESIAN_POINT('Ctrl Pts',(-6.,-6.29607548316964,-14.4788351250848));
#42919=CARTESIAN_POINT('Ctrl Pts',(-6.,-5.98683619106177,-14.1176562761461));
#42920=CARTESIAN_POINT('Ctrl Pts',(-6.,-5.70294292889293,-13.733479976679));
#42921=CARTESIAN_POINT('Ctrl Pts',(-6.,-5.44842667128605,-13.331796225766));
#42922=CARTESIAN_POINT('Ctrl Pts',(-6.,-5.19391041367936,-12.9301124748532));
#42923=CARTESIAN_POINT('Ctrl Pts',(-6.,-4.9687711606346,-12.5109212724947));
#42924=CARTESIAN_POINT('Ctrl Pts',(-6.,-4.77466771540665,-12.0768285359646));
#42925=CARTESIAN_POINT('Ctrl Pts',(-6.,-4.58056427017856,-11.6427357994341));
#42926=CARTESIAN_POINT('Ctrl Pts',(-6.,-4.41749663276733,-11.1937415287322));
#42927=CARTESIAN_POINT('Ctrl Pts',(-6.,-4.28772377567829,-10.7378297759092));
#42928=CARTESIAN_POINT('Ctrl Pts',(-6.,-4.15795091858935,-10.2819180230865));
#42929=CARTESIAN_POINT('Ctrl Pts',(-6.,-4.06147284182256,-9.8190887881429));
#42930=CARTESIAN_POINT('Ctrl Pts',(-6.,-3.99788654320472,-9.34661202518238));
#42931=CARTESIAN_POINT('Origin',(-5.599999999997,-9.6786310860259,-17.0348569100619));
#42932=CARTESIAN_POINT('Origin',(-5.6,-9.67863108604804,-17.0348569101035));
#42933=CARTESIAN_POINT('Ctrl Pts',(-6.05070079238961,-6.2176939973095,-8.31864695491407));
#42934=CARTESIAN_POINT('Ctrl Pts',(-6.05139768547269,-6.23880305073253,
-8.30250772584274));
#42935=CARTESIAN_POINT('Ctrl Pts',(-6.04731850243085,-6.29402509020919,
-8.26303317773159));
#42936=CARTESIAN_POINT('Ctrl Pts',(-6.01624003938889,-6.39018722730729,
-8.20516961886834));
#42937=CARTESIAN_POINT('Ctrl Pts',(-5.94855011433123,-6.49933487298712,
-8.15385676121418));
#42938=CARTESIAN_POINT('Ctrl Pts',(-5.85055911347944,-6.60029897666562,
-8.12196082013419));
#42939=CARTESIAN_POINT('Ctrl Pts',(-5.76530777443809,-6.65832830405139,
-8.11641163255942));
#42940=CARTESIAN_POINT('Ctrl Pts',(-5.71755809134908,-6.68344389358587,
-8.11883822207412));
#42941=CARTESIAN_POINT('Ctrl Pts',(-5.71204816250035,-6.68624967619076,
-8.11918746206646));
#42942=CARTESIAN_POINT('Ctrl Pts',(-5.91199124611904,-6.04862265685342,
-8.09100626630052));
#42943=CARTESIAN_POINT('Ctrl Pts',(-5.91263110712145,-6.06761428475678,
-8.07647455597469));
#42944=CARTESIAN_POINT('Ctrl Pts',(-5.90889016285839,-6.11754050550086,
-8.04084303944076));
#42945=CARTESIAN_POINT('Ctrl Pts',(-5.8800819863844,-6.20535025391518,-7.98841262080049));
#42946=CARTESIAN_POINT('Ctrl Pts',(-5.81697232658341,-6.30576567345289,
-7.9419541048996));
#42947=CARTESIAN_POINT('Ctrl Pts',(-5.72538958464469,-6.39904806928683,
-7.91336636114985));
#42948=CARTESIAN_POINT('Ctrl Pts',(-5.64571477447322,-6.45276327292691,
-7.90880982817913));
#42949=CARTESIAN_POINT('Ctrl Pts',(-5.60114858206858,-6.47601774174994,
-7.91130704060933));
#42950=CARTESIAN_POINT('Ctrl Pts',(-5.59600687463879,-6.47861573314325,
-7.91165826841064));
#42951=CARTESIAN_POINT('Ctrl Pts',(-6.02851383329436,-5.86812573387379,
-7.8597274090204));
#42952=CARTESIAN_POINT('Ctrl Pts',(-6.02951717986534,-5.89741436718577,
-7.83734246590686));
#42953=CARTESIAN_POINT('Ctrl Pts',(-6.02361102927941,-5.97279895728111,
-7.78345987269494));
#42954=CARTESIAN_POINT('Ctrl Pts',(-5.98092154264836,-6.0997335165731,-7.70691568628475));
#42955=CARTESIAN_POINT('Ctrl Pts',(-5.89068578849719,-6.24049313343636,
-7.64049778117552));
#42956=CARTESIAN_POINT('Ctrl Pts',(-5.7617298699184,-6.36959713087669,-7.59964063210728));
#42957=CARTESIAN_POINT('Ctrl Pts',(-5.64952879318203,-6.44421982544224,
-7.5926595670497));
#42958=CARTESIAN_POINT('Ctrl Pts',(-5.58623246546378,-6.47685794718921,
-7.59598379230037));
#42959=CARTESIAN_POINT('Ctrl Pts',(-5.57892201417051,-6.48050945436716,
-7.596458488021));
#42960=CARTESIAN_POINT('Ctrl Pts',(-6.32392448294239,-5.79446202133885,
-7.77634070202551));
#42961=CARTESIAN_POINT('Ctrl Pts',(-6.32547368216801,-5.83971563927917,
-7.74178710117615));
#42962=CARTESIAN_POINT('Ctrl Pts',(-6.31631749247212,-5.9546328246946,-7.65951716937307));
#42963=CARTESIAN_POINT('Ctrl Pts',(-6.25268993559297,-6.14253537363754,
-7.54511130591315));
#42964=CARTESIAN_POINT('Ctrl Pts',(-6.12139435816593,-6.34628266567896,
-7.44699738981473));
#42965=CARTESIAN_POINT('Ctrl Pts',(-5.93577020055708,-6.53124176918286,
-7.38633197376381));
#42966=CARTESIAN_POINT('Ctrl Pts',(-5.77425080851983,-6.63829527819499,
-7.37509770946464));
#42967=CARTESIAN_POINT('Ctrl Pts',(-5.6825824374102,-6.68541379044458,-7.37946349065171));
#42968=CARTESIAN_POINT('Ctrl Pts',(-5.67198720706453,-6.69068987183275,
-7.3801022400051));
#42969=CARTESIAN_POINT('',(-5.73278770456533,-6.6558833922326,-8.10254681684203));
#42970=CARTESIAN_POINT('',(-5.72001815523952,-6.64700891660902,-7.39409230498819));
#42971=CARTESIAN_POINT('Origin',(-5.8987602805625,-6.95917384373578,-7.74135788191406));
#42972=CARTESIAN_POINT('',(-5.99999999681378,-6.44014573036754,-7.42970716684666));
#42973=CARTESIAN_POINT('Ctrl Pts',(-6.0000000832888,-6.44014586670658,-7.42970731664913));
#42974=CARTESIAN_POINT('Ctrl Pts',(-5.95915137667849,-6.47968145316765,
-7.41730531005402));
#42975=CARTESIAN_POINT('Ctrl Pts',(-5.91542827660156,-6.5166771191331,-7.40809722880095));
#42976=CARTESIAN_POINT('Ctrl Pts',(-5.868798937096,-6.55119699478441,-7.40209707843446));
#42977=CARTESIAN_POINT('Ctrl Pts',(-5.82216959558716,-6.58571687191874,
-7.39609692781019));
#42978=CARTESIAN_POINT('Ctrl Pts',(-5.77263377981968,-6.6177605887956,-7.39330427821582));
#42979=CARTESIAN_POINT('Ctrl Pts',(-5.72001867762135,-6.64700982892112,
-7.39409331981127));
#42980=CARTESIAN_POINT('',(-5.99998808311055,-6.09546019408016,-8.13557730954211));
#42981=CARTESIAN_POINT('Ctrl Pts',(-5.99998808311055,-6.09546019408016,
-8.13557730954211));
#42982=CARTESIAN_POINT('Ctrl Pts',(-5.99998579341257,-6.09905757126837,
-8.1076121115612));
#42983=CARTESIAN_POINT('Ctrl Pts',(-5.99998684302836,-6.10332349437861,
-8.08015310005243));
#42984=CARTESIAN_POINT('Ctrl Pts',(-5.99998299213941,-6.10828599559105,
-8.05321832362444));
#42985=CARTESIAN_POINT('Ctrl Pts',(-5.99998186316054,-6.10974086979519,
-8.04532175902083));
#42986=CARTESIAN_POINT('Ctrl Pts',(-5.99998012470112,-6.11125530650231,
-8.03747020572751));
#42987=CARTESIAN_POINT('Ctrl Pts',(-5.99997728564091,-6.11282931570554,
-8.02966396994754));
#42988=CARTESIAN_POINT('Ctrl Pts',(-5.99996366274466,-6.12038201360534,
-7.99220666635636));
#42989=CARTESIAN_POINT('Ctrl Pts',(-5.99992845213204,-6.12930815877995,
-7.95579590653871));
#42990=CARTESIAN_POINT('Ctrl Pts',(-5.99991578864617,-6.13957445794852,
-7.92039221214192));
#42991=CARTESIAN_POINT('Ctrl Pts',(-5.99991509179514,-6.14013939569574,
-7.91844400441608));
#42992=CARTESIAN_POINT('Ctrl Pts',(-5.99991445763287,-6.14070839032029,
-7.91649883611599));
#42993=CARTESIAN_POINT('Ctrl Pts',(-5.99991389241991,-6.14128143696332,
-7.91455669723407));
#42994=CARTESIAN_POINT('Ctrl Pts',(-5.99990495768377,-6.15034000586679,
-7.88385588239449));
#42995=CARTESIAN_POINT('Ctrl Pts',(-5.99990284924714,-6.16043170965493,
-7.85392609166195));
#42996=CARTESIAN_POINT('Ctrl Pts',(-5.99990385986942,-6.17154887581139,
-7.82477895973108));
#42997=CARTESIAN_POINT('Ctrl Pts',(-5.99990456954584,-6.17935554187285,
-7.8043113403368));
#42998=CARTESIAN_POINT('Ctrl Pts',(-5.99990725999096,-6.18766785808837,
-7.78422897762939));
#42999=CARTESIAN_POINT('Ctrl Pts',(-5.99991517244305,-6.1964942566548,-7.76452836981471));
#43000=CARTESIAN_POINT('Ctrl Pts',(-5.999918104499,-6.1997649866577,-7.75722806850045));
#43001=CARTESIAN_POINT('Ctrl Pts',(-5.9999261926437,-6.20321482930646,-7.74973181446826));
#43002=CARTESIAN_POINT('Ctrl Pts',(-5.99993157519488,-6.20670228942552,
-7.74238378435717));
#43003=CARTESIAN_POINT('Ctrl Pts',(-5.99993702627722,-6.21023415222328,
-7.73494219841775));
#43004=CARTESIAN_POINT('Ctrl Pts',(-5.99993942941342,-6.21380446476958,
-7.72765294100298));
#43005=CARTESIAN_POINT('Ctrl Pts',(-5.99994447142085,-6.21721465616354,
-7.72086215695556));
#43006=CARTESIAN_POINT('Ctrl Pts',(-5.99994530679784,-6.21777966831269,
-7.71973703667761));
#43007=CARTESIAN_POINT('Ctrl Pts',(-5.99994624919116,-6.21834017787097,
-7.7186255700337));
#43008=CARTESIAN_POINT('Ctrl Pts',(-5.99994736554133,-6.21889515985152,
-7.71752929521157));
#43009=CARTESIAN_POINT('Ctrl Pts',(-5.99997424180662,-6.23225641805852,
-7.69113634647166));
#43010=CARTESIAN_POINT('Ctrl Pts',(-5.99996041212331,-6.24653889545146,
-7.66574508274203));
#43011=CARTESIAN_POINT('Ctrl Pts',(-5.99993586626681,-6.26166900270897,
-7.6413218863139));
#43012=CARTESIAN_POINT('Ctrl Pts',(-5.99991529890311,-6.27434676030037,
-7.6208573014532));
#43013=CARTESIAN_POINT('Ctrl Pts',(-5.99988811606785,-6.2876205692234,-7.60107176789985));
#43014=CARTESIAN_POINT('Ctrl Pts',(-5.99987116820446,-6.30147515965944,
-7.58195086878649));
#43015=CARTESIAN_POINT('Ctrl Pts',(-5.99985202391289,-6.31712529282017,
-7.56035191797967));
#43016=CARTESIAN_POINT('Ctrl Pts',(-5.99984750492891,-6.33351668140582,
-7.53959965094863));
#43017=CARTESIAN_POINT('Ctrl Pts',(-5.99986528484166,-6.35066442453289,
-7.51969184647213));
#43018=CARTESIAN_POINT('Ctrl Pts',(-5.99988250987291,-6.36727701511488,
-7.50040533146525));
#43019=CARTESIAN_POINT('Ctrl Pts',(-5.99992124591386,-6.38460059983747,
-7.48191118790163));
#43020=CARTESIAN_POINT('Ctrl Pts',(-5.99995587754498,-6.40266648904051,
-7.4642385727826));
#43021=CARTESIAN_POINT('Ctrl Pts',(-5.99997917503714,-6.41481982685424,
-7.45234979946069));
#43022=CARTESIAN_POINT('Ctrl Pts',(-5.99999991524962,-6.42730946144769,
-7.44083350199229));
#43023=CARTESIAN_POINT('Ctrl Pts',(-5.99999992273984,-6.44014559311225,
-7.4297070085014));
#43024=CARTESIAN_POINT('Ctrl Pts',(-5.99998808311055,-6.09546019408016,
-8.13557730954211));
#43025=CARTESIAN_POINT('Ctrl Pts',(-5.99998551891527,-6.11109455318528,
-8.12979418173387));
#43026=CARTESIAN_POINT('Ctrl Pts',(-5.9992401947774,-6.12784559555232,-8.12408493904144));
#43027=CARTESIAN_POINT('Ctrl Pts',(-5.99754680984414,-6.14566703424288,
-8.1185774313553));
#43028=CARTESIAN_POINT('Ctrl Pts',(-5.99687196598229,-6.15276919292727,
-8.11638259208213));
#43029=CARTESIAN_POINT('Ctrl Pts',(-5.99604634715655,-6.16004095183898,
-8.11422011573065));
#43030=CARTESIAN_POINT('Ctrl Pts',(-5.99505598209878,-6.16747772038915,
-8.11209946841976));
#43031=CARTESIAN_POINT('Ctrl Pts',(-5.99264929774847,-6.18554979830235,
-8.10694608719373));
#43032=CARTESIAN_POINT('Ctrl Pts',(-5.9892694657102,-6.20459955905458,-8.10203798932087));
#43033=CARTESIAN_POINT('Ctrl Pts',(-5.98476114151186,-6.22452690538448,
-8.0975132784811));
#43034=CARTESIAN_POINT('Ctrl Pts',(-5.98055933700287,-6.24309939706376,
-8.09329620145381));
#43035=CARTESIAN_POINT('Ctrl Pts',(-5.97537763983944,-6.2624343485505,-8.08941191476389));
#43036=CARTESIAN_POINT('Ctrl Pts',(-5.96908598759027,-6.2824110980282,-8.08599595429554));
#43037=CARTESIAN_POINT('Ctrl Pts',(-5.96754611749363,-6.28730037002395,
-8.08515990437285));
#43038=CARTESIAN_POINT('Ctrl Pts',(-5.96593972255001,-6.29222788468966,
-8.08435203394631));
#43039=CARTESIAN_POINT('Ctrl Pts',(-5.96426481096664,-6.29719146243715,
-8.08357459006554));
#43040=CARTESIAN_POINT('Ctrl Pts',(-5.96381007642168,-6.29853906209006,
-8.08336351588535));
#43041=CARTESIAN_POINT('Ctrl Pts',(-5.9633502911682,-6.29988931898542,-8.08315468514074));
#43042=CARTESIAN_POINT('Ctrl Pts',(-5.96288542938708,-6.30124219280347,
-8.08294813476418));
#43043=CARTESIAN_POINT('Ctrl Pts',(-5.9582989837985,-6.3145899929598,-8.08091025576045));
#43044=CARTESIAN_POINT('Ctrl Pts',(-5.95321825970403,-6.32819323848442,
-8.07909402244848));
#43045=CARTESIAN_POINT('Ctrl Pts',(-5.94761928847918,-6.34200851301402,
-8.0775370834204));
#43046=CARTESIAN_POINT('Ctrl Pts',(-5.94481980286676,-6.34891615027881,
-8.07675861390635));
#43047=CARTESIAN_POINT('Ctrl Pts',(-5.94189071345292,-6.3558767794314,-8.07604498720728));
#43048=CARTESIAN_POINT('Ctrl Pts',(-5.93882920449365,-6.36288396966655,
-8.07540138572607));
#43049=CARTESIAN_POINT('Ctrl Pts',(-5.93729845001401,-6.36638756478413,
-8.07507958498547));
#43050=CARTESIAN_POINT('Ctrl Pts',(-5.93573458735359,-6.36990279902876,
-8.07477529198379));
#43051=CARTESIAN_POINT('Ctrl Pts',(-5.93413726064459,-6.373428827563,-8.07448917805385));
#43052=CARTESIAN_POINT('Ctrl Pts',(-5.93307815068233,-6.37576676627447,
-8.07429946976698));
#43053=CARTESIAN_POINT('Ctrl Pts',(-5.93173234134964,-6.37870044829973,
-8.07407323849032));
#43054=CARTESIAN_POINT('Ctrl Pts',(-5.93063879363215,-6.38105333357039,
-8.07390055787731));
#43055=CARTESIAN_POINT('Ctrl Pts',(-5.93008307636399,-6.38224901891086,
-8.07381280532935));
#43056=CARTESIAN_POINT('Ctrl Pts',(-5.92959342492817,-6.38329503672707,
-8.07373826411038));
#43057=CARTESIAN_POINT('Ctrl Pts',(-5.92924452468266,-6.38403842738213,
-8.07368606009921));
#43058=CARTESIAN_POINT('Ctrl Pts',(-5.92334533252883,-6.39660764845899,
-8.07280339665307));
#43059=CARTESIAN_POINT('Ctrl Pts',(-5.91666161280742,-6.41008271491505,
-8.07210940739551));
#43060=CARTESIAN_POINT('Ctrl Pts',(-5.90905330569263,-6.42435950584694,
-8.07173091984199));
#43061=CARTESIAN_POINT('Ctrl Pts',(-5.90809031583021,-6.42616653134261,
-8.07168301435243));
#43062=CARTESIAN_POINT('Ctrl Pts',(-5.90711250287754,-6.4279863444395,-8.07164020169699));
#43063=CARTESIAN_POINT('Ctrl Pts',(-5.90611957366789,-6.42981868289155,
-8.07160277367536));
#43064=CARTESIAN_POINT('Ctrl Pts',(-5.89855598641619,-6.4437764269301,-8.0713176676431));
#43065=CARTESIAN_POINT('Ctrl Pts',(-5.89011476605191,-6.45846421800495,
-8.07134329748215));
#43066=CARTESIAN_POINT('Ctrl Pts',(-5.88068115795978,-6.47375412525542,
-8.07180866003445));
#43067=CARTESIAN_POINT('Ctrl Pts',(-5.8736586626388,-6.48513612258624,-8.07215508171257));
#43068=CARTESIAN_POINT('Ctrl Pts',(-5.86608628545536,-6.49685114602332,
-8.0727455237084));
#43069=CARTESIAN_POINT('Ctrl Pts',(-5.85791981639649,-6.50882979367172,
-8.07364182408336));
#43070=CARTESIAN_POINT('Ctrl Pts',(-5.84746905717488,-6.52415905794388,
-8.07478883380587));
#43071=CARTESIAN_POINT('Ctrl Pts',(-5.83604470384628,-6.53992227767247,
-8.07643553931398));
#43072=CARTESIAN_POINT('Ctrl Pts',(-5.82356408719711,-6.55593067209317,
-8.07873403133492));
#43073=CARTESIAN_POINT('Ctrl Pts',(-5.81185651825911,-6.57094750872356,
-8.08089015507022));
#43074=CARTESIAN_POINT('Ctrl Pts',(-5.79921850083814,-6.5861794471044,-8.08362064648541));
#43075=CARTESIAN_POINT('Ctrl Pts',(-5.78561695045326,-6.60144653247346,
-8.08704934513203));
#43076=CARTESIAN_POINT('Ctrl Pts',(-5.7728923678692,-6.6157292637136,-8.09025697645716));
#43077=CARTESIAN_POINT('Ctrl Pts',(-5.75932437550369,-6.63004293553971,
-8.09407553435004));
#43078=CARTESIAN_POINT('Ctrl Pts',(-5.74490778875738,-6.64420241550599,
-8.09862150095951));
#43079=CARTESIAN_POINT('Ctrl Pts',(-5.74093127011729,-6.64810801653422,
-8.09987541225473));
#43080=CARTESIAN_POINT('Ctrl Pts',(-5.73689033060084,-6.6520016430365,-8.10118476717543));
#43081=CARTESIAN_POINT('Ctrl Pts',(-5.73278520330964,-6.65587882437944,
-8.10255225722823));
#43082=CARTESIAN_POINT('Ctrl Pts',(-5.71725974766235,-6.24680066241192,
-7.76998179414862));
#43083=CARTESIAN_POINT('Ctrl Pts',(-5.7183153287713,-6.59326365452918,-8.03228739331712));
#43084=CARTESIAN_POINT('Ctrl Pts',(-5.7204069205709,-7.31940961941998,-8.65807896524696));
#43085=CARTESIAN_POINT('Ctrl Pts',(-5.72308359607531,-8.29718049086054,
-9.77129138847913));
#43086=CARTESIAN_POINT('Ctrl Pts',(-5.72473137529731,-9.14170426243484,
-11.0927069646456));
#43087=CARTESIAN_POINT('Ctrl Pts',(-5.725483124375,-9.77722228596547,-12.5261362769566));
#43088=CARTESIAN_POINT('Ctrl Pts',(-5.7253232146161,-10.1890896647104,-14.0392346326023));
#43089=CARTESIAN_POINT('Ctrl Pts',(-5.7240590756321,-10.362720345492,-15.5563820479767));
#43090=CARTESIAN_POINT('Ctrl Pts',(-5.72276355651685,-10.3310899414738,
-16.5600585885505));
#43091=CARTESIAN_POINT('Ctrl Pts',(-5.7220426403927,-10.2826264095249,-17.0373217476865));
#43092=CARTESIAN_POINT('Ctrl Pts',(-5.89595647066798,-6.21376083080576,
-7.81369164428259));
#43093=CARTESIAN_POINT('Ctrl Pts',(-5.89686291373834,-6.5580751590849,-8.07499205702994));
#43094=CARTESIAN_POINT('Ctrl Pts',(-5.89864718970208,-7.27968139022067,
-8.69817451202807));
#43095=CARTESIAN_POINT('Ctrl Pts',(-5.90092480081758,-8.25107147177759,
-9.80603802544213));
#43096=CARTESIAN_POINT('Ctrl Pts',(-5.90232044313017,-9.09019307701646,
-11.1204529998163));
#43097=CARTESIAN_POINT('Ctrl Pts',(-5.90295638986529,-9.72175698666846,
-12.5458378515269));
#43098=CARTESIAN_POINT('Ctrl Pts',(-5.90282113710503,-10.1313596816372,
-14.050327350289));
#43099=CARTESIAN_POINT('Ctrl Pts',(-5.90175163079886,-10.3045934944351,
-15.5587586508462));
#43100=CARTESIAN_POINT('Ctrl Pts',(-5.9006514436638,-10.2737520765702,-16.5568830510553));
#43101=CARTESIAN_POINT('Ctrl Pts',(-5.90003850788786,-10.2258942358848,
-17.0315309081517));
#43102=CARTESIAN_POINT('Ctrl Pts',(-6.00511198583713,-6.12219220459409,
-7.93483169827869));
#43103=CARTESIAN_POINT('Ctrl Pts',(-6.00560095016558,-6.46119445239523,
-8.19249553837079));
#43104=CARTESIAN_POINT('Ctrl Pts',(-6.00654860595358,-7.17172454535513,
-8.80693673850609));
#43105=CARTESIAN_POINT('Ctrl Pts',(-6.00775096201441,-8.12793979442155,
-9.89868707557194));
#43106=CARTESIAN_POINT('Ctrl Pts',(-6.00847951651781,-8.95409328932254,
-11.1936989420205));
#43107=CARTESIAN_POINT('Ctrl Pts',(-6.00881050940341,-9.57591183211347,
-12.5976250407049));
#43108=CARTESIAN_POINT('Ctrl Pts',(-6.00874014451152,-9.97942249726841,
-14.079558861051));
#43109=CARTESIAN_POINT('Ctrl Pts',(-6.00818336787537,-10.1504022323851,
-15.5651409909013));
#43110=CARTESIAN_POINT('Ctrl Pts',(-6.00760534674583,-10.1204055268136,
-16.5484230576379));
#43111=CARTESIAN_POINT('Ctrl Pts',(-6.00728240995462,-10.0734760765557,
-17.0159731176358));
#43112=CARTESIAN_POINT('Ctrl Pts',(-5.99984081826169,-6.00940195879855,
-8.08404669773291));
#43113=CARTESIAN_POINT('Ctrl Pts',(-5.99981404919679,-6.34209366151083,
-8.33692329269028));
#43114=CARTESIAN_POINT('Ctrl Pts',(-5.99973665501392,-7.03952549705589,
-8.94005087392584));
#43115=CARTESIAN_POINT('Ctrl Pts',(-5.99962568199747,-7.97795713266765,
-10.0114872699567));
#43116=CARTESIAN_POINT('Ctrl Pts',(-5.99954401869402,-8.78886222453736,
-11.2825987957422));
#43117=CARTESIAN_POINT('Ctrl Pts',(-5.9995051685709,-9.39911593306368,-12.6603955354204));
#43118=CARTESIAN_POINT('Ctrl Pts',(-5.99951348191174,-9.795189453441,-14.1150179548503));
#43119=CARTESIAN_POINT('Ctrl Pts',(-5.99957860547203,-9.96297502994334,
-15.5729285367099));
#43120=CARTESIAN_POINT('Ctrl Pts',(-5.99963682134737,-9.9335331720651,-16.538125769813));
#43121=CARTESIAN_POINT('Ctrl Pts',(-5.99966773997577,-9.88747576114577,
-16.9969875051557));
#43122=CARTESIAN_POINT('',(-5.99999997114735,-9.91329953294255,-16.8993693187113));
#43123=CARTESIAN_POINT('Ctrl Pts',(-6.,-6.09546019522424,-8.13557730902212));
#43124=CARTESIAN_POINT('Ctrl Pts',(-6.,-6.47284397492114,-8.42688307326569));
#43125=CARTESIAN_POINT('Ctrl Pts',(-6.,-6.82542683076759,-8.74185019941709));
#43126=CARTESIAN_POINT('Ctrl Pts',(-6.,-7.1553715768929,-9.08219270129307));
#43127=CARTESIAN_POINT('Ctrl Pts',(-6.,-7.48531632301845,-9.42253520316929));
#43128=CARTESIAN_POINT('Ctrl Pts',(-6.,-7.79262295942282,-9.78825308077012));
#43129=CARTESIAN_POINT('Ctrl Pts',(-6.,-8.07150656549643,-10.1733979628959));
#43130=CARTESIAN_POINT('Ctrl Pts',(-6.,-8.35039017156985,-10.5585428450215));
#43131=CARTESIAN_POINT('Ctrl Pts',(-6.,-8.60085074731254,-10.9631147316719));
#43132=CARTESIAN_POINT('Ctrl Pts',(-6.,-8.82146093334939,-11.3843741331592));
#43133=CARTESIAN_POINT('Ctrl Pts',(-6.,-9.0420711193864,-11.8056335346468));
#43134=CARTESIAN_POINT('Ctrl Pts',(-6.,-9.23283091571751,-12.2435804509713));
#43135=CARTESIAN_POINT('Ctrl Pts',(-6.,-9.39100132287916,-12.6919789565551));
#43136=CARTESIAN_POINT('Ctrl Pts',(-6.,-9.5491717300407,-13.1403774621387));
#43137=CARTESIAN_POINT('Ctrl Pts',(-6.,-9.67475274803281,-13.5992275569817));
#43138=CARTESIAN_POINT('Ctrl Pts',(-6.,-9.76681039167948,-14.0658327420193));
#43139=CARTESIAN_POINT('Ctrl Pts',(-6.,-9.85886803532621,-14.5324379270572));
#43140=CARTESIAN_POINT('Ctrl Pts',(-6.,-9.91740230462745,-15.0067982022898));
#43141=CARTESIAN_POINT('Ctrl Pts',(-6.,-9.94189523605327,-15.4800412501003));
#43142=CARTESIAN_POINT('Ctrl Pts',(-6.,-9.9663881501513,-15.95328396311));
#43143=CARTESIAN_POINT('Ctrl Pts',(-6.,-9.95683977453971,-16.4254094502785));
#43144=CARTESIAN_POINT('Ctrl Pts',(-6.,-9.91329811959712,-16.8993691888704));
#43145=CARTESIAN_POINT('',(-5.736443569433,-10.2877321037677,-16.9337809547651));
#43146=CARTESIAN_POINT('Origin',(-5.5999816381251,-9.91328781245259,-16.8993685785925));
#43147=CARTESIAN_POINT('Ctrl Pts',(-5.732787929952,-6.65588380271171,-8.10254632761798));
#43148=CARTESIAN_POINT('Ctrl Pts',(-5.73461480971849,-7.28539041071228,
-8.63201072144939));
#43149=CARTESIAN_POINT('Ctrl Pts',(-5.73605973940586,-7.85267746104921,
-9.23785131481548));
#43150=CARTESIAN_POINT('Ctrl Pts',(-5.73818934991676,-8.82745379673076,
-10.569912416548));
#43151=CARTESIAN_POINT('Ctrl Pts',(-5.73887403074029,-9.23545520213591,
-11.2957033768654));
#43152=CARTESIAN_POINT('Ctrl Pts',(-5.73948314352351,-9.86673752911049,
-12.8258684638728));
#43153=CARTESIAN_POINT('Ctrl Pts',(-5.7394075754832,-10.0903327788716,-13.630101648187));
#43154=CARTESIAN_POINT('Ctrl Pts',(-5.73849619057915,-10.3386823729398,
-15.2703412948045));
#43155=CARTESIAN_POINT('Ctrl Pts',(-5.73766037378285,-10.3633358173586,
-16.1063565589225));
#43156=CARTESIAN_POINT('Ctrl Pts',(-5.73644356975675,-10.2877321238833,
-16.9337807346159));
#43157=CARTESIAN_POINT('Origin',(-5.599999999997,-9.91330329119812,-16.8993688492357));
#43158=CARTESIAN_POINT('',(-5.593361696257,-10.1144356127388,-17.245059060506));
#43159=CARTESIAN_POINT('Origin',(-5.599999999997,-9.91330329119812,-16.8993688492357));
#43160=CARTESIAN_POINT('Origin',(-5.6,-9.91330329122126,-16.8993688492756));
#43161=CARTESIAN_POINT('Ctrl Pts',(-5.59335880963394,-10.1144382223412,
-17.2450574867612));
#43162=CARTESIAN_POINT('Ctrl Pts',(-5.59335897597996,-10.1110305794363,
-17.2470401530682));
#43163=CARTESIAN_POINT('Ctrl Pts',(-5.59336249921667,-10.0355852078339,
-17.290921844848));
#43164=CARTESIAN_POINT('Ctrl Pts',(-5.59336249921667,-9.95658496883865,
-17.3365326540989));
#43165=CARTESIAN_POINT('Ctrl Pts',(-5.59335897597996,-9.88085962320038,
-17.3799294166115));
#43166=CARTESIAN_POINT('Ctrl Pts',(-5.59335880963394,-9.87743876235887,
-17.3818891887806));
#43167=CARTESIAN_POINT('Ctrl Pts',(-5.8307400439972,-10.1164205431219,-17.2484645412161));
#43168=CARTESIAN_POINT('Ctrl Pts',(-5.83074021197856,-10.1130125214895,
-17.2504473136498));
#43169=CARTESIAN_POINT('Ctrl Pts',(-5.83074376985082,-10.0375588131129,
-17.2943314352281));
#43170=CARTESIAN_POINT('Ctrl Pts',(-5.83074376985082,-9.95855095808477,
-17.3399466416001));
#43171=CARTESIAN_POINT('Ctrl Pts',(-5.83074021197856,-9.88281933979065,
-17.3833494090707));
#43172=CARTESIAN_POINT('Ctrl Pts',(-5.8307400439972,-9.87939819767686,-17.3853094561641));
#43173=CARTESIAN_POINT('Ctrl Pts',(-6.0000034748831,-10.0326983105079,-17.1045694621535));
#43174=CARTESIAN_POINT('Ctrl Pts',(-6.0000035736193,-10.0293041517827,-17.106544087307));
#43175=CARTESIAN_POINT('Ctrl Pts',(-6.00000566486658,-9.95415740055512,
-17.1502479470959));
#43176=CARTESIAN_POINT('Ctrl Pts',(-6.00000566486658,-9.87547170337369,
-17.1956771555441));
#43177=CARTESIAN_POINT('Ctrl Pts',(-6.0000035736193,-9.80004967494144,-17.2389042212266));
#43178=CARTESIAN_POINT('Ctrl Pts',(-6.0000034748831,-9.79664252003289,-17.2408563363306));
#43179=CARTESIAN_POINT('Ctrl Pts',(-5.9999999999769,-9.91330295482212,-16.8993622715432));
#43180=CARTESIAN_POINT('Ctrl Pts',(-5.99999999996752,-9.90992861632663,
-16.9013253647287));
#43181=CARTESIAN_POINT('Ctrl Pts',(-5.99999999976692,-9.83522068214657,
-16.9447739934751));
#43182=CARTESIAN_POINT('Ctrl Pts',(-5.99999999976692,-9.75699439892162,
-16.98993795915));
#43183=CARTESIAN_POINT('Ctrl Pts',(-5.99999999996752,-9.68201281558226,
-17.0329126136425));
#43184=CARTESIAN_POINT('Ctrl Pts',(-5.9999999999769,-9.67862555776588,-17.034853329908));
#43185=CARTESIAN_POINT('Origin',(-5.47627053108701,8.61179369525734,14.9160892206269));
#43186=CARTESIAN_POINT('Ctrl Pts',(-6.00000000001697,-9.91329802718485,
-16.8993701947934));
#43187=CARTESIAN_POINT('Ctrl Pts',(-6.00000000001005,-9.90992616536128,
-16.9013320391245));
#43188=CARTESIAN_POINT('Ctrl Pts',(-6.00000000000346,-9.90655400604935,
-16.9032934158647));
#43189=CARTESIAN_POINT('Ctrl Pts',(-5.9999999999973,-9.90318155035885,-16.905254322156));
#43190=CARTESIAN_POINT('Ctrl Pts',(-5.99999999993207,-9.86751358933604,
-16.9259933727434));
#43191=CARTESIAN_POINT('Ctrl Pts',(-5.99999999990816,-9.83181247294484,
-16.9466797991169));
#43192=CARTESIAN_POINT('Ctrl Pts',(-5.99999999990816,-9.79607949297214,
-16.9673102431511));
#43193=CARTESIAN_POINT('Ctrl Pts',(-5.99999999990816,-9.76034664910772,
-16.9879406086032));
#43194=CARTESIAN_POINT('Ctrl Pts',(-5.99999999993208,-9.72458194169243,
-17.0085149922644));
#43195=CARTESIAN_POINT('Ctrl Pts',(-5.9999999999973,-9.68878892570765,-17.0290339621738));
#43196=CARTESIAN_POINT('Ctrl Pts',(-6.00000000000347,-9.68540449666689,
-17.0309741450765));
#43197=CARTESIAN_POINT('Ctrl Pts',(-6.00000000001005,-9.68201981452002,
-17.0329138325687));
#43198=CARTESIAN_POINT('Ctrl Pts',(-6.00000000001698,-9.67863488229806,
-17.0348530251248));
#43199=CARTESIAN_POINT('Ctrl Pts',(-5.67775659312587,-10.3018870984969,
-17.1369879289495));
#43200=CARTESIAN_POINT('Ctrl Pts',(-3.78517106208391,-11.0756618795401,
-16.643292974773));
#43201=CARTESIAN_POINT('Ctrl Pts',(-2.07379858077616E-10,-11.843298151568,
-16.1396478044549));
#43202=CARTESIAN_POINT('Ctrl Pts',(3.78517106166931,-11.0756618796282,-16.6432929747198));
#43203=CARTESIAN_POINT('Ctrl Pts',(5.67775659250446,-10.3018870987529,-17.1369879287883));
#43204=CARTESIAN_POINT('Ctrl Pts',(-5.67775659312587,-10.1072397989495,
-17.2516485514189));
#43205=CARTESIAN_POINT('Ctrl Pts',(-3.78517106208391,-10.3778358613942,
-17.0589591624347));
#43206=CARTESIAN_POINT('Ctrl Pts',(-2.07379858077616E-10,-10.7266017361378,
-16.9925638790986));
#43207=CARTESIAN_POINT('Ctrl Pts',(3.78517106166931,-10.3778358614304,-17.0589591624264));
#43208=CARTESIAN_POINT('Ctrl Pts',(5.67775659250446,-10.1072397990368,-17.2516485513547));
#43209=CARTESIAN_POINT('Ctrl Pts',(-5.67775659312587,-9.91157799214669,
-17.3647063741836));
#43210=CARTESIAN_POINT('Ctrl Pts',(-3.78517106208391,-9.67397381460403,
-17.4658518041024));
#43211=CARTESIAN_POINT('Ctrl Pts',(-2.07379858077616E-10,-9.51037124759094,
-17.7031909445496));
#43212=CARTESIAN_POINT('Ctrl Pts',(3.78517106166931,-9.67397381458855,-17.4658518041304));
#43213=CARTESIAN_POINT('Ctrl Pts',(5.67775659250446,-9.91157799207137,-17.3647063742117));
#43214=CARTESIAN_POINT('Ctrl Pts',(-5.67775659312587,-9.71502995626686,
-17.4760873358231));
#43215=CARTESIAN_POINT('Ctrl Pts',(-3.78517106208391,-8.96547267303902,
-17.8631643796455));
#43216=CARTESIAN_POINT('Ctrl Pts',(-2.07379858077616E-10,-8.21962531101494,
-18.2570844908793));
#43217=CARTESIAN_POINT('Ctrl Pts',(3.78517106166931,-8.96547267295871,-17.8631643796807));
#43218=CARTESIAN_POINT('Ctrl Pts',(5.67775659250446,-9.71502995601854,-17.4760873359463));
#43219=CARTESIAN_POINT('Ctrl Pts',(-5.59336169625719,-10.1144356127329,
-17.2450590604958));
#43220=CARTESIAN_POINT('Ctrl Pts',(-5.58012472829267,-10.1196353101486,
-17.2417795393872));
#43221=CARTESIAN_POINT('Ctrl Pts',(-5.56080272167237,-10.1272212315458,
-17.236996622306));
#43222=CARTESIAN_POINT('Ctrl Pts',(-5.53535951912591,-10.1371328509956,
-17.2307531058563));
#43223=CARTESIAN_POINT('Ctrl Pts',(-5.51000522085286,-10.1470098370174,
-17.2245314056576));
#43224=CARTESIAN_POINT('Ctrl Pts',(-5.4785722740891,-10.1591964229874,-17.2168593627599));
#43225=CARTESIAN_POINT('Ctrl Pts',(-5.44100421609337,-10.1735931464556,
-17.2078052457423));
#43226=CARTESIAN_POINT('Ctrl Pts',(-5.4135757571343,-10.1841042018537,-17.201194830132));
#43227=CARTESIAN_POINT('Ctrl Pts',(-5.38287654760146,-10.1957925666765,
-17.193848248765));
#43228=CARTESIAN_POINT('Ctrl Pts',(-5.34887846376144,-10.2086053972353,
-17.1858004892764));
#43229=CARTESIAN_POINT('Ctrl Pts',(-5.30328327342022,-10.2257888200095,
-17.1750075537855));
#43230=CARTESIAN_POINT('Ctrl Pts',(-5.25175535625055,-10.2449963320756,
-17.1629524969779));
#43231=CARTESIAN_POINT('Ctrl Pts',(-5.19421238137895,-10.2660648138751,
-17.149741746653));
#43232=CARTESIAN_POINT('Ctrl Pts',(-5.15775456135626,-10.2794132881121,
-17.1413717386931));
#43233=CARTESIAN_POINT('Ctrl Pts',(-5.11888187196832,-10.2935079656825,
-17.132538302818));
#43234=CARTESIAN_POINT('Ctrl Pts',(-5.07757050664895,-10.3082982014974,
-17.1232736070199));
#43235=CARTESIAN_POINT('Ctrl Pts',(-5.01427929152024,-10.3309576316452,
-17.1090795988983));
#43236=CARTESIAN_POINT('Ctrl Pts',(-4.94526457275114,-10.3552518085848,
-17.0938720536587));
#43237=CARTESIAN_POINT('Ctrl Pts',(-4.8704300836545,-10.3809642378146,-17.0777883362319));
#43238=CARTESIAN_POINT('Ctrl Pts',(-4.84061248884309,-10.3912092839911,
-17.0713798235918));
#43239=CARTESIAN_POINT('Ctrl Pts',(-4.80987082608312,-10.4016790077201,
-17.0648324870689));
#43240=CARTESIAN_POINT('Ctrl Pts',(-4.77819856291882,-10.4123577253344,
-17.0581561389736));
#43241=CARTESIAN_POINT('Ctrl Pts',(-4.7010630993418,-10.4383649553613,-17.0418963850475));
#43242=CARTESIAN_POINT('Ctrl Pts',(-4.61840846666524,-10.4656148338015,
-17.0248696191768));
#43243=CARTESIAN_POINT('Ctrl Pts',(-4.53013413338453,-10.4938511480454,
-17.0072368403959));
#43244=CARTESIAN_POINT('Ctrl Pts',(-4.50292955811853,-10.5025530765396,
-17.0018027324319));
#43245=CARTESIAN_POINT('Ctrl Pts',(-4.4751911941991,-10.5113483768928,-16.9963112527045));
#43246=CARTESIAN_POINT('Ctrl Pts',(-4.44691597455289,-10.520228683786,-16.9907676180755));
#43247=CARTESIAN_POINT('Ctrl Pts',(-4.35781070905515,-10.5482136866724,
-16.9732976552732));
#43248=CARTESIAN_POINT('Ctrl Pts',(-4.26337415633484,-10.5770461790196,
-16.9553077638445));
#43249=CARTESIAN_POINT('Ctrl Pts',(-4.16350817952473,-10.6064366031141,
-16.9369792766364));
#43250=CARTESIAN_POINT('Ctrl Pts',(-4.13544195081837,-10.6146964568777,
-16.9318282579386));
#43251=CARTESIAN_POINT('Ctrl Pts',(-4.10694687152408,-10.6230001091607,
-16.9266506566067));
#43252=CARTESIAN_POINT('Ctrl Pts',(-4.07802072640047,-10.6313404886027,
-16.921450882072));
#43253=CARTESIAN_POINT('Ctrl Pts',(-3.98959649917496,-10.6568361640123,
-16.9055557103159));
#43254=CARTESIAN_POINT('Ctrl Pts',(-3.89714408356194,-10.6826770133847,
-16.889452138432));
#43255=CARTESIAN_POINT('Ctrl Pts',(-3.80060148524953,-10.7086443711872,
-16.8732769081817));
#43256=CARTESIAN_POINT('Ctrl Pts',(-3.75616521987444,-10.7205965293285,
-16.8658318338159));
#43257=CARTESIAN_POINT('Ctrl Pts',(-3.71086243888832,-10.7325751201715,
-16.8583718019914));
#43258=CARTESIAN_POINT('Ctrl Pts',(-3.66468717718357,-10.7445568543748,
-16.8509113382743));
#43259=CARTESIAN_POINT('Ctrl Pts',(-3.62904937723011,-10.7538042875428,
-16.845153395521));
#43260=CARTESIAN_POINT('Ctrl Pts',(-3.59289186918105,-10.7630535677352,
-16.8393952106142));
#43261=CARTESIAN_POINT('Ctrl Pts',(-3.5562120702994,-10.7722935290167,-16.8336437594243));
#43262=CARTESIAN_POINT('Ctrl Pts',(-3.51410949029397,-10.782899536164,-16.8270420074723));
#43263=CARTESIAN_POINT('Ctrl Pts',(-3.47131870452021,-10.7934934543348,
-16.8204490092829));
#43264=CARTESIAN_POINT('Ctrl Pts',(-3.42783597889092,-10.8040574386497,
-16.813875902478));
#43265=CARTESIAN_POINT('Ctrl Pts',(-3.40609461607628,-10.8093394308071,
-16.8105893490756));
#43266=CARTESIAN_POINT('Ctrl Pts',(-3.3841802682972,-10.8146139394134,-16.8073077683825));
#43267=CARTESIAN_POINT('Ctrl Pts',(-3.36209246612069,-10.8198786844039,
-16.8040325823261));
#43268=CARTESIAN_POINT('Ctrl Pts',(-3.35104856503244,-10.8225110568992,
-16.8023949892978));
#43269=CARTESIAN_POINT('Ctrl Pts',(-3.33996130034482,-10.825140988483,-16.8007589949167));
#43270=CARTESIAN_POINT('Ctrl Pts',(-3.32883061462407,-10.8277681893696,
-16.7991247798285));
#43271=CARTESIAN_POINT('Ctrl Pts',(-3.3232652717637,-10.8290817898129,-16.7983076722845));
#43272=CARTESIAN_POINT('Ctrl Pts',(-3.31768907364504,-10.8303947075814,
-16.7974910095628));
#43273=CARTESIAN_POINT('Ctrl Pts',(-3.31210201314107,-10.831706906117,-16.7966748144487));
#43274=CARTESIAN_POINT('Ctrl Pts',(-3.30651495263711,-10.8330191046525,
-16.7958586193346));
#43275=CARTESIAN_POINT('Ctrl Pts',(-3.30209405058536,-10.8340555250056,
-16.7952139715887));
#43276=CARTESIAN_POINT('Ctrl Pts',(-3.29530823736295,-10.8356413073638,
-16.7942276547745));
#43277=CARTESIAN_POINT('Ctrl Pts',(-3.26371351550637,-10.8430247042966,
-16.7896353672494));
#43278=CARTESIAN_POINT('Ctrl Pts',(-3.23221976326762,-10.8502790172281,
-16.7851240198793));
#43279=CARTESIAN_POINT('Ctrl Pts',(-3.20082837941875,-10.857405906264,-16.7806925395476));
#43280=CARTESIAN_POINT('Ctrl Pts',(-3.02529692313373,-10.8972573896286,
-16.755912994948));
#43281=CARTESIAN_POINT('Ctrl Pts',(-2.85296934939383,-10.9331235998,-16.7336312409334));
#43282=CARTESIAN_POINT('Ctrl Pts',(-2.68408332988402,-10.9653143544167,
-16.7136486696483));
#43283=CARTESIAN_POINT('Ctrl Pts',(-2.50184473255019,-11.0000501956988,
-16.6920862231373));
#43284=CARTESIAN_POINT('Ctrl Pts',(-2.32361410469579,-11.0305070294388,
-16.6732004871531));
#43285=CARTESIAN_POINT('Ctrl Pts',(-2.14965775603431,-11.0571033277888,
-16.656724449575));
#43286=CARTESIAN_POINT('Ctrl Pts',(-2.13682704056364,-11.059065024153,-16.6555092059126));
#43287=CARTESIAN_POINT('Ctrl Pts',(-2.12401955526259,-11.0610057211373,
-16.6543070705806));
#43288=CARTESIAN_POINT('Ctrl Pts',(-2.11123539610953,-11.0629255879676,
-16.6531179359837));
#43289=CARTESIAN_POINT('Ctrl Pts',(-1.93625472004346,-11.0892033894171,
-16.6368418889479));
#43290=CARTESIAN_POINT('Ctrl Pts',(-1.76564841864985,-11.1115791716701,
-16.6230010120623));
#43291=CARTESIAN_POINT('Ctrl Pts',(-1.59964960282788,-11.1305058856433,
-16.6113061329138));
#43292=CARTESIAN_POINT('Ctrl Pts',(-1.55747658935585,-11.1353143329772,
-16.6083349774063));
#43293=CARTESIAN_POINT('Ctrl Pts',(-1.51560070218881,-11.1399001376491,
-16.6055023611455));
#43294=CARTESIAN_POINT('Ctrl Pts',(-1.47402524336761,-11.1442706692096,
-16.6028036016203));
#43295=CARTESIAN_POINT('Ctrl Pts',(-1.30954622475426,-11.161561175731,-16.59212688678));
#43296=CARTESIAN_POINT('Ctrl Pts',(-1.14977310552627,-11.1754837801492,
-16.5835441025915));
#43297=CARTESIAN_POINT('Ctrl Pts',(-0.994888664990271,-11.1865079150371,
-16.5767563060732));
#43298=CARTESIAN_POINT('Ctrl Pts',(-0.923054601787837,-11.1916208133989,
-16.5736081847873));
#43299=CARTESIAN_POINT('Ctrl Pts',(-0.852271416166483,-11.1961100038712,
-16.5708463593852));
#43300=CARTESIAN_POINT('Ctrl Pts',(-0.782553962123819,-11.2000210008409,
-16.5684420216565));
#43301=CARTESIAN_POINT('Ctrl Pts',(-0.633225991298167,-11.2083979740022,
-16.563292165295));
#43302=CARTESIAN_POINT('Ctrl Pts',(-0.488789985414885,-11.2141242830436,
-16.5597808094322));
#43303=CARTESIAN_POINT('Ctrl Pts',(-0.349367804833761,-11.2176486586726,
-16.5576200264894));
#43304=CARTESIAN_POINT('Ctrl Pts',(-0.262283841740363,-11.21985000566,-16.5562703879939));
#43305=CARTESIAN_POINT('Ctrl Pts',(-0.177155094990459,-11.2211917674833,
-16.5554480857796));
#43306=CARTESIAN_POINT('Ctrl Pts',(-0.0940037411538417,-11.2217777919864,
-16.5550872420774));
#43307=CARTESIAN_POINT('Ctrl Pts',(0.0408033095314012,-11.2227278695407,
-16.5545022332591));
#43308=CARTESIAN_POINT('Ctrl Pts',(0.170411322734702,-11.2216936622582,
-16.5551292702637));
#43309=CARTESIAN_POINT('Ctrl Pts',(0.294749910394146,-11.2191042251408,
-16.5567126569722));
#43310=CARTESIAN_POINT('Ctrl Pts',(0.343180997798596,-11.2180956142363,
-16.5573294014723));
#43311=CARTESIAN_POINT('Ctrl Pts',(0.390812982750298,-11.216850659833,-16.558091441881));
#43312=CARTESIAN_POINT('Ctrl Pts',(0.437643011558179,-11.2153932381847,
-16.5589844415374));
#43313=CARTESIAN_POINT('Ctrl Pts',(0.474088856675121,-11.2142589881103,
-16.5596794256746));
#43314=CARTESIAN_POINT('Ctrl Pts',(0.510048983107251,-11.2129960331579,
-16.5604537385973));
#43315=CARTESIAN_POINT('Ctrl Pts',(0.545522325941037,-11.2116152815913,
-16.5613008068628));
#43316=CARTESIAN_POINT('Ctrl Pts',(0.575342929721347,-11.2104545551952,
-16.5620128933228));
#43317=CARTESIAN_POINT('Ctrl Pts',(0.604819534315609,-11.2092105794191,
-16.5627763970877));
#43318=CARTESIAN_POINT('Ctrl Pts',(0.633951734731624,-11.2078897952418,
-16.5635874263828));
#43319=CARTESIAN_POINT('Ctrl Pts',(0.665845058433713,-11.2064438283492,
-16.564475324292));
#43320=CARTESIAN_POINT('Ctrl Pts',(0.697325520347901,-11.2049058146175,
-16.5654201765311));
#43321=CARTESIAN_POINT('Ctrl Pts',(0.728392804494912,-11.2032839637244,
-16.5664170102246));
#43322=CARTESIAN_POINT('Ctrl Pts',(0.743926446568417,-11.2024730382779,
-16.5669154270713));
#43323=CARTESIAN_POINT('Ctrl Pts',(0.759356794199198,-11.2016411533226,
-16.5674268389585));
#43324=CARTESIAN_POINT('Ctrl Pts',(0.774683802193014,-11.2007893104001,
-16.5679506381934));
#43325=CARTESIAN_POINT('Ctrl Pts',(0.782347306189922,-11.2003633889388,
-16.5682125378109));
#43326=CARTESIAN_POINT('Ctrl Pts',(0.789984975277527,-11.1999324779726,
-16.5684775342458));
#43327=CARTESIAN_POINT('Ctrl Pts',(0.797596805103168,-11.1994967017585,
-16.5687455519958));
#43328=CARTESIAN_POINT('Ctrl Pts',(0.805208634928809,-11.1990609255445,
-16.5690135697459));
#43329=CARTESIAN_POINT('Ctrl Pts',(0.814558096372233,-11.1985163947011,
-16.5693485181722));
#43330=CARTESIAN_POINT('Ctrl Pts',(0.820354772663952,-11.1981749011472,
-16.5695585939035));
#43331=CARTESIAN_POINT('Ctrl Pts',(0.913219558123246,-11.1927040547485,
-16.5729240807328));
#43332=CARTESIAN_POINT('Ctrl Pts',(1.01097505007198,-11.18602334519,-16.5770368529345));
#43333=CARTESIAN_POINT('Ctrl Pts',(1.11356403244014,-11.1778368406865,-16.5820825950803));
#43334=CARTESIAN_POINT('Ctrl Pts',(1.22619397592018,-11.1688490769107,-16.5876221924093));
#43335=CARTESIAN_POINT('Ctrl Pts',(1.3446506836048,-11.1580464090106,-16.5942863065747));
#43336=CARTESIAN_POINT('Ctrl Pts',(1.46882933599734,-11.1450092847503,-16.6023380665375));
#43337=CARTESIAN_POINT('Ctrl Pts',(1.51533012697266,-11.1401273136669,-16.6053531838688));
#43338=CARTESIAN_POINT('Ctrl Pts',(1.56263293993733,-11.1349316887056,-16.6085631034439));
#43339=CARTESIAN_POINT('Ctrl Pts',(1.61073097180307,-11.1293992405122,-16.6119824130128));
#43340=CARTESIAN_POINT('Ctrl Pts',(1.74016071397297,-11.114511659556,-16.621183628504));
#43341=CARTESIAN_POINT('Ctrl Pts',(1.87535186247608,-11.0971867682461,-16.6318998991873));
#43342=CARTESIAN_POINT('Ctrl Pts',(2.0161480133904,-11.076962068608,-16.6444228013579));
#43343=CARTESIAN_POINT('Ctrl Pts',(2.02946096582092,-11.0750497261011,-16.6456069019161));
#43344=CARTESIAN_POINT('Ctrl Pts',(2.04282399839302,-11.0731114398401,-16.6468071672487));
#43345=CARTESIAN_POINT('Ctrl Pts',(2.05623695836665,-11.0711468080309,-16.6480238514605));
#43346=CARTESIAN_POINT('Ctrl Pts',(2.18613474374757,-11.052120335007,-16.659806827398));
#43347=CARTESIAN_POINT('Ctrl Pts',(2.32071794504607,-11.0306238249927,-16.6731290660953));
#43348=CARTESIAN_POINT('Ctrl Pts',(2.45983349748882,-11.0062919740499,-16.6882214249664));
#43349=CARTESIAN_POINT('Ctrl Pts',(2.57754555014244,-10.9857036784276,-16.7009917623652));
#43350=CARTESIAN_POINT('Ctrl Pts',(2.69850206667232,-10.9630849751568,-16.7150297166465));
#43351=CARTESIAN_POINT('Ctrl Pts',(2.82259417732661,-10.9382138516592,-16.7304759714643));
#43352=CARTESIAN_POINT('Ctrl Pts',(2.92928969130115,-10.9168294357546,-16.7437568004233));
#43353=CARTESIAN_POINT('Ctrl Pts',(3.03830297427961,-10.8937797171167,-16.7580788499927));
#43354=CARTESIAN_POINT('Ctrl Pts',(3.14955604559843,-10.8689251872062,-16.7735308186299));
#43355=CARTESIAN_POINT('Ctrl Pts',(3.24644396472019,-10.8472799089659,-16.7869876074613));
#43356=CARTESIAN_POINT('Ctrl Pts',(3.34503044443255,-10.8242657538655,-16.8013013974624));
#43357=CARTESIAN_POINT('Ctrl Pts',(3.4452591362198,-10.7997924913389,-16.8165298503263));
#43358=CARTESIAN_POINT('Ctrl Pts',(3.44870611269044,-10.7989508285517,-16.8170535738007));
#43359=CARTESIAN_POINT('Ctrl Pts',(3.45215503088173,-10.7981074401231,-16.817578379043));
#43360=CARTESIAN_POINT('Ctrl Pts',(3.45560588843955,-10.7972623224504,-16.8181042683679));
#43361=CARTESIAN_POINT('Ctrl Pts',(3.53367151632138,-10.7781439900793,-16.830000986692));
#43362=CARTESIAN_POINT('Ctrl Pts',(3.61272981791193,-10.7581406445687,-16.842452520378));
#43363=CARTESIAN_POINT('Ctrl Pts',(3.6927523583703,-10.7372109243013,-16.8554855073975));
#43364=CARTESIAN_POINT('Ctrl Pts',(3.6994455828851,-10.7354603260826,-16.8565756091078));
#43365=CARTESIAN_POINT('Ctrl Pts',(3.70614555314959,-10.7337032472821,-16.8576697785203));
#43366=CARTESIAN_POINT('Ctrl Pts',(3.71285225154974,-10.7319396639566,-16.8587680310963));
#43367=CARTESIAN_POINT('Ctrl Pts',(3.74623736860275,-10.7231607637824,-16.8642349968991));
#43368=CARTESIAN_POINT('Ctrl Pts',(3.77978920910826,-10.7142206840802,-16.8698031415053));
#43369=CARTESIAN_POINT('Ctrl Pts',(3.8135056146136,-10.7051165161308,-16.8754743575615));
#43370=CARTESIAN_POINT('Ctrl Pts',(3.83375044264756,-10.6996499691556,-16.8788796076788));
#43371=CARTESIAN_POINT('Ctrl Pts',(3.85405460221175,-10.6941242623235,-16.882322018926));
#43372=CARTESIAN_POINT('Ctrl Pts',(3.87441762408892,-10.6885387708392,-16.8858019987448));
#43373=CARTESIAN_POINT('Ctrl Pts',(3.8845991350275,-10.685746025097,-16.8875419886541));
#43374=CARTESIAN_POINT('Ctrl Pts',(3.89479536154432,-10.6829383331958,-16.889291370713));
#43375=CARTESIAN_POINT('Ctrl Pts',(3.9050062438488,-10.6801156172595,-16.8910501957667));
#43376=CARTESIAN_POINT('Ctrl Pts',(3.91011168500104,-10.6787042592913,-16.8919296082936));
#43377=CARTESIAN_POINT('Ctrl Pts',(3.9152207901002,-10.6772891453145,-16.8928113815695));
#43378=CARTESIAN_POINT('Ctrl Pts',(3.92033355162271,-10.6758702656219,-16.8936955219368));
#43379=CARTESIAN_POINT('Ctrl Pts',(3.92544631314522,-10.6744513859293,-16.8945796623041));
#43380=CARTESIAN_POINT('Ctrl Pts',(3.93232800673322,-10.6725369449989,-16.8957726344704));
#43381=CARTESIAN_POINT('Ctrl Pts',(3.93568279791968,-10.6716023196972,-16.896355050652));
#43382=CARTESIAN_POINT('Ctrl Pts',(3.94201776597147,-10.6698374344637,-16.8974548472408));
#43383=CARTESIAN_POINT('Ctrl Pts',(3.94833529222159,-10.6680732144636,-16.8985542612453));
#43384=CARTESIAN_POINT('Ctrl Pts',(3.95463539437183,-10.6663097239537,-16.8996532525245));
#43385=CARTESIAN_POINT('Ctrl Pts',(4.029847930132,-10.6452566378487,-16.9127733446943));
#43386=CARTESIAN_POINT('Ctrl Pts',(4.10257711988876,-10.6243083475567,-16.9258326928244));
#43387=CARTESIAN_POINT('Ctrl Pts',(4.17285368553367,-10.6035689783872,-16.938766316102));
#43388=CARTESIAN_POINT('Ctrl Pts',(4.24078041999403,-10.5835230696334,-16.951267478985));
#43389=CARTESIAN_POINT('Ctrl Pts',(4.30641583381684,-10.5636722621969,-16.9636512381799));
#43390=CARTESIAN_POINT('Ctrl Pts',(4.36978780547811,-10.5441021612752,-16.9758641581216));
#43391=CARTESIAN_POINT('Ctrl Pts',(4.43123718186365,-10.5251257831396,-16.9877065593377));
#43392=CARTESIAN_POINT('Ctrl Pts',(4.49055838833727,-10.5064132731806,-16.9993883734015));
#43393=CARTESIAN_POINT('Ctrl Pts',(4.54777651243732,-10.4880356345445,-17.0108652653892));
#43394=CARTESIAN_POINT('Ctrl Pts',(4.60352991910268,-10.470128442085,-17.0220483622892));
#43395=CARTESIAN_POINT('Ctrl Pts',(4.65728654873519,-10.4525391465315,-17.0330369286175));
#43396=CARTESIAN_POINT('Ctrl Pts',(4.70906899456592,-10.4353274409371,-17.0437936677973));
#43397=CARTESIAN_POINT('Ctrl Pts',(4.75988646526016,-10.4184364785539,-17.0543499532192));
#43398=CARTESIAN_POINT('Ctrl Pts',(4.80880265148368,-10.4019091283525,-17.0646829976357));
#43399=CARTESIAN_POINT('Ctrl Pts',(4.85583810557444,-10.3857965650477,-17.0747607860637));
#43400=CARTESIAN_POINT('Ctrl Pts',(4.90206735032973,-10.3699601784952,-17.0846658365588));
#43401=CARTESIAN_POINT('Ctrl Pts',(4.946479786719,-10.3545244514947,-17.0943243290815));
#43402=CARTESIAN_POINT('Ctrl Pts',(4.98909401540873,-10.3395333433219,-17.103708699377));
#43403=CARTESIAN_POINT('Ctrl Pts',(4.98946319241318,-10.3394034718546,-17.1037899983661));
#43404=CARTESIAN_POINT('Ctrl Pts',(4.98983223445392,-10.3392736337286,-17.1038712767975));
#43405=CARTESIAN_POINT('Ctrl Pts',(4.99020114154273,-10.3391438289709,-17.1039525346539));
#43406=CARTESIAN_POINT('Ctrl Pts',(5.03326624116998,-10.3239908135093,-17.1134383314568));
#43407=CARTESIAN_POINT('Ctrl Pts',(5.07449235854055,-10.3092929024427,-17.1226435416269));
#43408=CARTESIAN_POINT('Ctrl Pts',(5.1138976567057,-10.2950910016694,-17.1315424101203));
#43409=CARTESIAN_POINT('Ctrl Pts',(5.15370169377103,-10.2807453930557,-17.140531325516));
#43410=CARTESIAN_POINT('Ctrl Pts',(5.19164787993578,-10.2669058765484,-17.149207678055));
#43411=CARTESIAN_POINT('Ctrl Pts',(5.22775373278064,-10.2536101379609,-17.1575475826569));
#43412=CARTESIAN_POINT('Ctrl Pts',(5.26453890978093,-10.240064242801,-17.1660444008394));
#43413=CARTESIAN_POINT('Ctrl Pts',(5.29941385717798,-10.2270827796985,-17.1741919971205));
#43414=CARTESIAN_POINT('Ctrl Pts',(5.33239574608239,-10.2147010350817,-17.1819677752936));
#43415=CARTESIAN_POINT('Ctrl Pts',(5.36640991178116,-10.2019317630047,-17.1899869220437));
#43416=CARTESIAN_POINT('Ctrl Pts',(5.39841067752601,-10.1898003462685,-17.19761061042));
#43417=CARTESIAN_POINT('Ctrl Pts',(5.42841530805322,-10.178340594185,-17.2048168552523));
#43418=CARTESIAN_POINT('Ctrl Pts',(5.45996274036015,-10.1662915955219,-17.2123936364703));
#43419=CARTESIAN_POINT('Ctrl Pts',(5.48930350857564,-10.1549851364485,-17.2195089260922));
#43420=CARTESIAN_POINT('Ctrl Pts',(5.51645571937467,-10.1444548599959,-17.2261403666752));
#43421=CARTESIAN_POINT('Ctrl Pts',(5.54440396502199,-10.1336158621991,-17.232966224495));
#43422=CARTESIAN_POINT('Ctrl Pts',(5.57003347968119,-10.1235992310435,-17.2392794342393));
#43423=CARTESIAN_POINT('Ctrl Pts',(5.5933616600179,-10.1144355422305,-17.2450591005858));
#43424=CARTESIAN_POINT('Ctrl Pts',(-5.84637332548169,-10.2457285222001,
-16.9490859041272));
#43425=CARTESIAN_POINT('Ctrl Pts',(-5.81071186277041,-10.2597918225017,
-16.9400659709806));
#43426=CARTESIAN_POINT('Ctrl Pts',(-5.69191724338071,-10.3062068549176,
-16.9103314356046));
#43427=CARTESIAN_POINT('Ctrl Pts',(-5.48049048445379,-10.3862539649999,
-16.8592260848499));
#43428=CARTESIAN_POINT('Ctrl Pts',(-5.20214452272255,-10.4866571133216,
-16.7953170882305));
#43429=CARTESIAN_POINT('Ctrl Pts',(-4.89413796043385,-10.5916763009553,
-16.7286060724361));
#43430=CARTESIAN_POINT('Ctrl Pts',(-4.55276036895968,-10.7006317075456,
-16.6594985240082));
#43431=CARTESIAN_POINT('Ctrl Pts',(-4.17237911330225,-10.8128338020862,
-16.5884198593204));
#43432=CARTESIAN_POINT('Ctrl Pts',(-3.74657608403547,-10.9269277982907,
-16.5162278749803));
#43433=CARTESIAN_POINT('Ctrl Pts',(-3.27004596366195,-11.0401715973013,
-16.4446665253294));
#43434=CARTESIAN_POINT('Ctrl Pts',(-2.73872015992667,-11.1484285626666,
-16.3763657772148));
#43435=CARTESIAN_POINT('Ctrl Pts',(-2.14782149455781,-11.2465594493992,
-16.314586419439));
#43436=CARTESIAN_POINT('Ctrl Pts',(-1.49674277405162,-11.3274272171767,
-16.263833005406));
#43437=CARTESIAN_POINT('Ctrl Pts',(-0.805541188003819,-11.3814775262563,
-16.2300679937111));
#43438=CARTESIAN_POINT('Ctrl Pts',(-0.113422498730109,-11.4024991021397,
-16.2170495617272));
#43439=CARTESIAN_POINT('Ctrl Pts',(0.536119675481227,-11.3923378993577,
-16.2233276646495));
#43440=CARTESIAN_POINT('Ctrl Pts',(1.11982241638366,-11.3587982050083,-16.2442236936773));
#43441=CARTESIAN_POINT('Ctrl Pts',(1.63691910407471,-11.3100218589162,-16.2747549957963));
#43442=CARTESIAN_POINT('Ctrl Pts',(2.09764987884417,-11.2515354414113,-16.3114736122001));
#43443=CARTESIAN_POINT('Ctrl Pts',(2.51229038323631,-11.1867215225181,-16.3522535319986));
#43444=CARTESIAN_POINT('Ctrl Pts',(2.88628054447622,-11.1183510319995,-16.3953417834328));
#43445=CARTESIAN_POINT('Ctrl Pts',(3.2233003370683,-11.0487029073154,-16.4392911535778));
#43446=CARTESIAN_POINT('Ctrl Pts',(3.52771849233986,-10.9792399963371,-16.483168618013));
#43447=CARTESIAN_POINT('Ctrl Pts',(3.80296220772403,-10.9110754271386,-16.5262629591106));
#43448=CARTESIAN_POINT('Ctrl Pts',(4.05167352300846,-10.8451033354659,-16.5680024561924));
#43449=CARTESIAN_POINT('Ctrl Pts',(4.27619687662968,-10.7819779872887,-16.6079681104034));
#43450=CARTESIAN_POINT('Ctrl Pts',(4.47888810571171,-10.7220827433237,-16.6459133079799));
#43451=CARTESIAN_POINT('Ctrl Pts',(4.66210367536694,-10.6655684627837,-16.6817395203754));
#43452=CARTESIAN_POINT('Ctrl Pts',(4.82816201161895,-10.6123989400204,-16.7154675137374));
#43453=CARTESIAN_POINT('Ctrl Pts',(4.97930409772923,-10.5623954933759,-16.7472090922686));
#43454=CARTESIAN_POINT('Ctrl Pts',(5.11759466981168,-10.5152990600229,-16.777127743207));
#43455=CARTESIAN_POINT('Ctrl Pts',(5.2446356860934,-10.4708992468505,-16.8053566586536));
#43456=CARTESIAN_POINT('Ctrl Pts',(5.361519589857,-10.4290877510992,-16.8319645189151));
#43457=CARTESIAN_POINT('Ctrl Pts',(5.46894761068017,-10.389845269209,-16.8569634140839));
#43458=CARTESIAN_POINT('Ctrl Pts',(5.56755786494024,-10.353137310211,-16.8803748902788));
#43459=CARTESIAN_POINT('Ctrl Pts',(5.65799402488361,-10.3188938968047,-16.9022427847047));
#43460=CARTESIAN_POINT('Ctrl Pts',(5.74090216942931,-10.2870141534843,-16.922630231597));
#43461=CARTESIAN_POINT('Ctrl Pts',(5.80283684814847,-10.262865189594,-16.9380975469863));
#43462=CARTESIAN_POINT('Ctrl Pts',(5.83721009878716,-10.2493419733393,-16.9467690913668));
#43463=CARTESIAN_POINT('Ctrl Pts',(5.84634760391269,-10.2457385356534,-16.94908046904));
#43464=CARTESIAN_POINT('Ctrl Pts',(-5.81214087226646,-10.2495588877839,
-17.0923483286303));
#43465=CARTESIAN_POINT('Ctrl Pts',(-5.77669421366777,-10.263585043884,-17.0833806892945));
#43466=CARTESIAN_POINT('Ctrl Pts',(-5.65860674633896,-10.3098810943373,
-17.0538165479733));
#43467=CARTESIAN_POINT('Ctrl Pts',(-5.44839807609833,-10.3897402705518,
-17.002994561743));
#43468=CARTESIAN_POINT('Ctrl Pts',(-5.17161875998938,-10.4899251179542,
-16.9394319559991));
#43469=CARTESIAN_POINT('Ctrl Pts',(-4.86533505594304,-10.5947248316,-16.8730806258442));
#43470=CARTESIAN_POINT('Ctrl Pts',(-4.52587295636493,-10.7034566982716,
-16.8043472696556));
#43471=CARTESIAN_POINT('Ctrl Pts',(-4.14764429910443,-10.815429902991,-16.7336572517321));
#43472=CARTESIAN_POINT('Ctrl Pts',(-3.72427883476413,-10.9292907205645,
-16.6618651175188));
#43473=CARTESIAN_POINT('Ctrl Pts',(-3.2505124902038,-11.0423015126171,-16.5907059004491));
#43474=CARTESIAN_POINT('Ctrl Pts',(-2.72230931494296,-11.1503335008612,
-16.522794637113));
#43475=CARTESIAN_POINT('Ctrl Pts',(-2.13492568104469,-11.2482580101081,
-16.4613723404917));
#43476=CARTESIAN_POINT('Ctrl Pts',(-1.48775542557803,-11.3289535679597,
-16.4109153319803));
#43477=CARTESIAN_POINT('Ctrl Pts',(-0.800722870402349,-11.3828875444853,
-16.3773484312674));
#43478=CARTESIAN_POINT('Ctrl Pts',(-0.112751530280082,-11.4038638339061,
-16.3644057238811));
#43479=CARTESIAN_POINT('Ctrl Pts',(0.532923322872193,-11.393724488833,-16.3706474396948));
#43480=CARTESIAN_POINT('Ctrl Pts',(1.11310674869981,-11.3602570986451,-16.3914210675063));
#43481=CARTESIAN_POINT('Ctrl Pts',(1.62709029934784,-11.3115853094998,-16.421773479825));
#43482=CARTESIAN_POINT('Ctrl Pts',(2.08505695572989,-11.2532232613542,-16.4582779258125));
#43483=CARTESIAN_POINT('Ctrl Pts',(2.49722536832563,-11.1885459997271,-16.4988216357698));
#43484=CARTESIAN_POINT('Ctrl Pts',(2.8690023751527,-11.1203184890061,-16.5416623854398));
#43485=CARTESIAN_POINT('Ctrl Pts',(3.20404389664109,-11.0508149453896,-16.5853615650137));
#43486=CARTESIAN_POINT('Ctrl Pts',(3.50668982747596,-10.9814953247755,-16.6289915145168));
#43487=CARTESIAN_POINT('Ctrl Pts',(3.78034401638953,-10.9134706619404,-16.6718449093925));
#43488=CARTESIAN_POINT('Ctrl Pts',(4.02762985992248,-10.8476334958496,-16.7133529789763));
#43489=CARTESIAN_POINT('Ctrl Pts',(4.25087514568035,-10.7846370103216,-16.7530987152803));
#43490=CARTESIAN_POINT('Ctrl Pts',(4.4524193755322,-10.7248640421826,-16.7908364851191));
#43491=CARTESIAN_POINT('Ctrl Pts',(4.63460310804401,-10.6684653950088,-16.8264679115715));
#43492=CARTESIAN_POINT('Ctrl Pts',(4.7997295023731,-10.615405180405,-16.8600132720348));
#43493=CARTESIAN_POINT('Ctrl Pts',(4.95002508579651,-10.5655053209492,-16.8915834110162));
#43494=CARTESIAN_POINT('Ctrl Pts',(5.08754142422316,-10.5185075294211,-16.9213406010467));
#43495=CARTESIAN_POINT('Ctrl Pts',(5.21387010174365,-10.4742021033152,-16.949416999978));
#43496=CARTESIAN_POINT('Ctrl Pts',(5.33009618342973,-10.4324812281455,-16.9758806130043));
#43497=CARTESIAN_POINT('Ctrl Pts',(5.43691587090918,-10.3933258857094,-17.000743180377));
#43498=CARTESIAN_POINT('Ctrl Pts',(5.53496282001455,-10.3567018589229,-17.0240258852323));
#43499=CARTESIAN_POINT('Ctrl Pts',(5.62487650588722,-10.3225394406628,-17.0457721441461));
#43500=CARTESIAN_POINT('Ctrl Pts',(5.70729921987737,-10.2907379563893,-17.0660446662553));
#43501=CARTESIAN_POINT('Ctrl Pts',(5.76886605571337,-10.2666505418325,-17.0814235370967));
#43502=CARTESIAN_POINT('Ctrl Pts',(5.80303331070594,-10.2531625980629,-17.0900450461037));
#43503=CARTESIAN_POINT('Ctrl Pts',(5.81211594917672,-10.2495686064607,-17.0923430612159));
#43504=CARTESIAN_POINT('Ctrl Pts',(-5.75637734409201,-10.1837214316228,
-17.211851398876));
#43505=CARTESIAN_POINT('Ctrl Pts',(-5.72124284752165,-10.1976641910222,
-17.2029834527919));
#43506=CARTESIAN_POINT('Ctrl Pts',(-5.60419033019956,-10.2436872748253,
-17.1737470798349));
#43507=CARTESIAN_POINT('Ctrl Pts',(-5.39580264084002,-10.3230857151126,
-17.1234851683103));
#43508=CARTESIAN_POINT('Ctrl Pts',(-5.12141647158099,-10.42269850384,-17.0606253549015));
#43509=CARTESIAN_POINT('Ctrl Pts',(-4.81780583424873,-10.5268967653542,
-16.9950167689353));
#43510=CARTESIAN_POINT('Ctrl Pts',(-4.48135309698756,-10.6349959889591,
-16.9270663881488));
#43511=CARTESIAN_POINT('Ctrl Pts',(-4.10654376052558,-10.7463050991349,
-16.8571984811656));
#43512=CARTESIAN_POINT('Ctrl Pts',(-3.68709091827589,-10.8594751597388,
-16.7862604612738));
#43513=CARTESIAN_POINT('Ctrl Pts',(-3.21780670798508,-10.971783037663,-16.7159682018366));
#43514=CARTESIAN_POINT('Ctrl Pts',(-2.69471979108215,-11.0791253962985,
-16.6489041174503));
#43515=CARTESIAN_POINT('Ctrl Pts',(-2.11315352363968,-11.1764086181218,
-16.5882650970455));
#43516=CARTESIAN_POINT('Ctrl Pts',(-1.47251555563333,-11.2565631728444,
-16.5384635825327));
#43517=CARTESIAN_POINT('Ctrl Pts',(-0.792512707503636,-11.3101287606434,
-16.5053381510962));
#43518=CARTESIAN_POINT('Ctrl Pts',(-0.111600877647295,-11.3309605049197,
-16.4925657128992));
#43519=CARTESIAN_POINT('Ctrl Pts',(0.527465568466855,-11.3208910656544,
-16.498725432769));
#43520=CARTESIAN_POINT('Ctrl Pts',(1.10169493934813,-11.2876532359364,-16.5192254848422));
#43521=CARTESIAN_POINT('Ctrl Pts',(1.61044354821197,-11.2393115573349,-16.549180465967));
#43522=CARTESIAN_POINT('Ctrl Pts',(2.06379404302651,-11.1813397325491,-16.5852117077644));
#43523=CARTESIAN_POINT('Ctrl Pts',(2.471861519669,-11.1170880815756,-16.6252363961343));
#43524=CARTESIAN_POINT('Ctrl Pts',(2.83999173167234,-11.0493021153008,-16.6675363377561));
#43525=CARTESIAN_POINT('Ctrl Pts',(3.17179488221991,-10.9802409395444,-16.7106918698678));
#43526=CARTESIAN_POINT('Ctrl Pts',(3.47155832012703,-10.9113554185891,-16.7537869552704));
#43527=CARTESIAN_POINT('Ctrl Pts',(3.74264328254365,-10.8437502095096,-16.796122535093));
#43528=CARTESIAN_POINT('Ctrl Pts',(3.98763901526073,-10.7783131840131,-16.8371359548506));
#43529=CARTESIAN_POINT('Ctrl Pts',(4.20884309009698,-10.7156945421076,-16.8764141939803));
#43530=CARTESIAN_POINT('Ctrl Pts',(4.40856598476383,-10.6562758598002,-16.9137134248617));
#43531=CARTESIAN_POINT('Ctrl Pts',(4.58912056820789,-10.6002080549719,-16.9489353282972));
#43532=CARTESIAN_POINT('Ctrl Pts',(4.75278392451138,-10.5474563849102,-16.9820989261338));
#43533=CARTESIAN_POINT('Ctrl Pts',(4.90175832806563,-10.4978446501649,-17.0133128760172));
#43534=CARTESIAN_POINT('Ctrl Pts',(5.03807359652703,-10.4511168044891,-17.0427368019685));
#43535=CARTESIAN_POINT('Ctrl Pts',(5.16330433230364,-10.4070650240004,-17.0705006587464));
#43536=CARTESIAN_POINT('Ctrl Pts',(5.27852354531286,-10.3655827319811,-17.0966710388853));
#43537=CARTESIAN_POINT('Ctrl Pts',(5.38441915340594,-10.3266515868676,-17.1212589517494));
#43538=CARTESIAN_POINT('Ctrl Pts',(5.48161746197151,-10.2902380611074,-17.1442848117902));
#43539=CARTESIAN_POINT('Ctrl Pts',(5.57075099042334,-10.2562732309174,-17.165791113276));
#43540=CARTESIAN_POINT('Ctrl Pts',(5.65245559249821,-10.2246572217323,-17.1858395574668));
#43541=CARTESIAN_POINT('Ctrl Pts',(5.71348329886499,-10.2007116154242,-17.2010479984918));
#43542=CARTESIAN_POINT('Ctrl Pts',(5.74735040680101,-10.1873035413794,-17.2095738079189));
#43543=CARTESIAN_POINT('Ctrl Pts',(5.75635321170445,-10.183730856004,-17.2118463092144));
#43544=CARTESIAN_POINT('Ctrl Pts',(-5.69417817154424,-10.0659581588309,
-17.2751179674529));
#43545=CARTESIAN_POINT('Ctrl Pts',(-5.65936864914472,-10.0797938193227,
-17.2663701428645));
#43546=CARTESIAN_POINT('Ctrl Pts',(-5.54339858367167,-10.1254637566733,
-17.2375302403083));
#43547=CARTESIAN_POINT('Ctrl Pts',(-5.33694163763027,-10.2042532095778,
-17.1879536089715));
#43548=CARTESIAN_POINT('Ctrl Pts',(-5.06512710375388,-10.3030947989692,
-17.1259628950955));
#43549=CARTESIAN_POINT('Ctrl Pts',(-4.76441598180649,-10.4064721735374,
-17.0612792228816));
#43550=CARTESIAN_POINT('Ctrl Pts',(-4.43125170592017,-10.5137006103613,
-16.9943088394544));
#43551=CARTESIAN_POINT('Ctrl Pts',(-4.0602026902282,-10.6240898693539,-16.9254741696221));
#43552=CARTESIAN_POINT('Ctrl Pts',(-3.64507829848461,-10.7362982384052,
-16.855613542186));
#43553=CARTESIAN_POINT('Ctrl Pts',(-3.18078122530719,-10.8476232159053,
-16.7864186128264));
#43554=CARTESIAN_POINT('Ctrl Pts',(-2.66341923621865,-10.9539976173594,
-16.7204303040473));
#43555=CARTESIAN_POINT('Ctrl Pts',(-2.08839798587963,-11.0503779004316,
-16.6607889637688));
#43556=CARTESIAN_POINT('Ctrl Pts',(-1.45514799384261,-11.1297688198829,
-16.6118247794394));
#43557=CARTESIAN_POINT('Ctrl Pts',(-0.783132822844211,-11.1828134874774,
-16.5792648005158));
#43558=CARTESIAN_POINT('Ctrl Pts',(-0.110281963132231,-11.2034404779047,
-16.5667111358745));
#43559=CARTESIAN_POINT('Ctrl Pts',(0.521223569944504,-11.1934701070349,
-16.5727654222531));
#43560=CARTESIAN_POINT('Ctrl Pts',(1.088675687679,-11.1605570758883,-16.5929146993741));
#43561=CARTESIAN_POINT('Ctrl Pts',(1.59148448878036,-11.112681877478,-16.6223611758767));
#43562=CARTESIAN_POINT('Ctrl Pts',(2.03961626720081,-11.0552607044016,-16.6577881393295));
#43563=CARTESIAN_POINT('Ctrl Pts',(2.4430640223962,-10.9916086294779,-16.6971513458778));
#43564=CARTESIAN_POINT('Ctrl Pts',(2.80710095595344,-10.9244434772457,-16.7387634185779));
#43565=CARTESIAN_POINT('Ctrl Pts',(3.13528225919823,-10.8560029362005,-16.7812288621149));
#43566=CARTESIAN_POINT('Ctrl Pts',(3.4318332440259,-10.7877250356114,-16.8236463772724));
#43567=CARTESIAN_POINT('Ctrl Pts',(3.70006480314895,-10.7207054935996,-16.8653273080683));
#43568=CARTESIAN_POINT('Ctrl Pts',(3.94252576464268,-10.6558257052943,-16.9057166281625));
#43569=CARTESIAN_POINT('Ctrl Pts',(4.16147809567636,-10.5937317915771,-16.9444062223776));
#43570=CARTESIAN_POINT('Ctrl Pts',(4.3591984151706,-10.5348036715704,-16.9811544051073));
#43571=CARTESIAN_POINT('Ctrl Pts',(4.53796761309588,-10.4791925166925,-17.0158628051438));
#43572=CARTESIAN_POINT('Ctrl Pts',(4.7000329475385,-10.4268652489092,-17.0485487613563));
#43573=CARTESIAN_POINT('Ctrl Pts',(4.84756920767978,-10.377648313081,-17.0793181086446));
#43574=CARTESIAN_POINT('Ctrl Pts',(4.98258177189424,-10.3312887637657,-17.1083271049463));
#43575=CARTESIAN_POINT('Ctrl Pts',(5.10662625028276,-10.2875813360151,-17.1357029288908));
#43576=CARTESIAN_POINT('Ctrl Pts',(5.22076218401111,-10.2464211057805,-17.1615104048565));
#43577=CARTESIAN_POINT('Ctrl Pts',(5.32566819367259,-10.2077906165106,-17.1857596279649));
#43578=CARTESIAN_POINT('Ctrl Pts',(5.42196233402055,-10.1716572594301,-17.2084700461599));
#43579=CARTESIAN_POINT('Ctrl Pts',(5.51026929292823,-10.137953195577,-17.2296829791277));
#43580=CARTESIAN_POINT('Ctrl Pts',(5.59121757886941,-10.1065797333569,-17.2494588099646));
#43581=CARTESIAN_POINT('Ctrl Pts',(5.65168088096111,-10.0828178525011,-17.2644609425763));
#43582=CARTESIAN_POINT('Ctrl Pts',(5.68523498109198,-10.0695126493564,-17.2728712786581));
#43583=CARTESIAN_POINT('Ctrl Pts',(5.69415460746513,-10.065967369274,-17.2751130174018));
#43584=CARTESIAN_POINT('',(5.73644274981206,-10.2877306125196,-16.9337807222045));
#43585=CARTESIAN_POINT('Origin',(5.599999999773,-9.91330329131332,-16.8993688489362));
#43586=CARTESIAN_POINT('Ctrl Pts',(-5.73644387793508,-10.2877346863084,
-16.9337810350649));
#43587=CARTESIAN_POINT('Ctrl Pts',(-5.66411038088194,-10.3157397295418,
-16.9158630928389));
#43588=CARTESIAN_POINT('Ctrl Pts',(-5.58548128629471,-10.3456524214079,
-16.8967577754712));
#43589=CARTESIAN_POINT('Ctrl Pts',(-5.50055659255391,-10.3771725884232,
-16.8766547496469));
#43590=CARTESIAN_POINT('Ctrl Pts',(-5.41741953929581,-10.4080292649496,
-16.8569748867591));
#43591=CARTESIAN_POINT('Ctrl Pts',(-5.32824913848286,-10.4404262972982,
-16.8363389758404));
#43592=CARTESIAN_POINT('Ctrl Pts',(-5.23304538859569,-10.4740375140448,
-16.8149530263938));
#43593=CARTESIAN_POINT('Ctrl Pts',(-5.13477098481712,-10.5087328100804,
-16.7928773052841));
#43594=CARTESIAN_POINT('Ctrl Pts',(-5.03006776232682,-10.5447221363093,
-16.7700022193492));
#43595=CARTESIAN_POINT('Ctrl Pts',(-4.91893571945363,-10.5815974269667,
-16.7465854206368));
#43596=CARTESIAN_POINT('Ctrl Pts',(-4.80780367658045,-10.618472717624,-16.7231686219243));
#43597=CARTESIAN_POINT('Ctrl Pts',(-4.69024281332438,-10.6562339759072,
-16.6992101083396));
#43598=CARTESIAN_POINT('Ctrl Pts',(-4.56625312801428,-10.6944230049809,
-16.6749991117564));
#43599=CARTESIAN_POINT('Ctrl Pts',(-4.44622756306065,-10.7313910783988,
-16.651562173952));
#43600=CARTESIAN_POINT('Ctrl Pts',(-4.32017768330217,-10.7687597630938,
-16.6278887933617));
#43601=CARTESIAN_POINT('Ctrl Pts',(-4.18810348873885,-10.8060686256879,
-16.6042695578197));
#43602=CARTESIAN_POINT('Ctrl Pts',(-4.0516176077232,-10.8446237196462,-16.5798613667834));
#43603=CARTESIAN_POINT('Ctrl Pts',(-3.90869822869223,-10.8831151989686,
-16.555510827552));
#43604=CARTESIAN_POINT('Ctrl Pts',(-3.75934535164596,-10.9209854312692,
-16.5315698199977));
#43605=CARTESIAN_POINT('Ctrl Pts',(-3.60999247459969,-10.9588556635699,
-16.5076288124434));
#43606=CARTESIAN_POINT('Ctrl Pts',(-3.4542060995381,-10.9961046535704,-16.4840973331131));
#43607=CARTESIAN_POINT('Ctrl Pts',(-3.29198622646121,-11.0321243882891,
-16.4613590111071));
#43608=CARTESIAN_POINT('Ctrl Pts',(-3.21175020597794,-11.0499402089889,
-16.4501123467151));
#43609=CARTESIAN_POINT('Ctrl Pts',(-3.12994028314089,-11.0674545261354,
-16.4390602110145));
#43610=CARTESIAN_POINT('Ctrl Pts',(-3.04655646263601,-11.084589205439,-16.4282519173722));
#43611=CARTESIAN_POINT('Ctrl Pts',(-3.00486455238357,-11.0931565450908,
-16.4228477705511));
#43612=CARTESIAN_POINT('Ctrl Pts',(-2.96277915898731,-11.1016289310983,
-16.4175045824374));
#43613=CARTESIAN_POINT('Ctrl Pts',(-2.9203002937044,-11.1099963096612,-16.4122287337783));
#43614=CARTESIAN_POINT('Ctrl Pts',(-2.89906086106294,-11.1141799989426,
-16.4095908094488));
#43615=CARTESIAN_POINT('Ctrl Pts',(-2.87772305988289,-11.1183374336123,
-16.4069697198654));
#43616=CARTESIAN_POINT('Ctrl Pts',(-2.85628689001648,-11.122467339776,-16.4043662682671));
#43617=CARTESIAN_POINT('Ctrl Pts',(-2.84556880508328,-11.1245322928579,
-16.403064542468));
#43618=CARTESIAN_POINT('Ctrl Pts',(-2.83482612794603,-11.1265903636395,
-16.4017672261584));
#43619=CARTESIAN_POINT('Ctrl Pts',(-2.82405885859587,-11.1286413917732,
-16.4004744204714));
#43620=CARTESIAN_POINT('Ctrl Pts',(-2.81867522392079,-11.12966690584,-16.3998280176279));
#43621=CARTESIAN_POINT('Ctrl Pts',(-2.81328544119046,-11.1306906592339,
-16.3991827424396));
#43622=CARTESIAN_POINT('Ctrl Pts',(-2.80788951040494,-11.1317126318419,
-16.3985386075961));
#43623=CARTESIAN_POINT('Ctrl Pts',(-2.80249357961942,-11.1327346044499,
-16.3978944727525));
#43624=CARTESIAN_POINT('Ctrl Pts',(-2.79531854980475,-11.1340886500716,
-16.3970410666963));
#43625=CARTESIAN_POINT('Ctrl Pts',(-2.79168327387877,-11.1347731871501,
-16.3966096368024));
#43626=CARTESIAN_POINT('Ctrl Pts',(-2.0459690089911,-11.2751941826081,-16.3081092223224));
#43627=CARTESIAN_POINT('Ctrl Pts',(-1.30026708119672,-11.3593704604482,
-16.255262289602));
#43628=CARTESIAN_POINT('Ctrl Pts',(-0.55454783475753,-11.3872667590075,
-16.2380733656739));
#43629=CARTESIAN_POINT('Ctrl Pts',(-0.369699771189191,-11.3941816626982,
-16.2338125941864));
#43630=CARTESIAN_POINT('Ctrl Pts',(-0.184850643494956,-11.3976383226358,
-16.2317429663731));
#43631=CARTESIAN_POINT('Ctrl Pts',(1.57296398128892E-12,-11.39763584854,
-16.2318648968627));
#43632=CARTESIAN_POINT('Ctrl Pts',(6.95448539688949E-5,-11.3976358476092,
-16.2318649427356));
#43633=CARTESIAN_POINT('Ctrl Pts',(0.000139089706577813,-11.3976358461888,
-16.2318649889188));
#43634=CARTESIAN_POINT('Ctrl Pts',(0.00020863455940168,-11.3976358442788,
-16.2318650354121));
#43635=CARTESIAN_POINT('Ctrl Pts',(0.4655335588341,-11.397623064167,-16.2321761224093));
#43636=CARTESIAN_POINT('Ctrl Pts',(0.930858482086974,-11.3756953217017,
-16.2460734435159));
#43637=CARTESIAN_POINT('Ctrl Pts',(1.39618340431804,-11.3318636296086,-16.2735530557509));
#43638=CARTESIAN_POINT('Ctrl Pts',(1.62884586543357,-11.3099477835621,-16.2872928618684));
#43639=CARTESIAN_POINT('Ctrl Pts',(1.86150832640041,-11.2825561673347,-16.3044279609873));
#43640=CARTESIAN_POINT('Ctrl Pts',(2.09417078585648,-11.2496914820838,-16.3249561696155));
#43641=CARTESIAN_POINT('Ctrl Pts',(2.21050201558451,-11.2332591394584,-16.3352202739296));
#43642=CARTESIAN_POINT('Ctrl Pts',(2.32683324685152,-11.2154585426896,-16.3463326560338));
#43643=CARTESIAN_POINT('Ctrl Pts',(2.44316447733801,-11.1962901146661,-16.3582929162943));
#43644=CARTESIAN_POINT('Ctrl Pts',(2.50133009258126,-11.1867059006543,-16.3642730464246));
#43645=CARTESIAN_POINT('Ctrl Pts',(2.55949570773231,-11.1767797296686,-16.3704651461174));
#43646=CARTESIAN_POINT('Ctrl Pts',(2.61766132280913,-11.1665116597524,-16.3768691619699));
#43647=CARTESIAN_POINT('Ctrl Pts',(2.64674413034754,-11.1613776247943,-16.3800711698961));
#43648=CARTESIAN_POINT('Ctrl Pts',(2.67582693787642,-11.156158115155,-16.3833261568642));
#43649=CARTESIAN_POINT('Ctrl Pts',(2.70490974539752,-11.1508531384236,-16.3866341157703));
#43650=CARTESIAN_POINT('Ctrl Pts',(2.73217487744855,-11.1458797227379,-16.3897353272447));
#43651=CARTESIAN_POINT('Ctrl Pts',(2.75944000949303,-11.1408311894926,-16.3928830960866));
#43652=CARTESIAN_POINT('Ctrl Pts',(2.78670514153725,-11.1357075451166,-16.3960774162571));
#43653=CARTESIAN_POINT('Ctrl Pts',(2.78852281700686,-11.1353659688249,-16.3962903709351));
#43654=CARTESIAN_POINT('Ctrl Pts',(2.7917228120462,-11.1347637864464,-16.3966657965686));
#43655=CARTESIAN_POINT('Ctrl Pts',(2.79215816794584,-11.1346818147619,-16.3967169009717));
#43656=CARTESIAN_POINT('Ctrl Pts',(2.80635173931964,-11.1320093553875,-16.3983830182642));
#43657=CARTESIAN_POINT('Ctrl Pts',(2.82657061154179,-11.128185218442,-16.4007801386854));
#43658=CARTESIAN_POINT('Ctrl Pts',(2.85281478461229,-11.1231354779899,-16.403954948736));
#43659=CARTESIAN_POINT('Ctrl Pts',(2.87905925167368,-11.11808568097,-16.4071297943512));
#43660=CARTESIAN_POINT('Ctrl Pts',(2.91132915457671,-11.1118102528191,-16.4110823469024));
#43661=CARTESIAN_POINT('Ctrl Pts',(2.94962449332137,-11.1041911936577,-16.4158871377949));
#43662=CARTESIAN_POINT('Ctrl Pts',(2.98792028538756,-11.0965720443055,-16.4206919855641));
#43663=CARTESIAN_POINT('Ctrl Pts',(3.03224165594858,-11.0876092319031,-16.4263490916455));
#43664=CARTESIAN_POINT('Ctrl Pts',(3.08258860500442,-11.0771406830763,-16.4329608363572));
#43665=CARTESIAN_POINT('Ctrl Pts',(3.13293654055834,-11.0666719291288,-16.4395727106193));
#43666=CARTESIAN_POINT('Ctrl Pts',(3.18931029073976,-11.0546973795104,-16.4471392605945));
#43667=CARTESIAN_POINT('Ctrl Pts',(3.25170985554867,-11.0410108839757,-16.4557907238688));
#43668=CARTESIAN_POINT('Ctrl Pts',(3.31411012526371,-11.0273242338295,-16.4644422848758));
#43669=CARTESIAN_POINT('Ctrl Pts',(3.38253634575007,-11.0119255987223,-16.4741787833184));
#43670=CARTESIAN_POINT('Ctrl Pts',(3.45698851700775,-10.994564758146,-16.4851583180191));
#43671=CARTESIAN_POINT('Ctrl Pts',(3.53144210666456,-10.9772035868257,-16.4961380618926));
#43672=CARTESIAN_POINT('Ctrl Pts',(3.61192187669741,-10.9578801348977,-16.5083608888898));
#43673=CARTESIAN_POINT('Ctrl Pts',(3.69842782710629,-10.9363001083078,-16.522012771196));
#43674=CARTESIAN_POINT('Ctrl Pts',(3.77372513295017,-10.9175162228689,-16.5338957682904));
#43675=CARTESIAN_POINT('Ctrl Pts',(3.8535881563074,-10.8970219759816,-16.5468619110245));
#43676=CARTESIAN_POINT('Ctrl Pts',(3.93801689717799,-10.8745961180402,-16.5610510335625));
#43677=CARTESIAN_POINT('Ctrl Pts',(3.98561590417564,-10.8619529285519,-16.5690505386601));
#43678=CARTESIAN_POINT('Ctrl Pts',(4.03466610085732,-10.848695329643,-16.577439050651));
#43679=CARTESIAN_POINT('Ctrl Pts',(4.08516749280931,-10.8347801299124,-16.5862438846901));
#43680=CARTESIAN_POINT('Ctrl Pts',(4.1104181887853,-10.8278225300471,-16.5906463017096));
#43681=CARTESIAN_POINT('Ctrl Pts',(4.13603167403025,-10.8207004942125,-16.5951527971566));
#43682=CARTESIAN_POINT('Ctrl Pts',(4.16200796064675,-10.8134083791393,-16.5997669698694));
#43683=CARTESIAN_POINT('Ctrl Pts',(4.174996103955,-10.8097623216026,-16.6020740562258));
#43684=CARTESIAN_POINT('Ctrl Pts',(4.18807494701854,-10.8060737420132,-16.6044080617712));
#43685=CARTESIAN_POINT('Ctrl Pts',(4.20124448968825,-10.8023419207142,-16.6067694410442));
#43686=CARTESIAN_POINT('Ctrl Pts',(4.20782926102311,-10.8004760100647,-16.6079501306807));
#43687=CARTESIAN_POINT('Ctrl Pts',(4.21443670722149,-10.7985992888488,-16.6091376637407));
#43688=CARTESIAN_POINT('Ctrl Pts',(4.22106682828487,-10.7967116661656,-16.6103320976921));
#43689=CARTESIAN_POINT('Ctrl Pts',(4.22769694934825,-10.7948240434824,-16.6115265316436));
#43690=CARTESIAN_POINT('Ctrl Pts',(4.23593845337816,-10.7924710696898,-16.6130154304985));
#43691=CARTESIAN_POINT('Ctrl Pts',(4.24102521599387,-10.7910160022244,-16.613936159866));
#43692=CARTESIAN_POINT('Ctrl Pts',(4.37039631656774,-10.7540094238506,-16.6373529733884));
#43693=CARTESIAN_POINT('Ctrl Pts',(4.49374156102956,-10.717036468039,-16.6607655980989));
#43694=CARTESIAN_POINT('Ctrl Pts',(4.61106095067793,-10.6805477767372,-16.6838896275652));
#43695=CARTESIAN_POINT('Ctrl Pts',(4.72934382251309,-10.6437594230846,-16.7072035624728));
#43696=CARTESIAN_POINT('Ctrl Pts',(4.8415014587966,-10.6074633789056,-16.7302241060399));
#43697=CARTESIAN_POINT('Ctrl Pts',(4.94753386085931,-10.5720761142316,-16.7526883702007));
#43698=CARTESIAN_POINT('Ctrl Pts',(5.05275937819688,-10.536958139348,-16.7749816859414));
#43699=CARTESIAN_POINT('Ctrl Pts',(5.15195253014755,-10.5027351059202,-16.7967271939759));
#43700=CARTESIAN_POINT('Ctrl Pts',(5.24511331801198,-10.4697697435228,-16.8176958739611));
#43701=CARTESIAN_POINT('Ctrl Pts',(5.33934566178715,-10.436425206263,-16.8389057403242));
#43702=CARTESIAN_POINT('Ctrl Pts',(5.42740607222585,-10.4043675230243,-16.8593207521068));
#43703=CARTESIAN_POINT('Ctrl Pts',(5.50929455067416,-10.3739261855197,-16.8787328097754));
#43704=CARTESIAN_POINT('Ctrl Pts',(5.59118302912246,-10.3434848480152,-16.8981448674441));
#43705=CARTESIAN_POINT('Ctrl Pts',(5.66689957558038,-10.3146598542873,-16.9165539721416));
#43706=CARTESIAN_POINT('Ctrl Pts',(5.73644419139399,-10.2877345675643,-16.9337810842183));
#43707=CARTESIAN_POINT('Origin',(5.6,-9.91330329119712,-16.8993688492374));
#43708=CARTESIAN_POINT('Origin',(5.59997427807579,-9.91328074797112,-16.8993778521222));
#43709=CARTESIAN_POINT('Ctrl Pts',(5.71191448556623,-6.68641831441597,-8.11927463999024));
#43710=CARTESIAN_POINT('Ctrl Pts',(5.7168759054207,-6.68389354726089,-8.11895890170305));
#43711=CARTESIAN_POINT('Ctrl Pts',(5.76414643547332,-6.65912533256178,-8.11648535844413));
#43712=CARTESIAN_POINT('Ctrl Pts',(5.84911284240881,-6.60163408410921,-8.12175910200295));
#43713=CARTESIAN_POINT('Ctrl Pts',(5.94753227223416,-6.50077330422613,-8.15338978637534));
#43714=CARTESIAN_POINT('Ctrl Pts',(6.01567270245349,-6.3915836303806,-8.20453568510677));
#43715=CARTESIAN_POINT('Ctrl Pts',(6.047167932251,-6.29514927095438,-8.26241592878045));
#43716=CARTESIAN_POINT('Ctrl Pts',(6.05142447490775,-6.23968542500596,-8.30199013668189));
#43717=CARTESIAN_POINT('Ctrl Pts',(6.05077307745104,-6.21841924779483,-8.3182258932679));
#43718=CARTESIAN_POINT('Ctrl Pts',(5.5958237720461,-6.47865804576311,-7.91172653548768));
#43719=CARTESIAN_POINT('Ctrl Pts',(5.60045279817831,-6.47632066092237,-7.91140915880332));
#43720=CARTESIAN_POINT('Ctrl Pts',(5.64456317555875,-6.45339163238793,-7.9088723405948));
#43721=CARTESIAN_POINT('Ctrl Pts',(5.7239570434588,-6.40018274878796,-7.91317737346647));
#43722=CARTESIAN_POINT('Ctrl Pts',(5.81592621444901,-6.30700766623194,-7.94151439908247));
#43723=CARTESIAN_POINT('Ctrl Pts',(5.87944784527059,-6.20656378539426,-7.9878106170003));
#43724=CARTESIAN_POINT('Ctrl Pts',(5.90863950647487,-6.11851238644606,-8.04024697029675));
#43725=CARTESIAN_POINT('Ctrl Pts',(5.91254319769911,-6.0683720124862,-8.0759627702088));
#43726=CARTESIAN_POINT('Ctrl Pts',(5.91194524499303,-6.04924136375469,-8.09057876431784));
#43727=CARTESIAN_POINT('Ctrl Pts',(5.57866412926808,-6.48058524862489,-7.59641729171106));
#43728=CARTESIAN_POINT('Ctrl Pts',(5.5852468819953,-6.47729943274961,-7.59598815404801));
#43729=CARTESIAN_POINT('Ctrl Pts',(5.64791407954493,-6.44510808730406,-7.59260301057773));
#43730=CARTESIAN_POINT('Ctrl Pts',(5.75974745989275,-6.37116557785623,-7.59922899854909));
#43731=CARTESIAN_POINT('Ctrl Pts',(5.88925329949016,-6.24220063399352,-7.63974090522205));
#43732=CARTESIAN_POINT('Ctrl Pts',(5.9800639380707,-6.10141985758422,-7.70592676409287));
#43733=CARTESIAN_POINT('Ctrl Pts',(6.02330320121339,-5.97417844313933,-7.7824635611915));
#43734=CARTESIAN_POINT('Ctrl Pts',(6.02945845991953,-5.89849949258906,-7.83645796824914));
#43735=CARTESIAN_POINT('Ctrl Pts',(6.02852064698248,-5.86900455921464,-7.85896864395111));
#43736=CARTESIAN_POINT('Ctrl Pts',(5.67168409656827,-6.6909363017478,-7.38004192628035));
#43737=CARTESIAN_POINT('Ctrl Pts',(5.68122596548323,-6.68618796862182,-7.3794641679516));
#43738=CARTESIAN_POINT('Ctrl Pts',(5.77200236259354,-6.63970455067086,-7.37500175316839));
#43739=CARTESIAN_POINT('Ctrl Pts',(5.93302216132211,-6.53360398538186,-7.38571690041905));
#43740=CARTESIAN_POINT('Ctrl Pts',(6.11944510133186,-6.34883503080788,-7.44589119956688));
#43741=CARTESIAN_POINT('Ctrl Pts',(6.25156373113289,-6.14507680730802,-7.54366771878732));
#43742=CARTESIAN_POINT('Ctrl Pts',(6.31599311123261,-5.956762721389,-7.65805067473802));
#43743=CARTESIAN_POINT('Ctrl Pts',(6.32552838135578,-5.84142450668251,-7.74047848722718));
#43744=CARTESIAN_POINT('Ctrl Pts',(6.32408019253049,-5.79585959851974,-7.77522307010303));
#43745=CARTESIAN_POINT('',(5.99998739574857,-6.0954555957118,-8.13557466247078));
#43746=CARTESIAN_POINT('',(5.99999998791472,-6.44014497786806,-7.42970782965953));
#43747=CARTESIAN_POINT('Ctrl Pts',(5.99998739574857,-6.0954555957118,-8.13557466247078));
#43748=CARTESIAN_POINT('Ctrl Pts',(5.9999852507051,-6.09852553841938,-8.11170571829663));
#43749=CARTESIAN_POINT('Ctrl Pts',(5.99998676083024,-6.10206236150406,-8.08798616475802));
#43750=CARTESIAN_POINT('Ctrl Pts',(5.99999979802884,-6.10612978800577,-8.06451310294154));
#43751=CARTESIAN_POINT('Ctrl Pts',(6.00000674447814,-6.10829698456647,-8.05200624170718));
#43752=CARTESIAN_POINT('Ctrl Pts',(6.00001622801463,-6.11061426766856,-8.03956966677541));
#43753=CARTESIAN_POINT('Ctrl Pts',(6.00002591391681,-6.11308675051894,-8.02721971866998));
#43754=CARTESIAN_POINT('Ctrl Pts',(6.00004505311857,-6.11797234064786,-8.00281640094944));
#43755=CARTESIAN_POINT('Ctrl Pts',(6.00006656966194,-6.12346689318343,-7.97875098022345));
#43756=CARTESIAN_POINT('Ctrl Pts',(6.00008775917612,-6.12957143329631,-7.95514338530885));
#43757=CARTESIAN_POINT('Ctrl Pts',(6.00010095494808,-6.13337303622687,-7.94044175335113));
#43758=CARTESIAN_POINT('Ctrl Pts',(6.00011343875003,-6.1374102015521,-7.92591787378617));
#43759=CARTESIAN_POINT('Ctrl Pts',(6.00012222024973,-6.14167330870094,-7.91160086667585));
#43760=CARTESIAN_POINT('Ctrl Pts',(6.000136666637,-6.14868651816037,-7.88804805268568));
#43761=CARTESIAN_POINT('Ctrl Pts',(6.00013998635602,-6.15631378632345,-7.8650561610896));
#43762=CARTESIAN_POINT('Ctrl Pts',(6.00012429255407,-6.16447084918693,-7.84274607149054));
#43763=CARTESIAN_POINT('Ctrl Pts',(6.0001192880969,-6.16707198254142,-7.83563180509723));
#43764=CARTESIAN_POINT('Ctrl Pts',(6.00011246210241,-6.16972662339921,-7.82858674352641));
#43765=CARTESIAN_POINT('Ctrl Pts',(6.00010394449708,-6.17243108075715,-7.8216143988938));
#43766=CARTESIAN_POINT('Ctrl Pts',(6.00009903895563,-6.1739886579333,-7.81759881889872));
#43767=CARTESIAN_POINT('Ctrl Pts',(6.00009357731723,-6.1755627513357,-7.81360735402424));
#43768=CARTESIAN_POINT('Ctrl Pts',(6.0000876760401,-6.1771526374344,-7.80964059033505));
#43769=CARTESIAN_POINT('Ctrl Pts',(6.0000691361879,-6.18214753136233,-7.79717833666742));
#43770=CARTESIAN_POINT('Ctrl Pts',(6.00005142588151,-6.1873620291741,-7.78478770193526));
#43771=CARTESIAN_POINT('Ctrl Pts',(6.00003087539323,-6.19270944962128,-7.77268560910881));
#43772=CARTESIAN_POINT('Ctrl Pts',(6.00001013895765,-6.19810525521661,-7.76047401272637));
#43773=CARTESIAN_POINT('Ctrl Pts',(5.99998605869799,-6.20363625240065,-7.74855670970051));
#43774=CARTESIAN_POINT('Ctrl Pts',(5.9999679811411,-6.20916221676034,-7.73714583029187));
#43775=CARTESIAN_POINT('Ctrl Pts',(5.9999573196392,-6.21242123455163,-7.73041609832358));
#43776=CARTESIAN_POINT('Ctrl Pts',(5.9999490416756,-6.21567752560429,-7.72386226018103));
#43777=CARTESIAN_POINT('Ctrl Pts',(5.99994794613539,-6.21889483549495,-7.7175251660673));
#43778=CARTESIAN_POINT('Ctrl Pts',(5.99994403320275,-6.23038607679768,-7.69489101514807));
#43779=CARTESIAN_POINT('Ctrl Pts',(5.99996394684146,-6.24267989067564,-7.67262426789394));
#43780=CARTESIAN_POINT('Ctrl Pts',(5.99998990573708,-6.25576816623256,-7.65088898742367));
#43781=CARTESIAN_POINT('Ctrl Pts',(6.00001571597285,-6.26878148863728,-7.6292781792552));
#43782=CARTESIAN_POINT('Ctrl Pts',(6.00004678534973,-6.28258014939282,-7.60819371272941));
#43783=CARTESIAN_POINT('Ctrl Pts',(6.00006724493389,-6.29710486864247,-7.58779355113598));
#43784=CARTESIAN_POINT('Ctrl Pts',(6.00007042028293,-6.29935912039344,-7.58462742453473));
#43785=CARTESIAN_POINT('Ctrl Pts',(6.00007335502221,-6.30163076232049,-7.58147775836599));
#43786=CARTESIAN_POINT('Ctrl Pts',(6.00007600935326,-6.30391946558269,-7.57834511352832));
#43787=CARTESIAN_POINT('Ctrl Pts',(6.00009312908458,-6.31868099461108,-7.55814038516948));
#43788=CARTESIAN_POINT('Ctrl Pts',(6.00009752375211,-6.33415600309633,-7.53864552190102));
#43789=CARTESIAN_POINT('Ctrl Pts',(6.00008809825533,-6.35023290373304,-7.51999565200792));
#43790=CARTESIAN_POINT('Ctrl Pts',(6.00007855534302,-6.36651007792217,-7.50111345650805));
#43791=CARTESIAN_POINT('Ctrl Pts',(6.00005445377403,-6.38340350354771,-7.48309820525124));
#43792=CARTESIAN_POINT('Ctrl Pts',(6.00003199274435,-6.40075610903027,-7.46606026200349));
#43793=CARTESIAN_POINT('Ctrl Pts',(6.00001529295041,-6.41365778539459,-7.45339253726803));
#43794=CARTESIAN_POINT('Ctrl Pts',(5.99999988409202,-6.42681233722686,-7.44126443393272));
#43795=CARTESIAN_POINT('Ctrl Pts',(5.99999988835028,-6.44014484659843,-7.4297076782196));
#43796=CARTESIAN_POINT('',(5.72001531319857,-6.64701102057165,-7.39409186140856));
#43797=CARTESIAN_POINT('Ctrl Pts',(5.72001583932162,-6.64701193943656,-7.39409288351738));
#43798=CARTESIAN_POINT('Ctrl Pts',(5.77262443156593,-6.61776628438278,-7.39330399074791));
#43799=CARTESIAN_POINT('Ctrl Pts',(5.82215801012378,-6.58572561272941,-7.39609520796243));
#43800=CARTESIAN_POINT('Ctrl Pts',(5.86878812167724,-6.55120568929977,-7.40209507796886));
#43801=CARTESIAN_POINT('Ctrl Pts',(5.91541823323071,-6.51668576587012,-7.40809494797528));
#43802=CARTESIAN_POINT('Ctrl Pts',(5.95914511084897,-6.47968695772417,-7.41730389800646));
#43803=CARTESIAN_POINT('Ctrl Pts',(6.00000005306065,-6.44014511329477,-7.42970798589524));
#43804=CARTESIAN_POINT('',(5.732785031286,-6.65588656996562,-8.10254649550562));
#43805=CARTESIAN_POINT('Origin',(5.89877289526359,-6.9591999244832,-7.74135689824448));
#43806=CARTESIAN_POINT('Ctrl Pts',(5.73278241139749,-6.65588178673174,-8.1025521928097));
#43807=CARTESIAN_POINT('Ctrl Pts',(5.74767871087474,-6.64180973010437,-8.09758786339362));
#43808=CARTESIAN_POINT('Ctrl Pts',(5.76173626685014,-6.62751756008203,-8.09338492315945));
#43809=CARTESIAN_POINT('Ctrl Pts',(5.77495191999532,-6.61320028672805,-8.08982392122754));
#43810=CARTESIAN_POINT('Ctrl Pts',(5.78903153877291,-6.59794702996169,-8.08603012086695));
#43811=CARTESIAN_POINT('Ctrl Pts',(5.8021557260155,-6.58266504801332,-8.08296512516117));
#43812=CARTESIAN_POINT('Ctrl Pts',(5.81434877348918,-6.56754232129755,-8.08050383231665));
#43813=CARTESIAN_POINT('Ctrl Pts',(5.8170465327943,-6.56419635903469,-8.07995926167602));
#43814=CARTESIAN_POINT('Ctrl Pts',(5.81969880745718,-6.56085802597551,-8.07944430865289));
#43815=CARTESIAN_POINT('Ctrl Pts',(5.82230601940132,-6.557529086438,-8.07895772156423));
#43816=CARTESIAN_POINT('Ctrl Pts',(5.83435660366248,-6.5421426632179,-8.0767087065866));
#43817=CARTESIAN_POINT('Ctrl Pts',(5.84544361982858,-6.52696063865089,-8.07506371238998));
#43818=CARTESIAN_POINT('Ctrl Pts',(5.85563656380534,-6.51215017531834,-8.07388973150728));
#43819=CARTESIAN_POINT('Ctrl Pts',(5.85625536372891,-6.51125105200331,-8.0738184607064));
#43820=CARTESIAN_POINT('Ctrl Pts',(5.85687087189929,-6.51035328450495,-8.07374893287642));
#43821=CARTESIAN_POINT('Ctrl Pts',(5.85748310512795,-6.50945690510748,-8.07368112089833));
#43822=CARTESIAN_POINT('Ctrl Pts',(5.86845369943394,-6.49339470159828,-8.07246599949395));
#43823=CARTESIAN_POINT('Ctrl Pts',(5.87837191641668,-6.47778228369507,-8.07179977148889));
#43824=CARTESIAN_POINT('Ctrl Pts',(5.88734075182149,-6.46277817850691,-8.07154035811203));
#43825=CARTESIAN_POINT('Ctrl Pts',(5.89145115664845,-6.45590181790867,-8.0714214693212));
#43826=CARTESIAN_POINT('Ctrl Pts',(5.89536230645623,-6.44915254784001,-8.07138837201233));
#43827=CARTESIAN_POINT('Ctrl Pts',(5.89908474664214,-6.44254252224732,-8.07142897801076));
#43828=CARTESIAN_POINT('Ctrl Pts',(5.90118652860432,-6.43881033801699,-8.07145190516359));
#43829=CARTESIAN_POINT('Ctrl Pts',(5.90322815576402,-6.43512251272292,-8.07149834565494));
#43830=CARTESIAN_POINT('Ctrl Pts',(5.90521156699562,-6.43148099641133,-8.07156624623327));
#43831=CARTESIAN_POINT('Ctrl Pts',(5.90881698396612,-6.42486149940584,-8.07168967494717));
#43832=CARTESIAN_POINT('Ctrl Pts',(5.91223006400224,-6.41839514362771,-8.07188393007648));
#43833=CARTESIAN_POINT('Ctrl Pts',(5.91546372479684,-6.41209325625483,-8.07213628843071));
#43834=CARTESIAN_POINT('Ctrl Pts',(5.91797000559497,-6.407208916085,-8.07233188127042));
#43835=CARTESIAN_POINT('Ctrl Pts',(5.92036843480492,-6.40242343749142,-8.07256237877867));
#43836=CARTESIAN_POINT('Ctrl Pts',(5.9226649903207,-6.39774121022765,-8.07282239460074));
#43837=CARTESIAN_POINT('Ctrl Pts',(5.92381326807859,-6.39540009659577,-8.07295240251177));
#43838=CARTESIAN_POINT('Ctrl Pts',(5.92493607055781,-6.39308479275801,-8.07308979378538));
#43839=CARTESIAN_POINT('Ctrl Pts',(5.92603412444383,-6.39079580758985,-8.07323393102872));
#43840=CARTESIAN_POINT('Ctrl Pts',(5.92680721312934,-6.38918423956271,-8.07333541135988));
#43841=CARTESIAN_POINT('Ctrl Pts',(5.92725985702953,-6.38823408194907,-8.07339689715456));
#43842=CARTESIAN_POINT('Ctrl Pts',(5.9280443649142,-6.38657648170654,-8.07350892546876));
#43843=CARTESIAN_POINT('Ctrl Pts',(5.92837413013627,-6.38587971508029,-8.07355601618974));
#43844=CARTESIAN_POINT('Ctrl Pts',(5.92876221469405,-6.38505782686567,-8.07361225806707));
#43845=CARTESIAN_POINT('Ctrl Pts',(5.9292547487712,-6.38400829604505,-8.07368595978997));
#43846=CARTESIAN_POINT('Ctrl Pts',(5.93919911343165,-6.36281805218796,-8.07517401278488));
#43847=CARTESIAN_POINT('Ctrl Pts',(5.94793617525635,-6.34198588487123,-8.07733346319839));
#43848=CARTESIAN_POINT('Ctrl Pts',(5.95554257224008,-6.32167919878544,-8.08002789788969));
#43849=CARTESIAN_POINT('Ctrl Pts',(5.95842928866023,-6.31397257444173,-8.08105046729844));
#43850=CARTESIAN_POINT('Ctrl Pts',(5.96115320640223,-6.30634113839236,-8.08215034001233));
#43851=CARTESIAN_POINT('Ctrl Pts',(5.96371874232458,-6.29879233915127,-8.08332088594868));
#43852=CARTESIAN_POINT('Ctrl Pts',(5.97059811501146,-6.27855056320671,-8.08645965382682));
#43853=CARTESIAN_POINT('Ctrl Pts',(5.97633958227157,-6.25890622506058,-8.09010441703621));
#43854=CARTESIAN_POINT('Ctrl Pts',(5.98107332870542,-6.23999045283084,-8.09411401504301));
#43855=CARTESIAN_POINT('Ctrl Pts',(5.98611100847453,-6.21986018087598,-8.09838105195412));
#43856=CARTESIAN_POINT('Ctrl Pts',(5.99000695822762,-6.20055486208303,-8.10306152212758));
#43857=CARTESIAN_POINT('Ctrl Pts',(5.9929112894325,-6.18218287564415,-8.10801549090924));
#43858=CARTESIAN_POINT('Ctrl Pts',(5.99361898202317,-6.17770621035992,-8.10922261459931));
#43859=CARTESIAN_POINT('Ctrl Pts',(5.99426778624819,-6.17328474936486,-8.11044610040774));
#43860=CARTESIAN_POINT('Ctrl Pts',(5.99485986278369,-6.16891966840703,-8.11168415004286));
#43861=CARTESIAN_POINT('Ctrl Pts',(5.99739682055055,-6.15021596141139,-8.1169890041441));
#43862=CARTESIAN_POINT('Ctrl Pts',(5.99889426451141,-6.1325504049427,-8.12255868624874));
#43863=CARTESIAN_POINT('Ctrl Pts',(5.99956526180203,-6.11598503100764,-8.12825285692962));
#43864=CARTESIAN_POINT('Ctrl Pts',(5.99985052305375,-6.10894258930165,-8.1306736211841));
#43865=CARTESIAN_POINT('Ctrl Pts',(5.9999861332358,-6.10209851722248,-8.1331172754017));
#43866=CARTESIAN_POINT('Ctrl Pts',(5.99998739574857,-6.0954555957118,-8.13557466247077));
#43867=CARTESIAN_POINT('Ctrl Pts',(5.99970218884702,-6.00683889572887,-8.08733125571215));
#43868=CARTESIAN_POINT('Ctrl Pts',(5.99970218884702,-6.35108172829139,-8.34755327096762));
#43869=CARTESIAN_POINT('Ctrl Pts',(5.99970218884702,-7.06961527830159,-8.96852445968389));
#43870=CARTESIAN_POINT('Ctrl Pts',(5.99970218884702,-8.03090172607189,-10.0756749999051));
#43871=CARTESIAN_POINT('Ctrl Pts',(5.99970218884702,-8.85234907043669,-11.3899817047342));
#43872=CARTESIAN_POINT('Ctrl Pts',(5.99970218884702,-9.45956831200042,-12.8151106326851));
#43873=CARTESIAN_POINT('Ctrl Pts',(5.99970218884702,-9.8386683762363,-14.3182479126164));
#43874=CARTESIAN_POINT('Ctrl Pts',(5.99970218884702,-9.96649290703559,-15.7255792696104));
#43875=CARTESIAN_POINT('Ctrl Pts',(5.99970218884702,-9.92671360417176,-16.6207571809547));
#43876=CARTESIAN_POINT('Ctrl Pts',(5.99970218884702,-9.88830104579072,-16.997130460064));
#43877=CARTESIAN_POINT('Ctrl Pts',(6.00690077783577,-6.11926434196324,-7.93859628419385));
#43878=CARTESIAN_POINT('Ctrl Pts',(6.00690077783577,-6.47001458246786,-8.20373515941894));
#43879=CARTESIAN_POINT('Ctrl Pts',(6.00690077783577,-7.20199451917009,-8.83632563854109));
#43880=CARTESIAN_POINT('Ctrl Pts',(6.00690077783577,-8.18145565313282,-9.96441656147784));
#43881=CARTESIAN_POINT('Ctrl Pts',(6.00690077783577,-9.01829931826486,-11.3033520080679));
#43882=CARTESIAN_POINT('Ctrl Pts',(6.00690077783577,-9.63699837320393,-12.7554188501705));
#43883=CARTESIAN_POINT('Ctrl Pts',(6.00690077783577,-10.0232003582101,-14.2867394397005));
#43884=CARTESIAN_POINT('Ctrl Pts',(6.00690077783577,-10.1534445291253,-15.7206518840566));
#43885=CARTESIAN_POINT('Ctrl Pts',(6.00690077783577,-10.1129217549952,-16.6325905678065));
#43886=CARTESIAN_POINT('Ctrl Pts',(6.00690077783577,-10.0737824039727,-17.0160648976741));
#43887=CARTESIAN_POINT('Ctrl Pts',(5.89988019332797,-6.21151563398466,-7.81655101996858));
#43888=CARTESIAN_POINT('Ctrl Pts',(5.89988019332797,-6.56760556234862,-8.08572445053743));
#43889=CARTESIAN_POINT('Ctrl Pts',(5.89988019332797,-7.31061900246748,-8.72784919959662));
#43890=CARTESIAN_POINT('Ctrl Pts',(5.89988019332797,-8.30499347090845,-9.87312286385892));
#43891=CARTESIAN_POINT('Ctrl Pts',(5.89988019332797,-9.15447066813245,-11.2322675542128));
#43892=CARTESIAN_POINT('Ctrl Pts',(5.89988019332797,-9.78258954439533,-12.7064384436462));
#43893=CARTESIAN_POINT('Ctrl Pts',(5.89988019332797,-10.174619047903,-14.2608849963055));
#43894=CARTESIAN_POINT('Ctrl Pts',(5.89988019332797,-10.3068486672459,-15.7166086918849));
#43895=CARTESIAN_POINT('Ctrl Pts',(5.89988019332797,-10.265715833855,-16.6423005157086));
#43896=CARTESIAN_POINT('Ctrl Pts',(5.89988019332797,-10.2259801093083,-17.0316016501771));
#43897=CARTESIAN_POINT('Ctrl Pts',(5.72194804881404,-6.24586098767294,-7.77111330658825));
#43898=CARTESIAN_POINT('Ctrl Pts',(5.72194804881404,-6.60393889326845,-8.04178881075682));
#43899=CARTESIAN_POINT('Ctrl Pts',(5.72194804881404,-7.35106013034822,-8.68746318894069));
#43900=CARTESIAN_POINT('Ctrl Pts',(5.72194804881404,-8.35098686517315,-9.83913402461853));
#43901=CARTESIAN_POINT('Ctrl Pts',(5.72194804881404,-9.20516755346836,-11.2058026597302));
#43902=CARTESIAN_POINT('Ctrl Pts',(5.72194804881404,-9.83679344939564,-12.6882029333488));
#43903=CARTESIAN_POINT('Ctrl Pts',(5.72194804881404,-10.2309925505249,-14.2512593316319));
#43904=CARTESIAN_POINT('Ctrl Pts',(5.72194804881404,-10.3639613565709,-15.7151034027759));
#43905=CARTESIAN_POINT('Ctrl Pts',(5.72194804881404,-10.3226013968126,-16.6459155501193));
#43906=CARTESIAN_POINT('Ctrl Pts',(5.72194804881404,-10.2826436411267,-17.0373860164276));
#43907=CARTESIAN_POINT('Ctrl Pts',(5.73278343892927,-6.6558836604587,-8.10254996082558));
#43908=CARTESIAN_POINT('Ctrl Pts',(5.73338951161688,-6.8647510746576,-8.27821818491745));
#43909=CARTESIAN_POINT('Ctrl Pts',(5.73395354695775,-7.06684952503181,-8.46233459868889));
#43910=CARTESIAN_POINT('Ctrl Pts',(5.73447555411707,-7.26144433882555,-8.65430876002968));
#43911=CARTESIAN_POINT('Ctrl Pts',(5.73532470425807,-7.57799213059554,-8.96659353095752));
#43912=CARTESIAN_POINT('Ctrl Pts',(5.73606264101921,-7.87468578917018,-9.29967289629772));
#43913=CARTESIAN_POINT('Ctrl Pts',(5.73668942284259,-8.14888325133039,-9.65097686333643));
#43914=CARTESIAN_POINT('Ctrl Pts',(5.73681690262199,-8.20465167135523,-9.72242780615646));
#43915=CARTESIAN_POINT('Ctrl Pts',(5.73693978433038,-8.25948937240233,-9.79463252356511));
#43916=CARTESIAN_POINT('Ctrl Pts',(5.73705806848171,-8.31337392813761,-9.86756921526368));
#43917=CARTESIAN_POINT('Ctrl Pts',(5.73707478428951,-8.32098884414092,-9.87787656165014));
#43918=CARTESIAN_POINT('Ctrl Pts',(5.7370914082791,-8.32858472468886,-9.88819852625709));
#43919=CARTESIAN_POINT('Ctrl Pts',(5.73710794045192,-8.33616152004608,-9.89853503587695));
#43920=CARTESIAN_POINT('Ctrl Pts',(5.73767502817431,-8.59606127247122,-10.2530986956414));
#43921=CARTESIAN_POINT('Ctrl Pts',(5.73813408881152,-8.8335074050344,-10.6247800471307));
#43922=CARTESIAN_POINT('Ctrl Pts',(5.73848518367663,-9.04647680356154,-11.0106030415808));
#43923=CARTESIAN_POINT('Ctrl Pts',(5.73855071710724,-9.08622849658298,-11.0826186332201));
#43924=CARTESIAN_POINT('Ctrl Pts',(5.7386124889711,-9.12512733602101,-11.1551268007166));
#43925=CARTESIAN_POINT('Ctrl Pts',(5.73867049958713,-9.16316004565204,-11.228108028484));
#43926=CARTESIAN_POINT('Ctrl Pts',(5.73897977938334,-9.36592894363117,-11.6172026596877));
#43927=CARTESIAN_POINT('Ctrl Pts',(5.7391821511709,-9.54408075696241,-12.0197473164057));
#43928=CARTESIAN_POINT('Ctrl Pts',(5.73927764632406,-9.69602494696988,-12.4324947986501));
#43929=CARTESIAN_POINT('Ctrl Pts',(5.73929840882887,-9.72906057097882,-12.5222341340823));
#43930=CARTESIAN_POINT('Ctrl Pts',(5.73931411902672,-9.76085723580346,-12.6124555976131));
#43931=CARTESIAN_POINT('Ctrl Pts',(5.73932477703702,-9.79139843860385,-12.7031255267129));
#43932=CARTESIAN_POINT('Ctrl Pts',(5.7393735862753,-9.9312643988762,-13.1183559544157));
#43933=CARTESIAN_POINT('Ctrl Pts',(5.73931644079582,-10.0448015289714,-13.5429957199903));
#43934=CARTESIAN_POINT('Ctrl Pts',(5.73915333152432,-10.1308662049193,-13.9736567908168));
#43935=CARTESIAN_POINT('Ctrl Pts',(5.7391174741561,-10.1497863603912,-14.0683318049964));
#43936=CARTESIAN_POINT('Ctrl Pts',(5.73907649563359,-10.1673787538509,-14.1632976307152));
#43937=CARTESIAN_POINT('Ctrl Pts',(5.73903039564908,-10.1836311146258,-14.2585179559314));
#43938=CARTESIAN_POINT('Ctrl Pts',(5.73900084443474,-10.194049274242,-14.31955650661));
#43939=CARTESIAN_POINT('Ctrl Pts',(5.73896918874735,-10.2039167967521,-14.3806996319841));
#43940=CARTESIAN_POINT('Ctrl Pts',(5.73893542849059,-10.2132325779621,-14.4419375696272));
#43941=CARTESIAN_POINT('Ctrl Pts',(5.73869640194468,-10.2791893928211,-14.8755092931832));
#43942=CARTESIAN_POINT('Ctrl Pts',(5.73835187087254,-10.3174891438493,-15.3138381747238));
#43943=CARTESIAN_POINT('Ctrl Pts',(5.73790179978098,-10.3277354971762,-15.7534299763543));
#43944=CARTESIAN_POINT('Ctrl Pts',(5.73786596841969,-10.3285512367224,-15.7884270533972));
#43945=CARTESIAN_POINT('Ctrl Pts',(5.73782946811548,-10.3291891649064,-15.8234321079199));
#43946=CARTESIAN_POINT('Ctrl Pts',(5.73779229884493,-10.3296490796853,-15.8584433625832));
#43947=CARTESIAN_POINT('Ctrl Pts',(5.73741169570001,-10.33435848099,-16.2169490161895));
#43948=CARTESIAN_POINT('Ctrl Pts',(5.73696095042926,-10.3204029417981,-16.576106838384));
#43949=CARTESIAN_POINT('Ctrl Pts',(5.73644003522184,-10.287721746545,-16.9337799081518));
#43950=CARTESIAN_POINT('Ctrl Pts',(5.9999999993059,-6.09545559723548,-8.1355746616996));
#43951=CARTESIAN_POINT('Ctrl Pts',(5.9999999993156,-6.21632000246365,-8.22886961536299));
#43952=CARTESIAN_POINT('Ctrl Pts',(5.99999999835916,-6.33462436300169,-8.3246240217504));
#43953=CARTESIAN_POINT('Ctrl Pts',(5.99999999609535,-6.45047432846417,-8.42285685600839));
#43954=CARTESIAN_POINT('Ctrl Pts',(5.99999999382032,-6.56689816955468,-8.52157629748484));
#43955=CARTESIAN_POINT('Ctrl Pts',(5.9999999902401,-6.68084357504832,-8.62279909937612));
#43956=CARTESIAN_POINT('Ctrl Pts',(5.99999999039156,-6.79238504196438,-8.7265856228609));
#43957=CARTESIAN_POINT('Ctrl Pts',(5.99999999048548,-6.86154926350248,-8.79094118766957));
#43958=CARTESIAN_POINT('Ctrl Pts',(5.99999999231393,-6.92978852009233,-8.85628328040707));
#43959=CARTESIAN_POINT('Ctrl Pts',(5.99999999505289,-6.99711341831894,-8.9226333709323));
#43960=CARTESIAN_POINT('Ctrl Pts',(5.9999999972169,-7.05030583281631,-8.97505560416431));
#43961=CARTESIAN_POINT('Ctrl Pts',(5.99999999999962,-7.10292736651186,-9.02810717281959));
#43962=CARTESIAN_POINT('Ctrl Pts',(5.99999999999962,-7.15498473399384,-9.08180207094362));
#43963=CARTESIAN_POINT('Ctrl Pts',(5.99999999999962,-7.28285593185063,-9.2136956198115));
#43964=CARTESIAN_POINT('Ctrl Pts',(5.99999998462023,-7.40736537484194,-9.34940593933384));
#43965=CARTESIAN_POINT('Ctrl Pts',(5.99999998025195,-7.52813264110009,-9.48859830995591));
#43966=CARTESIAN_POINT('Ctrl Pts',(5.99999997588669,-7.64881610288076,-9.62769409029944));
#43967=CARTESIAN_POINT('Ctrl Pts',(5.99999998175304,-7.76576225718329,-9.77026676590069));
#43968=CARTESIAN_POINT('Ctrl Pts',(5.99999999007195,-7.87862812274216,-9.91594547377447));
#43969=CARTESIAN_POINT('Ctrl Pts',(5.99999999337621,-7.92345823073153,-9.9738087805714));
#43970=CARTESIAN_POINT('Ctrl Pts',(5.99999999675166,-7.96764503899738,-10.0321617334311));
#43971=CARTESIAN_POINT('Ctrl Pts',(5.99999999861007,-8.01116883173431,-10.0909796561054));
#43972=CARTESIAN_POINT('Ctrl Pts',(5.99999999947163,-8.03134643779373,-10.1182476122812));
#43973=CARTESIAN_POINT('Ctrl Pts',(5.99999999999962,-8.05138156043679,-10.1456154909224));
#43974=CARTESIAN_POINT('Ctrl Pts',(5.99999999999962,-8.07127252639277,-10.1730804652344));
#43975=CARTESIAN_POINT('Ctrl Pts',(5.99999999999962,-8.19608224407421,-10.3454147650165));
#43976=CARTESIAN_POINT('Ctrl Pts',(5.99999998564321,-8.31516617400978,-10.5216179734177));
#43977=CARTESIAN_POINT('Ctrl Pts',(5.99999998504708,-8.42843403911075,-10.7014457915073));
#43978=CARTESIAN_POINT('Ctrl Pts',(5.99999998445023,-8.54183900473007,-10.8814912749255));
#43979=CARTESIAN_POINT('Ctrl Pts',(5.99999999412996,-8.64941414963471,-11.0651706214989));
#43980=CARTESIAN_POINT('Ctrl Pts',(5.9999999983805,-8.7510270922678,-11.2522696464205));
#43981=CARTESIAN_POINT('Ctrl Pts',(5.99999999937175,-8.77472398227683,-11.295902523291));
#43982=CARTESIAN_POINT('Ctrl Pts',(5.99999999999963,-8.79809642264477,-11.3397214970844));
#43983=CARTESIAN_POINT('Ctrl Pts',(5.99999999999963,-8.82114237775435,-11.3837240507049));
#43984=CARTESIAN_POINT('Ctrl Pts',(5.99999999999963,-8.82427077957775,-11.3896972320431));
#43985=CARTESIAN_POINT('Ctrl Pts',(5.99999999998808,-8.82739320263783,-11.3956737752782));
#43986=CARTESIAN_POINT('Ctrl Pts',(5.99999999996603,-8.83050963567541,-11.4016536636707));
#43987=CARTESIAN_POINT('Ctrl Pts',(5.99999999925238,-8.93137509851493,-11.5951967955668));
#43988=CARTESIAN_POINT('Ctrl Pts',(5.99999999047918,-9.0259620484505,-11.7922463184232));
#43989=CARTESIAN_POINT('Ctrl Pts',(5.99999999007257,-9.11398098223997,-11.9922073236602));
#43990=CARTESIAN_POINT('Ctrl Pts',(5.9999999896657,-9.20205429336523,-12.1922918630763));
#43991=CARTESIAN_POINT('Ctrl Pts',(5.99999999693156,-9.28355123916782,-12.395290972675));
#43992=CARTESIAN_POINT('Ctrl Pts',(5.99999999941396,-9.35822889393878,-12.6005865753142));
#43993=CARTESIAN_POINT('Ctrl Pts',(5.99999999977838,-9.36919170568964,-12.6307243327453));
#43994=CARTESIAN_POINT('Ctrl Pts',(5.99999999999963,-9.38000764283712,-12.6609115505662));
#43995=CARTESIAN_POINT('Ctrl Pts',(5.99999999999963,-9.3906760268368,-12.6911462437714));
#43996=CARTESIAN_POINT('Ctrl Pts',(5.99999999999963,-9.40612090546474,-12.7349177434587));
#43997=CARTESIAN_POINT('Ctrl Pts',(5.99999999953036,-9.42125510905206,-12.7787890010936));
#43998=CARTESIAN_POINT('Ctrl Pts',(5.99999999872729,-9.43607771846652,-12.82275774804));
#43999=CARTESIAN_POINT('Ctrl Pts',(5.99999999501562,-9.50458504372292,-13.0259730635049));
#44000=CARTESIAN_POINT('Ctrl Pts',(5.99999998445147,-9.56644039632124,-13.2312698568886));
#44001=CARTESIAN_POINT('Ctrl Pts',(5.99999998419192,-9.62157188140313,-13.4383965501976));
#44002=CARTESIAN_POINT('Ctrl Pts',(5.99999998393238,-9.67670336648502,-13.6455232435065));
#44003=CARTESIAN_POINT('Ctrl Pts',(5.99999999999963,-9.72511108983177,-13.8544804123467));
#44004=CARTESIAN_POINT('Ctrl Pts',(5.99999999999962,-9.76667145420375,-14.0650241450564));
#44005=CARTESIAN_POINT('Ctrl Pts',(5.99999999999962,-9.7835072985383,-14.1503140977091));
#44006=CARTESIAN_POINT('Ctrl Pts',(5.99999999597128,-9.79923294555681,-14.2358640307631));
#44007=CARTESIAN_POINT('Ctrl Pts',(5.99999999157414,-9.81383348710217,-14.3216199001221));
#44008=CARTESIAN_POINT('Ctrl Pts',(5.99999998233605,-9.84450828541726,-14.5017874636846));
#44009=CARTESIAN_POINT('Ctrl Pts',(5.99999997355903,-9.87021359544724,-14.6828643853021));
#44010=CARTESIAN_POINT('Ctrl Pts',(5.99999997660565,-9.89091099303221,-14.8643517495919));
#44011=CARTESIAN_POINT('Ctrl Pts',(5.99999997965609,-9.91163423873525,-15.0460657658943));
#44012=CARTESIAN_POINT('Ctrl Pts',(5.99999999487371,-9.92733703853263,-15.2281907937088));
#44013=CARTESIAN_POINT('Ctrl Pts',(5.9999999991423,-9.9380328969175,-15.4102231927563));
#44014=CARTESIAN_POINT('Ctrl Pts',(5.99999999968359,-9.93938920244837,-15.4333061039863));
#44015=CARTESIAN_POINT('Ctrl Pts',(5.99999999999963,-9.94066506549936,-15.4563875273483));
#44016=CARTESIAN_POINT('Ctrl Pts',(5.99999999999963,-9.94186057345894,-15.4794664384282));
#44017=CARTESIAN_POINT('Ctrl Pts',(5.99999999999963,-9.94849006795469,-15.6074467774512));
#44018=CARTESIAN_POINT('Ctrl Pts',(5.99999999306092,-9.95260895372041,-15.7353412105235));
#44019=CARTESIAN_POINT('Ctrl Pts',(5.99999999145036,-9.9542448330683,-15.8632214087634));
#44020=CARTESIAN_POINT('Ctrl Pts',(5.99999998952808,-9.95619734135282,-16.0158531702759));
#44021=CARTESIAN_POINT('Ctrl Pts',(5.99999999274889,-9.95461394974177,-16.1684648502107));
#44022=CARTESIAN_POINT('Ctrl Pts',(5.99999999547939,-9.94950717517158,-16.3211506606758));
#44023=CARTESIAN_POINT('Ctrl Pts',(5.99999999819765,-9.94442331957945,-16.4731512239872));
#44024=CARTESIAN_POINT('Ctrl Pts',(5.99999999961507,-9.93584763338568,-16.6252257133007));
#44025=CARTESIAN_POINT('Ctrl Pts',(5.99999999985074,-9.92374096699956,-16.7774656808718));
#44026=CARTESIAN_POINT('Ctrl Pts',(5.99999999991362,-9.92051052208515,-16.8180881621829));
#44027=CARTESIAN_POINT('Ctrl Pts',(5.99999999993317,-9.91702838885872,-16.8587223964478));
#44028=CARTESIAN_POINT('Ctrl Pts',(5.99999999993286,-9.91329319860811,-16.8993700414499));
#44029=CARTESIAN_POINT('Ctrl Pts',(-5.843530343916,-6.4054425445004,-7.94861181432332));
#44030=CARTESIAN_POINT('Ctrl Pts',(-3.895686895944,-7.50111660415432,-7.93455833697476));
#44031=CARTESIAN_POINT('Ctrl Pts',(0.0001666015266142,-8.59741061726458,
-7.91991847694548));
#44032=CARTESIAN_POINT('Ctrl Pts',(3.896020098997,-7.50102283673824,-7.93455958914352));
#44033=CARTESIAN_POINT('Ctrl Pts',(5.844030148496,-6.4051613892978,-7.94861542050703));
#44034=CARTESIAN_POINT('Ctrl Pts',(-5.843530343916,-7.02207566989846,-8.43809511982169));
#44035=CARTESIAN_POINT('Ctrl Pts',(-3.895686895944,-8.0413509136543,-8.43217728733141));
#44036=CARTESIAN_POINT('Ctrl Pts',(0.0001666015266142,-9.06227941450043,
-8.42460895688274));
#44037=CARTESIAN_POINT('Ctrl Pts',(3.896020098997,-8.04126359234196,-8.43217793466096));
#44038=CARTESIAN_POINT('Ctrl Pts',(5.844030148496,-7.02181411900168,-8.43809663834368));
#44039=CARTESIAN_POINT('Ctrl Pts',(-5.843530343916,-8.22106584996092,-9.63752182400419));
#44040=CARTESIAN_POINT('Ctrl Pts',(-3.895686895944,-9.09188988950535,-9.61305631917377));
#44041=CARTESIAN_POINT('Ctrl Pts',(0.0001666015266142,-9.96180820070112,
-9.58947287128109));
#44042=CARTESIAN_POINT('Ctrl Pts',(3.896020098997,-9.09181548429369,-9.61305833630071));
#44043=CARTESIAN_POINT('Ctrl Pts',(5.844030148496,-8.22084239233718,-9.63752810198184));
#44044=CARTESIAN_POINT('Ctrl Pts',(-5.843530343916,-9.55783038259166,-11.8732201358514));
#44045=CARTESIAN_POINT('Ctrl Pts',(-3.895686895944,-10.2763900681484,-11.732826252669));
#44046=CARTESIAN_POINT('Ctrl Pts',(0.0001666015266142,-10.9955725683266,
-11.5921560888784));
#44047=CARTESIAN_POINT('Ctrl Pts',(3.896020098997,-10.2763285555545,-11.7328382843669));
#44048=CARTESIAN_POINT('Ctrl Pts',(5.844030148496,-9.55764599674235,-11.8732561615906));
#44049=CARTESIAN_POINT('Ctrl Pts',(-5.843530343916,-10.2973084082931,-14.4766646359851));
#44050=CARTESIAN_POINT('Ctrl Pts',(-3.895686895944,-10.9728038426106,-14.1582376099169));
#44051=CARTESIAN_POINT('Ctrl Pts',(0.0001666015266142,-11.6469750229257,
-13.8399443711029));
#44052=CARTESIAN_POINT('Ctrl Pts',(3.896020098997,-10.972746179898,-14.1582648339447));
#44053=CARTESIAN_POINT('Ctrl Pts',(5.844030148496,-10.2971350729153,-14.4767463458862));
#44054=CARTESIAN_POINT('Ctrl Pts',(-5.843530343916,-10.3258757623353,-16.2770693533102));
#44055=CARTESIAN_POINT('Ctrl Pts',(-3.895686895944,-11.0553896713365,-15.8346874642404));
#44056=CARTESIAN_POINT('Ctrl Pts',(0.0001666015266142,-11.7876699880132,
-15.3921227748421));
#44057=CARTESIAN_POINT('Ctrl Pts',(3.896020098997,-11.0553270384729,-15.8347253173623));
#44058=CARTESIAN_POINT('Ctrl Pts',(5.844030148496,-10.3256885656043,-16.2771828706193));
#44059=CARTESIAN_POINT('Ctrl Pts',(-5.843530343916,-10.225161154803,-17.1593148751532));
#44060=CARTESIAN_POINT('Ctrl Pts',(-3.895686895944,-11.003363098979,-16.6619434543588));
#44061=CARTESIAN_POINT('Ctrl Pts',(0.0001666015266142,-11.7816843621865,
-16.1645455971594));
#44062=CARTESIAN_POINT('Ctrl Pts',(3.896020098997,-11.0032965281671,-16.6619859974273));
#44063=CARTESIAN_POINT('Ctrl Pts',(5.844030148496,-10.2249614644564,-17.1594425030394));
#44064=CARTESIAN_POINT('Ctrl Pts',(-5.73278975501823,-6.65588713914762,
-8.10254235490726));
#44065=CARTESIAN_POINT('Ctrl Pts',(-5.37897179112506,-6.85202415254095,
-8.10465391657496));
#44066=CARTESIAN_POINT('Ctrl Pts',(-5.01613184499411,-7.0312284216845,-8.10373386681346));
#44067=CARTESIAN_POINT('Ctrl Pts',(-4.64588304903464,-7.19219343306865,
-8.10100473255839));
#44068=CARTESIAN_POINT('Ctrl Pts',(-4.37154851834488,-7.31145988670049,
-8.09898259022268));
#44069=CARTESIAN_POINT('Ctrl Pts',(-4.09314651694435,-7.42070943831706,
-8.09596903559524));
#44070=CARTESIAN_POINT('Ctrl Pts',(-3.81133323615115,-7.51943452553296,
-8.09247487047289));
#44071=CARTESIAN_POINT('Ctrl Pts',(-3.57225617964817,-7.6031882194261,-8.08951058607141));
#44072=CARTESIAN_POINT('Ctrl Pts',(-3.33072401753176,-7.67936667759463,
-8.0862006579435));
#44073=CARTESIAN_POINT('Ctrl Pts',(-3.08713739488102,-7.74770051014093,
-8.08285930770894));
#44074=CARTESIAN_POINT('Ctrl Pts',(-3.0435950629987,-7.7599155258226,-8.08226202457711));
#44075=CARTESIAN_POINT('Ctrl Pts',(-2.99998708420428,-7.77188001335109,
-8.08166373982413));
#44076=CARTESIAN_POINT('Ctrl Pts',(-2.95631574691158,-7.78359262272358,
-8.0810662505597));
#44077=CARTESIAN_POINT('Ctrl Pts',(-2.75788908834141,-7.83681045586082,
-8.07835147685176));
#44078=CARTESIAN_POINT('Ctrl Pts',(-2.55814961936489,-7.88487194894928,
-8.07569834222977));
#44079=CARTESIAN_POINT('Ctrl Pts',(-2.35736414035255,-7.92758001824303,
-8.07319712986884));
#44080=CARTESIAN_POINT('Ctrl Pts',(-2.16341814364899,-7.96883329565734,
-8.07078111788085));
#44081=CARTESIAN_POINT('Ctrl Pts',(-1.96849618498995,-8.00509159254689,
-8.06850686502789));
#44082=CARTESIAN_POINT('Ctrl Pts',(-1.7728387183633,-8.03622543206867,-8.06645526106578));
#44083=CARTESIAN_POINT('Ctrl Pts',(-1.58027048296615,-8.06686770011606,
-8.06443604983132));
#44084=CARTESIAN_POINT('Ctrl Pts',(-1.38698978208197,-8.09254589079393,
-8.06263252184692));
#44085=CARTESIAN_POINT('Ctrl Pts',(-1.19322585901438,-8.11318585606419,
-8.06112117401782));
#44086=CARTESIAN_POINT('Ctrl Pts',(-0.995042175532004,-8.13429661950999,
-8.05957535230316));
#44087=CARTESIAN_POINT('Ctrl Pts',(-0.796352973824406,-8.15013618939897,
-8.05833520502664));
#44088=CARTESIAN_POINT('Ctrl Pts',(-0.597403544878113,-8.16068270620361,
-8.05748174952326));
#44089=CARTESIAN_POINT('Ctrl Pts',(-0.408635679381983,-8.17068948770669,
-8.05667197100556));
#44090=CARTESIAN_POINT('Ctrl Pts',(-0.219633540211193,-8.17593135769825,
-8.05621031569765));
#44091=CARTESIAN_POINT('Ctrl Pts',(-0.030606653255842,-8.17644149281921,
-8.05616518408145));
#44092=CARTESIAN_POINT('Ctrl Pts',(-0.0204111189774602,-8.17646900795315,
-8.05616274981959));
#44093=CARTESIAN_POINT('Ctrl Pts',(-0.0102155127029499,-8.17648277019785,
-8.05616152710882));
#44094=CARTESIAN_POINT('Ctrl Pts',(-1.98673096702962E-5,-8.17648278911332,
-8.05616152661429));
#44095=CARTESIAN_POINT('Ctrl Pts',(-1.32448725733915E-5,-8.1764827891256,
-8.05616152661397));
#44096=CARTESIAN_POINT('Ctrl Pts',(-6.62243549213079E-6,-8.17648278913209,
-8.05616152661416));
#44097=CARTESIAN_POINT('Ctrl Pts',(1.57207580286922E-12,-8.17648278913278,
-8.05616152661487));
#44098=CARTESIAN_POINT('Ctrl Pts',(0.189380764722651,-8.17648280885812,
-8.05616154692102));
#44099=CARTESIAN_POINT('Ctrl Pts',(0.378748155853062,-8.17173673284014,
-8.05658332229546));
#44100=CARTESIAN_POINT('Ctrl Pts',(0.567891470777629,-8.16220840147887,
-8.05735811422046));
#44101=CARTESIAN_POINT('Ctrl Pts',(0.76929744390324,-8.15206232335369,-8.05818313794223));
#44102=CARTESIAN_POINT('Ctrl Pts',(0.970449344071629,-8.13649340887974,
-8.0594084403906));
#44103=CARTESIAN_POINT('Ctrl Pts',(1.17109277311662,-8.11552159247827,-8.06095004077886));
#44104=CARTESIAN_POINT('Ctrl Pts',(1.36687872490619,-8.09505749328269,-8.06245431979129));
#44105=CARTESIAN_POINT('Ctrl Pts',(1.5621805272216,-8.06944945144144,-8.0642597540552));
#44106=CARTESIAN_POINT('Ctrl Pts',(1.75676181475598,-8.03877216157455,-8.06628749697816));
#44107=CARTESIAN_POINT('Ctrl Pts',(1.95858448633675,-8.00695320983338,-8.06839070278574));
#44108=CARTESIAN_POINT('Ctrl Pts',(2.15963201702165,-7.96968067936552,-8.07073306287983));
#44109=CARTESIAN_POINT('Ctrl Pts',(2.35964065808733,-7.92709592124367,-8.07322586199765));
#44110=CARTESIAN_POINT('Ctrl Pts',(2.55964929915301,-7.88451116312181,-8.07571866111547));
#44111=CARTESIAN_POINT('Ctrl Pts',(2.75861905059947,-7.8366145558886,-8.078361884372));
#44112=CARTESIAN_POINT('Ctrl Pts',(2.95628616370335,-7.78360100621361,-8.08106628369463));
#44113=CARTESIAN_POINT('Ctrl Pts',(3.19882702103404,-7.71855249315338,-8.08438462694341));
#44114=CARTESIAN_POINT('Ctrl Pts',(3.43941382619942,-7.64573047320529,-8.08772747266317));
#44115=CARTESIAN_POINT('Ctrl Pts',(3.67765454918082,-7.56538919415433,-8.09078719554358));
#44116=CARTESIAN_POINT('Ctrl Pts',(3.96256884455284,-7.4693083116602,-8.09444634658038));
#44117=CARTESIAN_POINT('Ctrl Pts',(4.24412777542588,-7.36247414363688,-8.09770025029678));
#44118=CARTESIAN_POINT('Ctrl Pts',(4.52166081822969,-7.24539697669584,-8.10002600204554));
#44119=CARTESIAN_POINT('Ctrl Pts',(4.88863124915102,-7.09059069500283,-8.10310124711487));
#44120=CARTESIAN_POINT('Ctrl Pts',(5.2485629478173,-6.91788157640933,-8.10455102844123));
#44121=CARTESIAN_POINT('Ctrl Pts',(5.59990580189133,-6.72852560770424,-8.10319440285958));
#44122=CARTESIAN_POINT('Ctrl Pts',(5.64433782730844,-6.7045790008021,-8.10302283932377));
#44123=CARTESIAN_POINT('Ctrl Pts',(5.68863249132303,-6.68036614677505,-8.1028064622695));
#44124=CARTESIAN_POINT('Ctrl Pts',(5.7327866587865,-6.65588954538727,-8.10254295270174));
#44125=CARTESIAN_POINT('Ctrl Pts',(-5.84422295831999,-6.60976874991002,
-8.11490727298548));
#44126=CARTESIAN_POINT('Ctrl Pts',(-5.38938859865608,-6.87258866136879,
-8.12252792038973));
#44127=CARTESIAN_POINT('Ctrl Pts',(-4.35944142742656,-7.38493398830133,
-8.12651592016639));
#44128=CARTESIAN_POINT('Ctrl Pts',(-2.6946127460268,-7.93716129789442,-8.10974134360217));
#44129=CARTESIAN_POINT('Ctrl Pts',(-0.898320559210476,-8.22897502366934,
-8.09288659504273));
#44130=CARTESIAN_POINT('Ctrl Pts',(0.901429467966184,-8.22872398638616,
-8.09290350846181));
#44131=CARTESIAN_POINT('Ctrl Pts',(2.69770232818102,-7.93640182698235,-8.10977803300697));
#44132=CARTESIAN_POINT('Ctrl Pts',(4.36144900498123,-7.38403171477856,-8.12652349002812));
#44133=CARTESIAN_POINT('Ctrl Pts',(5.39040673669931,-6.87200650754738,-8.12251173095811));
#44134=CARTESIAN_POINT('Ctrl Pts',(5.84433195526982,-6.60970579078957,-8.11490540146884));
#44135=CARTESIAN_POINT('Ctrl Pts',(-5.72538011317797,-6.40695333589681,
-7.90742516593913));
#44136=CARTESIAN_POINT('Ctrl Pts',(-5.27970274304097,-6.66325795360347,
-7.91616927074093));
#44137=CARTESIAN_POINT('Ctrl Pts',(-4.27051957708516,-7.16304589521579,
-7.92255131832025));
#44138=CARTESIAN_POINT('Ctrl Pts',(-2.63947098547294,-7.70187917833143,
-7.90877350684347));
#44139=CARTESIAN_POINT('Ctrl Pts',(-0.879898351178121,-7.98663045155091,
-7.89367055524914));
#44140=CARTESIAN_POINT('Ctrl Pts',(0.882943541812166,-7.98638549093034,
-7.8936859086404));
#44141=CARTESIAN_POINT('Ctrl Pts',(2.64249762386501,-7.70113809089933,-7.90880579224764));
#44142=CARTESIAN_POINT('Ctrl Pts',(4.27248663614319,-7.16216559288129,-7.92255439312653));
#44143=CARTESIAN_POINT('Ctrl Pts',(5.28070038169628,-6.66269021335986,-7.91615058063814));
#44144=CARTESIAN_POINT('Ctrl Pts',(5.72548691629843,-6.40689193398313,-7.90742302702228));
#44145=CARTESIAN_POINT('Ctrl Pts',(-5.71943342809842,-6.40362121884893,
-7.5939596963265));
#44146=CARTESIAN_POINT('Ctrl Pts',(-5.27504920141105,-6.65726716852875,
-7.60270658234416));
#44147=CARTESIAN_POINT('Ctrl Pts',(-4.26853728029364,-7.15224503866711,
-7.60918179401112));
#44148=CARTESIAN_POINT('Ctrl Pts',(-2.63985305700298,-7.68689312320676,
-7.59558855876745));
#44149=CARTESIAN_POINT('Ctrl Pts',(-0.880379460818149,-7.96992923865942,
-7.58057647387013));
#44150=CARTESIAN_POINT('Ctrl Pts',(0.883425978655007,-7.96968558206291,
-7.58059176063567));
#44151=CARTESIAN_POINT('Ctrl Pts',(2.6428776046023,-7.68615698642532,-7.59562058355163));
#44152=CARTESIAN_POINT('Ctrl Pts',(4.2704995400594,-7.15137263723294,-7.60918461824791));
#44153=CARTESIAN_POINT('Ctrl Pts',(5.27604396018071,-6.65670529607616,-7.60268786578122));
#44154=CARTESIAN_POINT('Ctrl Pts',(5.71953991627837,-6.40356045813047,-7.59395755126392));
#44155=CARTESIAN_POINT('Ctrl Pts',(-5.83024166502501,-6.60193592346308,
-7.37785692368633));
#44156=CARTESIAN_POINT('Ctrl Pts',(-5.3784477878881,-6.85850456404399,-7.38548409954249));
#44157=CARTESIAN_POINT('Ctrl Pts',(-4.35478131953797,-7.35954007744269,
-7.38969113283958));
#44158=CARTESIAN_POINT('Ctrl Pts',(-2.69551165346364,-7.90192684740847,
-7.37335052155497));
#44159=CARTESIAN_POINT('Ctrl Pts',(-0.899451974758108,-8.18970778644358,
-7.35670941095802));
#44160=CARTESIAN_POINT('Ctrl Pts',(0.902564004795844,-8.18945981524842,
-7.35672616772986));
#44161=CARTESIAN_POINT('Ctrl Pts',(2.69859632014915,-7.90117901678993,-7.37338659820303));
#44162=CARTESIAN_POINT('Ctrl Pts',(4.35677761289836,-7.35865638110693,-7.38969811357579));
#44163=CARTESIAN_POINT('Ctrl Pts',(5.37945915464754,-6.85793620703642,-7.38546784792074));
#44164=CARTESIAN_POINT('Ctrl Pts',(5.83034992147577,-6.60187447197138,-7.37785503772092));
#44165=CARTESIAN_POINT('Ctrl Pts',(-5.7200175232721,-6.64700781289157,-7.39409107725312));
#44166=CARTESIAN_POINT('Ctrl Pts',(-5.51371324185327,-6.76166932142692,
-7.39720426684975));
#44167=CARTESIAN_POINT('Ctrl Pts',(-5.30244990809323,-6.87155186606564,
-7.39917723806279));
#44168=CARTESIAN_POINT('Ctrl Pts',(-5.08630387814312,-6.97606931525954,
-7.40024850210269));
#44169=CARTESIAN_POINT('Ctrl Pts',(-4.87015784819301,-7.08058676445345,
-7.40131976614259));
#44170=CARTESIAN_POINT('Ctrl Pts',(-4.64912885670142,-7.17973930199014,
-7.40148918223241));
#44171=CARTESIAN_POINT('Ctrl Pts',(-4.4233223550221,-7.27289273489692,-7.40101846283964));
#44172=CARTESIAN_POINT('Ctrl Pts',(-4.41102142472513,-7.27796731812011,
-7.40099282014823));
#44173=CARTESIAN_POINT('Ctrl Pts',(-4.39870632454384,-7.28302408624263,
-7.40096528384693));
#44174=CARTESIAN_POINT('Ctrl Pts',(-4.38637708600296,-7.28806293330809,
-7.40093589965471));
#44175=CARTESIAN_POINT('Ctrl Pts',(-4.17423011394607,-7.37476546112847,
-7.400430291187));
#44176=CARTESIAN_POINT('Ctrl Pts',(-3.95789714003301,-7.45617951152167,
-7.39936226650764));
#44177=CARTESIAN_POINT('Ctrl Pts',(-3.73752760079179,-7.53183568206427,
-7.39788683592457));
#44178=CARTESIAN_POINT('Ctrl Pts',(-3.71639529957566,-7.53909071826515,
-7.39774534974816));
#44179=CARTESIAN_POINT('Ctrl Pts',(-3.69522588741974,-7.54629276995919,
-7.39760013151133));
#44180=CARTESIAN_POINT('Ctrl Pts',(-3.67401950167808,-7.55344139995593,
-7.39745132725152));
#44181=CARTESIAN_POINT('Ctrl Pts',(-3.55284525913626,-7.59428899348834,
-7.39660105301393));
#44182=CARTESIAN_POINT('Ctrl Pts',(-3.43046441960889,-7.63339399527552,
-7.39563199523097));
#44183=CARTESIAN_POINT('Ctrl Pts',(-3.30690773257217,-7.67068044224599,
-7.39456257166012));
#44184=CARTESIAN_POINT('Ctrl Pts',(-3.24512938905381,-7.68932366573122,
-7.3940278598747));
#44185=CARTESIAN_POINT('Ctrl Pts',(-3.18305707852317,-7.70751223189553,
-7.39346803903621));
#44186=CARTESIAN_POINT('Ctrl Pts',(-3.12069513729051,-7.72523682409344,
-7.39288485977133));
#44187=CARTESIAN_POINT('Ctrl Pts',(-3.08951416667418,-7.73409912019239,
-7.39259327013889));
#44188=CARTESIAN_POINT('Ctrl Pts',(-3.05826078818309,-7.74284542176459,
-7.39229583995104));
#44189=CARTESIAN_POINT('Ctrl Pts',(-3.02693555934582,-7.75147456866553,
-7.39199276680285));
#44190=CARTESIAN_POINT('Ctrl Pts',(-3.0038616182549,-7.75783073698889,-7.3917695252743));
#44191=CARTESIAN_POINT('Ctrl Pts',(-2.97980770982277,-7.76437813570979,
-7.39153386934831));
#44192=CARTESIAN_POINT('Ctrl Pts',(-2.95685308918717,-7.77055206877725,
-7.39130652327029));
#44193=CARTESIAN_POINT('Ctrl Pts',(-2.94864447067566,-7.77275987966077,
-7.39122522385549));
#44194=CARTESIAN_POINT('Ctrl Pts',(-2.94057656484299,-7.77492041245755,
-7.39114499476737));
#44195=CARTESIAN_POINT('Ctrl Pts',(-2.93274488786755,-7.77700938676643,
-7.39106680435592));
#44196=CARTESIAN_POINT('Ctrl Pts',(-2.84286196192221,-7.80098421663956,
-7.3901694252909));
#44197=CARTESIAN_POINT('Ctrl Pts',(-2.75267957579997,-7.82388471216904,
-7.38926607338874));
#44198=CARTESIAN_POINT('Ctrl Pts',(-2.66221234566274,-7.84569650678844,
-7.38837077971031));
#44199=CARTESIAN_POINT('Ctrl Pts',(-2.40391363455117,-7.9079727412733,-7.38581457009881));
#44200=CARTESIAN_POINT('Ctrl Pts',(-2.14329376638944,-7.96137761868093,
-7.38332392021102));
#44201=CARTESIAN_POINT('Ctrl Pts',(-1.88082100481702,-8.00567783504727,
-7.38110967219702));
#44202=CARTESIAN_POINT('Ctrl Pts',(-1.62315194251182,-8.04916728188605,
-7.37893594869877));
#44203=CARTESIAN_POINT('Ctrl Pts',(-1.36369666562235,-8.08388241259931,
-7.37702839999861));
#44204=CARTESIAN_POINT('Ctrl Pts',(-1.10289072817735,-8.10955302367032,
-7.37558982376376));
#44205=CARTESIAN_POINT('Ctrl Pts',(-1.0302688443648,-8.11670105163647,-7.37518924961577));
#44206=CARTESIAN_POINT('Ctrl Pts',(-0.957542217175731,-8.12314750265828,
-7.374825067595));
#44207=CARTESIAN_POINT('Ctrl Pts',(-0.884720229343273,-8.12888581949315,
-7.37450173617424));
#44208=CARTESIAN_POINT('Ctrl Pts',(-0.621866153454331,-8.14959851923789,
-7.37333465759893));
#44209=CARTESIAN_POINT('Ctrl Pts',(-0.357769019522488,-8.16108897896362,
-7.37269961871155));
#44210=CARTESIAN_POINT('Ctrl Pts',(-0.0929439746577478,-8.16327002316267,
-7.37257848004112));
#44211=CARTESIAN_POINT('Ctrl Pts',(-0.0619677561530355,-8.16352513688015,
-7.37256431061872));
#44212=CARTESIAN_POINT('Ctrl Pts',(-0.0309815892461447,-8.16365282469521,
-7.37255717553758));
#44213=CARTESIAN_POINT('Ctrl Pts',(1.36919838106928E-5,-8.16365290107928,
-7.37255704847296));
#44214=CARTESIAN_POINT('Ctrl Pts',(0.260481133587845,-8.1636535429694,-7.3725559806912));
#44215=CARTESIAN_POINT('Ctrl Pts',(0.520290709605892,-8.15466266469011,
-7.37303196871935));
#44216=CARTESIAN_POINT('Ctrl Pts',(0.778967847162538,-8.13675976149421,
-7.37401334251466));
#44217=CARTESIAN_POINT('Ctrl Pts',(0.815264655427029,-8.1342476792483,-7.37415104597319));
#44218=CARTESIAN_POINT('Ctrl Pts',(0.851539175291451,-8.13156004608175,
-7.37429870473853));
#44219=CARTESIAN_POINT('Ctrl Pts',(0.887790101292666,-8.12869700051921,
-7.37445640166713));
#44220=CARTESIAN_POINT('Ctrl Pts',(1.08697684364434,-8.11296552047956,-7.37532289367028));
#44221=CARTESIAN_POINT('Ctrl Pts',(1.28545136831308,-8.09193964782705,-7.37649227436005));
#44222=CARTESIAN_POINT('Ctrl Pts',(1.48302725142221,-8.06574169304764,-7.37787936089373));
#44223=CARTESIAN_POINT('Ctrl Pts',(1.72792448366118,-8.03326907283289,-7.37959866816763));
#44224=CARTESIAN_POINT('Ctrl Pts',(1.97142847485369,-7.99282198952477,-7.38168606335154));
#44225=CARTESIAN_POINT('Ctrl Pts',(2.21317518510619,-7.94461687274513,-7.38396070087494));
#44226=CARTESIAN_POINT('Ctrl Pts',(2.33404854023243,-7.92051431435531,-7.38509801963663));
#44227=CARTESIAN_POINT('Ctrl Pts',(2.45448288511245,-7.89447302683783,-7.38628058810975));
#44228=CARTESIAN_POINT('Ctrl Pts',(2.5744345461666,-7.86652469780926,-7.38747652781115));
#44229=CARTESIAN_POINT('Ctrl Pts',(2.60474934218281,-7.85946145344858,-7.38777877179658));
#44230=CARTESIAN_POINT('Ctrl Pts',(2.6350333592709,-7.85227644061828,-7.38808180844263));
#44231=CARTESIAN_POINT('Ctrl Pts',(2.66528580642343,-7.84497013890992,-7.38838515239865));
#44232=CARTESIAN_POINT('Ctrl Pts',(2.694885836671,-7.83782140312418,-7.38868195451282));
#44233=CARTESIAN_POINT('Ctrl Pts',(2.72445564398435,-7.83055655339874,-7.3889790508266));
#44234=CARTESIAN_POINT('Ctrl Pts',(2.75399469624353,-7.82317623364713,-7.38927581213863));
#44235=CARTESIAN_POINT('Ctrl Pts',(2.78385928494455,-7.81571457875279,-7.38957584392192));
#44236=CARTESIAN_POINT('Ctrl Pts',(2.81369238495066,-7.80813485455885,-7.38987558891595));
#44237=CARTESIAN_POINT('Ctrl Pts',(2.8434933475593,-7.80043765701813,-7.3901744906164));
#44238=CARTESIAN_POINT('Ctrl Pts',(2.86560649665769,-7.79472612081399,-7.39039628405156));
#44239=CARTESIAN_POINT('Ctrl Pts',(2.88674831666762,-7.78920060926862,-7.39060806890174));
#44240=CARTESIAN_POINT('Ctrl Pts',(2.90904172325111,-7.7833043905423,-7.39083087286923));
#44241=CARTESIAN_POINT('Ctrl Pts',(2.91679220472072,-7.78125452284676,-7.3909083324542));
#44242=CARTESIAN_POINT('Ctrl Pts',(2.92468175519996,-7.77915941817535,-7.39098711927652));
#44243=CARTESIAN_POINT('Ctrl Pts',(2.93279917759592,-7.77699424572049,-7.391068097953));
#44244=CARTESIAN_POINT('Ctrl Pts',(3.15805061537049,-7.71691258621102,-7.39331518605765));
#44245=CARTESIAN_POINT('Ctrl Pts',(3.37963538387188,-7.65068123739186,-7.39538046713975));
#44246=CARTESIAN_POINT('Ctrl Pts',(3.59738192019367,-7.57882478942696,-7.39706852248287));
#44247=CARTESIAN_POINT('Ctrl Pts',(3.82052223618586,-7.5051883919172,-7.39879839249155));
#44248=CARTESIAN_POINT('Ctrl Pts',(4.03963186912597,-7.42564470520827,-7.40013221739745));
#44249=CARTESIAN_POINT('Ctrl Pts',(4.25454557778461,-7.34071227879178,-7.40088182818385));
#44250=CARTESIAN_POINT('Ctrl Pts',(4.31206231045888,-7.31798205978405,-7.401082444345));
#44251=CARTESIAN_POINT('Ctrl Pts',(4.36927861548813,-7.29486562978467,-7.40124133192306));
#44252=CARTESIAN_POINT('Ctrl Pts',(4.42619154442692,-7.27137239769755,-7.40135512978351));
#44253=CARTESIAN_POINT('Ctrl Pts',(4.65147047778588,-7.17837893620424,-7.40180557682775));
#44254=CARTESIAN_POINT('Ctrl Pts',(4.8719950275897,-7.07948568452959,-7.40154785261369));
#44255=CARTESIAN_POINT('Ctrl Pts',(5.08766384430848,-6.97524835766162,-7.40039572003413));
#44256=CARTESIAN_POINT('Ctrl Pts',(5.30333266102726,-6.87101103079365,-7.39924358745457));
#44257=CARTESIAN_POINT('Ctrl Pts',(5.51414587167326,-6.76142934734901,-7.39719722479767));
#44258=CARTESIAN_POINT('Ctrl Pts',(5.72001467857883,-6.64700991222121,-7.39409062851839));
#44259=CARTESIAN_POINT('Ctrl Pts',(6.05066939030811,-10.3127953565056,-1.22617515269708));
#44260=CARTESIAN_POINT('Ctrl Pts',(6.05130921732087,-10.3094309468474,-1.25222015897757));
#44261=CARTESIAN_POINT('Ctrl Pts',(6.04716617417261,-10.3028567867706,-1.31997136664705));
#44262=CARTESIAN_POINT('Ctrl Pts',(6.01576910230258,-10.3008720417499,-1.43277663512264));
#44263=CARTESIAN_POINT('Ctrl Pts',(5.94717377016299,-10.3112693333796,-1.55348066131538));
#44264=CARTESIAN_POINT('Ctrl Pts',(5.84901708021604,-10.334275868274,-1.65610810365757));
#44265=CARTESIAN_POINT('Ctrl Pts',(5.76450435111265,-10.3583100007465,-1.70838528469582));
#44266=CARTESIAN_POINT('Ctrl Pts',(5.71748516972109,-10.37274644705,-1.72859734565015));
#44267=CARTESIAN_POINT('Ctrl Pts',(5.71213042723896,-10.3744035443872,-1.73079093733939));
#44268=CARTESIAN_POINT('Ctrl Pts',(5.91207393029035,-10.0311964577302,-1.19349828764901));
#44269=CARTESIAN_POINT('Ctrl Pts',(5.91266157430069,-10.0281594687441,-1.21694391136227));
#44270=CARTESIAN_POINT('Ctrl Pts',(5.90886049650901,-10.0222648764306,-1.27818392833765));
#44271=CARTESIAN_POINT('Ctrl Pts',(5.87975076332791,-10.0208075082426,-1.38101232835033));
#44272=CARTESIAN_POINT('Ctrl Pts',(5.81578180589495,-10.0310304108616,-1.49171175501008));
#44273=CARTESIAN_POINT('Ctrl Pts',(5.72402711176062,-10.0530519067873,-1.58611209758615));
#44274=CARTESIAN_POINT('Ctrl Pts',(5.64503109213434,-10.0757988066388,-1.6342245583265));
#44275=CARTESIAN_POINT('Ctrl Pts',(5.60113930969898,-10.089381109962,-1.65281889954393));
#44276=CARTESIAN_POINT('Ctrl Pts',(5.59614154922131,-10.0909391882732,-1.65483685123968));
#44277=CARTESIAN_POINT('Ctrl Pts',(6.02856620736513,-9.74070678474308,-1.15324175165922));
#44278=CARTESIAN_POINT('Ctrl Pts',(6.02948707486004,-9.73604662848835,-1.18936361391473));
#44279=CARTESIAN_POINT('Ctrl Pts',(6.02349351115603,-9.72707553668167,-1.28184356126626));
#44280=CARTESIAN_POINT('Ctrl Pts',(5.98036953308613,-9.72431468556907,-1.43080025677482));
#44281=CARTESIAN_POINT('Ctrl Pts',(5.88895461810126,-9.7375088295263,-1.58654545187936));
#44282=CARTESIAN_POINT('Ctrl Pts',(5.75979132356852,-9.76686971121646,-1.71781231137828));
#44283=CARTESIAN_POINT('Ctrl Pts',(5.64854720753488,-9.79791761496062,-1.78497284675799));
#44284=CARTESIAN_POINT('Ctrl Pts',(5.58621679756139,-9.81682449515364,-1.81115576311391));
#44285=CARTESIAN_POINT('Ctrl Pts',(5.57911215103403,-9.81899805900445,-1.81400075163189));
#44286=CARTESIAN_POINT('Ctrl Pts',(6.32386216337528,-9.63155076077824,-1.13176716249797));
#44287=CARTESIAN_POINT('Ctrl Pts',(6.32528345230293,-9.62437976652278,-1.18753995793898));
#44288=CARTESIAN_POINT('Ctrl Pts',(6.31599868199734,-9.61059072740038,-1.32855375525905));
#44289=CARTESIAN_POINT('Ctrl Pts',(6.25173598350599,-9.60554910845383,-1.54953718978642));
#44290=CARTESIAN_POINT('Ctrl Pts',(6.11877552868139,-9.62291443242936,-1.77588068427804));
#44291=CARTESIAN_POINT('Ctrl Pts',(5.93288973882408,-9.66313299096965,-1.9649659533792));
#44292=CARTESIAN_POINT('Ctrl Pts',(5.77275010998209,-9.70663429398153,-2.0619138892666));
#44293=CARTESIAN_POINT('Ctrl Pts',(5.6824894231339,-9.73355771741979,-2.09992236202094));
#44294=CARTESIAN_POINT('Ctrl Pts',(5.67219369876869,-9.73665822595086,-2.10405548617845));
#44295=CARTESIAN_POINT('',(5.73278505653102,-10.3449524964723,-1.71289224212846));
#44296=CARTESIAN_POINT('',(5.72001587123307,-9.72697769588761,-2.0594345452005));
#44297=CARTESIAN_POINT('Origin',(5.89875825683544,-10.1838012062076,-2.15614435592649));
#44298=CARTESIAN_POINT('',(5.99999998667943,-9.65438790406946,-1.86247695099856));
#44299=CARTESIAN_POINT('Ctrl Pts',(6.00000003796097,-9.65438809185475,-1.86247698722521));
#44300=CARTESIAN_POINT('Ctrl Pts',(5.95882273790821,-9.66348805825028,-1.90324205679966));
#44301=CARTESIAN_POINT('Ctrl Pts',(5.91487788445314,-9.67407471952828,-1.93999595034449));
#44302=CARTESIAN_POINT('Ctrl Pts',(5.86822767748739,-9.68615017643769,-1.97285849162915));
#44303=CARTESIAN_POINT('Ctrl Pts',(5.82157747052231,-9.69822563334693,-2.00572103291333));
#44304=CARTESIAN_POINT('Ctrl Pts',(5.77222173582301,-9.71178946761864,-2.03469214155817));
#44305=CARTESIAN_POINT('Ctrl Pts',(5.72001606109556,-9.72697818111165,-2.0594346479375));
#44306=CARTESIAN_POINT('',(5.99998684676694,-10.0933419068472,-1.2110347738228));
#44307=CARTESIAN_POINT('Ctrl Pts',(5.99998684676694,-10.0933419068472,-1.2110347738228));
#44308=CARTESIAN_POINT('Ctrl Pts',(5.99998481317996,-10.0709318263906,-1.22812637108207));
#44309=CARTESIAN_POINT('Ctrl Pts',(5.99998609830006,-10.0492937981165,-1.2455430819064));
#44310=CARTESIAN_POINT('Ctrl Pts',(5.99998227627453,-10.0284575477685,-1.26330025491489));
#44311=CARTESIAN_POINT('Ctrl Pts',(5.99998116448161,-10.0223964695217,-1.26846565719452));
#44312=CARTESIAN_POINT('Ctrl Pts',(5.99997943623455,-10.0164030435298,-1.27365962773701));
#44313=CARTESIAN_POINT('Ctrl Pts',(5.99997660921889,-10.0104775368722,-1.27888202729153));
#44314=CARTESIAN_POINT('Ctrl Pts',(5.99996297131451,-9.98189209455754,-1.30407558622867));
#44315=CARTESIAN_POINT('Ctrl Pts',(5.99992758485034,-9.954890878723,-1.32993076951105));
#44316=CARTESIAN_POINT('Ctrl Pts',(5.99991487015089,-9.92942364904202,-1.35643845475696));
#44317=CARTESIAN_POINT('Ctrl Pts',(5.99991410384967,-9.92788876656782,-1.35803604436625));
#44318=CARTESIAN_POINT('Ctrl Pts',(5.99991341291059,-9.92635944489813,-1.35963600871984));
#44319=CARTESIAN_POINT('Ctrl Pts',(5.99991280551292,-9.92483566959625,-1.36123834883611));
#44320=CARTESIAN_POINT('Ctrl Pts',(5.99990375315627,-9.90212607069442,-1.38511883915503));
#44321=CARTESIAN_POINT('Ctrl Pts',(5.99990215490928,-9.88067245865394,-1.40953845039357));
#44322=CARTESIAN_POINT('Ctrl Pts',(5.99990391521304,-9.86048117020938,-1.43448402417505));
#44323=CARTESIAN_POINT('Ctrl Pts',(5.99990506541729,-9.84728793261089,-1.45078377061438));
#44324=CARTESIAN_POINT('Ctrl Pts',(5.99990801397928,-9.83463312599759,-1.46730846004701));
#44325=CARTESIAN_POINT('Ctrl Pts',(5.99991561449138,-9.82251772060994,-1.48406637309734));
#44326=CARTESIAN_POINT('Ctrl Pts',(5.99991855526553,-9.81783005346036,-1.49055030953925));
#44327=CARTESIAN_POINT('Ctrl Pts',(5.99992663423283,-9.81306236424672,-1.49728724114274));
#44328=CARTESIAN_POINT('Ctrl Pts',(5.99993199795079,-9.80844193835796,-1.50398256147571));
#44329=CARTESIAN_POINT('Ctrl Pts',(5.99993742991546,-9.80376272322492,-1.51076307153622));
#44330=CARTESIAN_POINT('Ctrl Pts',(5.99993980443271,-9.79923474176042,-1.5175006375891));
#44331=CARTESIAN_POINT('Ctrl Pts',(5.99994481678224,-9.79505843631892,-1.52385025354702));
#44332=CARTESIAN_POINT('Ctrl Pts',(5.99994564462708,-9.79436867338557,-1.5248989626968));
#44333=CARTESIAN_POINT('Ctrl Pts',(5.99994657878526,-9.79368842452149,-1.52593701198677));
#44334=CARTESIAN_POINT('Ctrl Pts',(5.99994768557723,-9.79301850146117,-1.52696276047398));
#44335=CARTESIAN_POINT('Ctrl Pts',(5.99997440659629,-9.77684470615519,-1.55172716559746));
#44336=CARTESIAN_POINT('Ctrl Pts',(5.99996041292407,-9.76199870702985,-1.57678838130543));
#44337=CARTESIAN_POINT('Ctrl Pts',(5.99993581405304,-9.74841451382906,-1.60209969757037));
#44338=CARTESIAN_POINT('Ctrl Pts',(5.9999133458294,-9.73600692445224,-1.62521865753805));
#44339=CARTESIAN_POINT('Ctrl Pts',(5.99988325061035,-9.72465152383613,-1.64854730625723));
#44340=CARTESIAN_POINT('Ctrl Pts',(5.99986690142854,-9.71432348654574,-1.67207885292539));
#44341=CARTESIAN_POINT('Ctrl Pts',(5.9998499952577,-9.70364359045972,-1.6964120796647));
#44342=CARTESIAN_POINT('Ctrl Pts',(5.99984921018281,-9.6940616097742,-1.72096348561248));
#44343=CARTESIAN_POINT('Ctrl Pts',(5.99986989539589,-9.6855862564238,-1.7457479612625));
#44344=CARTESIAN_POINT('Ctrl Pts',(5.99988995086758,-9.6773689270412,-1.76977789742815));
#44345=CARTESIAN_POINT('Ctrl Pts',(5.99993074885979,-9.67019227989532,-1.79402798208124));
#44346=CARTESIAN_POINT('Ctrl Pts',(5.99996386685918,-9.66409962585232,-1.81851012398838));
#44347=CARTESIAN_POINT('Ctrl Pts',(5.99998358101823,-9.66047285029037,-1.833083614186));
#44348=CARTESIAN_POINT('Ctrl Pts',(5.99999988542516,-9.65723085510648,-1.84773922258285));
#44349=CARTESIAN_POINT('Ctrl Pts',(5.9999998883105,-9.65438772860653,-1.86247691714912));
#44350=CARTESIAN_POINT('Ctrl Pts',(5.99998684676694,-10.0933419068472,-1.2110347738228));
#44351=CARTESIAN_POINT('Ctrl Pts',(5.99998426938999,-10.0961503515468,-1.22746145677463));
#44352=CARTESIAN_POINT('Ctrl Pts',(5.99923948339792,-10.0995808523923,-1.24481847430359));
#44353=CARTESIAN_POINT('Ctrl Pts',(5.99754684899445,-10.1037210615654,-1.26300200081039));
#44354=CARTESIAN_POINT('Ctrl Pts',(5.9968763249387,-10.1053611734765,-1.27020526450167));
#44355=CARTESIAN_POINT('Ctrl Pts',(5.99605684860915,-10.107112741282,-1.27753773151475));
#44356=CARTESIAN_POINT('Ctrl Pts',(5.99507466942231,-10.1089815685309,-1.28499086684201));
#44357=CARTESIAN_POINT('Ctrl Pts',(5.99262347430917,-10.1136455445967,-1.30359143294694));
#44358=CARTESIAN_POINT('Ctrl Pts',(5.98915863196479,-10.119039980799,-1.32294760085419));
#44359=CARTESIAN_POINT('Ctrl Pts',(5.98451505832419,-10.1252388252198,-1.34289325113992));
#44360=CARTESIAN_POINT('Ctrl Pts',(5.98028205895253,-10.1308895818501,-1.36107535218136));
#44361=CARTESIAN_POINT('Ctrl Pts',(5.97506991267794,-10.1372086565094,-1.379747387453));
#44362=CARTESIAN_POINT('Ctrl Pts',(5.96874928910461,-10.144252797769,-1.3987369167749));
#44363=CARTESIAN_POINT('Ctrl Pts',(5.96715206381112,-10.1460328564073,-1.40353558200036));
#44364=CARTESIAN_POINT('Ctrl Pts',(5.96548401521494,-10.147859224561,-1.4083542693434));
#44365=CARTESIAN_POINT('Ctrl Pts',(5.96374296268477,-10.1497328399762,-1.41318965844888));
#44366=CARTESIAN_POINT('Ctrl Pts',(5.96325809545566,-10.1502546247581,-1.41453627015452));
#44367=CARTESIAN_POINT('Ctrl Pts',(5.9627675659131,-10.1507800739942,-1.41588417576981));
#44368=CARTESIAN_POINT('Ctrl Pts',(5.96227134381333,-10.1513092015444,-1.4172333118891));
#44369=CARTESIAN_POINT('Ctrl Pts',(5.95760675368347,-10.1562831096983,-1.42991546979536));
#44370=CARTESIAN_POINT('Ctrl Pts',(5.9524390259647,-10.1615821167091,-1.44270716308485));
#44371=CARTESIAN_POINT('Ctrl Pts',(5.94674392266645,-10.1672172490246,-1.45555037537036));
#44372=CARTESIAN_POINT('Ctrl Pts',(5.94389637101732,-10.1700348151824,-1.46197198151312));
#44373=CARTESIAN_POINT('Ctrl Pts',(5.94091693215639,-10.1729364220193,-1.46840644352367));
#44374=CARTESIAN_POINT('Ctrl Pts',(5.93780276751921,-10.1759233538012,-1.47484536375715));
#44375=CARTESIAN_POINT('Ctrl Pts',(5.93624568520062,-10.1774168196921,-1.47806482387389));
#44376=CARTESIAN_POINT('Ctrl Pts',(5.93465491803602,-10.1789316175185,-1.48128539676445));
#44377=CARTESIAN_POINT('Ctrl Pts',(5.93303010738351,-10.1804679076617,-1.4845059837072));
#44378=CARTESIAN_POINT('Ctrl Pts',(5.93196067779295,-10.1814790741852,-1.48662573284243));
#44379=CARTESIAN_POINT('Ctrl Pts',(5.93060067674035,-10.1827593132383,-1.48928202609314));
#44380=CARTESIAN_POINT('Ctrl Pts',(5.92949260106467,-10.1837965823635,-1.4914137818749));
#44381=CARTESIAN_POINT('Ctrl Pts',(5.9289171501412,-10.1843352617056,-1.49252085502897));
#44382=CARTESIAN_POINT('Ctrl Pts',(5.92841059870599,-10.1848080231713,-1.4934870775402));
#44383=CARTESIAN_POINT('Ctrl Pts',(5.92805317832642,-10.1851414168011,-1.49416665862601));
#44384=CARTESIAN_POINT('Ctrl Pts',(5.92203018796046,-10.1907595257142,-1.50561846878198));
#44385=CARTESIAN_POINT('Ctrl Pts',(5.91521672355695,-10.19699388167,-1.51774083623431));
#44386=CARTESIAN_POINT('Ctrl Pts',(5.90747417723844,-10.2039017430124,-1.53037783789015));
#44387=CARTESIAN_POINT('Ctrl Pts',(5.90656459425261,-10.2047132684314,-1.53186241431051));
#44388=CARTESIAN_POINT('Ctrl Pts',(5.90564218022057,-10.2055340931858,-1.5333540344392));
#44389=CARTESIAN_POINT('Ctrl Pts',(5.90470670386827,-10.2063643133579,-1.53485239646646));
#44390=CARTESIAN_POINT('Ctrl Pts',(5.89691024349106,-10.2132835461743,-1.54734006667594));
#44391=CARTESIAN_POINT('Ctrl Pts',(5.88820589338057,-10.2208555536035,-1.56029993766635));
#44392=CARTESIAN_POINT('Ctrl Pts',(5.87847600952666,-10.229129372186,-1.57354685685025));
#44393=CARTESIAN_POINT('Ctrl Pts',(5.8695253575908,-10.2367405699583,-1.58573287721985));
#44394=CARTESIAN_POINT('Ctrl Pts',(5.85970668664249,-10.2449456918696,-1.59816197806437));
#44395=CARTESIAN_POINT('Ctrl Pts',(5.84893607357442,-10.2537808325076,-1.61064804237114));
#44396=CARTESIAN_POINT('Ctrl Pts',(5.84055528470297,-10.2606555988621,-1.62036365169894));
#44397=CARTESIAN_POINT('Ctrl Pts',(5.83159823346717,-10.2679117770402,-1.63011310189377));
#44398=CARTESIAN_POINT('Ctrl Pts',(5.82203000190611,-10.2755653475831,-1.63978717038512));
#44399=CARTESIAN_POINT('Ctrl Pts',(5.81023610680679,-10.2849992129262,-1.65171152111205));
#44400=CARTESIAN_POINT('Ctrl Pts',(5.7975122424402,-10.2950373199467,-1.66352224698458));
#44401=CARTESIAN_POINT('Ctrl Pts',(5.78382720703097,-10.3056961993029,-1.67500097984752));
#44402=CARTESIAN_POINT('Ctrl Pts',(5.77101414445683,-10.3156759241686,-1.68574831940832));
#44403=CARTESIAN_POINT('Ctrl Pts',(5.75735837270392,-10.3261997944818,-1.6962048619838));
#44404=CARTESIAN_POINT('Ctrl Pts',(5.74285647658939,-10.3372754895292,-1.70615098188076));
#44405=CARTESIAN_POINT('Ctrl Pts',(5.73954258787944,-10.3398064427564,-1.7084238111835));
#44406=CARTESIAN_POINT('Ctrl Pts',(5.73618461711692,-10.3423661872688,-1.71066980157742));
#44407=CARTESIAN_POINT('Ctrl Pts',(5.73278271249385,-10.3449547711923,-1.7128859870255));
#44408=CARTESIAN_POINT('Ctrl Pts',(5.99928507441619,-19.6591035773105,-0.0581387038097093));
#44409=CARTESIAN_POINT('Ctrl Pts',(5.99928507441619,-19.6322147488868,-0.0775484860915536));
#44410=CARTESIAN_POINT('Ctrl Pts',(5.99928507441619,-19.2058449769004,-0.38207282190903));
#44411=CARTESIAN_POINT('Ctrl Pts',(5.99928507441619,-18.3334658087218,-0.906210204715289));
#44412=CARTESIAN_POINT('Ctrl Pts',(5.99928507441619,-16.9710147391481,-1.46998745478167));
#44413=CARTESIAN_POINT('Ctrl Pts',(5.99928507441619,-15.5398213819416,-1.82605993958607));
#44414=CARTESIAN_POINT('Ctrl Pts',(5.99928507441619,-14.0709556091875,-1.9661845044543));
#44415=CARTESIAN_POINT('Ctrl Pts',(5.99928507441619,-12.5966799711141,-1.88736698540332));
#44416=CARTESIAN_POINT('Ctrl Pts',(5.99928507441619,-11.2335282355129,-1.60731118852257));
#44417=CARTESIAN_POINT('Ctrl Pts',(5.99928507441619,-10.3852024002489,-1.308971212486));
#44418=CARTESIAN_POINT('Ctrl Pts',(5.99928507441619,-10.0105704181296,-1.15061620805415));
#44419=CARTESIAN_POINT('Ctrl Pts',(6.0106662077061,-19.7703827345453,-0.212268579484425));
#44420=CARTESIAN_POINT('Ctrl Pts',(6.0106662077061,-19.7429754823504,-0.232052356751892));
#44421=CARTESIAN_POINT('Ctrl Pts',(6.0106662077061,-19.308392033223,-0.542440795747545));
#44422=CARTESIAN_POINT('Ctrl Pts',(6.0106662077061,-18.4193939491244,-1.0765722015714));
#44423=CARTESIAN_POINT('Ctrl Pts',(6.0106662077061,-17.0306058173753,-1.65124564686108));
#44424=CARTESIAN_POINT('Ctrl Pts',(6.0106662077061,-15.5720774343996,-2.01411525356481));
#44425=CARTESIAN_POINT('Ctrl Pts',(6.0106662077061,-14.0748737875543,-2.15695124058169));
#44426=CARTESIAN_POINT('Ctrl Pts',(6.0106662077061,-12.5723725487962,-2.07661671511421));
#44427=CARTESIAN_POINT('Ctrl Pts',(6.0106662077061,-11.1829429890494,-1.79116790615583));
#44428=CARTESIAN_POINT('Ctrl Pts',(6.0106662077061,-10.3184089964746,-1.48712752681436));
#44429=CARTESIAN_POINT('Ctrl Pts',(6.0106662077061,-9.93655135940431,-1.32571656146796));
#44430=CARTESIAN_POINT('Ctrl Pts',(5.90294096085745,-19.862565198381,-0.339948120237213));
#44431=CARTESIAN_POINT('Ctrl Pts',(5.90294096085745,-19.8347284894849,-0.360041710955224));
#44432=CARTESIAN_POINT('Ctrl Pts',(5.90294096085745,-19.3933409180546,-0.675287910315859));
#44433=CARTESIAN_POINT('Ctrl Pts',(5.90294096085745,-18.4905759017301,-1.21769825793309));
#44434=CARTESIAN_POINT('Ctrl Pts',(5.90294096085745,-17.0799704293154,-1.80139799481888));
#44435=CARTESIAN_POINT('Ctrl Pts',(5.90294096085745,-15.5987980033129,-2.1698982646174));
#44436=CARTESIAN_POINT('Ctrl Pts',(5.90294096085745,-14.0781195646156,-2.31498036474823));
#44437=CARTESIAN_POINT('Ctrl Pts',(5.90294096085745,-12.5522365400888,-2.23338916738684));
#44438=CARTESIAN_POINT('Ctrl Pts',(5.90294096085745,-11.1410387118318,-1.94347284489393));
#44439=CARTESIAN_POINT('Ctrl Pts',(5.90294096085745,-10.2630780550711,-1.63471031241584));
#44440=CARTESIAN_POINT('Ctrl Pts',(5.90294096085745,-9.87523476270989,-1.47076782172808));
#44441=CARTESIAN_POINT('Ctrl Pts',(5.72069737671822,-19.8963286151593,-0.386712953469083));
#44442=CARTESIAN_POINT('Ctrl Pts',(5.72069737671822,-19.8683346103358,-0.406920018701532));
#44443=CARTESIAN_POINT('Ctrl Pts',(5.72069737671822,-19.4244549117969,-0.723945456553586));
#44444=CARTESIAN_POINT('Ctrl Pts',(5.72069737671822,-18.5166475191755,-1.26938810934469));
#44445=CARTESIAN_POINT('Ctrl Pts',(5.72069737671822,-17.0980510695729,-1.85639388115812));
#44446=CARTESIAN_POINT('Ctrl Pts',(5.72069737671822,-15.6085848723892,-2.2269564784001));
#44447=CARTESIAN_POINT('Ctrl Pts',(5.72069737671822,-14.0793083864286,-2.37286125618635));
#44448=CARTESIAN_POINT('Ctrl Pts',(5.72069737671822,-12.5448613797185,-2.29080978107595));
#44449=CARTESIAN_POINT('Ctrl Pts',(5.72069737671822,-11.1256905477962,-1.99925715472402));
#44450=CARTESIAN_POINT('Ctrl Pts',(5.72069737671822,-10.2428121437751,-1.68876505223976));
#44451=CARTESIAN_POINT('Ctrl Pts',(5.72069737671822,-9.85277650196055,-1.52389534674733));
#44452=CARTESIAN_POINT('',(6.,-19.5919343770476,-0.135488060647564));
#44453=CARTESIAN_POINT('Ctrl Pts',(5.99999999999966,-19.5919343770476,-0.135488060647564));
#44454=CARTESIAN_POINT('Ctrl Pts',(5.99999999999966,-19.4672328514344,-0.223609559568266));
#44455=CARTESIAN_POINT('Ctrl Pts',(6.00000000003739,-19.3409290917707,-0.308575891732745));
#44456=CARTESIAN_POINT('Ctrl Pts',(5.99999999795214,-19.2129690542321,-0.390478611967978));
#44457=CARTESIAN_POINT('Ctrl Pts',(5.99999999585997,-19.0845844257286,-0.472653097948809));
#44458=CARTESIAN_POINT('Ctrl Pts',(5.99999999148602,-18.9545321024225,-0.551743827842384));
#44459=CARTESIAN_POINT('Ctrl Pts',(5.99999999087342,-18.8227280871197,-0.627799835747431));
#44460=CARTESIAN_POINT('Ctrl Pts',(5.99999999026181,-18.6911389312267,-0.703731861473865));
#44461=CARTESIAN_POINT('Ctrl Pts',(5.99999999695614,-18.5578033768638,-0.77663926113671));
#44462=CARTESIAN_POINT('Ctrl Pts',(5.99999999953305,-18.4226147447749,-0.846524436286946));
#44463=CARTESIAN_POINT('Ctrl Pts',(5.99999999982096,-18.4075107787358,-0.85433236581324));
#44464=CARTESIAN_POINT('Ctrl Pts',(5.99999999999967,-18.3923836616462,-0.862102520704987));
#44465=CARTESIAN_POINT('Ctrl Pts',(5.99999999999967,-18.3772332302815,-0.869834866403388));
#44466=CARTESIAN_POINT('Ctrl Pts',(5.99999999999967,-18.3604562921101,-0.87839733453245));
#44467=CARTESIAN_POINT('Ctrl Pts',(5.99999999977963,-18.3436511842488,-0.886914343334167));
#44468=CARTESIAN_POINT('Ctrl Pts',(5.99999999940194,-18.32681838664,-0.895385513523014));
#44469=CARTESIAN_POINT('Ctrl Pts',(5.99999999572685,-18.1630285952216,-0.977813356508454));
#44470=CARTESIAN_POINT('Ctrl Pts',(5.99999998184218,-17.9966147415131,-1.05589757934824));
#44471=CARTESIAN_POINT('Ctrl Pts',(5.99999998033312,-17.8280085898849,-1.1293841227804));
#44472=CARTESIAN_POINT('Ctrl Pts',(5.99999997882264,-17.6592457266025,-1.20293896857085));
#44473=CARTESIAN_POINT('Ctrl Pts',(5.99999998731013,-17.4882868866805,-1.27188737333842));
#44474=CARTESIAN_POINT('Ctrl Pts',(5.99999999411993,-17.3155904515192,-1.33602010545033));
#44475=CARTESIAN_POINT('Ctrl Pts',(5.99999999739302,-17.2325847521993,-1.36684519036461));
#44476=CARTESIAN_POINT('Ctrl Pts',(5.99999999999966,-17.1491779727451,-1.39655845354114));
#44477=CARTESIAN_POINT('Ctrl Pts',(5.99999999999966,-17.0654226749711,-1.42514061332152));
#44478=CARTESIAN_POINT('Ctrl Pts',(5.99999999999966,-17.0325873369324,-1.43634593290379));
#44479=CARTESIAN_POINT('Ctrl Pts',(5.99999999960401,-16.9996980274663,-1.44737619951995));
#44480=CARTESIAN_POINT('Ctrl Pts',(5.99999999898846,-16.9667557482006,-1.45823114416469));
#44481=CARTESIAN_POINT('Ctrl Pts',(5.99999999507825,-16.757495451753,-1.527185356955));
#44482=CARTESIAN_POINT('Ctrl Pts',(5.99999998615646,-16.5460993317685,-1.5890690609484));
#44483=CARTESIAN_POINT('Ctrl Pts',(5.99999998771982,-16.332868561363,-1.64383881309663));
#44484=CARTESIAN_POINT('Ctrl Pts',(5.99999998928318,-16.1196377909574,-1.69860856524486));
#44485=CARTESIAN_POINT('Ctrl Pts',(5.99999999999966,-15.9045717674932,-1.74626453331427));
#44486=CARTESIAN_POINT('Ctrl Pts',(5.99999999999966,-15.68795707336,-1.78671132790344));
#44487=CARTESIAN_POINT('Ctrl Pts',(5.99999999999966,-15.6384076362316,-1.79596331292486));
#44488=CARTESIAN_POINT('Ctrl Pts',(5.9999999993466,-15.5887774796856,-1.80484067673141));
#44489=CARTESIAN_POINT('Ctrl Pts',(5.99999999845562,-15.5390744582055,-1.81334105408883));
#44490=CARTESIAN_POINT('Ctrl Pts',(5.99999999449748,-15.318269498527,-1.85110385851732));
#44491=CARTESIAN_POINT('Ctrl Pts',(5.99999998895124,-15.0960256116076,-1.88142252412455));
#44492=CARTESIAN_POINT('Ctrl Pts',(5.99999999115148,-14.8730323063916,-1.90421165291904));
#44493=CARTESIAN_POINT('Ctrl Pts',(5.99999999312717,-14.6727973227676,-1.92467496156659));
#44494=CARTESIAN_POINT('Ctrl Pts',(5.99999999999966,-14.4719585640787,-1.93906784227255));
#44495=CARTESIAN_POINT('Ctrl Pts',(5.99999999999966,-14.2710197611708,-1.94736399681091));
#44496=CARTESIAN_POINT('Ctrl Pts',(5.99999999999966,-14.2042169245834,-1.9501220835911));
#44497=CARTESIAN_POINT('Ctrl Pts',(5.99999999913623,-14.1374034485751,-1.95220396613166));
#44498=CARTESIAN_POINT('Ctrl Pts',(5.99999999780774,-14.0705875841289,-1.95360920069132));
#44499=CARTESIAN_POINT('Ctrl Pts',(5.99999999336888,-13.8473363769314,-1.95830449745114));
#44500=CARTESIAN_POINT('Ctrl Pts',(5.99999998477716,-13.6240582050389,-1.95544949150961));
#44501=CARTESIAN_POINT('Ctrl Pts',(5.99999998688347,-13.4010835092815,-1.94504172700609));
#44502=CARTESIAN_POINT('Ctrl Pts',(5.99999998862997,-13.2161992305184,-1.93641190456264));
#44503=CARTESIAN_POINT('Ctrl Pts',(5.99999999999966,-13.0315234335482,-1.92258841196678));
#44504=CARTESIAN_POINT('Ctrl Pts',(5.99999999999966,-12.8472489165034,-1.90354302704818));
#44505=CARTESIAN_POINT('Ctrl Pts',(5.99999999999966,-12.7639712033068,-1.89493599809809));
#44506=CARTESIAN_POINT('Ctrl Pts',(5.99999999683364,-12.6807722730351,-1.88527335009052));
#44507=CARTESIAN_POINT('Ctrl Pts',(5.99999999319098,-12.5976982773605,-1.87455629001131));
#44508=CARTESIAN_POINT('Ctrl Pts',(5.99999998466696,-12.4033004224575,-1.84947776244868));
#44509=CARTESIAN_POINT('Ctrl Pts',(5.99999997595983,-12.2095874450291,-1.81862158500248));
#44510=CARTESIAN_POINT('Ctrl Pts',(5.99999997954449,-12.0171122800012,-1.78211795983844));
#44511=CARTESIAN_POINT('Ctrl Pts',(5.99999998312914,-11.8246371149733,-1.7456143346744));
#44512=CARTESIAN_POINT('Ctrl Pts',(5.99999999999966,-11.6334002754345,-1.70346341636846));
#44513=CARTESIAN_POINT('Ctrl Pts',(5.99999999999966,-11.4439400773904,-1.65585042832456));
#44514=CARTESIAN_POINT('Ctrl Pts',(5.99999999999966,-11.3471401948288,-1.6315237797797));
#44515=CARTESIAN_POINT('Ctrl Pts',(5.99999999545176,-11.2508153992569,-1.60575152809878));
#44516=CARTESIAN_POINT('Ctrl Pts',(5.999999993073,-11.1549313534934,-1.5785357340368));
#44517=CARTESIAN_POINT('Ctrl Pts',(5.9999999894094,-11.0072572292376,-1.53661980816997));
#44518=CARTESIAN_POINT('Ctrl Pts',(5.9999999903115,-10.8606278293027,-1.49128219580575));
#44519=CARTESIAN_POINT('Ctrl Pts',(5.99999999276227,-10.7149545825572,-1.44250806010649));
#44520=CARTESIAN_POINT('Ctrl Pts',(5.99999999520009,-10.5700511250866,-1.39399166429694));
#44521=CARTESIAN_POINT('Ctrl Pts',(5.99999999786769,-10.4260933029596,-1.34207482786142));
#44522=CARTESIAN_POINT('Ctrl Pts',(5.99999999875682,-10.2830101379701,-1.28669419616467));
#44523=CARTESIAN_POINT('Ctrl Pts',(5.99999999915075,-10.2196170517512,-1.26215777246824));
#44524=CARTESIAN_POINT('Ctrl Pts',(5.99999999931868,-10.1563959085591,-1.23694079652416));
#44525=CARTESIAN_POINT('Ctrl Pts',(5.9999999993144,-10.09334190697,-1.2110347753893));
#44526=CARTESIAN_POINT('',(5.73644276520434,-19.8089520716699,-0.442549441855225));
#44527=CARTESIAN_POINT('Origin',(5.6,-19.5919343769637,-0.135488060672991));
#44528=CARTESIAN_POINT('Ctrl Pts',(5.73644276397732,-19.8089520717783,-0.442549442641763));
#44529=CARTESIAN_POINT('Ctrl Pts',(5.73708792252315,-19.4467189750557,-0.69823621872471));
#44530=CARTESIAN_POINT('Ctrl Pts',(5.7376256311114,-19.0680989321009,-0.930502816120376));
#44531=CARTESIAN_POINT('Ctrl Pts',(5.73805595543272,-18.6765903412666,-1.13733215216818));
#44532=CARTESIAN_POINT('Ctrl Pts',(5.73812189842541,-18.6165954795657,-1.16902672465618));
#44533=CARTESIAN_POINT('Ctrl Pts',(5.73818531973857,-18.556297873286,-1.20012401087123));
#44534=CARTESIAN_POINT('Ctrl Pts',(5.73824621957922,-18.4957100153502,-1.23061680204324));
#44535=CARTESIAN_POINT('Ctrl Pts',(5.73865147695443,-18.0925287259873,-1.43353077325557));
#44536=CARTESIAN_POINT('Ctrl Pts',(5.73894508021586,-17.6764985474971,-1.60967514468296));
#44537=CARTESIAN_POINT('Ctrl Pts',(5.73912707517464,-17.2512541404434,-1.75776137787843));
#44538=CARTESIAN_POINT('Ctrl Pts',(5.73915087505913,-17.1956439859834,-1.7771269431035));
#44539=CARTESIAN_POINT('Ctrl Pts',(5.73917276624537,-17.1398761856756,-1.79601269644437));
#44540=CARTESIAN_POINT('Ctrl Pts',(5.7391927487951,-17.0839588053956,-1.81441577480908));
#44541=CARTESIAN_POINT('Ctrl Pts',(5.73934700449672,-16.6523034438383,-1.95647871490941));
#44542=CARTESIAN_POINT('Ctrl Pts',(5.73938752580933,-16.2117387040006,-2.06977798720686));
#44543=CARTESIAN_POINT('Ctrl Pts',(5.7393143196508,-15.7661080919655,-2.15355053910136));
#44544=CARTESIAN_POINT('Ctrl Pts',(5.73930536900858,-15.7116225097048,-2.16379309458155));
#44545=CARTESIAN_POINT('Ctrl Pts',(5.73929471820266,-15.6570611342258,-2.17359426297402));
#44546=CARTESIAN_POINT('Ctrl Pts',(5.73928236720583,-15.6024309377374,-2.18295265701575));
#44547=CARTESIAN_POINT('Ctrl Pts',(5.73918135677838,-15.1556476072041,-2.25948861564609));
#44548=CARTESIAN_POINT('Ctrl Pts',(5.73896663207976,-14.7042654992233,-2.30640975727857));
#44549=CARTESIAN_POINT('Ctrl Pts',(5.73863815775707,-14.2522673186949,-2.32359669154592));
#44550=CARTESIAN_POINT('Ctrl Pts',(5.73859603594245,-14.1943054560695,-2.3258006533446));
#44551=CARTESIAN_POINT('Ctrl Pts',(5.73855204356702,-14.1363333925184,-2.32751565966289));
#44552=CARTESIAN_POINT('Ctrl Pts',(5.73850618051795,-14.0783594649322,-2.32874145708037));
#44553=CARTESIAN_POINT('Ctrl Pts',(5.73815298603535,-13.6318982772197,-2.33818140696285));
#44554=CARTESIAN_POINT('Ctrl Pts',(5.73768885011018,-13.1853304843906,-2.31860861075337));
#44555=CARTESIAN_POINT('Ctrl Pts',(5.73711370893976,-12.7423972722186,-2.27028161284945));
#44556=CARTESIAN_POINT('Ctrl Pts',(5.73703020877366,-12.6780913266681,-2.2632654009005));
#44557=CARTESIAN_POINT('Ctrl Pts',(5.73694436871282,-12.613861905765,-2.25564310254086));
#44558=CARTESIAN_POINT('Ctrl Pts',(5.73685618856742,-12.5497203746937,-2.24741549855154));
#44559=CARTESIAN_POINT('Ctrl Pts',(5.73622838727498,-12.0930627459389,-2.18883881562326));
#44560=CARTESIAN_POINT('Ctrl Pts',(5.73548197177282,-11.64086407108,-2.09958206443846));
#44561=CARTESIAN_POINT('Ctrl Pts',(5.73461687538872,-11.1970132530861,-1.98082802790191));
#44562=CARTESIAN_POINT('Ctrl Pts',(5.73452248333111,-11.1485839765889,-1.96787058400987));
#44563=CARTESIAN_POINT('Ctrl Pts',(5.73442667835076,-11.1002540362984,-1.95456194727603));
#44564=CARTESIAN_POINT('Ctrl Pts',(5.73432946037475,-11.0520284489647,-1.94090364135816));
#44565=CARTESIAN_POINT('Ctrl Pts',(5.73384874378987,-10.8135659690821,-1.87336701442942));
#44566=CARTESIAN_POINT('Ctrl Pts',(5.7333334786831,-10.5776553353801,-1.79728101389105));
#44567=CARTESIAN_POINT('Ctrl Pts',(5.7327836581836,-10.3449538542818,-1.71288850780721));
#44568=CARTESIAN_POINT('Ctrl Pts',(5.99999999997498,-19.5919300856734,0.135488304642552));
#44569=CARTESIAN_POINT('Ctrl Pts',(5.99999999997498,-19.5922326969623,0.0451632714407379));
#44570=CARTESIAN_POINT('Ctrl Pts',(5.99999999997498,-19.5922327064356,-0.0451632753777587));
#44571=CARTESIAN_POINT('Ctrl Pts',(5.99999999997498,-19.5919299350173,-0.135488872440526));
#44572=CARTESIAN_POINT('Ctrl Pts',(6.00000263487348,-19.829340627416,0.136284098535467));
#44573=CARTESIAN_POINT('Ctrl Pts',(6.00000263487349,-19.8296450131427,0.0454285037125645));
#44574=CARTESIAN_POINT('Ctrl Pts',(6.00000263487349,-19.8296450228323,-0.0454285076490772));
#44575=CARTESIAN_POINT('Ctrl Pts',(6.00000263487349,-19.8293404729368,-0.136284669416119));
#44576=CARTESIAN_POINT('Ctrl Pts',(5.83074066842648,-19.9958175555659,0.136842124817994));
#44577=CARTESIAN_POINT('Ctrl Pts',(5.8307406684265,-19.9961231855639,0.0456144897823355));
#44578=CARTESIAN_POINT('Ctrl Pts',(5.83074066842656,-19.9961231954074,-0.0456144937216663));
#44579=CARTESIAN_POINT('Ctrl Pts',(5.83074066842658,-19.9958173984086,-0.136842697865391));
#44580=CARTESIAN_POINT('Ctrl Pts',(5.59336110044015,-19.9918771871017,0.136828916806682));
#44581=CARTESIAN_POINT('Ctrl Pts',(5.59336110044031,-19.9921827876479,0.0456100876475798));
#44582=CARTESIAN_POINT('Ctrl Pts',(5.59336110044072,-19.9921827974882,-0.0456100915888983));
#44583=CARTESIAN_POINT('Ctrl Pts',(5.59336110044085,-19.9918770300065,-0.136829489802511));
#44584=CARTESIAN_POINT('',(5.99999999995608,-19.5919320087386,0.13548105287313));
#44585=CARTESIAN_POINT('',(5.59336167790261,-19.9918770519493,0.1368286131514));
#44586=CARTESIAN_POINT('Origin',(5.6,-19.5919343769583,0.135488060981343));
#44587=CARTESIAN_POINT('',(5.59336169562602,-19.9918770422853,-0.136828655448461));
#44588=CARTESIAN_POINT('Origin',(5.59336169592167,-15.0909939730293,-0.0604595362332659));
#44589=CARTESIAN_POINT('Origin',(5.6,-19.5919343771351,-0.13548806067611));
#44590=CARTESIAN_POINT('Ctrl Pts',(5.99999999999155,-19.5919320204748,0.13547755313224));
#44591=CARTESIAN_POINT('Ctrl Pts',(5.9999999999916,-19.592033064815,0.105317242942897));
#44592=CARTESIAN_POINT('Ctrl Pts',(5.99999999999962,-19.5921021554889,0.0751629221398726));
#44593=CARTESIAN_POINT('Ctrl Pts',(5.99999999999962,-19.5921363906274,0.0450478998554133));
#44594=CARTESIAN_POINT('Ctrl Pts',(5.99999999999962,-19.5921706257659,0.0149328775709451));
#44595=CARTESIAN_POINT('Ctrl Pts',(5.99999999999962,-19.592170005369,-0.0151428461949581));
#44596=CARTESIAN_POINT('Ctrl Pts',(5.99999999999962,-19.592136154094,-0.0452268828020266));
#44597=CARTESIAN_POINT('Ctrl Pts',(5.99999999999962,-19.5921023028189,-0.0753109194090861));
#44598=CARTESIAN_POINT('Ctrl Pts',(5.99999999999962,-19.5920352206656,-0.105403268857311));
#44599=CARTESIAN_POINT('Ctrl Pts',(5.99999999999962,-19.5919343770476,-0.135488060647564));
#44600=CARTESIAN_POINT('Origin',(5.6,-19.5919343769637,-0.135488060672991));
#44601=CARTESIAN_POINT('Origin',(5.600000004205,-19.5919343763234,-0.135488059062013));
#44602=CARTESIAN_POINT('Ctrl Pts',(-5.69266360647973,-19.9935541771414,
-0.0765565325209773));
#44603=CARTESIAN_POINT('Ctrl Pts',(-5.6578995530005,-19.9929007298199,-0.0929913866614558));
#44604=CARTESIAN_POINT('Ctrl Pts',(-5.54372467194083,-19.9908049362471,
-0.146471463308));
#44605=CARTESIAN_POINT('Ctrl Pts',(-5.34116840847122,-19.987350077468,-0.238479594457668));
#44606=CARTESIAN_POINT('Ctrl Pts',(-5.07576710978616,-19.983202471478,-0.353603245841893));
#44607=CARTESIAN_POINT('Ctrl Pts',(-4.78281267364433,-19.9789916798394,
-0.474026331255006));
#44608=CARTESIAN_POINT('Ctrl Pts',(-4.45929925449721,-19.9747248164902,
-0.598868153552744));
#44609=CARTESIAN_POINT('Ctrl Pts',(-4.10061014600622,-19.9704190336396,
-0.727254430583034));
#44610=CARTESIAN_POINT('Ctrl Pts',(-3.70134367776404,-19.9661195472229,
-0.857717930438492));
#44611=CARTESIAN_POINT('Ctrl Pts',(-3.25667261673587,-19.9619191732372,
-0.987522036063985));
#44612=CARTESIAN_POINT('Ctrl Pts',(-2.76260093160989,-19.9579588248915,
-1.11253953923502));
#44613=CARTESIAN_POINT('Ctrl Pts',(-2.21454168290653,-19.9544128020434,
-1.22755651364308));
#44614=CARTESIAN_POINT('Ctrl Pts',(-1.60546929114103,-19.9514859205532,
-1.32618245506953));
#44615=CARTESIAN_POINT('Ctrl Pts',(-0.938933076131297,-19.949459711508,
-1.39845731726721));
#44616=CARTESIAN_POINT('Ctrl Pts',(-0.23664535309699,-19.9485854307057,
-1.43362310534642));
#44617=CARTESIAN_POINT('Ctrl Pts',(0.4642466792577,-19.9487493934321,-1.4264266824266));
#44618=CARTESIAN_POINT('Ctrl Pts',(1.12888137961817,-19.9499401109169,-1.38089562429621));
#44619=CARTESIAN_POINT('Ctrl Pts',(1.73416986117937,-19.9520478855029,-1.3069947786214));
#44620=CARTESIAN_POINT('Ctrl Pts',(2.27382162043129,-19.9547877467897,-1.21535248098602));
#44621=CARTESIAN_POINT('Ctrl Pts',(2.75209716617804,-19.9579163581483,-1.11403336275034));
#44622=CARTESIAN_POINT('Ctrl Pts',(3.17956622801571,-19.9612850210495,-1.00747931862904));
#44623=CARTESIAN_POINT('Ctrl Pts',(3.56235593972046,-19.9647716235928,-0.8992296013094));
#44624=CARTESIAN_POINT('Ctrl Pts',(3.90389825972422,-19.9682668684595,-0.792406671009068));
#44625=CARTESIAN_POINT('Ctrl Pts',(4.20699235679262,-19.9716806547345,-0.689549337621442));
#44626=CARTESIAN_POINT('Ctrl Pts',(4.47553242579083,-19.9749594786553,-0.592113806854402));
#44627=CARTESIAN_POINT('Ctrl Pts',(4.71438132200868,-19.978087085808,-0.500492678804996));
#44628=CARTESIAN_POINT('Ctrl Pts',(4.92834984087647,-19.9810702155991,-0.41446474837091));
#44629=CARTESIAN_POINT('Ctrl Pts',(5.12118003508217,-19.983920132778,-0.333744232114557));
#44630=CARTESIAN_POINT('Ctrl Pts',(5.29544654744959,-19.9866446715028,-0.258197188744821));
#44631=CARTESIAN_POINT('Ctrl Pts',(5.45302073834614,-19.9892496568072,-0.18776958817749));
#44632=CARTESIAN_POINT('Ctrl Pts',(5.58355273456747,-19.9915337709002,-0.127837493099847));
#44633=CARTESIAN_POINT('Ctrl Pts',(5.66171486337773,-19.9929726011947,-0.0911864449715727));
#44634=CARTESIAN_POINT('Ctrl Pts',(5.692637247095,-19.9935542262535,-0.0765617004061338));
#44635=CARTESIAN_POINT('Ctrl Pts',(-5.75649789773431,-19.9991160246718,
-0.213743948047012));
#44636=CARTESIAN_POINT('Ctrl Pts',(-5.72140176446517,-19.9983763933301,
-0.230336779007504));
#44637=CARTESIAN_POINT('Ctrl Pts',(-5.6061363574476,-19.9959936786861,-0.284330788506753));
#44638=CARTESIAN_POINT('Ctrl Pts',(-5.40164108897797,-19.99200518302,-0.377224041508724));
#44639=CARTESIAN_POINT('Ctrl Pts',(-5.1336693786725,-19.9871042033416,-0.493465170018192));
#44640=CARTESIAN_POINT('Ctrl Pts',(-4.83782308796822,-19.982028337394,-0.615074766632991));
#44641=CARTESIAN_POINT('Ctrl Pts',(-4.51104023764979,-19.9767961134772,
-0.741169298308892));
#44642=CARTESIAN_POINT('Ctrl Pts',(-4.14862925030658,-19.9714345889302,
-0.870870253872186));
#44643=CARTESIAN_POINT('Ctrl Pts',(-3.7451010284537,-19.9660004924145,-1.00269864832984));
#44644=CARTESIAN_POINT('Ctrl Pts',(-3.29554242555684,-19.9606068553778,
-1.13389062270015));
#44645=CARTESIAN_POINT('Ctrl Pts',(-2.7958791388129,-19.9554270637761,-1.26027308336245));
#44646=CARTESIAN_POINT('Ctrl Pts',(-2.24144276789872,-19.9506811305415,
-1.37656929671114));
#44647=CARTESIAN_POINT('Ctrl Pts',(-1.6251068839532,-19.9466381361631,-1.47630757617145));
#44648=CARTESIAN_POINT('Ctrl Pts',(-0.950466599309452,-19.9437069324571,
-1.54940294776633));
#44649=CARTESIAN_POINT('Ctrl Pts',(-0.239549742799721,-19.9423158121451,
-1.58496415386577));
#44650=CARTESIAN_POINT('Ctrl Pts',(0.469949066288936,-19.9425954820282,
-1.57768764486034));
#44651=CARTESIAN_POINT('Ctrl Pts',(1.14273524885353,-19.9444157720885,-1.53164185334408));
#44652=CARTESIAN_POINT('Ctrl Pts',(1.7553509886388,-19.9474228366483,-1.4569028237362));
#44653=CARTESIAN_POINT('Ctrl Pts',(2.30141447279339,-19.9511844635576,-1.36422916038421));
#44654=CARTESIAN_POINT('Ctrl Pts',(2.78524782072098,-19.9553661337753,-1.26178440856533));
#44655=CARTESIAN_POINT('Ctrl Pts',(3.2175668220097,-19.9597796002856,-1.15406529307948));
#44656=CARTESIAN_POINT('Ctrl Pts',(3.60459389090943,-19.9642748189524,-1.04465245493347));
#44657=CARTESIAN_POINT('Ctrl Pts',(3.94982589636675,-19.9687199844506,-0.936702115595601));
#44658=CARTESIAN_POINT('Ctrl Pts',(4.25611894267221,-19.97300856616,-0.832778034999717));
#44659=CARTESIAN_POINT('Ctrl Pts',(4.52743270510596,-19.9770800474319,-0.734348454396371));
#44660=CARTESIAN_POINT('Ctrl Pts',(4.76870079203887,-19.9809191981262,-0.64180654650571));
#44661=CARTESIAN_POINT('Ctrl Pts',(4.98479925050148,-19.9845374733531,-0.554925572284122));
#44662=CARTESIAN_POINT('Ctrl Pts',(5.17952065874217,-19.9879503114012,-0.47341384725153));
#44663=CARTESIAN_POINT('Ctrl Pts',(5.35547601561356,-19.9911683754546,-0.39713317740571));
#44664=CARTESIAN_POINT('Ctrl Pts',(5.51456435191784,-19.9942009298587,-0.326026136389495));
#44665=CARTESIAN_POINT('Ctrl Pts',(5.64634486806084,-19.9968224547552,-0.265517744872236));
#44666=CARTESIAN_POINT('Ctrl Pts',(5.72525346105499,-19.9984580797953,-0.228514505250355));
#44667=CARTESIAN_POINT('Ctrl Pts',(5.75647083566732,-19.999118312624,-0.213749311958633));
#44668=CARTESIAN_POINT('Ctrl Pts',(-5.81361929054906,-19.9261291309016,
-0.33332743564323));
#44669=CARTESIAN_POINT('Ctrl Pts',(-5.77819666234262,-19.9253136755351,
-0.350029910484856));
#44670=CARTESIAN_POINT('Ctrl Pts',(-5.66186327713482,-19.9226787667006,
-0.404375005602182));
#44671=CARTESIAN_POINT('Ctrl Pts',(-5.45549017824741,-19.9182225720687,
-0.497841767049385));
#44672=CARTESIAN_POINT('Ctrl Pts',(-5.18505475622245,-19.9126637158777,
-0.614753500436186));
#44673=CARTESIAN_POINT('Ctrl Pts',(-4.88646290762062,-19.9068351818877,
-0.737031525938342));
#44674=CARTESIAN_POINT('Ctrl Pts',(-4.55660702641851,-19.9007662575288,
-0.863795521452588));
#44675=CARTESIAN_POINT('Ctrl Pts',(-4.19073575184427,-19.8944934655263,
-0.994167366746355));
#44676=CARTESIAN_POINT('Ctrl Pts',(-3.78329193486844,-19.8880843570324,
-1.12666201965898));
#44677=CARTESIAN_POINT('Ctrl Pts',(-3.32929912805282,-19.8816701335577,
-1.25850001195665));
#44678=CARTESIAN_POINT('Ctrl Pts',(-2.82462928254054,-19.8754524902486,
-1.38548279361662));
#44679=CARTESIAN_POINT('Ctrl Pts',(-2.26455890682294,-19.8696904124827,
-1.50230118360881));
#44680=CARTESIAN_POINT('Ctrl Pts',(-1.64189026826602,-19.8647068292226,
-1.60244613802217));
#44681=CARTESIAN_POINT('Ctrl Pts',(-0.960272299876233,-19.8610163311095,
-1.6757919689123));
#44682=CARTESIAN_POINT('Ctrl Pts',(-0.242005517629495,-19.8591930557594,
-1.71142835480064));
#44683=CARTESIAN_POINT('Ctrl Pts',(0.474779168951458,-19.85956938191,-1.70414269385846));
#44684=CARTESIAN_POINT('Ctrl Pts',(1.15453262843177,-19.8619165859985,-1.65797498745275));
#44685=CARTESIAN_POINT('Ctrl Pts',(1.77347554177536,-19.86567899107,-1.58296511398592));
#44686=CARTESIAN_POINT('Ctrl Pts',(2.32514101758377,-19.8703024011944,-1.48990602506843));
#44687=CARTESIAN_POINT('Ctrl Pts',(2.81388750100801,-19.8753761019103,-1.38699980286476));
#44688=CARTESIAN_POINT('Ctrl Pts',(3.25054379792609,-19.880678426273,-1.27877109361568));
#44689=CARTESIAN_POINT('Ctrl Pts',(3.64140302971636,-19.8860353147015,-1.1688235090255));
#44690=CARTESIAN_POINT('Ctrl Pts',(3.99000761186061,-19.8912952372146,-1.06033298708642));
#44691=CARTESIAN_POINT('Ctrl Pts',(4.29925370235094,-19.8963369129699,-0.955878719607947));
#44692=CARTESIAN_POINT('Ctrl Pts',(4.57315108204409,-19.9010930802668,-0.856937659179218));
#44693=CARTESIAN_POINT('Ctrl Pts',(4.81669094406161,-19.905548736309,-0.763905192229798));
#44694=CARTESIAN_POINT('Ctrl Pts',(5.03480427220289,-19.9097188605832,-0.676552771581171));
#44695=CARTESIAN_POINT('Ctrl Pts',(5.23132679680547,-19.9136220551603,-0.59458595913314));
#44696=CARTESIAN_POINT('Ctrl Pts',(5.40890088270857,-19.91727106624,-0.517864337069929));
#44697=CARTESIAN_POINT('Ctrl Pts',(5.56945003295899,-19.9206778466155,-0.446329088409351));
#44698=CARTESIAN_POINT('Ctrl Pts',(5.70244415132626,-19.9235953792304,-0.385439711430928));
#44699=CARTESIAN_POINT('Ctrl Pts',(5.7820841767363,-19.9254039957874,-0.348195793130167));
#44700=CARTESIAN_POINT('Ctrl Pts',(5.81359177736081,-19.9261333785129,-0.333334173054417));
#44701=CARTESIAN_POINT('Ctrl Pts',(-5.84786851513962,-19.7956125204352,
-0.401492745344046));
#44702=CARTESIAN_POINT('Ctrl Pts',(-5.81221747993369,-19.7947530449905,
-0.418225664741117));
#44703=CARTESIAN_POINT('Ctrl Pts',(-5.69514122740039,-19.791971991235,-0.472660196859671));
#44704=CARTESIAN_POINT('Ctrl Pts',(-5.48748337881077,-19.7872462977438,
-0.566227652874011));
#44705=CARTESIAN_POINT('Ctrl Pts',(-5.2153886925705,-19.781311093658,-0.68317497857044));
#44706=CARTESIAN_POINT('Ctrl Pts',(-4.91497503518046,-19.7750551206435,
-0.805416130630983));
#44707=CARTESIAN_POINT('Ctrl Pts',(-4.58311256625854,-19.7685147237548,
-0.932079108994651));
#44708=CARTESIAN_POINT('Ctrl Pts',(-4.21502210732507,-19.7617327707534,
-1.06229067382155));
#44709=CARTESIAN_POINT('Ctrl Pts',(-3.80511703616425,-19.7547838809892,
-1.19456711399924));
#44710=CARTESIAN_POINT('Ctrl Pts',(-3.34839805974144,-19.7478102400708,
-1.32612935869123));
#44711=CARTESIAN_POINT('Ctrl Pts',(-2.84072303534511,-19.7410296838559,
-1.4527809575621));
#44712=CARTESIAN_POINT('Ctrl Pts',(-2.27735525004778,-19.734722413695,-1.56921970799552));
#44713=CARTESIAN_POINT('Ctrl Pts',(-1.65107529416229,-19.7292395749277,
-1.6689534337654));
#44714=CARTESIAN_POINT('Ctrl Pts',(-0.965578662808645,-19.725150041307,
-1.74191112574034));
#44715=CARTESIAN_POINT('Ctrl Pts',(-0.243318637187852,-19.7231014047023,
-1.77728251315008));
#44716=CARTESIAN_POINT('Ctrl Pts',(0.477371881719029,-19.7235280256043,
-1.77006092556454));
#44717=CARTESIAN_POINT('Ctrl Pts',(1.16093897371515,-19.7261505983202,-1.72419699779472));
#44718=CARTESIAN_POINT('Ctrl Pts',(1.78342015357474,-19.7303109488223,-1.64955795707234));
#44719=CARTESIAN_POINT('Ctrl Pts',(2.33829376637848,-19.7353926172284,-1.55686585596026));
#44720=CARTESIAN_POINT('Ctrl Pts',(2.82991911146498,-19.740945210087,-1.45429027277005));
#44721=CARTESIAN_POINT('Ctrl Pts',(3.2691730799956,-19.7467292140027,-1.34634906850792));
#44722=CARTESIAN_POINT('Ctrl Pts',(3.66237499389563,-19.752557259858,-1.23664397669946));
#44723=CARTESIAN_POINT('Ctrl Pts',(4.01308062613083,-19.7582664543786,-1.12835107947497));
#44724=CARTESIAN_POINT('Ctrl Pts',(4.324198027549,-19.7637266189471,-1.02405114962652));
#44725=CARTESIAN_POINT('Ctrl Pts',(4.59975757565947,-19.7688659250237,-0.925224072311745));
#44726=CARTESIAN_POINT('Ctrl Pts',(4.84477861694369,-19.7736687391877,-0.832268454398782));
#44727=CARTESIAN_POINT('Ctrl Pts',(5.06422123234029,-19.7781513802583,-0.744958162908533));
#44728=CARTESIAN_POINT('Ctrl Pts',(5.26194473317568,-19.7823337120554,-0.662999920489588));
#44729=CARTESIAN_POINT('Ctrl Pts',(5.44060899256178,-19.7862292306473,-0.586253735975595));
#44730=CARTESIAN_POINT('Ctrl Pts',(5.60215186593309,-19.7898510677042,-0.514661792941206));
#44731=CARTESIAN_POINT('Ctrl Pts',(5.73598088940997,-19.7929394945044,-0.453693877884493));
#44732=CARTESIAN_POINT('Ctrl Pts',(5.81613009557532,-19.7948483759911,-0.416388525266093));
#44733=CARTESIAN_POINT('Ctrl Pts',(5.8478409291635,-19.79561789436,-0.401501639466543));
#44734=CARTESIAN_POINT('',(-5.593361696257,-19.9918770425327,-0.136828655009776));
#44735=CARTESIAN_POINT('Ctrl Pts',(-5.593361696257,-19.9918770425327,-0.136828655009776));
#44736=CARTESIAN_POINT('Ctrl Pts',(-5.53987020056264,-19.9909059753986,
-0.161652254976759));
#44737=CARTESIAN_POINT('Ctrl Pts',(-5.479349726203,-19.9898406677287,-0.189279917712342));
#44738=CARTESIAN_POINT('Ctrl Pts',(-5.37802554666591,-19.9881259346619,
-0.234797771553107));
#44739=CARTESIAN_POINT('Ctrl Pts',(-5.34249357548727,-19.9875348396451,
-0.250641374196676));
#44740=CARTESIAN_POINT('Ctrl Pts',(-5.2865597517199,-19.9866219206319,-0.275323558975893));
#44741=CARTESIAN_POINT('Ctrl Pts',(-5.25793387308637,-19.9861588948391,
-0.287893099482891));
#44742=CARTESIAN_POINT('Ctrl Pts',(-5.22831954432805,-19.985686638106,-0.300781885343407));
#44743=CARTESIAN_POINT('Ctrl Pts',(-5.20835700290589,-19.9853698241558,
-0.309442305333269));
#44744=CARTESIAN_POINT('Ctrl Pts',(-5.19631311251836,-19.9851797336765,
-0.314648127603555));
#44745=CARTESIAN_POINT('Ctrl Pts',(-5.12207990283231,-19.9840128909541,
-0.346642302652193));
#44746=CARTESIAN_POINT('Ctrl Pts',(-5.04939710257819,-19.9829026197028,
-0.377391298242854));
#44747=CARTESIAN_POINT('Ctrl Pts',(-4.93032631473058,-19.9811479246296,
-0.426585798090019));
#44748=CARTESIAN_POINT('Ctrl Pts',(-4.88896162087032,-19.9805481587181,
-0.443491790520733));
#44749=CARTESIAN_POINT('Ctrl Pts',(-4.8244029332133,-19.9796290973292,-0.469528375465107));
#44750=CARTESIAN_POINT('Ctrl Pts',(-4.79149567766814,-19.9791647189891,
-0.482715712402016));
#44751=CARTESIAN_POINT('Ctrl Pts',(-4.75200503402798,-19.9786151662145,
-0.498374697482097));
#44752=CARTESIAN_POINT('Ctrl Pts',(-4.73484500557417,-19.9783780583391,
-0.50514176176339));
#44753=CARTESIAN_POINT('Ctrl Pts',(-4.72335266062857,-19.9782196434084,
-0.509665304276756));
#44754=CARTESIAN_POINT('Ctrl Pts',(-4.71643686245319,-19.9781245780082,
-0.51238154988444));
#44755=CARTESIAN_POINT('Ctrl Pts',(-4.56282068320486,-19.9760172189209,
-0.572619677228507));
#44756=CARTESIAN_POINT('Ctrl Pts',(-4.38688909346539,-19.9737322566863,
-0.638684826646137));
#44757=CARTESIAN_POINT('Ctrl Pts',(-4.08253603951726,-19.9701218617751,
-0.744793257689181));
#44758=CARTESIAN_POINT('Ctrl Pts',(-3.97434240997806,-19.9688883655198,
-0.781293850177061));
#44759=CARTESIAN_POINT('Ctrl Pts',(-3.80193804833453,-19.9670227815378,
-0.836868705234022));
#44760=CARTESIAN_POINT('Ctrl Pts',(-3.71320738817908,-19.9660862577162,
-0.864859033956662));
#44761=CARTESIAN_POINT('Ctrl Pts',(-3.60526344583045,-19.964994870515,-0.89764772607499));
#44762=CARTESIAN_POINT('Ctrl Pts',(-3.55018526494765,-19.9644505593352,
-0.914045544112392));
#44763=CARTESIAN_POINT('Ctrl Pts',(-3.52634328534606,-19.9642176976363,
-0.921070682546635));
#44764=CARTESIAN_POINT('Ctrl Pts',(-3.51039595562554,-19.9640625620639,
-0.925753187407788));
#44765=CARTESIAN_POINT('Ctrl Pts',(-3.50119799341242,-19.9639734865516,
-0.928443254817963));
#44766=CARTESIAN_POINT('Ctrl Pts',(-3.27586137135579,-19.9617989531766,
-0.994142053109484));
#44767=CARTESIAN_POINT('Ctrl Pts',(-3.02941181863928,-19.9596442378471,
-1.06010677386181));
#44768=CARTESIAN_POINT('Ctrl Pts',(-2.61782551984484,-19.9566053802805,
-1.15486737579028));
#44769=CARTESIAN_POINT('Ctrl Pts',(-2.47364475862675,-19.9556253433564,
-1.18573178195283));
#44770=CARTESIAN_POINT('Ctrl Pts',(-2.24689562436969,-19.9542426642482,
-1.2297975138448));
#44771=CARTESIAN_POINT('Ctrl Pts',(-2.16956624754569,-19.9537963634296,
-1.244113003799));
#44772=CARTESIAN_POINT('Ctrl Pts',(-2.01141482975437,-19.9529394759166,
-1.27179246316136));
#44773=CARTESIAN_POINT('Ctrl Pts',(-1.93261264247602,-19.9525384232272,
-1.2848437335703));
#44774=CARTESIAN_POINT('Ctrl Pts',(-1.50967150883639,-19.9505433693017,
-1.35031376335494));
#44775=CARTESIAN_POINT('Ctrl Pts',(-1.15506197268932,-19.9493582218701,
-1.39106252074058));
#44776=CARTESIAN_POINT('Ctrl Pts',(-0.598762724615647,-19.9483492700185,
-1.42765146731114));
#44777=CARTESIAN_POINT('Ctrl Pts',(-0.409265484615582,-19.9481398188074,
-1.43576259964849));
#44778=CARTESIAN_POINT('Ctrl Pts',(-0.118923388652217,-19.9480099636445,
-1.44097617568032));
#44779=CARTESIAN_POINT('Ctrl Pts',(-0.0211266506705514,-19.9479967667065,
-1.44155574198219));
#44780=CARTESIAN_POINT('Ctrl Pts',(0.127092515292763,-19.9480204726378,
-1.44059056689962));
#44781=CARTESIAN_POINT('Ctrl Pts',(0.201583113022127,-19.948043564824,-1.43964942808039));
#44782=CARTESIAN_POINT('Ctrl Pts',(0.276645232873043,-19.9480847522935,
-1.43800298297456));
#44783=CARTESIAN_POINT('Ctrl Pts',(0.326813651022889,-19.9481163609107,
-1.43674672693249));
#44784=CARTESIAN_POINT('Ctrl Pts',(0.353716444626537,-19.9481356343534,
-1.43598444819588));
#44785=CARTESIAN_POINT('Ctrl Pts',(0.752470687267383,-19.9484522622495,
-1.42352583710267));
#44786=CARTESIAN_POINT('Ctrl Pts',(1.10888528711956,-19.94924020033,-1.39466314562183));
#44787=CARTESIAN_POINT('Ctrl Pts',(1.61518192059489,-19.9510623368019,-1.3331689588221));
#44788=CARTESIAN_POINT('Ctrl Pts',(1.86124892075682,-19.9521291255488,-1.29787744892242));
#44789=CARTESIAN_POINT('Ctrl Pts',(2.13593478360488,-19.9535986471434,-1.25040494578588));
#44790=CARTESIAN_POINT('Ctrl Pts',(2.25100180253815,-19.9542710478476,-1.2288842616072));
#44791=CARTESIAN_POINT('Ctrl Pts',(2.32712303877902,-19.954728184487,-1.21429513010396));
#44792=CARTESIAN_POINT('Ctrl Pts',(2.36664298291456,-19.9549722906808,-1.20652715275755));
#44793=CARTESIAN_POINT('Ctrl Pts',(2.68808813071481,-19.9570066067568,-1.14195559351965));
#44794=CARTESIAN_POINT('Ctrl Pts',(2.94934760456572,-19.9590245821492,-1.07929220022979));
#44795=CARTESIAN_POINT('Ctrl Pts',(3.30453249571811,-19.9621129152685,-0.984801908720499));
#44796=CARTESIAN_POINT('Ctrl Pts',(3.41681007283158,-19.9631531096153,-0.953206328513377));
#44797=CARTESIAN_POINT('Ctrl Pts',(3.57605035859579,-19.964703024329,-0.906426490572821));
#44798=CARTESIAN_POINT('Ctrl Pts',(3.6533764815014,-19.965475443408,-0.883188111121659));
#44799=CARTESIAN_POINT('Ctrl Pts',(3.73957575659907,-19.966366921966,-0.856488313231046));
#44800=CARTESIAN_POINT('Ctrl Pts',(3.77565804557831,-19.9667463830614,-0.845148104339534));
#44801=CARTESIAN_POINT('Ctrl Pts',(3.79952173656643,-19.9669987212599,-0.837612313145826));
#44802=CARTESIAN_POINT('Ctrl Pts',(3.80961452999613,-19.9671059351478,-0.834412391154652));
#44803=CARTESIAN_POINT('Ctrl Pts',(4.03884499603919,-19.9695563463032,-0.761336544705132));
#44804=CARTESIAN_POINT('Ctrl Pts',(4.23284563458667,-19.9718571567274,-0.69355479857008));
#44805=CARTESIAN_POINT('Ctrl Pts',(4.49122806875653,-19.9751161272079,-0.598760536622438));
#44806=CARTESIAN_POINT('Ctrl Pts',(4.5719191262046,-19.9761713988021,-0.568286225150129));
#44807=CARTESIAN_POINT('Ctrl Pts',(4.68480108146387,-19.9776910507615,-0.524711922251623));
#44808=CARTESIAN_POINT('Ctrl Pts',(4.73920340136529,-19.9784351075424,-0.50345661051287));
#44809=CARTESIAN_POINT('Ctrl Pts',(4.79910512355925,-19.9792722874665,-0.479661705607389));
#44810=CARTESIAN_POINT('Ctrl Pts',(4.82401279356573,-19.9796241229337,-0.469684812447406));
#44811=CARTESIAN_POINT('Ctrl Pts',(4.84044801875936,-19.9798570968037,-0.463083263109677));
#44812=CARTESIAN_POINT('Ctrl Pts',(4.84692845458122,-19.9799492057087,-0.460474746581707));
#44813=CARTESIAN_POINT('Ctrl Pts',(4.93422806898291,-19.9811954511744,-0.425211237863346));
#44814=CARTESIAN_POINT('Ctrl Pts',(5.00665608368955,-19.9822655538964,-0.395187232802343));
#44815=CARTESIAN_POINT('Ctrl Pts',(5.10754064194054,-19.9837976839523,-0.352644522552055));
#44816=CARTESIAN_POINT('Ctrl Pts',(5.15604355511379,-19.9845455683222,-0.331992751655454));
#44817=CARTESIAN_POINT('Ctrl Pts',(5.20923639673284,-19.9853831869685,-0.309054215570777));
#44818=CARTESIAN_POINT('Ctrl Pts',(5.2313060666232,-19.9857343668377,-0.299475845519313));
#44819=CARTESIAN_POINT('Ctrl Pts',(5.24585756605408,-19.9859667178632,-0.29314682790016));
#44820=CARTESIAN_POINT('Ctrl Pts',(5.251989654479,-19.9860649191825,-0.290474904973647));
#44821=CARTESIAN_POINT('Ctrl Pts',(5.39099848893191,-19.9883000550751,-0.229750246669846));
#44822=CARTESIAN_POINT('Ctrl Pts',(5.5020635061168,-19.9902196450197,-0.179197068989747));
#44823=CARTESIAN_POINT('Ctrl Pts',(5.593361696298,-19.9918770423739,-0.136828655184827));
#44824=CARTESIAN_POINT('',(-5.73644346265456,-19.808951158735,-0.442548130349197));
#44825=CARTESIAN_POINT('Origin',(-5.599999999997,-19.5919343769627,-0.135488060674723));
#44826=CARTESIAN_POINT('Ctrl Pts',(-5.73644387762025,-19.8089519016918,
-0.442549068003315));
#44827=CARTESIAN_POINT('Ctrl Pts',(-5.73644352459178,-19.8089518942983,
-0.442549230096899));
#44828=CARTESIAN_POINT('Ctrl Pts',(-5.73644317156308,-19.8089518869049,
-0.442549392190579));
#44829=CARTESIAN_POINT('Ctrl Pts',(-5.73644281853413,-19.8089518795114,
-0.442549554284354));
#44830=CARTESIAN_POINT('Ctrl Pts',(-5.67992322800445,-19.8077681932076,
-0.468500609840852));
#44831=CARTESIAN_POINT('Ctrl Pts',(-5.61717096311638,-19.8064997639747,
-0.496914357267869));
#44832=CARTESIAN_POINT('Ctrl Pts',(-5.54808344604347,-19.8051527722357,
-0.527556343709489));
#44833=CARTESIAN_POINT('Ctrl Pts',(-5.52951991964327,-19.8047908411986,
-0.535789717093907));
#44834=CARTESIAN_POINT('Ctrl Pts',(-5.51049891108683,-19.8044231966611,
-0.544183691954582));
#44835=CARTESIAN_POINT('Ctrl Pts',(-5.49101823034769,-19.8040498532496,
-0.552733116195771));
#44836=CARTESIAN_POINT('Ctrl Pts',(-5.42195695738163,-19.802726307548,-0.583041816858224));
#44837=CARTESIAN_POINT('Ctrl Pts',(-5.34711975453104,-19.8013309991599,
-0.615307999901524));
#44838=CARTESIAN_POINT('Ctrl Pts',(-5.26639707370599,-19.7998745194251,
-0.649265632063439));
#44839=CARTESIAN_POINT('Ctrl Pts',(-5.25084851317281,-19.7995939766694,
-0.655806449264208));
#44840=CARTESIAN_POINT('Ctrl Pts',(-5.23508154960726,-19.7993111671559,
-0.662409872904726));
#44841=CARTESIAN_POINT('Ctrl Pts',(-5.21909533754653,-19.7990261703001,
-0.669073785702921));
#44842=CARTESIAN_POINT('Ctrl Pts',(-5.19132318127546,-19.7985310575625,
-0.680650713802282));
#44843=CARTESIAN_POINT('Ctrl Pts',(-5.16288932753674,-19.7980293405181,
-0.692410241756752));
#44844=CARTESIAN_POINT('Ctrl Pts',(-5.13378929916158,-19.7975215543759,
-0.70434063927198));
#44845=CARTESIAN_POINT('Ctrl Pts',(-5.06602552723238,-19.7963390983355,
-0.732122355695892));
#44846=CARTESIAN_POINT('Ctrl Pts',(-4.99464964026495,-19.7951236537926,
-0.760832113190979));
#44847=CARTESIAN_POINT('Ctrl Pts',(-4.91960196679892,-19.7938827764332,
-0.790306636991108));
#44848=CARTESIAN_POINT('Ctrl Pts',(-4.82891093456434,-19.7923832436242,
-0.825924996156716));
#44849=CARTESIAN_POINT('Ctrl Pts',(-4.73285787622835,-19.7908464468696,
-0.862661733594464));
#44850=CARTESIAN_POINT('Ctrl Pts',(-4.63133263561869,-19.789288958625,-0.900183444709471));
#44851=CARTESIAN_POINT('Ctrl Pts',(-4.61738480421122,-19.789074986382,-0.905338285984501));
#44852=CARTESIAN_POINT('Ctrl Pts',(-4.60333368087305,-19.7888606286327,
-0.910507863030616));
#44853=CARTESIAN_POINT('Ctrl Pts',(-4.58917897112926,-19.7886459332474,
-0.91569123384208));
#44854=CARTESIAN_POINT('Ctrl Pts',(-4.5569989083199,-19.7881578334482,-0.927475382107651));
#44855=CARTESIAN_POINT('Ctrl Pts',(-4.52428345175846,-19.7876679863891,
-0.939330860040537));
#44856=CARTESIAN_POINT('Ctrl Pts',(-4.49102921787,-19.7871769688327,-0.951246233153467));
#44857=CARTESIAN_POINT('Ctrl Pts',(-4.45061974413422,-19.7865803001162,
-0.965725410706443));
#44858=CARTESIAN_POINT('Ctrl Pts',(-4.40941469472378,-19.7859819008893,
-0.980293065109979));
#44859=CARTESIAN_POINT('Ctrl Pts',(-4.36740795073453,-19.7853828769608,
-0.994927609811942));
#44860=CARTESIAN_POINT('Ctrl Pts',(-4.34640457873991,-19.7850833649966,
-1.00224488216292));
#44861=CARTESIAN_POINT('Ctrl Pts',(-4.3252007791973,-19.7847836891736,-1.00957886551706));
#44862=CARTESIAN_POINT('Ctrl Pts',(-4.30379578735247,-19.7844840053655,
-1.01692674026769));
#44863=CARTESIAN_POINT('Ctrl Pts',(-4.29309329143005,-19.7843341634614,
-1.02060067764301));
#44864=CARTESIAN_POINT('Ctrl Pts',(-4.28234049717896,-19.7841843190688,
-1.02427808712802));
#44865=CARTESIAN_POINT('Ctrl Pts',(-4.27153730830466,-19.7840344905978,
-1.02795861025227));
#44866=CARTESIAN_POINT('Ctrl Pts',(-4.26343491664894,-19.7839221192445,
-1.03071900259545));
#44867=CARTESIAN_POINT('Ctrl Pts',(-4.25530417799723,-19.7838097568063,
-1.03348114629917));
#44868=CARTESIAN_POINT('Ctrl Pts',(-4.24714505165301,-19.7836974110832,
-1.03624488840223));
#44869=CARTESIAN_POINT('Ctrl Pts',(-4.24442534287161,-19.7836599625088,
-1.03716613576992));
#44870=CARTESIAN_POINT('Ctrl Pts',(-4.24040571674569,-19.7836047034882,
-1.03852596299984));
#44871=CARTESIAN_POINT('Ctrl Pts',(-4.2389764612492,-19.7835850712593,-1.03900915753671));
#44872=CARTESIAN_POINT('Ctrl Pts',(-4.23363824302541,-19.7835117455856,
-1.0408138718713));
#44873=CARTESIAN_POINT('Ctrl Pts',(-4.22827574141502,-19.7834382142521,
-1.0426233946655));
#44874=CARTESIAN_POINT('Ctrl Pts',(-4.22288893010133,-19.7833644814854,
-1.04443764064879));
#44875=CARTESIAN_POINT('Ctrl Pts',(-4.14210743949879,-19.7822587730341,
-1.07164436579935));
#44876=CARTESIAN_POINT('Ctrl Pts',(-4.05585946314527,-19.7811075327797,
-1.09991742926328));
#44877=CARTESIAN_POINT('Ctrl Pts',(-3.96405509253658,-19.7799263357334,
-1.12894321402821));
#44878=CARTESIAN_POINT('Ctrl Pts',(-3.91582494302358,-19.7793057845574,
-1.14419213877616));
#44879=CARTESIAN_POINT('Ctrl Pts',(-3.86606114192558,-19.7786770117211,
-1.15964798280796));
#44880=CARTESIAN_POINT('Ctrl Pts',(-3.81475024023462,-19.7780426029928,
-1.17525948392769));
#44881=CARTESIAN_POINT('Ctrl Pts',(-3.7199189720691,-19.7768701078258,-1.20411219164403));
#44882=CARTESIAN_POINT('Ctrl Pts',(-3.61980308476554,-19.7756781932112,
-1.23349960388482));
#44883=CARTESIAN_POINT('Ctrl Pts',(-3.51432014675643,-19.7744851328542,
-1.26306109037886));
#44884=CARTESIAN_POINT('Ctrl Pts',(-3.46379574875574,-19.7739136787645,
-1.27722050172355));
#44885=CARTESIAN_POINT('Ctrl Pts',(-3.41204003840321,-19.7733420037037,
-1.29141910527109));
#44886=CARTESIAN_POINT('Ctrl Pts',(-3.35904414017396,-19.7727723575387,
-1.30561300663643));
#44887=CARTESIAN_POINT('Ctrl Pts',(-3.24837095335384,-19.7715827455394,
-1.33525462702593));
#44888=CARTESIAN_POINT('Ctrl Pts',(-3.13228852468873,-19.770401775826,-1.36487935655462));
#44889=CARTESIAN_POINT('Ctrl Pts',(-3.01072522401274,-19.7692520420384,
-1.39404936396976));
#44890=CARTESIAN_POINT('Ctrl Pts',(-2.96856990915526,-19.7688533412006,
-1.4041648415863));
#44891=CARTESIAN_POINT('Ctrl Pts',(-2.92501779804032,-19.7684516366423,
-1.41439774391956));
#44892=CARTESIAN_POINT('Ctrl Pts',(-2.88137003129703,-19.7680601552081,
-1.42441922738617));
#44893=CARTESIAN_POINT('Ctrl Pts',(-2.87181245808014,-19.7679744323235,
-1.42661363661076));
#44894=CARTESIAN_POINT('Ctrl Pts',(-2.86225034694103,-19.7678891900111,
-1.42879810081594));
#44895=CARTESIAN_POINT('Ctrl Pts',(-2.85269743997054,-19.7678045507344,
-1.43096949490122));
#44896=CARTESIAN_POINT('Ctrl Pts',(-2.83187074692257,-19.7676200250983,
-1.43570344219496));
#44897=CARTESIAN_POINT('Ctrl Pts',(-2.81108776110388,-19.7674383746355,
-1.44037508987938));
#44898=CARTESIAN_POINT('Ctrl Pts',(-2.79049137151887,-19.7672607679526,
-1.44495405126276));
#44899=CARTESIAN_POINT('Ctrl Pts',(-2.6196981206351,-19.7657879844525,-1.48292457503392));
#44900=CARTESIAN_POINT('Ctrl Pts',(-2.45356651026147,-19.7645069952526,
-1.51636436532049));
#44901=CARTESIAN_POINT('Ctrl Pts',(-2.29233862831246,-19.7633934519586,
-1.54579440365611));
#44902=CARTESIAN_POINT('Ctrl Pts',(-2.12998975108742,-19.7622721663513,
-1.57542906499829));
#44903=CARTESIAN_POINT('Ctrl Pts',(-1.97261303665365,-19.7613206253537,
-1.60099901719817));
#44904=CARTESIAN_POINT('Ctrl Pts',(-1.82041652058115,-19.7605131854738,
-1.62304689261556));
#44905=CARTESIAN_POINT('Ctrl Pts',(-1.76985268919714,-19.7602449319356,
-1.63037179783514));
#44906=CARTESIAN_POINT('Ctrl Pts',(-1.71986020171909,-19.7599925807726,
-1.63730784898285));
#44907=CARTESIAN_POINT('Ctrl Pts',(-1.67044548267176,-19.7597551865412,
-1.64387459616671));
#44908=CARTESIAN_POINT('Ctrl Pts',(-1.52120349901276,-19.7590382101689,
-1.66370743939237));
#44909=CARTESIAN_POINT('Ctrl Pts',(-1.37723517551391,-19.7584576260427,
-1.6801737259978));
#44910=CARTESIAN_POINT('Ctrl Pts',(-1.23869613188679,-19.757987037978,-1.69381367693242));
#44911=CARTESIAN_POINT('Ctrl Pts',(-1.14905168103962,-19.7576825345865,
-1.70263967918495));
#44912=CARTESIAN_POINT('Ctrl Pts',(-1.06167946637608,-19.7574240937746,
-1.71028177339375));
#44913=CARTESIAN_POINT('Ctrl Pts',(-0.976611993859875,-19.7572047093365,
-1.71687997626486));
#44914=CARTESIAN_POINT('Ctrl Pts',(-0.844717359987299,-19.756864560167,
-1.72711029728134));
#44915=CARTESIAN_POINT('Ctrl Pts',(-0.718364957082741,-19.7566182850543,
-1.73483337531946));
#44916=CARTESIAN_POINT('Ctrl Pts',(-0.597648913556363,-19.756441381481,
-1.74055570107211));
#44917=CARTESIAN_POINT('Ctrl Pts',(-0.48095024269112,-19.7562703651746,
-1.74608759053837));
#44918=CARTESIAN_POINT('Ctrl Pts',(-0.369518421291674,-19.7561641579339,
-1.74974956680164));
#44919=CARTESIAN_POINT('Ctrl Pts',(-0.263409266590326,-19.7561013445667,
-1.75196333668237));
#44920=CARTESIAN_POINT('Ctrl Pts',(-0.255798651790982,-19.756096839316,
-1.75212211798511));
#44921=CARTESIAN_POINT('Ctrl Pts',(-0.248215408177043,-19.7560925576963,
-1.75227343376927));
#44922=CARTESIAN_POINT('Ctrl Pts',(-0.240659551508548,-19.7560884920149,
-1.75241743246341));
#44923=CARTESIAN_POINT('Ctrl Pts',(-0.202148470861223,-19.7560677698397,
-1.75315137244754));
#44924=CARTESIAN_POINT('Ctrl Pts',(-0.164348875388144,-19.7560526530864,
-1.75369529114276));
#44925=CARTESIAN_POINT('Ctrl Pts',(-0.127262578344625,-19.7560420066296,
-1.75406887712268));
#44926=CARTESIAN_POINT('Ctrl Pts',(-0.105081272439121,-19.7560356389862,
-1.7542923188131));
#44927=CARTESIAN_POINT('Ctrl Pts',(-0.0831551352012425,-19.7560308625404,
-1.75445481924016));
#44928=CARTESIAN_POINT('Ctrl Pts',(-0.0614844746947158,-19.7560274564565,
-1.7545604529612));
#44929=CARTESIAN_POINT('Ctrl Pts',(-0.0416881516813964,-19.7560243449713,
-1.75465695021666));
#44930=CARTESIAN_POINT('Ctrl Pts',(-0.0231003093163219,-19.7560224629351,
-1.75470532598937));
#44931=CARTESIAN_POINT('Ctrl Pts',(-0.0029935776222741,-19.7560213813544,
-1.75471055955774));
#44932=CARTESIAN_POINT('Ctrl Pts',(-0.00108985029600973,-19.7560212789491,
-1.75471105507771));
#44933=CARTESIAN_POINT('Ctrl Pts',(0.000827493160234799,-19.7560211858688,
-1.75471112543437));
#44934=CARTESIAN_POINT('Ctrl Pts',(0.00276076763666115,-19.7560211031285,
-1.75471075018705));
#44935=CARTESIAN_POINT('Ctrl Pts',(0.115380441349963,-19.7560162832307,
-1.75468889078143));
#44936=CARTESIAN_POINT('Ctrl Pts',(0.233554088058695,-19.7560516460445,
-1.75316472129386));
#44937=CARTESIAN_POINT('Ctrl Pts',(0.35722758239336,-19.7561526828529,-1.74966567156876));
#44938=CARTESIAN_POINT('Ctrl Pts',(0.400683612468718,-19.7561881848706,
-1.74843618572859));
#44939=CARTESIAN_POINT('Ctrl Pts',(0.444818431363851,-19.756231813793,-1.74696248033964));
#44940=CARTESIAN_POINT('Ctrl Pts',(0.489628808892576,-19.756284734668,-1.74522279165275));
#44941=CARTESIAN_POINT('Ctrl Pts',(0.616894590528152,-19.7564350350423,
-1.74028190847459));
#44942=CARTESIAN_POINT('Ctrl Pts',(0.749612277410095,-19.7566602638825,
-1.73319794676817));
#44943=CARTESIAN_POINT('Ctrl Pts',(0.887682915219207,-19.756985291486,-1.72346286287803));
#44944=CARTESIAN_POINT('Ctrl Pts',(0.982201834953153,-19.7572077954047,
-1.71679852332389));
#44945=CARTESIAN_POINT('Ctrl Pts',(1.0792286314599,-19.7574770829128,-1.70889105456743));
#44946=CARTESIAN_POINT('Ctrl Pts',(1.1787205097217,-19.7578012083461,-1.69956860986377));
#44947=CARTESIAN_POINT('Ctrl Pts',(1.32351032467892,-19.7582729057581,-1.68600172312716));
#44948=CARTESIAN_POINT('Ctrl Pts',(1.47352295597801,-19.7588607225255,-1.66943864957755));
#44949=CARTESIAN_POINT('Ctrl Pts',(1.62859652258685,-19.7595906934866,-1.64934494633714));
#44950=CARTESIAN_POINT('Ctrl Pts',(1.68654895278824,-19.7598634904055,-1.64183574306032));
#44951=CARTESIAN_POINT('Ctrl Pts',(1.74520771954632,-19.7601561426315,-1.63383324635661));
#44952=CARTESIAN_POINT('Ctrl Pts',(1.80456261864638,-19.7604700126065,-1.62530885106478));
#44953=CARTESIAN_POINT('Ctrl Pts',(1.96229922867042,-19.7613041271716,-1.60265513189035));
#44954=CARTESIAN_POINT('Ctrl Pts',(2.12495580523365,-19.7622881347575,-1.57631599568825));
#44955=CARTESIAN_POINT('Ctrl Pts',(2.29231727829962,-19.7634467629545,-1.54576502076645));
#44956=CARTESIAN_POINT('Ctrl Pts',(2.31269526472841,-19.7635878378939,-1.54204512429961));
#44957=CARTESIAN_POINT('Ctrl Pts',(2.33314294078153,-19.7637315009022,-1.53826277673018));
#44958=CARTESIAN_POINT('Ctrl Pts',(2.3536598645813,-19.7638777958942,-1.53441702176428));
#44959=CARTESIAN_POINT('Ctrl Pts',(2.36243866162264,-19.7639403927072,-1.53277149718927));
#44960=CARTESIAN_POINT('Ctrl Pts',(2.37123013652142,-19.7640034713866,-1.53111436384921));
#44961=CARTESIAN_POINT('Ctrl Pts',(2.38003425591168,-19.7640670353362,-1.52944554910264));
#44962=CARTESIAN_POINT('Ctrl Pts',(2.44797134134356,-19.7645575272622,-1.5165681215051));
#44963=CARTESIAN_POINT('Ctrl Pts',(2.51666144909491,-19.7650769166499,-1.50299512176215));
#44964=CARTESIAN_POINT('Ctrl Pts',(2.58608847144018,-19.7656267527821,-1.48869322497577));
#44965=CARTESIAN_POINT('Ctrl Pts',(2.62080198261281,-19.7659016708482,-1.48154227658258));
#44966=CARTESIAN_POINT('Ctrl Pts',(2.65569972199575,-19.7661841992526,-1.47420910177566));
#44967=CARTESIAN_POINT('Ctrl Pts',(2.69077952007956,-19.7664745298379,-1.46668955142345));
#44968=CARTESIAN_POINT('Ctrl Pts',(2.70831941912146,-19.7666196951305,-1.46292977624734));
#44969=CARTESIAN_POINT('Ctrl Pts',(2.72590483281955,-19.7667668109062,-1.45912340708514));
#44970=CARTESIAN_POINT('Ctrl Pts',(2.74353548471427,-19.7669159007815,-1.45526992577017));
#44971=CARTESIAN_POINT('Ctrl Pts',(2.75886023000185,-19.7670454912457,-1.45192043988757));
#44972=CARTESIAN_POINT('Ctrl Pts',(2.7756378903939,-19.7671887562763,-1.44822069089754));
#44973=CARTESIAN_POINT('Ctrl Pts',(2.79016868314641,-19.7673139548209,-1.44499062909974));
#44974=CARTESIAN_POINT('Ctrl Pts',(2.79235512412055,-19.7673327933821,-1.4445046033485));
#44975=CARTESIAN_POINT('Ctrl Pts',(2.79449071570788,-19.7673512181178,-1.44402930676067));
#44976=CARTESIAN_POINT('Ctrl Pts',(2.79656287568912,-19.7673691161307,-1.44356762735337));
#44977=CARTESIAN_POINT('Ctrl Pts',(2.81155194714093,-19.7674985822905,-1.44022804658432));
#44978=CARTESIAN_POINT('Ctrl Pts',(2.82653495595638,-19.7676293154915,-1.43686280029191));
#44979=CARTESIAN_POINT('Ctrl Pts',(2.84151182044054,-19.7677613100067,-1.43347196866226));
#44980=CARTESIAN_POINT('Ctrl Pts',(2.98776197929538,-19.7690502459406,-1.40036025392311));
#44981=CARTESIAN_POINT('Ctrl Pts',(3.1334262372296,-19.7704594601723,-1.36480881552503));
#44982=CARTESIAN_POINT('Ctrl Pts',(3.27843755210209,-19.7719832405925,-1.32690025755523));
#44983=CARTESIAN_POINT('Ctrl Pts',(3.40982752551187,-19.7733638878136,-1.29255256249409));
#44984=CARTESIAN_POINT('Ctrl Pts',(3.54068146012917,-19.7748385888251,-1.25626977173964));
#44985=CARTESIAN_POINT('Ctrl Pts',(3.67095575809886,-19.7764027584285,-1.21811749018528));
#44986=CARTESIAN_POINT('Ctrl Pts',(3.78813027867816,-19.7778096424128,-1.18380162458624));
#44987=CARTESIAN_POINT('Ctrl Pts',(3.90483587261737,-19.7792889066611,-1.14797333960089));
#44988=CARTESIAN_POINT('Ctrl Pts',(4.02104510454438,-19.7808368957976,-1.11068244027831));
#44989=CARTESIAN_POINT('Ctrl Pts',(4.12468783511056,-19.7822174902506,-1.07742406168849));
#44990=CARTESIAN_POINT('Ctrl Pts',(4.22793574927265,-19.7836527500369,-1.04300229081));
#44991=CARTESIAN_POINT('Ctrl Pts',(4.33077217731849,-19.785139809244,-1.00745340168723));
#44992=CARTESIAN_POINT('Ctrl Pts',(4.42240217239439,-19.7864648185856,-0.975778395104719));
#44993=CARTESIAN_POINT('Ctrl Pts',(4.51370547672763,-19.787830953176,-0.943208537633732));
#44994=CARTESIAN_POINT('Ctrl Pts',(4.60467210497002,-19.7892359781879,-0.909769871237187));
#44995=CARTESIAN_POINT('Ctrl Pts',(4.68609298330715,-19.7904935643242,-0.879840152602627));
#44996=CARTESIAN_POINT('Ctrl Pts',(4.76724413735086,-19.7917823072661,-0.849214398468669));
#44997=CARTESIAN_POINT('Ctrl Pts',(4.84811962990798,-19.7931004999907,-0.817911356901049));
#44998=CARTESIAN_POINT('Ctrl Pts',(4.92104264859151,-19.7942890750416,-0.789686338259283));
#44999=CARTESIAN_POINT('Ctrl Pts',(4.9937415516435,-19.7955015932102,-0.760910679207981));
#45000=CARTESIAN_POINT('Ctrl Pts',(5.0662128614275,-19.7967368734856,-0.731597969779734));
#45001=CARTESIAN_POINT('Ctrl Pts',(5.13211260417619,-19.7978601407842,-0.704943283720578));
#45002=CARTESIAN_POINT('Ctrl Pts',(5.19782415727909,-19.7990022294067,-0.677844529277353));
#45003=CARTESIAN_POINT('Ctrl Pts',(5.26334554179462,-19.8001626395314,-0.650311508810309));
#45004=CARTESIAN_POINT('Ctrl Pts',(5.32292696860345,-19.8012178506114,-0.62527454330793));
#45005=CARTESIAN_POINT('Ctrl Pts',(5.38235114344313,-19.8022882117576,-0.59987848116738));
#45006=CARTESIAN_POINT('Ctrl Pts',(5.44161694959551,-19.8033743444023,-0.574129876715982));
#45007=CARTESIAN_POINT('Ctrl Pts',(5.495383784581,-19.8043597003516,-0.550770353636422));
#45008=CARTESIAN_POINT('Ctrl Pts',(5.54902027518269,-19.8053580364628,-0.527120674053056));
#45009=CARTESIAN_POINT('Ctrl Pts',(5.60252556055007,-19.8063718996398,-0.503184259300562));
#45010=CARTESIAN_POINT('Ctrl Pts',(5.64725681504635,-19.8072195050956,-0.483173042601675));
#45011=CARTESIAN_POINT('Ctrl Pts',(5.69189636725406,-19.8080779619371,-0.462961418909218));
#45012=CARTESIAN_POINT('Ctrl Pts',(5.73644276371317,-19.8089520713582,-0.442549442047294));
#45013=CARTESIAN_POINT('Ctrl Pts',(-5.843530256023,-19.9729833896359,-0.27559175820976));
#45014=CARTESIAN_POINT('Ctrl Pts',(-3.895686837349,-19.9313480702727,-1.19822011532892));
#45015=CARTESIAN_POINT('Ctrl Pts',(0.0001633689864733,-19.8897495499701,
-2.12096425758541));
#45016=CARTESIAN_POINT('Ctrl Pts',(3.896013575322,-19.9313515592134,-1.19814272318624));
#45017=CARTESIAN_POINT('Ctrl Pts',(5.844020362983,-19.9729938661567,-0.275359601183318));
#45018=CARTESIAN_POINT('Ctrl Pts',(-5.843530256023,-19.2592936008182,-0.803935998277621));
#45019=CARTESIAN_POINT('Ctrl Pts',(-3.895686837349,-19.2409365935521,-1.65690450594922));
#45020=CARTESIAN_POINT('Ctrl Pts',(0.0001633689864733,-19.2238044947448,
-2.51235948357542));
#45021=CARTESIAN_POINT('Ctrl Pts',(3.896013575322,-19.2409380304522,-1.65683275746512));
#45022=CARTESIAN_POINT('Ctrl Pts',(5.844020362983,-19.2592982199189,-0.803721369480543));
#45023=CARTESIAN_POINT('Ctrl Pts',(-5.843530256023,-17.6858136333434,-1.6793983649399));
#45024=CARTESIAN_POINT('Ctrl Pts',(-3.895686837349,-17.747795448815,-2.42360806358736));
#45025=CARTESIAN_POINT('Ctrl Pts',(0.0001633689864733,-17.809230949477,
-3.16660341450187));
#45026=CARTESIAN_POINT('Ctrl Pts',(3.896013575322,-17.7477902961142,-2.4235457472868));
#45027=CARTESIAN_POINT('Ctrl Pts',(5.844020362983,-17.6857980371155,-1.67921110261911));
#45028=CARTESIAN_POINT('Ctrl Pts',(-5.843530256023,-15.0614254644282,-2.34071387947306));
#45029=CARTESIAN_POINT('Ctrl Pts',(-3.895686837349,-15.2991206306984,-3.03320174206706));
#45030=CARTESIAN_POINT('Ctrl Pts',(0.0001633689864732,-15.5368877409607,
-3.72636654307133));
#45031=CARTESIAN_POINT('Ctrl Pts',(3.896013575322,-15.2991006887591,-3.03314360513899));
#45032=CARTESIAN_POINT('Ctrl Pts',(5.844020362983,-15.0613656542058,-2.34053963171711));
#45033=CARTESIAN_POINT('Ctrl Pts',(-5.843530256023,-12.4568668146763,-2.30089092035602));
#45034=CARTESIAN_POINT('Ctrl Pts',(-3.895686837349,-12.8710914025805,-3.06727952800882));
#45035=CARTESIAN_POINT('Ctrl Pts',(0.0001633689864735,-13.2856266664931,
-3.83244208505026));
#45036=CARTESIAN_POINT('Ctrl Pts',(3.896013575322,-12.8710566347918,-3.06721535250531));
#45037=CARTESIAN_POINT('Ctrl Pts',(5.844020362983,-12.4567625851234,-2.30069807725729));
#45038=CARTESIAN_POINT('Ctrl Pts',(-5.843530256023,-10.8186332244494,-1.86224588936189));
#45039=CARTESIAN_POINT('Ctrl Pts',(-3.895686837349,-11.3231463541034,-2.74792371556351));
#45040=CARTESIAN_POINT('Ctrl Pts',(0.0001633689864728,-11.8270563158389,
-3.6358578364456));
#45041=CARTESIAN_POINT('Ctrl Pts',(3.896013575322,-11.3231040903104,-2.74784924300041));
#45042=CARTESIAN_POINT('Ctrl Pts',(5.844020362983,-10.8185062759584,-1.86202303005818));
#45043=CARTESIAN_POINT('Ctrl Pts',(-5.843530256023,-10.0864076157968,-1.57296479340504));
#45044=CARTESIAN_POINT('Ctrl Pts',(-3.895686837349,-10.6220745328126,-2.52887436203661));
#45045=CARTESIAN_POINT('Ctrl Pts',(0.0001633689864728,-11.1575431674059,
-3.48561319739018));
#45046=CARTESIAN_POINT('Ctrl Pts',(3.896013575322,-10.6220296221396,-2.52879411870404));
#45047=CARTESIAN_POINT('Ctrl Pts',(5.844020362983,-10.0862728282186,-1.57272426197469));
#45048=CARTESIAN_POINT('',(-5.73278762856495,-10.3449531567002,-1.71289048058869));
#45049=CARTESIAN_POINT('Ctrl Pts',(-5.73644356953966,-19.8089503607358,
-0.442546999711169));
#45050=CARTESIAN_POINT('Ctrl Pts',(-5.73766037023715,-19.13018257123,-0.921733298671357));
#45051=CARTESIAN_POINT('Ctrl Pts',(-5.73849618481613,-18.393846050701,-1.31839021829628));
#45052=CARTESIAN_POINT('Ctrl Pts',(-5.73940756699886,-16.8491829909953,
-1.92343296233218));
#45053=CARTESIAN_POINT('Ctrl Pts',(-5.73948313453522,-16.0408992766055,
-2.13191056314112));
#45054=CARTESIAN_POINT('Ctrl Pts',(-5.73887402245753,-14.4000963331593,
-2.35028699763758));
#45055=CARTESIAN_POINT('Ctrl Pts',(-5.73818934284347,-13.5675419989661,
-2.35984313733086));
#45056=CARTESIAN_POINT('Ctrl Pts',(-5.73605973646493,-11.9265541666401,
-2.1816928390157));
#45057=CARTESIAN_POINT('Ctrl Pts',(-5.73461480970045,-11.1182366089558,
-1.99332811374448));
#45058=CARTESIAN_POINT('Ctrl Pts',(-5.732787734897,-10.344953053782,-1.71289076302532));
#45059=CARTESIAN_POINT('Ctrl Pts',(5.73278688084627,-10.3449507251019,-1.71289711530792));
#45060=CARTESIAN_POINT('Ctrl Pts',(5.37888843777514,-10.4448706571245,-1.88173932877861));
#45061=CARTESIAN_POINT('Ctrl Pts',(5.01595919747795,-10.5336950032638,-2.03742942677716));
#45062=CARTESIAN_POINT('Ctrl Pts',(4.64561269144281,-10.6118287908983,-2.1782223594122));
#45063=CARTESIAN_POINT('Ctrl Pts',(4.37133529018088,-10.6696944163975,-2.28249314109879));
#45064=CARTESIAN_POINT('Ctrl Pts',(4.09298964122314,-10.7216962259158,-2.37858913369378));
#45065=CARTESIAN_POINT('Ctrl Pts',(3.81123116921486,-10.7680223059877,-2.46581531638881));
#45066=CARTESIAN_POINT('Ctrl Pts',(3.57206776142054,-10.8073450035477,-2.53985501057632));
#45067=CARTESIAN_POINT('Ctrl Pts',(3.33044540604648,-10.8425781621285,-2.60750319913259));
#45068=CARTESIAN_POINT('Ctrl Pts',(3.08676494767327,-10.8738590874902,-2.6683687069462));
#45069=CARTESIAN_POINT('Ctrl Pts',(3.04336539559371,-10.8794302283129,-2.67920886948463));
#45070=CARTESIAN_POINT('Ctrl Pts',(2.99990056110183,-10.8848760740909,-2.68983400144025));
#45071=CARTESIAN_POINT('Ctrl Pts',(2.95637270868366,-10.8901974957882,-2.70024205336848));
#45072=CARTESIAN_POINT('Ctrl Pts',(2.75799589931633,-10.9144497067053,-2.74767642052765));
#45073=CARTESIAN_POINT('Ctrl Pts',(2.55830648556141,-10.9361785450978,-2.79061684543243));
#45074=CARTESIAN_POINT('Ctrl Pts',(2.35757129153615,-10.9553635756561,-2.82884755089333));
#45075=CARTESIAN_POINT('Ctrl Pts',(2.16366743985199,-10.9738957086884,-2.86577720379982));
#45076=CARTESIAN_POINT('Ctrl Pts',(1.96878777590427,-10.9900542072394,-2.89831218497539));
#45077=CARTESIAN_POINT('Ctrl Pts',(1.77317279899638,-11.0038443119457,-2.92629994189379));
#45078=CARTESIAN_POINT('Ctrl Pts',(1.58064315056598,-11.0174169128421,-2.95384626316751));
#45079=CARTESIAN_POINT('Ctrl Pts',(1.38740120163293,-11.0286951687085,-2.97698752542344));
#45080=CARTESIAN_POINT('Ctrl Pts',(1.19367625025074,-11.0377081848305,-2.99562128171204));
#45081=CARTESIAN_POINT('Ctrl Pts',(0.99541937006976,-11.0469320480686,-3.01469094910115));
#45082=CARTESIAN_POINT('Ctrl Pts',(0.796656624754899,-11.0537832045303,
-3.02903930284969));
#45083=CARTESIAN_POINT('Ctrl Pts',(0.597633784091129,-11.058320922494,-3.03860683125552));
#45084=CARTESIAN_POINT('Ctrl Pts',(0.408899185061013,-11.0626240686934,
-3.04767977801561));
#45085=CARTESIAN_POINT('Ctrl Pts',(0.219930686263253,-11.0648468971938,
-3.05245361771812));
#45086=CARTESIAN_POINT('Ctrl Pts',(0.0309378795019422,-11.0650651874903,
-3.05292291655167));
#45087=CARTESIAN_POINT('Ctrl Pts',(0.0206355625289282,-11.0650770868629,
-3.0529484988234));
#45088=CARTESIAN_POINT('Ctrl Pts',(0.010333173324214,-11.0650830359869,
-3.05296130133743));
#45089=CARTESIAN_POINT('Ctrl Pts',(3.07458380650083E-5,-11.0650830493252,
-3.05296132714325));
#45090=CARTESIAN_POINT('Ctrl Pts',(2.04972257753908E-5,-11.0650830493385,
-3.05296132716893));
#45091=CARTESIAN_POINT('Ctrl Pts',(1.02486135232418E-5,-11.0650830493459,
-3.05296132718195));
#45092=CARTESIAN_POINT('Ctrl Pts',(1.30820925200369E-12,-11.0650830493474,
-3.05296132718234));
#45093=CARTESIAN_POINT('Ctrl Pts',(-0.189346238011998,-11.0650830774452,
-3.05296133427582));
#45094=CARTESIAN_POINT('Ctrl Pts',(-0.378679741028174,-11.0630759761256,
-3.04864178284235));
#45095=CARTESIAN_POINT('Ctrl Pts',(-0.56778974481848,-11.0589841641667,
-3.04000565563741));
#45096=CARTESIAN_POINT('Ctrl Pts',(-0.769206894826438,-11.0546260599597,
-3.0308074953399));
#45097=CARTESIAN_POINT('Ctrl Pts',(-0.970370508673635,-11.0479028812665,
-3.01671229737493));
#45098=CARTESIAN_POINT('Ctrl Pts',(-1.17102593691553,-11.0387518606635,
-2.99777927914873));
#45099=CARTESIAN_POINT('Ctrl Pts',(-1.36677015451404,-11.0298248189988,
-2.97930966249326));
#45100=CARTESIAN_POINT('Ctrl Pts',(-1.56203075861168,-11.0185875790368,
-2.95623660831183));
#45101=CARTESIAN_POINT('Ctrl Pts',(-1.75657134412065,-11.0050092503527,
-2.9286641524004));
#45102=CARTESIAN_POINT('Ctrl Pts',(-1.95843344700961,-10.9909199024939,
-2.90005400959892));
#45103=CARTESIAN_POINT('Ctrl Pts',(-2.15952031581612,-10.9743099252187,
-2.86659942061579));
#45104=CARTESIAN_POINT('Ctrl Pts',(-2.35956783707536,-10.95517321442,-2.82846728755689));
#45105=CARTESIAN_POINT('Ctrl Pts',(-2.55961535833459,-10.9360365036213,
-2.79033515449799));
#45106=CARTESIAN_POINT('Ctrl Pts',(-2.75862353204654,-10.9143732358628,
-2.74752581297736));
#45107=CARTESIAN_POINT('Ctrl Pts',(-2.95632824474637,-10.8902036689342,
-2.70025289298462));
#45108=CARTESIAN_POINT('Ctrl Pts',(-3.19895907619652,-10.8605418463119,
-2.64223774642446));
#45109=CARTESIAN_POINT('Ctrl Pts',(-3.4396322657691,-10.8270117264881,-2.57747376778623));
#45110=CARTESIAN_POINT('Ctrl Pts',(-3.67795557690252,-10.7894741500217,
-2.50633569808409));
#45111=CARTESIAN_POINT('Ctrl Pts',(-3.96305364831295,-10.7445692239988,
-2.42123564480148));
#45112=CARTESIAN_POINT('Ctrl Pts',(-4.24478892074166,-10.6939295124197,
-2.32701475039204));
#45113=CARTESIAN_POINT('Ctrl Pts',(-4.52248991688278,-10.6373573471668,
-2.22437826455121));
#45114=CARTESIAN_POINT('Ctrl Pts',(-4.88935807875883,-10.5626203942278,
-2.08878617296681));
#45115=CARTESIAN_POINT('Ctrl Pts',(-5.24918529793651,-10.4775301564684,
-1.93851281801485));
#45116=CARTESIAN_POINT('Ctrl Pts',(-5.60042336716264,-10.3816929767705,
-1.77523602709409));
#45117=CARTESIAN_POINT('Ctrl Pts',(-5.64468291353218,-10.3696165235885,
-1.7546615013465));
#45118=CARTESIAN_POINT('Ctrl Pts',(-5.68880607668191,-10.3573694769593,
-1.73388045298063));
#45119=CARTESIAN_POINT('Ctrl Pts',(-5.73278975886993,-10.3449510884867,
-1.71289616972921));
#45120=CARTESIAN_POINT('Ctrl Pts',(5.84410998923895,-10.3323727011903,-1.66672064035875));
#45121=CARTESIAN_POINT('Ctrl Pts',(5.36057054894098,-10.479094582877,-1.90463347330094));
#45122=CARTESIAN_POINT('Ctrl Pts',(4.31408846255943,-10.7396037440786,-2.34942232840999));
#45123=CARTESIAN_POINT('Ctrl Pts',(2.64209705711627,-10.9963179139186,-2.82821487492597));
#45124=CARTESIAN_POINT('Ctrl Pts',(0.886920055989066,-11.1223996222838,
-3.07899637167777));
#45125=CARTESIAN_POINT('Ctrl Pts',(-0.875886341835384,-11.1227843119789,
-3.07977938393283));
#45126=CARTESIAN_POINT('Ctrl Pts',(-2.63119909167307,-10.9975191925275,
-2.83055183922051));
#45127=CARTESIAN_POINT('Ctrl Pts',(-4.30720311490177,-10.741126078388,-2.35211597616156));
#45128=CARTESIAN_POINT('Ctrl Pts',(-5.35738264311282,-10.4800665124644,
-1.90620695928531));
#45129=CARTESIAN_POINT('Ctrl Pts',(-5.8442271457114,-10.3323372091642,-1.66666302689571));
#45130=CARTESIAN_POINT('Ctrl Pts',(5.72541417918007,-10.0514442779705,-1.59501843129042));
#45131=CARTESIAN_POINT('Ctrl Pts',(5.25159834165599,-10.1957394661812,-1.82634278489692));
#45132=CARTESIAN_POINT('Ctrl Pts',(4.2261913450166,-10.4520386787258,-2.25899782340991));
#45133=CARTESIAN_POINT('Ctrl Pts',(2.58809547397256,-10.7047345563918,-2.72492011022138));
#45134=CARTESIAN_POINT('Ctrl Pts',(0.868755502373261,-10.8288843404259,
-2.96899426302417));
#45135=CARTESIAN_POINT('Ctrl Pts',(-0.857947639815771,-10.8292631798881,
-2.96975634944105));
#45136=CARTESIAN_POINT('Ctrl Pts',(-2.57741930712446,-10.705917294703,-2.72719450177864));
#45137=CARTESIAN_POINT('Ctrl Pts',(-4.21944479726212,-10.453536763772,-2.26161858227183));
#45138=CARTESIAN_POINT('Ctrl Pts',(-5.24847453496336,-10.1966953253984,
-1.82787271391779));
#45139=CARTESIAN_POINT('Ctrl Pts',(-5.72552897853899,-10.0514093727704,
-1.59496241647954));
#45140=CARTESIAN_POINT('Ctrl Pts',(5.71947389187913,-9.77852708496778,-1.74874490072951));
#45141=CARTESIAN_POINT('Ctrl Pts',(5.2470321869844,-9.921413239911,-1.97762113018203));
#45142=CARTESIAN_POINT('Ctrl Pts',(4.22431639454507,-10.1753945595949,-2.4060661741839));
#45143=CARTESIAN_POINT('Ctrl Pts',(2.5884933514872,-10.426209475828,-2.86836631045969));
#45144=CARTESIAN_POINT('Ctrl Pts',(0.869223760158633,-10.5496122855385,
-3.11097295137889));
#45145=CARTESIAN_POINT('Ctrl Pts',(-0.858411199827123,-10.5499890570998,
-3.11173099225105));
#45146=CARTESIAN_POINT('Ctrl Pts',(-2.57782411118657,-10.4273844882945,
-2.87062553047234));
#45147=CARTESIAN_POINT('Ctrl Pts',(-4.21758631945515,-10.1768799198358,
-2.40866315092365));
#45148=CARTESIAN_POINT('Ctrl Pts',(-5.24391750487453,-9.92235978674762,
-1.97913477439047));
#45149=CARTESIAN_POINT('Ctrl Pts',(-5.71958836908387,-9.77849251905957,
-1.74868947153473));
#45150=CARTESIAN_POINT('Ctrl Pts',(5.83013871823063,-9.69045696047479,-2.02829469174308));
#45151=CARTESIAN_POINT('Ctrl Pts',(5.34983126658624,-9.83386472624641,-2.26044942827995));
#45152=CARTESIAN_POINT('Ctrl Pts',(4.30967893787492,-10.0889220899972,-2.69533619417949));
#45153=CARTESIAN_POINT('Ctrl Pts',(2.64303317634597,-10.3412121496862,-3.16560929890304));
#45154=CARTESIAN_POINT('Ctrl Pts',(0.888021522624684,-10.4655369409606,
-3.41293915743986));
#45155=CARTESIAN_POINT('Ctrl Pts',(-0.876976757826566,-10.4659167668583,
-3.41371265444607));
#45156=CARTESIAN_POINT('Ctrl Pts',(-2.63215150136536,-10.3423952567662,
-3.16791057917455));
#45157=CARTESIAN_POINT('Ctrl Pts',(-4.30283233414894,-10.0904144949512,
-2.69797390537513));
#45158=CARTESIAN_POINT('Ctrl Pts',(-5.34666482197009,-9.83481475265889,
-2.26198461166413));
#45159=CARTESIAN_POINT('Ctrl Pts',(-5.8302551169916,-9.6904222664813,-2.02823845567536));
#45160=CARTESIAN_POINT('',(-5.72001850098467,-9.72697711277114,-2.05943260735066));
#45161=CARTESIAN_POINT('Origin',(-5.89877516387283,-10.1838115204741,-2.15616245823881));
#45162=CARTESIAN_POINT('Ctrl Pts',(5.72001565651808,-9.72697714714131,-2.05943442901332));
#45163=CARTESIAN_POINT('Ctrl Pts',(5.52235085864605,-9.7844910448374,-2.15308157960336));
#45164=CARTESIAN_POINT('Ctrl Pts',(5.32001672263882,-9.83893941594344,-2.2434991590881));
#45165=CARTESIAN_POINT('Ctrl Pts',(5.11307319479122,-9.89023368154803,-2.33012652189619));
#45166=CARTESIAN_POINT('Ctrl Pts',(4.91024846415452,-9.94050703734063,-2.41502974022856));
#45167=CARTESIAN_POINT('Ctrl Pts',(4.70299587527167,-9.98775055604259,-2.49629215637547));
#45168=CARTESIAN_POINT('Ctrl Pts',(4.49139522432464,-10.0318777162878,-2.57334139085351));
#45169=CARTESIAN_POINT('Ctrl Pts',(4.46219526166272,-10.0379670710501,-2.58397384760551));
#45170=CARTESIAN_POINT('Ctrl Pts',(4.43291253856575,-10.0439970772018,-2.59452600233919));
#45171=CARTESIAN_POINT('Ctrl Pts',(4.40354730271865,-10.0499675032233,-2.60499628183089));
#45172=CARTESIAN_POINT('Ctrl Pts',(4.37976748661062,-10.0548023233356,-2.61347506000958));
#45173=CARTESIAN_POINT('Ctrl Pts',(4.35593367343142,-10.0595979810214,-2.62190037307499));
#45174=CARTESIAN_POINT('Ctrl Pts',(4.332045973406,-10.0643543153132,-2.63027154851775));
#45175=CARTESIAN_POINT('Ctrl Pts',(4.12525023380215,-10.1055298854443,-2.70274078646022));
#45176=CARTESIAN_POINT('Ctrl Pts',(3.91441507757712,-10.1437589609266,-2.77115658712805));
#45177=CARTESIAN_POINT('Ctrl Pts',(3.69967486042235,-10.1789388853645,-2.83506100053878));
#45178=CARTESIAN_POINT('Ctrl Pts',(3.57990205462159,-10.1985607257148,-2.87070411852882));
#45179=CARTESIAN_POINT('Ctrl Pts',(3.45891509144413,-10.2172332521504,-2.9049447655403));
#45180=CARTESIAN_POINT('Ctrl Pts',(3.33674283377924,-10.2349335320187,-2.93770859495658));
#45181=CARTESIAN_POINT('Ctrl Pts',(3.27565670494679,-10.2437836719529,-2.95409050966471));
#45182=CARTESIAN_POINT('Ctrl Pts',(3.21427424700828,-10.2523907260036,-2.97010321289942));
#45183=CARTESIAN_POINT('Ctrl Pts',(3.15259957222235,-10.2607514410604,-2.98573783030413));
#45184=CARTESIAN_POINT('Ctrl Pts',(3.11638891678785,-10.2656602139588,-2.99491728273994));
#45185=CARTESIAN_POINT('Ctrl Pts',(3.07933300787028,-10.2705825379318,-3.00415159974981));
#45186=CARTESIAN_POINT('Ctrl Pts',(3.04274299872612,-10.2753423983666,-3.01310965170823));
#45187=CARTESIAN_POINT('Ctrl Pts',(3.01701221065459,-10.2786896224576,-3.01940912366429));
#45188=CARTESIAN_POINT('Ctrl Pts',(2.99151215360445,-10.2819570769124,-3.02557289989933));
#45189=CARTESIAN_POINT('Ctrl Pts',(2.96670303692837,-10.2850912093338,-3.0314985776476));
#45190=CARTESIAN_POINT('Ctrl Pts',(2.85030963482703,-10.2997951723937,-3.05929923665065));
#45191=CARTESIAN_POINT('Ctrl Pts',(2.73340197420777,-10.3135879903048,-3.08554917027159));
#45192=CARTESIAN_POINT('Ctrl Pts',(2.61601284445959,-10.3264799707405,-3.11020526841202));
#45193=CARTESIAN_POINT('Ctrl Pts',(2.35525340215346,-10.3551172528793,-3.1649744826854));
#45194=CARTESIAN_POINT('Ctrl Pts',(2.09211887583113,-10.3793110921927,-3.21188228216435));
#45195=CARTESIAN_POINT('Ctrl Pts',(1.8270977264198,-10.3991227910425,-3.25060580697337));
#45196=CARTESIAN_POINT('Ctrl Pts',(1.56723131899066,-10.4185491463224,-3.28857614744417));
#45197=CARTESIAN_POINT('Ctrl Pts',(1.30555044492713,-10.4337620611484,-3.31867769380861));
#45198=CARTESIAN_POINT('Ctrl Pts',(1.04251007652366,-10.4447978734305,-3.34056109478048));
#45199=CARTESIAN_POINT('Ctrl Pts',(0.985615250304729,-10.4471848858339,
-3.34529440740063));
#45200=CARTESIAN_POINT('Ctrl Pts',(0.928656816677235,-10.4493763974219,
-3.34964306254167));
#45201=CARTESIAN_POINT('Ctrl Pts',(0.871639381436839,-10.4513726478619,
-3.35360322592787));
#45202=CARTESIAN_POINT('Ctrl Pts',(0.606372392652728,-10.4606599709564,
-3.37202742568577));
#45203=CARTESIAN_POINT('Ctrl Pts',(0.339827581630843,-10.4657227545967,
-3.38204643130129));
#45204=CARTESIAN_POINT('Ctrl Pts',(0.0725412991722131,-10.4664986079721,
-3.38358403303145));
#45205=CARTESIAN_POINT('Ctrl Pts',(0.0484382047896898,-10.4665685721579,
-3.38372268945363));
#45206=CARTESIAN_POINT('Ctrl Pts',(0.0243290882578963,-10.4666036600148,
-3.38379234520509));
#45207=CARTESIAN_POINT('Ctrl Pts',(0.000214347814518571,-10.4666038166003,
-3.38379292606275));
#45208=CARTESIAN_POINT('Ctrl Pts',(-0.260553342450019,-10.4666055098569,
-3.38379920723792));
#45209=CARTESIAN_POINT('Ctrl Pts',(-0.520633949551103,-10.4625144980462,
-3.3757628994388));
#45210=CARTESIAN_POINT('Ctrl Pts',(-0.779551934798321,-10.4544007225929,
-3.35973491714526));
#45211=CARTESIAN_POINT('Ctrl Pts',(-0.806643725132065,-10.4535517406144,
-3.35805783497827));
#45212=CARTESIAN_POINT('Ctrl Pts',(-0.833722790373814,-10.452658694736,
-3.35629321491924));
#45213=CARTESIAN_POINT('Ctrl Pts',(-0.860788587592884,-10.4517216503606,
-3.35444108617536));
#45214=CARTESIAN_POINT('Ctrl Pts',(-1.07488422032283,-10.4443094501276,
-3.33979039356473));
#45215=CARTESIAN_POINT('Ctrl Pts',(-1.28814982980102,-10.434145049339,-3.31966611688754));
#45216=CARTESIAN_POINT('Ctrl Pts',(-1.50035118319147,-10.4212166860301,
-3.29424753095549));
#45217=CARTESIAN_POINT('Ctrl Pts',(-1.74805547483542,-10.4061253069018,
-3.26457621773205));
#45218=CARTESIAN_POINT('Ctrl Pts',(-1.99429862023719,-10.3872816790159,
-3.22765205927763));
#45219=CARTESIAN_POINT('Ctrl Pts',(-2.238704824599,-10.3646346324663,-3.18377136192204));
#45220=CARTESIAN_POINT('Ctrl Pts',(-2.36090792677991,-10.3533111091916,
-3.16183101324425));
#45221=CARTESIAN_POINT('Ctrl Pts',(-2.48265212251779,-10.3410357106285,
-3.13815307827137));
#45222=CARTESIAN_POINT('Ctrl Pts',(-2.60389237049849,-10.3277960057427,
-3.11278377543351));
#45223=CARTESIAN_POINT('Ctrl Pts',(-2.60428195105617,-10.3277534626788,
-3.1127022564057));
#45224=CARTESIAN_POINT('Ctrl Pts',(-2.60467152641047,-10.3277109096566,
-3.11262071991405));
#45225=CARTESIAN_POINT('Ctrl Pts',(-2.6050610965595,-10.3276683466758,-3.11253916595973));
#45226=CARTESIAN_POINT('Ctrl Pts',(-2.66529003077652,-10.3210879580644,
-3.09993063380649));
#45227=CARTESIAN_POINT('Ctrl Pts',(-2.72539454793682,-10.3142695391852,
-3.08690471014164));
#45228=CARTESIAN_POINT('Ctrl Pts',(-2.7853693764555,-10.3072116618264,-3.07346790953369));
#45229=CARTESIAN_POINT('Ctrl Pts',(-2.82091266841363,-10.3030289037967,
-3.06550476668215));
#45230=CARTESIAN_POINT('Ctrl Pts',(-2.85565628250159,-10.2988530195494,
-3.05757010167284));
#45231=CARTESIAN_POINT('Ctrl Pts',(-2.89093226624542,-10.2945248100442,
-3.04936312181237));
#45232=CARTESIAN_POINT('Ctrl Pts',(-2.91556507117471,-10.2915024722065,
-3.04363228421391));
#45233=CARTESIAN_POINT('Ctrl Pts',(-2.94045720811709,-10.2884053612001,
-3.03776780035864));
#45234=CARTESIAN_POINT('Ctrl Pts',(-2.96605816588864,-10.2851718529285,
-3.03165480338706));
#45235=CARTESIAN_POINT('Ctrl Pts',(-3.20039906137285,-10.2555736156018,
-2.97569888184707));
#45236=CARTESIAN_POINT('Ctrl Pts',(-3.43065223281089,-10.2224787982665,
-2.91412948280924));
#45237=CARTESIAN_POINT('Ctrl Pts',(-3.65662486529341,-10.1860042939441,
-2.84757563479633));
#45238=CARTESIAN_POINT('Ctrl Pts',(-3.88259749777593,-10.1495297896217,
-2.78102178678342));
#45239=CARTESIAN_POINT('Ctrl Pts',(-4.10428974370387,-10.1096756491821,
-2.70948313380135));
#45240=CARTESIAN_POINT('Ctrl Pts',(-4.32153106765576,-10.0665548789947,
-2.63353231928838));
#45241=CARTESIAN_POINT('Ctrl Pts',(-4.53975694790682,-10.0232386817811,
-2.55723728917454));
#45242=CARTESIAN_POINT('Ctrl Pts',(-4.75349214138674,-9.97662627109529,
-2.47648978122073));
#45243=CARTESIAN_POINT('Ctrl Pts',(-4.96264794993634,-9.92683360298108,
-2.39182310253517));
#45244=CARTESIAN_POINT('Ctrl Pts',(-5.1769245871331,-9.8758218450263,-2.30508350243911));
#45245=CARTESIAN_POINT('Ctrl Pts',(-5.38639491591567,-9.82147223720818,
-2.21423036493514));
#45246=CARTESIAN_POINT('Ctrl Pts',(-5.59097678902522,-9.76390332624704,
-2.11978463387151));
#45247=CARTESIAN_POINT('Ctrl Pts',(-5.63420911728029,-9.75173783954908,
-2.09982632189806));
#45248=CARTESIAN_POINT('Ctrl Pts',(-5.67722318912536,-9.73942856815475,
-2.0797073988229));
#45249=CARTESIAN_POINT('Ctrl Pts',(-5.72001829824668,-9.72697659463366,
-2.05943249764344));
#45250=CARTESIAN_POINT('Ctrl Pts',(-5.71222662189986,-10.3742949004598,
-1.73071937901633));
#45251=CARTESIAN_POINT('Ctrl Pts',(-5.71815984095385,-10.3724589996086,
-1.7282869964701));
#45252=CARTESIAN_POINT('Ctrl Pts',(-5.76567964049473,-10.3578830041957,
-1.70774113544913));
#45253=CARTESIAN_POINT('Ctrl Pts',(-5.85049323787678,-10.3338145218821,
-1.65484483353384));
#45254=CARTESIAN_POINT('Ctrl Pts',(-5.948215668862,-10.3109877388706,-1.55199932393069));
#45255=CARTESIAN_POINT('Ctrl Pts',(-6.01635745652966,-10.3007577513163,
-1.43124311968169));
#45256=CARTESIAN_POINT('Ctrl Pts',(-6.04741510867493,-10.3028711449483,
-1.31838657229349));
#45257=CARTESIAN_POINT('Ctrl Pts',(-6.0513323381477,-10.309530687115,-1.25061757017122));
#45258=CARTESIAN_POINT('Ctrl Pts',(-6.05059138821606,-10.3129418468683,
-1.22449919891673));
#45259=CARTESIAN_POINT('Ctrl Pts',(-5.59627044501229,-10.0908844432555,
-1.65483230450451));
#45260=CARTESIAN_POINT('Ctrl Pts',(-5.60180878284993,-10.0891580404173,
-1.65259441346381));
#45261=CARTESIAN_POINT('Ctrl Pts',(-5.64617398194355,-10.0754418826971,
-1.63369069961307));
#45262=CARTESIAN_POINT('Ctrl Pts',(-5.72546143917485,-10.0526570805557,
-1.58500246675733));
#45263=CARTESIAN_POINT('Ctrl Pts',(-5.81681904905107,-10.0308016578564,
-1.49039287045747));
#45264=CARTESIAN_POINT('Ctrl Pts',(-5.88036941811923,-10.0207355017336,
-1.37963866786923));
#45265=CARTESIAN_POINT('Ctrl Pts',(-5.90916535585768,-10.0223138650847,
-1.27675997058527));
#45266=CARTESIAN_POINT('Ctrl Pts',(-5.91275807104277,-10.0282885033146,
-1.21550396072571));
#45267=CARTESIAN_POINT('Ctrl Pts',(-5.91207749740188,-10.0313688521514,
-1.19199294725519));
#45268=CARTESIAN_POINT('Ctrl Pts',(-5.57929439471514,-9.81899473911404,
-1.81393819386833));
#45269=CARTESIAN_POINT('Ctrl Pts',(-5.58716647012282,-9.81658670486357,
-1.81078351792171));
#45270=CARTESIAN_POINT('Ctrl Pts',(-5.6501538878883,-9.79750079182511,-1.78417128597669));
#45271=CARTESIAN_POINT('Ctrl Pts',(-5.76178553763288,-9.76641565551527,
-1.71622516352867));
#45272=CARTESIAN_POINT('Ctrl Pts',(-5.89038954782538,-9.73728669160811,
-1.58467249327706));
#45273=CARTESIAN_POINT('Ctrl Pts',(-5.98122469506971,-9.72430629345384,
-1.42882521019155));
#45274=CARTESIAN_POINT('Ctrl Pts',(-6.02390479158533,-9.72723646949882,
-1.27974174396812));
#45275=CARTESIAN_POINT('Ctrl Pts',(-6.02958496996387,-9.73632704949079,
-1.18718217071838));
#45276=CARTESIAN_POINT('Ctrl Pts',(-6.02851816949953,-9.7410542982751,-1.15093231856939));
#45277=CARTESIAN_POINT('Ctrl Pts',(-5.67241100352444,-9.73660671891414,
-2.10388493024505));
#45278=CARTESIAN_POINT('Ctrl Pts',(-5.68381775092394,-9.73317212551118,
-2.09930232818442));
#45279=CARTESIAN_POINT('Ctrl Pts',(-5.77501394452402,-9.70600195136843,
-2.06067697444542));
#45280=CARTESIAN_POINT('Ctrl Pts',(-5.93568733722006,-9.66246593541034,
-1.96261338233826));
#45281=CARTESIAN_POINT('Ctrl Pts',(-6.12076716020052,-9.62257985011687,
-1.77312190199155));
#45282=CARTESIAN_POINT('Ctrl Pts',(-6.25290243570567,-9.60551482359818,
-1.54660477105814));
#45283=CARTESIAN_POINT('Ctrl Pts',(-6.31652387643652,-9.61079874693495,
-1.32537995208573));
#45284=CARTESIAN_POINT('Ctrl Pts',(-6.32533702444869,-9.62476639236188,
-1.18419183869603));
#45285=CARTESIAN_POINT('Ctrl Pts',(-6.32369022138811,-9.63204017725459,
-1.12819590352899));
#45286=CARTESIAN_POINT('',(-5.99998760030264,-10.0933467246824,-1.2110347037336));
#45287=CARTESIAN_POINT('',(-5.99999999751865,-9.65438795558276,-1.86247663369286));
#45288=CARTESIAN_POINT('Ctrl Pts',(-5.99998760030264,-10.0933467246824,
-1.2110347037336));
#45289=CARTESIAN_POINT('Ctrl Pts',(-5.99998607316774,-10.0742396970364,
-1.22560749002239));
#45290=CARTESIAN_POINT('Ctrl Pts',(-5.99998812583008,-10.0554931562148,
-1.24050908229297));
#45291=CARTESIAN_POINT('Ctrl Pts',(-6.00000075483295,-10.0372227691589,
-1.25574669535911));
#45292=CARTESIAN_POINT('Ctrl Pts',(-6.0000066757416,-10.0286569865797,-1.26289060972449));
#45293=CARTESIAN_POINT('Ctrl Pts',(-6.00001433938093,-10.0201958451556,
-1.27010784300164));
#45294=CARTESIAN_POINT('Ctrl Pts',(-6.00002217201098,-10.0118507476806,
-1.27739604002589));
#45295=CARTESIAN_POINT('Ctrl Pts',(-6.00003978018608,-9.99309051815821,
-1.29378030029239));
#45296=CARTESIAN_POINT('Ctrl Pts',(-6.00006006509509,-9.97491795491863,
-1.31052619883873));
#45297=CARTESIAN_POINT('Ctrl Pts',(-6.00008124713978,-9.95743900268535,
-1.32757773999911));
#45298=CARTESIAN_POINT('Ctrl Pts',(-6.0000957515782,-9.94547026264922,-1.33925380963076));
#45299=CARTESIAN_POINT('Ctrl Pts',(-6.00010993220736,-9.93382646569235,
-1.35107215192216));
#45300=CARTESIAN_POINT('Ctrl Pts',(-6.00011973283796,-9.92253515906925,
-1.36300284494533));
#45301=CARTESIAN_POINT('Ctrl Pts',(-6.00013439162104,-9.90564677491764,
-1.38084755802381));
#45302=CARTESIAN_POINT('Ctrl Pts',(-6.0001381190075,-9.88954895530081,-1.3989450314351));
#45303=CARTESIAN_POINT('Ctrl Pts',(-6.00012272533991,-9.87430471235906,
-1.41716232741016));
#45304=CARTESIAN_POINT('Ctrl Pts',(-6.00011846686318,-9.87008757219817,
-1.42220192765615));
#45305=CARTESIAN_POINT('Ctrl Pts',(-6.00011283313294,-9.86593553105825,
-1.42725050321475));
#45306=CARTESIAN_POINT('Ctrl Pts',(-6.00010589287417,-9.86184939866626,
-1.4323048409796));
#45307=CARTESIAN_POINT('Ctrl Pts',(-6.00010021774545,-9.85850812162791,
-1.43643783058878));
#45308=CARTESIAN_POINT('Ctrl Pts',(-6.00009367301605,-9.85521090958835,
-1.44057467085351));
#45309=CARTESIAN_POINT('Ctrl Pts',(-6.00008646895637,-9.85195805011668,
-1.44471365554858));
#45310=CARTESIAN_POINT('Ctrl Pts',(-6.00006816383533,-9.84369271237293,
-1.45523058894793));
#45311=CARTESIAN_POINT('Ctrl Pts',(-6.00005083454579,-9.83559537668922,
-1.46590386806272));
#45312=CARTESIAN_POINT('Ctrl Pts',(-6.00003062833731,-9.82781143086467,
-1.47654974030866));
#45313=CARTESIAN_POINT('Ctrl Pts',(-6.00001023986008,-9.81995727047922,
-1.48729164293069));
#45314=CARTESIAN_POINT('Ctrl Pts',(-5.99998647027655,-9.81242254560712,
-1.49800526520946));
#45315=CARTESIAN_POINT('Ctrl Pts',(-5.99996841664569,-9.80532177884617,
-1.5084628178353));
#45316=CARTESIAN_POINT('Ctrl Pts',(-5.9999575812154,-9.80106003981939,-1.51473923299587));
#45317=CARTESIAN_POINT('Ctrl Pts',(-5.99994910272377,-9.79695390267551,
-1.52092267040456));
#45318=CARTESIAN_POINT('Ctrl Pts',(-5.99994799710813,-9.79302171041628,
-1.52695840218962));
#45319=CARTESIAN_POINT('Ctrl Pts',(-5.99994410063521,-9.77916365692028,
-1.54822986819403));
#45320=CARTESIAN_POINT('Ctrl Pts',(-5.99996403848016,-9.76602534233863,
-1.57001276505637));
#45321=CARTESIAN_POINT('Ctrl Pts',(-5.99998999688529,-9.75374482436451,
-1.59221790778169));
#45322=CARTESIAN_POINT('Ctrl Pts',(-6.00001580522397,-9.74153530049751,
-1.61429468179451));
#45323=CARTESIAN_POINT('Ctrl Pts',(-6.00004684830186,-9.73017447649929,
-1.63678831739194));
#45324=CARTESIAN_POINT('Ctrl Pts',(-6.00006726238211,-9.71976949444447,
-1.65956840215017));
#45325=CARTESIAN_POINT('Ctrl Pts',(-6.00006992719727,-9.71841124789831,
-1.6625420710408));
#45326=CARTESIAN_POINT('Ctrl Pts',(-6.00007242162838,-9.71706923986762,
-1.66552056836441));
#45327=CARTESIAN_POINT('Ctrl Pts',(-6.00007472171134,-9.71574366257339,
-1.66850355851029));
#45328=CARTESIAN_POINT('Ctrl Pts',(-6.00009235696659,-9.70558016221269,
-1.69137481736148));
#45329=CARTESIAN_POINT('Ctrl Pts',(-6.00009751347439,-9.69638600040425,
-1.71451258302224));
#45330=CARTESIAN_POINT('Ctrl Pts',(-6.00008872575521,-9.68822341677773,
-1.73775334468263));
#45331=CARTESIAN_POINT('Ctrl Pts',(-6.00007982866157,-9.67995923929784,
-1.76128336751823));
#45332=CARTESIAN_POINT('Ctrl Pts',(-6.0000562406674,-9.67275278597893,-1.78491795340221));
#45333=CARTESIAN_POINT('Ctrl Pts',(-6.00003365310932,-9.66662223367053,
-1.80846626086191));
#45334=CARTESIAN_POINT('Ctrl Pts',(-6.00001630640013,-9.66191411481669,
-1.82655080280035));
#45335=CARTESIAN_POINT('Ctrl Pts',(-5.99999991734079,-9.6578395448413,-1.84458389836406));
#45336=CARTESIAN_POINT('Ctrl Pts',(-5.99999992038511,-9.65438777104218,
-1.86247659809221));
#45337=CARTESIAN_POINT('Ctrl Pts',(-5.72001867922522,-9.72697756829748,
-2.0594327038003));
#45338=CARTESIAN_POINT('Ctrl Pts',(-5.77222801794758,-9.71178780265897,
-2.03468832666118));
#45339=CARTESIAN_POINT('Ctrl Pts',(-5.82158476387888,-9.69822399312625,
-2.00571488891083));
#45340=CARTESIAN_POINT('Ctrl Pts',(-5.86823437671508,-9.68614875469511,
-1.97285223877799));
#45341=CARTESIAN_POINT('Ctrl Pts',(-5.91488398955128,-9.67407351626397,
-1.93998958864516));
#45342=CARTESIAN_POINT('Ctrl Pts',(-5.95882664449167,-9.6634872700105,-1.90323780725514));
#45343=CARTESIAN_POINT('Ctrl Pts',(-6.00000007205025,-9.65438813918026,
-1.8624766691116));
#45344=CARTESIAN_POINT('Ctrl Pts',(-5.73278528549769,-10.3449554307779,
-1.71288422662173));
#45345=CARTESIAN_POINT('Ctrl Pts',(-5.74758703926587,-10.3336956641858,
-1.70324286602081));
#45346=CARTESIAN_POINT('Ctrl Pts',(-5.76154733999022,-10.3229876482558,
-1.69304521941782));
#45347=CARTESIAN_POINT('Ctrl Pts',(-5.77466527474165,-10.312824454024,-1.68252036580709));
#45348=CARTESIAN_POINT('Ctrl Pts',(-5.78865529222855,-10.3019856087545,
-1.67129581797611));
#45349=CARTESIAN_POINT('Ctrl Pts',(-5.80168737233449,-10.2917664779376,
-1.65969882280271));
#45350=CARTESIAN_POINT('Ctrl Pts',(-5.81378838674191,-10.2821515626752,
-1.64795566811796));
#45351=CARTESIAN_POINT('Ctrl Pts',(-5.81702433828646,-10.2795804228643,
-1.64481541241207));
#45352=CARTESIAN_POINT('Ctrl Pts',(-5.82019384896885,-10.2770524509315,
-1.64166444950863));
#45353=CARTESIAN_POINT('Ctrl Pts',(-5.82329771974396,-10.2745672670514,
-1.63850657699136));
#45354=CARTESIAN_POINT('Ctrl Pts',(-5.8355361489205,-10.2647682937338,-1.62605522126444));
#45355=CARTESIAN_POINT('Ctrl Pts',(-5.84675316302517,-10.2556347018213,
-1.61350107932942));
#45356=CARTESIAN_POINT('Ctrl Pts',(-5.85702788756751,-10.2471307840155,
-1.60107214140025));
#45357=CARTESIAN_POINT('Ctrl Pts',(-5.86787652332103,-10.2381518662477,
-1.58794896521767));
#45358=CARTESIAN_POINT('Ctrl Pts',(-5.87767498429896,-10.2298749456108,
-1.57496478366363));
#45359=CARTESIAN_POINT('Ctrl Pts',(-5.88652865659392,-10.2222552746475,
-1.56232703905979));
#45360=CARTESIAN_POINT('Ctrl Pts',(-5.89063581815402,-10.2187205583582,
-1.55646447072499));
#45361=CARTESIAN_POINT('Ctrl Pts',(-5.89453980742874,-10.2153272436063,
-1.5506756773578));
#45362=CARTESIAN_POINT('Ctrl Pts',(-5.89825174144949,-10.2120707033626,
-1.54497772837812));
#45363=CARTESIAN_POINT('Ctrl Pts',(-5.90079700827138,-10.2098376992763,
-1.54107065448895));
#45364=CARTESIAN_POINT('Ctrl Pts',(-5.90325198131623,-10.2076690021697,
-1.5372062485125));
#45365=CARTESIAN_POINT('Ctrl Pts',(-5.90562031314519,-10.2055631001007,
-1.53338947434416));
#45366=CARTESIAN_POINT('Ctrl Pts',(-5.90870165683338,-10.2028231934842,
-1.52842361911682));
#45367=CARTESIAN_POINT('Ctrl Pts',(-5.91163635921931,-10.2001895742701,
-1.52353845169898));
#45368=CARTESIAN_POINT('Ctrl Pts',(-5.91443325305649,-10.1976585839042,
-1.5187447557545));
#45369=CARTESIAN_POINT('Ctrl Pts',(-5.91690655130083,-10.1954204245772,
-1.51450568181975));
#45370=CARTESIAN_POINT('Ctrl Pts',(-5.91927202264034,-10.193262552503,-1.5103382089865));
#45371=CARTESIAN_POINT('Ctrl Pts',(-5.92153571922348,-10.19118246343,-1.50624882670116));
#45372=CARTESIAN_POINT('Ctrl Pts',(-5.92266756751504,-10.1901424188935,
-1.50420413555849));
#45373=CARTESIAN_POINT('Ctrl Pts',(-5.92377396493195,-10.1891218219138,
-1.50217896241016));
#45374=CARTESIAN_POINT('Ctrl Pts',(-5.92485564717634,-10.1881203718994,
-1.50017406310495));
#45375=CARTESIAN_POINT('Ctrl Pts',(-5.92560719767657,-10.1874245665803,
-1.49878106337368));
#45376=CARTESIAN_POINT('Ctrl Pts',(-5.92602433317219,-10.1870369676126,
-1.49800196274449));
#45377=CARTESIAN_POINT('Ctrl Pts',(-5.92678068430343,-10.1863338258392,
-1.49657861446054));
#45378=CARTESIAN_POINT('Ctrl Pts',(-5.92711292480898,-10.1860249584777,
-1.49595338375233));
#45379=CARTESIAN_POINT('Ctrl Pts',(-5.92751030725292,-10.1856553325483,
-1.49520362583492));
#45380=CARTESIAN_POINT('Ctrl Pts',(-5.92802726401371,-10.1851731662489,
-1.49422091618995));
#45381=CARTESIAN_POINT('Ctrl Pts',(-5.93805899290194,-10.1758165585765,
-1.47515108775915));
#45382=CARTESIAN_POINT('Ctrl Pts',(-5.94688316212083,-10.167219859019,-1.45604567430618));
#45383=CARTESIAN_POINT('Ctrl Pts',(-5.95457617719396,-10.1593487697172,
-1.43711977445761));
#45384=CARTESIAN_POINT('Ctrl Pts',(-5.95804238262117,-10.1558023302267,
-1.42859242124872));
#45385=CARTESIAN_POINT('Ctrl Pts',(-5.96127901274585,-10.1524031576502,
-1.42010076683425));
#45386=CARTESIAN_POINT('Ctrl Pts',(-5.96429344506242,-10.1491478826819,
-1.41166115255928));
#45387=CARTESIAN_POINT('Ctrl Pts',(-5.97111461924745,-10.1417817204174,
-1.39256366653919));
#45388=CARTESIAN_POINT('Ctrl Pts',(-5.97679899638919,-10.1351521056581,
-1.37373632694532));
#45389=CARTESIAN_POINT('Ctrl Pts',(-5.9814779356399,-10.1292018249404,-1.35536282981741));
#45390=CARTESIAN_POINT('Ctrl Pts',(-5.98645891671279,-10.1228674328817,
-1.33580325946756));
#45391=CARTESIAN_POINT('Ctrl Pts',(-5.99030000768087,-10.1173030384771,
-1.31675774988199));
#45392=CARTESIAN_POINT('Ctrl Pts',(-5.99315258066888,-10.1124410972658,
-1.29838967202608));
#45393=CARTESIAN_POINT('Ctrl Pts',(-5.99393040688752,-10.1111153659476,
-1.29338115073585));
#45394=CARTESIAN_POINT('Ctrl Pts',(-5.99463471835723,-10.1098418656255,
-1.28842269455032));
#45395=CARTESIAN_POINT('Ctrl Pts',(-5.99526856528322,-10.1086192284365,
-1.28351696554966));
#45396=CARTESIAN_POINT('Ctrl Pts',(-5.99769622385822,-10.1039364800718,
-1.26472783115988));
#45397=CARTESIAN_POINT('Ctrl Pts',(-5.99909225943474,-10.0999991328637,
-1.24671594303783));
#45398=CARTESIAN_POINT('Ctrl Pts',(-5.99967114898183,-10.0967163116773,
-1.22960239785998));
#45399=CARTESIAN_POINT('Ctrl Pts',(-5.99988467765173,-10.0955054132512,
-1.22328991120778));
#45400=CARTESIAN_POINT('Ctrl Pts',(-5.99998680318323,-10.0943836490406,
-1.21709917912635));
#45401=CARTESIAN_POINT('Ctrl Pts',(-5.99998760030264,-10.0933467246824,
-1.2110347037336));
#45402=CARTESIAN_POINT('Ctrl Pts',(-5.72202416445507,-19.896080483841,-0.38635213055219));
#45403=CARTESIAN_POINT('Ctrl Pts',(-5.72274509910989,-19.5069873331202,
-0.666957234194769));
#45404=CARTESIAN_POINT('Ctrl Pts',(-5.72404064479545,-18.6535903875356,
-1.1961908244877));
#45405=CARTESIAN_POINT('Ctrl Pts',(-5.72530480851401,-17.2528827365553,
-1.80439821707277));
#45406=CARTESIAN_POINT('Ctrl Pts',(-5.72546472270845,-15.736565475542,-2.2042607128638));
#45407=CARTESIAN_POINT('Ctrl Pts',(-5.72471296068136,-14.1774181352031,
-2.37060073454058));
#45408=CARTESIAN_POINT('Ctrl Pts',(-5.72306515483269,-12.6107756304975,
-2.29992921776468));
#45409=CARTESIAN_POINT('Ctrl Pts',(-5.72038844431872,-11.1578233703468,
-2.00976160017932));
#45410=CARTESIAN_POINT('Ctrl Pts',(-5.7182968342637,-10.2528022212897,-1.69379809018474));
#45411=CARTESIAN_POINT('Ctrl Pts',(-5.71724124700401,-9.85241025758025,
-1.52490681965617));
#45412=CARTESIAN_POINT('Ctrl Pts',(-5.90060823215151,-19.8625946053881,
-0.339971041473725));
#45413=CARTESIAN_POINT('Ctrl Pts',(-5.90122084670813,-19.4754696620329,
-0.618738138938865));
#45414=CARTESIAN_POINT('Ctrl Pts',(-5.9023204460776,-18.6265003299919,-1.14450141769569));
#45415=CARTESIAN_POINT('Ctrl Pts',(-5.90338936516232,-17.2335638027759,
-1.74868173897509));
#45416=CARTESIAN_POINT('Ctrl Pts',(-5.90352454452386,-15.7258613601765,
-2.14619370052648));
#45417=CARTESIAN_POINT('Ctrl Pts',(-5.90288894892118,-14.1756858957418,
-2.31193403433321));
#45418=CARTESIAN_POINT('Ctrl Pts',(-5.901494071418,-12.6178346891394,-2.24244445825396));
#45419=CARTESIAN_POINT('Ctrl Pts',(-5.89921767773962,-11.1727295931907,
-1.95513745678009));
#45420=CARTESIAN_POINT('Ctrl Pts',(-5.89743434113683,-10.2722519885276,
-1.64180928578988));
#45421=CARTESIAN_POINT('Ctrl Pts',(-5.89652835820574,-9.87381091535684,
-1.47428053681659));
#45422=CARTESIAN_POINT('Ctrl Pts',(-6.00788367329973,-19.772514726196,-0.215201886826365));
#45423=CARTESIAN_POINT('Ctrl Pts',(-6.00820500171987,-19.3910981597869,
-0.489597435763965));
#45424=CARTESIAN_POINT('Ctrl Pts',(-6.00878012268355,-18.5546160874628,
-1.00717322647165));
#45425=CARTESIAN_POINT('Ctrl Pts',(-6.00933405165869,-17.182687364822,-1.60184063753912));
#45426=CARTESIAN_POINT('Ctrl Pts',(-6.00940405655402,-15.6976641614973,
-1.99332436904445));
#45427=CARTESIAN_POINT('Ctrl Pts',(-6.00907475857469,-14.1710484293059,
-2.15676410330651));
#45428=CARTESIAN_POINT('Ctrl Pts',(-6.00834991091154,-12.6365876990538,
-2.08880850537947));
#45429=CARTESIAN_POINT('Ctrl Pts',(-6.00715353710836,-11.2131204160208,
-1.80660613510079));
#45430=CARTESIAN_POINT('Ctrl Pts',(-6.00621053085834,-10.3258101505897,
-1.49852045391835));
#45431=CARTESIAN_POINT('Ctrl Pts',(-6.00572389292896,-9.93320084529256,
-1.33378507160552));
#45432=CARTESIAN_POINT('Ctrl Pts',(-5.99961011528539,-19.662775821354,-0.0632031012907194));
#45433=CARTESIAN_POINT('Ctrl Pts',(-5.999576626112,-19.2884675084672,-0.332486393375608));
#45434=CARTESIAN_POINT('Ctrl Pts',(-5.99951378747744,-18.4674126509003,
-0.840515375700035));
#45435=CARTESIAN_POINT('Ctrl Pts',(-5.99944414651886,-17.1211147651734,
-1.42408546730994));
#45436=CARTESIAN_POINT('Ctrl Pts',(-5.99943526138757,-15.6635358355136,
-1.8083351975207));
#45437=CARTESIAN_POINT('Ctrl Pts',(-5.9994767984071,-14.165407226967,-1.96871625381771));
#45438=CARTESIAN_POINT('Ctrl Pts',(-5.99956434621717,-12.659345301581,-1.90201657891025));
#45439=CARTESIAN_POINT('Ctrl Pts',(-5.99968486264664,-11.2624348032458,
-1.6250680610208));
#45440=CARTESIAN_POINT('Ctrl Pts',(-5.99976969499778,-10.3915173827786,
-1.32268120907084));
#45441=CARTESIAN_POINT('Ctrl Pts',(-5.99980021247357,-10.0062299524239,
-1.1610240938064));
#45442=CARTESIAN_POINT('',(-5.99999988467789,-19.5919337295697,-0.135483989339417));
#45443=CARTESIAN_POINT('Origin',(-5.59998164341111,-19.5919273324348,-0.135474139643786));
#45444=CARTESIAN_POINT('Ctrl Pts',(-6.,-19.5919320859662,-0.135483413483151));
#45445=CARTESIAN_POINT('Ctrl Pts',(-6.,-19.2032417091454,-0.410171487578889));
#45446=CARTESIAN_POINT('Ctrl Pts',(-6.,-18.7991432008221,-0.654503377429215));
#45447=CARTESIAN_POINT('Ctrl Pts',(-6.,-18.3770565087312,-0.869913253532343));
#45448=CARTESIAN_POINT('Ctrl Pts',(-6.,-17.9549695181175,-1.08532328198508));
#45449=CARTESIAN_POINT('Ctrl Pts',(-6.,-17.5148943182916,-1.27181125578016));
#45450=CARTESIAN_POINT('Ctrl Pts',(-6.,-17.0647735489823,-1.42538958558456));
#45451=CARTESIAN_POINT('Ctrl Pts',(-6.,-16.6146527796733,-1.57896791538885));
#45452=CARTESIAN_POINT('Ctrl Pts',(-6.,-16.1544864408809,-1.69963660120252));
#45453=CARTESIAN_POINT('Ctrl Pts',(-6.,-15.6870767394187,-1.78685625681736));
#45454=CARTESIAN_POINT('Ctrl Pts',(-6.,-15.2196670379562,-1.87407591243227));
#45455=CARTESIAN_POINT('Ctrl Pts',(-6.,-14.7450139738239,-1.9278465378483));
#45456=CARTESIAN_POINT('Ctrl Pts',(-6.,-14.2698875141637,-1.94742220575385));
#45457=CARTESIAN_POINT('Ctrl Pts',(-6.,-13.7947610545038,-1.96699787365938));
#45458=CARTESIAN_POINT('Ctrl Pts',(-6.,-13.3191611993158,-1.95237858405447));
#45459=CARTESIAN_POINT('Ctrl Pts',(-6.,-12.8461741404248,-1.9034307291296));
#45460=CARTESIAN_POINT('Ctrl Pts',(-6.,-12.3731870815335,-1.8544828742047));
#45461=CARTESIAN_POINT('Ctrl Pts',(-6.,-11.902812818939,-1.7712064539598));
#45462=CARTESIAN_POINT('Ctrl Pts',(-6.,-11.4430952346575,-1.65563716855819));
#45463=CARTESIAN_POINT('Ctrl Pts',(-6.,-10.9833776503763,-1.54006788315667));
#45464=CARTESIAN_POINT('Ctrl Pts',(-6.,-10.534316744408,-1.3922057325985));
#45465=CARTESIAN_POINT('Ctrl Pts',(-6.,-10.0933467248347,-1.21103470482109));
#45466=CARTESIAN_POINT('Origin',(-5.599999999997,-19.5919343769627,-0.135488060674723));
#45467=CARTESIAN_POINT('Origin',(-5.6,-19.5919343770088,-0.135488060674804));
#45468=CARTESIAN_POINT('Ctrl Pts',(-6.05109153972374,-10.3133667341249,
1.22786565167224));
#45469=CARTESIAN_POINT('Ctrl Pts',(-6.05168701826986,-10.3097181511851,
1.25641881093765));
#45470=CARTESIAN_POINT('Ctrl Pts',(-6.04650592810586,-10.3031083021162,
1.32768592853605));
#45471=CARTESIAN_POINT('Ctrl Pts',(-6.01133171463065,-10.3019952910507,
1.44465332307405));
#45472=CARTESIAN_POINT('Ctrl Pts',(-5.93768049219332,-10.3139871653149,
1.56711227223071));
#45473=CARTESIAN_POINT('Ctrl Pts',(-5.83457780306427,-10.338943074529,1.66810020812682));
#45474=CARTESIAN_POINT('Ctrl Pts',(-5.75268739346611,-10.3627238857495,
1.71461716070258));
#45475=CARTESIAN_POINT('Ctrl Pts',(-5.71134642253387,-10.3755278527837,
1.73144896239704));
#45476=CARTESIAN_POINT('Ctrl Pts',(-5.91162511589862,-10.0312698687459,
1.19498180009067));
#45477=CARTESIAN_POINT('Ctrl Pts',(-5.91217091556656,-10.0279827855256,
1.22064564700957));
#45478=CARTESIAN_POINT('Ctrl Pts',(-5.90742260833259,-10.0220743811926,
1.28499549547033));
#45479=CARTESIAN_POINT('Ctrl Pts',(-5.87483642927485,-10.0214543387037,
1.39153554130379));
#45480=CARTESIAN_POINT('Ctrl Pts',(-5.80621654839343,-10.0331762556504,
1.50374676368135));
#45481=CARTESIAN_POINT('Ctrl Pts',(-5.7099450100689,-10.0569984449157,1.5965419795219));
#45482=CARTESIAN_POINT('Ctrl Pts',(-5.63351072591731,-10.0794492920087,
1.63929312886841));
#45483=CARTESIAN_POINT('Ctrl Pts',(-5.59497657724959,-10.0914724853859,
1.65475784875777));
#45484=CARTESIAN_POINT('Ctrl Pts',(-6.02845068814037,-9.73989925133785,
1.1553984959079));
#45485=CARTESIAN_POINT('Ctrl Pts',(-6.02930891897681,-9.734848401818,1.19496164129932));
#45486=CARTESIAN_POINT('Ctrl Pts',(-6.02183770779464,-9.72585114962533,
1.29200191301737));
#45487=CARTESIAN_POINT('Ctrl Pts',(-5.97369625583695,-9.72423080924438,
1.44601588767161));
#45488=CARTESIAN_POINT('Ctrl Pts',(-5.87575056987504,-9.7394605190118,1.60373718212841));
#45489=CARTESIAN_POINT('Ctrl Pts',(-5.74020185361633,-9.77133573768165,
1.73283824846435));
#45490=CARTESIAN_POINT('Ctrl Pts',(-5.63231671304093,-9.80212962140831,
1.79269764930981));
#45491=CARTESIAN_POINT('Ctrl Pts',(-5.57746663048118,-9.81892782672867,
1.8145192676118));
#45492=CARTESIAN_POINT('Ctrl Pts',(-6.32476389007387,-9.63080942597427,
1.13513882712025));
#45493=CARTESIAN_POINT('Ctrl Pts',(-6.32609126151429,-9.62302909136911,
1.19625211045084));
#45494=CARTESIAN_POINT('Ctrl Pts',(-6.31453156942281,-9.60918339014722,
1.34409893727426));
#45495=CARTESIAN_POINT('Ctrl Pts',(-6.24291798999123,-9.60572710830813,
1.57227748454183));
#45496=CARTESIAN_POINT('Ctrl Pts',(-6.10056892161608,-9.62593624443112,
1.80134710805399));
#45497=CARTESIAN_POINT('Ctrl Pts',(-5.90545656698247,-9.66975696497354,
1.9873841556488));
#45498=CARTESIAN_POINT('Ctrl Pts',(-5.74989022311378,-9.71308195056143,
2.07397843945383));
#45499=CARTESIAN_POINT('Ctrl Pts',(-5.67032798222648,-9.73707173278376,
2.10570174094662));
#45500=CARTESIAN_POINT('',(-5.73278684135576,-10.3449539124238,1.71288839099263));
#45501=CARTESIAN_POINT('',(-5.72001801994993,-9.72697588660814,2.0594323552405));
#45502=CARTESIAN_POINT('Origin',(-5.89875570320666,-10.183796169743,2.15613415615742));
#45503=CARTESIAN_POINT('',(-5.99999929232988,-9.65439067775597,1.86246363135436));
#45504=CARTESIAN_POINT('Ctrl Pts',(-5.99999893849482,-9.65439067472951,
1.86246363077086));
#45505=CARTESIAN_POINT('Ctrl Pts',(-5.97805268655099,-9.65924092589487,
1.88418829577225));
#45506=CARTESIAN_POINT('Ctrl Pts',(-5.95524919802917,-9.66452973534359,
1.90483819465336));
#45507=CARTESIAN_POINT('Ctrl Pts',(-5.93158556654339,-9.67026253132554,
1.92442749634617));
#45508=CARTESIAN_POINT('Ctrl Pts',(-5.9160574628656,-9.67402439900105,1.93728201987288));
#45509=CARTESIAN_POINT('Ctrl Pts',(-5.90015824989656,-9.67797778998414,
1.94967915132359));
#45510=CARTESIAN_POINT('Ctrl Pts',(-5.88388032252451,-9.68212790070371,
1.96161343442713));
#45511=CARTESIAN_POINT('Ctrl Pts',(-5.87899228981368,-9.68337412059936,
1.96519713183879));
#45512=CARTESIAN_POINT('Ctrl Pts',(-5.87407007591581,-9.684638098141,1.96873903743644));
#45513=CARTESIAN_POINT('Ctrl Pts',(-5.8691134996699,-9.68591996775037,1.97223895502917));
#45514=CARTESIAN_POINT('Ctrl Pts',(-5.84413887119461,-9.69237890546449,
1.98987393878327));
#45515=CARTESIAN_POINT('Ctrl Pts',(-5.8182953080106,-9.69929107464239,2.00644232267157));
#45516=CARTESIAN_POINT('Ctrl Pts',(-5.79155901126676,-9.70667871645196,
2.02188615936239));
#45517=CARTESIAN_POINT('Ctrl Pts',(-5.76839010741707,-9.71308063383048,
2.03526934293446));
#45518=CARTESIAN_POINT('Ctrl Pts',(-5.74455030676941,-9.71983983716558,
2.04780760010186));
#45519=CARTESIAN_POINT('Ctrl Pts',(-5.72001861626288,-9.72697741058235,
2.05943267791248));
#45520=CARTESIAN_POINT('',(-5.99998819251561,-10.0933467209694,1.21103471954976));
#45521=CARTESIAN_POINT('Ctrl Pts',(-5.99998819251561,-10.0933467209694,
1.21103471954976));
#45522=CARTESIAN_POINT('Ctrl Pts',(-5.99998385620494,-10.0704631806786,
1.22848204334355));
#45523=CARTESIAN_POINT('Ctrl Pts',(-5.99998335501883,-10.0483848922226,
1.24627131943011));
#45524=CARTESIAN_POINT('Ctrl Pts',(-5.99998071362119,-10.0271414920569,
1.26441751382506));
#45525=CARTESIAN_POINT('Ctrl Pts',(-5.99997953604353,-10.0176708417291,
1.27250737988019));
#45526=CARTESIAN_POINT('Ctrl Pts',(-5.99997744109942,-10.0083656975942,
1.28066765022114));
#45527=CARTESIAN_POINT('Ctrl Pts',(-5.99997276079776,-9.99922669686015,
1.28889762257333));
#45528=CARTESIAN_POINT('Ctrl Pts',(-5.99995937880447,-9.97309631996056,
1.31242889100122));
#45529=CARTESIAN_POINT('Ctrl Pts',(-5.99992732479033,-9.94832580753097,
1.33652904861389));
#45530=CARTESIAN_POINT('Ctrl Pts',(-5.99991639997273,-9.92486788112492,
1.36119507363657));
#45531=CARTESIAN_POINT('Ctrl Pts',(-5.99990337118461,-9.89689227876561,
1.39061143789123));
#45532=CARTESIAN_POINT('Ctrl Pts',(-5.99990194905953,-9.87082206904309,
1.4208469219927));
#45533=CARTESIAN_POINT('Ctrl Pts',(-5.99990827523113,-9.8466640461254,1.4518882119366));
#45534=CARTESIAN_POINT('Ctrl Pts',(-5.99991044005314,-9.83839714741086,
1.46251057125836));
#45535=CARTESIAN_POINT('Ctrl Pts',(-5.99991349017294,-9.83035412851919,
1.47322774561128));
#45536=CARTESIAN_POINT('Ctrl Pts',(-5.99991818442103,-9.82253532698912,
1.48404251962809));
#45537=CARTESIAN_POINT('Ctrl Pts',(-5.99992099506536,-9.8178538807407,1.49051778096498));
#45538=CARTESIAN_POINT('Ctrl Pts',(-5.99992891243512,-9.8130914911253,1.4972467019501));
#45539=CARTESIAN_POINT('Ctrl Pts',(-5.9999340958716,-9.80847580936703,1.50393435657881));
#45540=CARTESIAN_POINT('Ctrl Pts',(-5.99993934522864,-9.80380142749364,
1.51070706171949));
#45541=CARTESIAN_POINT('Ctrl Pts',(-5.99994151967764,-9.79927770768895,
1.51743718021492));
#45542=CARTESIAN_POINT('Ctrl Pts',(-5.99994633539954,-9.79510546243412,
1.52377937107288));
#45543=CARTESIAN_POINT('Ctrl Pts',(-5.99994714803865,-9.79440140813732,
1.52484959740233));
#45544=CARTESIAN_POINT('Ctrl Pts',(-5.99994807169794,-9.79370727989116,
1.52590869658738));
#45545=CARTESIAN_POINT('Ctrl Pts',(-5.99994917731444,-9.79302394495788,
1.52695491650741));
#45546=CARTESIAN_POINT('Ctrl Pts',(-5.99997543479574,-9.77679530309569,
1.55180177792813));
#45547=CARTESIAN_POINT('Ctrl Pts',(-5.99996041338706,-9.7619038161661,1.57694685829143));
#45548=CARTESIAN_POINT('Ctrl Pts',(-5.99993528590784,-9.74828232671954,
1.60234427928765));
#45549=CARTESIAN_POINT('Ctrl Pts',(-5.99991079530336,-9.73500608410708,
1.62709798366042));
#45550=CARTESIAN_POINT('Ctrl Pts',(-5.99987824956351,-9.7229352977466,1.65209229785361));
#45551=CARTESIAN_POINT('Ctrl Pts',(-5.99986339636884,-9.71204080581989,
1.6773206358393));
#45552=CARTESIAN_POINT('Ctrl Pts',(-5.99985777962819,-9.7079210499701,1.68686074048081));
#45553=CARTESIAN_POINT('Ctrl Pts',(-5.99985454323938,-9.70396991374468,
1.69643460684258));
#45554=CARTESIAN_POINT('Ctrl Pts',(-5.99985429814471,-9.70018741400251,
1.70604274813774));
#45555=CARTESIAN_POINT('Ctrl Pts',(-5.99985368026242,-9.69065175332556,
1.73026481855996));
#45556=CARTESIAN_POINT('Ctrl Pts',(-5.999874605093,-9.68218513529061,1.75470487599331));
#45557=CARTESIAN_POINT('Ctrl Pts',(-5.99990791809376,-9.67481341330724,
1.77937946321238));
#45558=CARTESIAN_POINT('Ctrl Pts',(-5.99994036861482,-9.6676325465567,1.80341522084737));
#45559=CARTESIAN_POINT('Ctrl Pts',(-5.99998501038468,-9.66149118947295,
1.82767449085469));
#45560=CARTESIAN_POINT('Ctrl Pts',(-5.99999646663191,-9.65644537758714,
1.85216368682354));
#45561=CARTESIAN_POINT('Ctrl Pts',(-5.99999807067108,-9.65573889144184,
1.85559252603773));
#45562=CARTESIAN_POINT('Ctrl Pts',(-5.99999895813432,-9.65505392589765,
1.85902584493278));
#45563=CARTESIAN_POINT('Ctrl Pts',(-5.99999893849482,-9.65439067472951,
1.86246363077086));
#45564=CARTESIAN_POINT('Ctrl Pts',(-5.99998819251561,-10.0933467209694,
1.21103471954976));
#45565=CARTESIAN_POINT('Ctrl Pts',(-5.99998402550715,-10.0961384851397,
1.22737632814287));
#45566=CARTESIAN_POINT('Ctrl Pts',(-5.99924438896618,-10.0995471624567,
1.24464108102516));
#45567=CARTESIAN_POINT('Ctrl Pts',(-5.99756998416535,-10.1036582604973,
1.26272592288279));
#45568=CARTESIAN_POINT('Ctrl Pts',(-5.99660204936694,-10.1060347914599,
1.27318035286841));
#45569=CARTESIAN_POINT('Ctrl Pts',(-5.99532147474186,-10.1086461707087,
1.28390802980007));
#45570=CARTESIAN_POINT('Ctrl Pts',(-5.99368665768074,-10.1115100796409,
1.29488167197767));
#45571=CARTESIAN_POINT('Ctrl Pts',(-5.99144878963691,-10.1154304267136,
1.30990326903442));
#45572=CARTESIAN_POINT('Ctrl Pts',(-5.98854666000694,-10.1198241527659,
1.32538674595495));
#45573=CARTESIAN_POINT('Ctrl Pts',(-5.98489855986274,-10.1247279755564,
1.3412469846118));
#45574=CARTESIAN_POINT('Ctrl Pts',(-5.98070306937735,-10.1303676074323,
1.35948702127484));
#45575=CARTESIAN_POINT('Ctrl Pts',(-5.97552128947864,-10.1366817915978,
1.37822691854081));
#45576=CARTESIAN_POINT('Ctrl Pts',(-5.96922654119519,-10.1437264409335,
1.39729514499616));
#45577=CARTESIAN_POINT('Ctrl Pts',(-5.96732685751383,-10.1458524362523,
1.40304971960318));
#45578=CARTESIAN_POINT('Ctrl Pts',(-5.96532577018031,-10.1480449657855,
1.40883384962093));
#45579=CARTESIAN_POINT('Ctrl Pts',(-5.96321966706526,-10.150305591362,1.41464186523372));
#45580=CARTESIAN_POINT('Ctrl Pts',(-5.96201716271702,-10.1515963221273,
1.41795802006921));
#45581=CARTESIAN_POINT('Ctrl Pts',(-5.96078042200169,-10.1529092522677,
1.42128195300577));
#45582=CARTESIAN_POINT('Ctrl Pts',(-5.95950875996098,-10.1542446751975,
1.42461253551312));
#45583=CARTESIAN_POINT('Ctrl Pts',(-5.95597676213336,-10.1579537667138,
1.43386311452248));
#45584=CARTESIAN_POINT('Ctrl Pts',(-5.95217532292998,-10.161836398445,1.4431651786973));
#45585=CARTESIAN_POINT('Ctrl Pts',(-5.94809550841192,-10.1658966382478,
1.45249663410328));
#45586=CARTESIAN_POINT('Ctrl Pts',(-5.94532115205228,-10.1686576834054,
1.45884221244653));
#45587=CARTESIAN_POINT('Ctrl Pts',(-5.94241803296839,-10.1715009005813,
1.46520142973038));
#45588=CARTESIAN_POINT('Ctrl Pts',(-5.93938352102913,-10.1744274340502,
1.47156643417996));
#45589=CARTESIAN_POINT('Ctrl Pts',(-5.93786470710498,-10.1758922033017,
1.47475220427373));
#45590=CARTESIAN_POINT('Ctrl Pts',(-5.93608622095482,-10.177596339097,1.47840532593482));
#45591=CARTESIAN_POINT('Ctrl Pts',(-5.93438240493213,-10.1792142823947,
1.48182159957326));
#45592=CARTESIAN_POINT('Ctrl Pts',(-5.93268208435788,-10.1808289064154,
1.48523086458626));
#45593=CARTESIAN_POINT('Ctrl Pts',(-5.93105726019389,-10.1823572353098,
1.48840473398473));
#45594=CARTESIAN_POINT('Ctrl Pts',(-5.92988309980082,-10.1834582505981,
1.4906706473117));
#45595=CARTESIAN_POINT('Ctrl Pts',(-5.92268037136545,-10.1902122802619,
1.50457058674809));
#45596=CARTESIAN_POINT('Ctrl Pts',(-5.91461871252513,-10.1975738668864,
1.51888678624592));
#45597=CARTESIAN_POINT('Ctrl Pts',(-5.90558148547629,-10.2055918580846,
1.53344585887442));
#45598=CARTESIAN_POINT('Ctrl Pts',(-5.90267790306295,-10.208167968888,1.53812356222416));
#45599=CARTESIAN_POINT('Ctrl Pts',(-5.899673623005,-10.2108118399798,1.54282594880722));
#45600=CARTESIAN_POINT('Ctrl Pts',(-5.89656480451811,-10.2135250963317,
1.54754608499053));
#45601=CARTESIAN_POINT('Ctrl Pts',(-5.8871051820906,-10.2217810883578,1.56190868167757));
#45602=CARTESIAN_POINT('Ctrl Pts',(-5.87667643703934,-10.2306799225328,
1.5764390153283));
#45603=CARTESIAN_POINT('Ctrl Pts',(-5.86519923836702,-10.2402555319518,
1.59093668969711));
#45604=CARTESIAN_POINT('Ctrl Pts',(-5.85453478592901,-10.2491530542592,
1.60440772589525));
#45605=CARTESIAN_POINT('Ctrl Pts',(-5.84296508897445,-10.2586348387852,
1.61785078716441));
#45606=CARTESIAN_POINT('Ctrl Pts',(-5.83043950416598,-10.2687242962313,
1.6310627672712));
#45607=CARTESIAN_POINT('Ctrl Pts',(-5.82324245850783,-10.2745215733257,
1.63865420715343));
#45608=CARTESIAN_POINT('Ctrl Pts',(-5.81573006887528,-10.2805194060275,
1.64616855216329));
#45609=CARTESIAN_POINT('Ctrl Pts',(-5.80789496961468,-10.2867217253361,
1.65355967409042));
#45610=CARTESIAN_POINT('Ctrl Pts',(-5.79492426015451,-10.2969894295546,
1.66579539592531));
#45611=CARTESIAN_POINT('Ctrl Pts',(-5.78106749379734,-10.3078180566375,
1.67769523356719));
#45612=CARTESIAN_POINT('Ctrl Pts',(-5.76632933899584,-10.3192095047188,
1.68905255240334));
#45613=CARTESIAN_POINT('Ctrl Pts',(-5.7556093897998,-10.3274951921976,1.69731341562309));
#45614=CARTESIAN_POINT('Ctrl Pts',(-5.74442358376035,-10.3360784934701,
1.70528659045044));
#45615=CARTESIAN_POINT('Ctrl Pts',(-5.73278287705707,-10.3449577598948,
1.71287781032009));
#45616=CARTESIAN_POINT('Ctrl Pts',(-5.71725917948286,-9.85240188395848,
1.52489732935885));
#45617=CARTESIAN_POINT('Ctrl Pts',(-5.71831476133586,-10.2527968008031,
1.69379032983208));
#45618=CARTESIAN_POINT('Ctrl Pts',(-5.72040635428649,-11.1578213001714,
2.00975542479402));
#45619=CARTESIAN_POINT('Ctrl Pts',(-5.72308302960212,-12.6107763015806,
2.29992344875424));
#45620=CARTESIAN_POINT('Ctrl Pts',(-5.72473081064846,-14.177417972093,2.37059485980144));
#45621=CARTESIAN_POINT('Ctrl Pts',(-5.72548256087693,-15.7365643949578,
2.20425489419934));
#45622=CARTESIAN_POINT('Ctrl Pts',(-5.72532264924983,-17.2528807820375,
1.80439264348976));
#45623=CARTESIAN_POINT('Ctrl Pts',(-5.72405850848059,-18.6535837735938,
1.19618733853812));
#45624=CARTESIAN_POINT('Ctrl Pts',(-5.72276299024073,-19.5069768607809,
0.666956934041539));
#45625=CARTESIAN_POINT('Ctrl Pts',(-5.72204207444442,-19.8960667568706,
0.386354961461413));
#45626=CARTESIAN_POINT('Ctrl Pts',(-5.89585261036639,-9.8737233640862,1.47445851034686));
#45627=CARTESIAN_POINT('Ctrl Pts',(-5.89675914115004,-10.2721745670443,
1.64199409608624));
#45628=CARTESIAN_POINT('Ctrl Pts',(-5.89854359746305,-11.1726722809412,
1.95533375189407));
#45629=CARTESIAN_POINT('Ctrl Pts',(-5.90082144131746,-12.6178091621264,
2.24265196275686));
#45630=CARTESIAN_POINT('Ctrl Pts',(-5.90221723230456,-14.1756921586905,
2.31214594307168));
#45631=CARTESIAN_POINT('Ctrl Pts',(-5.90285324758004,-15.7259000244731,
2.14640349435437));
#45632=CARTESIAN_POINT('Ctrl Pts',(-5.90271797885401,-17.2336335815138,
1.74888303750554));
#45633=CARTESIAN_POINT('Ctrl Pts',(-5.90164835746724,-18.626594283756,1.14468975580972));
#45634=CARTESIAN_POINT('Ctrl Pts',(-5.90054805708195,-19.4755761504201,
0.618916685086739));
#45635=CARTESIAN_POINT('Ctrl Pts',(-5.8999350585698,-19.8627051211047,0.340145838838019));
#45636=CARTESIAN_POINT('Ctrl Pts',(-6.00500261470054,-9.93280259933369,
1.33469847615741));
#45637=CARTESIAN_POINT('Ctrl Pts',(-6.00549199806467,-10.3254530800207,
1.49945394791177));
#45638=CARTESIAN_POINT('Ctrl Pts',(-6.00644049339831,-11.2128530699392,
1.80757571669982));
#45639=CARTESIAN_POINT('Ctrl Pts',(-6.00764392772595,-12.6364651528179,
2.08981216442348));
#45640=CARTESIAN_POINT('Ctrl Pts',(-6.00837315204832,-14.1710787346948,
2.15777783010585));
#45641=CARTESIAN_POINT('Ctrl Pts',(-6.00870445126686,-15.6978483680812,
1.99432307775469));
#45642=CARTESIAN_POINT('Ctrl Pts',(-6.00863402048019,-17.1830197265236,
1.6027999689954));
#45643=CARTESIAN_POINT('Ctrl Pts',(-6.00807672884764,-18.5550818810673,
1.00807203283005));
#45644=CARTESIAN_POINT('Ctrl Pts',(-6.00749818443475,-19.3916421670331,
0.490445507156552));
#45645=CARTESIAN_POINT('Ctrl Pts',(-6.00717495695829,-19.7730930164904,
0.216024270399581));
#45646=CARTESIAN_POINT('Ctrl Pts',(-5.99984758538782,-10.0055962683619,
1.16249500094862));
#45647=CARTESIAN_POINT('Ctrl Pts',(-5.99982148563193,-10.3909492485856,
1.32418019721138));
#45648=CARTESIAN_POINT('Ctrl Pts',(-5.99974542173439,-11.2620102881678,
1.62661749324998));
#45649=CARTESIAN_POINT('Ctrl Pts',(-5.99963615320918,-12.6591509434668,
1.90361155864705));
#45650=CARTESIAN_POINT('Ctrl Pts',(-5.99955554136504,-14.1654554059707,
1.97032198330928));
#45651=CARTESIAN_POINT('Ctrl Pts',(-5.99951717118125,-15.6638272479816,
1.80991481185425));
#45652=CARTESIAN_POINT('Ctrl Pts',(-5.9995253825072,-17.1216405130251,1.42560331832749));
#45653=CARTESIAN_POINT('Ctrl Pts',(-5.99958969901559,-18.4681535226324,
0.841940074435576));
#45654=CARTESIAN_POINT('Ctrl Pts',(-5.99964708911067,-19.2893368186713,
0.333832287822943));
#45655=CARTESIAN_POINT('Ctrl Pts',(-5.99967754848037,-19.6637028813994,
0.0645081662955123));
#45656=CARTESIAN_POINT('',(-5.99999997114735,-19.5919329044497,0.135484571583753));
#45657=CARTESIAN_POINT('Ctrl Pts',(-6.,-10.0933467210045,1.21103472159936));
#45658=CARTESIAN_POINT('Ctrl Pts',(-6.,-10.5343167948856,1.39220577636874));
#45659=CARTESIAN_POINT('Ctrl Pts',(-6.,-10.9833777476598,1.54006792210967));
#45660=CARTESIAN_POINT('Ctrl Pts',(-6.,-11.4430953691779,1.65563720320492));
#45661=CARTESIAN_POINT('Ctrl Pts',(-6.,-11.9028129906963,1.77120648430025));
#45662=CARTESIAN_POINT('Ctrl Pts',(-6.,-12.3731872809587,1.85448290074985));
#45663=CARTESIAN_POINT('Ctrl Pts',(-6.,-12.8461743349553,1.90343074841346));
#45664=CARTESIAN_POINT('Ctrl Pts',(-6.,-13.3191613889517,1.95237859607703));
#45665=CARTESIAN_POINT('Ctrl Pts',(-6.,-13.7947612066823,1.96699787495466));
#45666=CARTESIAN_POINT('Ctrl Pts',(-6.,-14.2698876412527,1.94742220105327));
#45667=CARTESIAN_POINT('Ctrl Pts',(-6.,-14.7450140758233,1.92784652715188));
#45668=CARTESIAN_POINT('Ctrl Pts',(-6.,-15.2196671272337,1.87407590047143));
#45669=CARTESIAN_POINT('Ctrl Pts',(-6.,-15.6870768246027,1.78685624112379));
#45670=CARTESIAN_POINT('Ctrl Pts',(-6.,-16.1544865219714,1.69963658177622));
#45671=CARTESIAN_POINT('Ctrl Pts',(-6.,-16.6146528652989,1.5789678897615));
#45672=CARTESIAN_POINT('Ctrl Pts',(-6.,-17.0647736279836,1.42538955895495));
#45673=CARTESIAN_POINT('Ctrl Pts',(-6.,-17.5148943906687,1.2718112281483));
#45674=CARTESIAN_POINT('Ctrl Pts',(-6.,-17.9549695727112,1.08532325854976));
#45675=CARTESIAN_POINT('Ctrl Pts',(-6.,-18.3770565476116,0.869913233962045));
#45676=CARTESIAN_POINT('Ctrl Pts',(-6.,-18.7991432239094,0.654503361764737));
#45677=CARTESIAN_POINT('Ctrl Pts',(-6.,-19.2032417185164,0.410171475499673));
#45678=CARTESIAN_POINT('Ctrl Pts',(-6.,-19.5919320853514,0.135483412539487));
#45679=CARTESIAN_POINT('',(-5.73644356943,-19.8089505408291,0.442546871815091));
#45680=CARTESIAN_POINT('Origin',(-5.59998163820134,-19.5919264032878,0.13547479132357));
#45681=CARTESIAN_POINT('Ctrl Pts',(-5.732787366965,-10.3449534027376,1.71288979180163));
#45682=CARTESIAN_POINT('Ctrl Pts',(-5.7346148093355,-11.1182357980457,1.9933278196275));
#45683=CARTESIAN_POINT('Ctrl Pts',(-5.73605973905547,-11.926552686004,2.18169252040153));
#45684=CARTESIAN_POINT('Ctrl Pts',(-5.73818934963262,-13.567539631559,2.35984303331276));
#45685=CARTESIAN_POINT('Ctrl Pts',(-5.73887403048981,-14.4000937496392,
2.35028712857065));
#45686=CARTESIAN_POINT('Ctrl Pts',(-5.73948314334139,-16.0408967489411,
2.1319111059007));
#45687=CARTESIAN_POINT('Ctrl Pts',(-5.73940757533578,-16.8491807345991,
1.92343367553535));
#45688=CARTESIAN_POINT('Ctrl Pts',(-5.73849619050221,-18.3938447089082,
1.31839091028631));
#45689=CARTESIAN_POINT('Ctrl Pts',(-5.73766037374166,-19.1301818702781,
0.921733792798441));
#45690=CARTESIAN_POINT('Ctrl Pts',(-5.73644356975375,-19.8089503602323,
0.442546999310109));
#45691=CARTESIAN_POINT('Origin',(-5.599999999997,-19.5919343769573,0.135488060979611));
#45692=CARTESIAN_POINT('',(-5.593361696257,-19.9918770425242,0.136828655319171));
#45693=CARTESIAN_POINT('Origin',(-5.599999999997,-19.5919343769573,0.135488060979611));
#45694=CARTESIAN_POINT('Origin',(-5.6,-19.5919343770044,0.135488060981261));
#45695=CARTESIAN_POINT('Ctrl Pts',(-5.59335880963393,-19.9918769844261,
0.13683170217352));
#45696=CARTESIAN_POINT('Ctrl Pts',(-5.59335897597995,-19.9918902023629,
0.132889263698737));
#45697=CARTESIAN_POINT('Ctrl Pts',(-5.59336249921667,-19.9921701764066,
0.0456108094042422));
#45698=CARTESIAN_POINT('Ctrl Pts',(-5.59336249921666,-19.9921701764069,
-0.0456108090957055));
#45699=CARTESIAN_POINT('Ctrl Pts',(-5.59335897597995,-19.9918902023646,
-0.132889263387482));
#45700=CARTESIAN_POINT('Ctrl Pts',(-5.59335880963393,-19.9918769844279,
-0.136831701864102));
#45701=CARTESIAN_POINT('Ctrl Pts',(-5.83074004395823,-19.9958187405297,
0.136844915099748));
#45702=CARTESIAN_POINT('Ctrl Pts',(-5.83074021193959,-19.9958318610111,
0.132902095574058));
#45703=CARTESIAN_POINT('Ctrl Pts',(-5.83074376981186,-19.9961097709333,
0.0456152065241441));
#45704=CARTESIAN_POINT('Ctrl Pts',(-5.83074376981186,-19.9961097709314,
-0.045615206214134));
#45705=CARTESIAN_POINT('Ctrl Pts',(-5.83074021193959,-19.9958318610128,
-0.132902095265616));
#45706=CARTESIAN_POINT('Ctrl Pts',(-5.83074004395823,-19.9958187405316,
-0.136844914793341));
#45707=CARTESIAN_POINT('Ctrl Pts',(-6.0000034748386,-19.8293408303188,0.136286874323727));
#45708=CARTESIAN_POINT('Ctrl Pts',(-6.00000357357481,-19.829353826502,0.132360134067906));
#45709=CARTESIAN_POINT('Ctrl Pts',(-6.00000566482207,-19.8296291037065,
0.0454292086005623));
#45710=CARTESIAN_POINT('Ctrl Pts',(-6.00000566482207,-19.8296291037088,
-0.0454292082960309));
#45711=CARTESIAN_POINT('Ctrl Pts',(-6.00000357357481,-19.829353826505,-0.132360133764468));
#45712=CARTESIAN_POINT('Ctrl Pts',(-6.0000034748386,-19.8293408303218,-0.136286874022272));
#45713=CARTESIAN_POINT('Ctrl Pts',(-5.9999999999769,-19.5919285123994,0.135491058510803));
#45714=CARTESIAN_POINT('Ctrl Pts',(-5.99999999996753,-19.5919414317201,
0.131587249061451));
#45715=CARTESIAN_POINT('Ctrl Pts',(-5.99999999976693,-19.5922150808804,
0.0451639658275807));
#45716=CARTESIAN_POINT('Ctrl Pts',(-5.99999999976693,-19.5922150808839,
-0.0451639655258958));
#45717=CARTESIAN_POINT('Ctrl Pts',(-5.99999999996752,-19.5919414317231,
-0.131587248762213));
#45718=CARTESIAN_POINT('Ctrl Pts',(-5.9999999999769,-19.5919285124023,-0.135491058213592));
#45719=CARTESIAN_POINT('Origin',(-5.47627985805297,17.2206464622639,-6.06762124375979E-6));
#45720=CARTESIAN_POINT('Ctrl Pts',(-6.00000000001697,-19.5919329102801,
0.135482829560807));
#45721=CARTESIAN_POINT('Ctrl Pts',(-6.00000000001005,-19.5919459863973,
0.131581789353999));
#45722=CARTESIAN_POINT('Ctrl Pts',(-6.00000000000347,-19.5919585088244,
0.127680725310898));
#45723=CARTESIAN_POINT('Ctrl Pts',(-5.9999999999973,-19.5919704756413,0.123779639821488));
#45724=CARTESIAN_POINT('Ctrl Pts',(-5.99999999993208,-19.592097039782,0.0825207541337165));
#45725=CARTESIAN_POINT('Ctrl Pts',(-5.99999999990817,-19.5921614523066,
0.0412594672354874));
#45726=CARTESIAN_POINT('Ctrl Pts',(-5.99999999990817,-19.5921614509454,
-1.42316775524837E-6));
#45727=CARTESIAN_POINT('Ctrl Pts',(-5.99999999990817,-19.5921614495841,
-0.0412621564085699));
#45728=CARTESIAN_POINT('Ctrl Pts',(-5.99999999993208,-19.5920970348271,
-0.082522493401898));
#45729=CARTESIAN_POINT('Ctrl Pts',(-5.9999999999973,-19.5919704760377,-0.123779639519363));
#45730=CARTESIAN_POINT('Ctrl Pts',(-6.00000000000346,-19.5919585091991,
-0.127680732537362));
#45731=CARTESIAN_POINT('Ctrl Pts',(-6.00000000001004,-19.5919459867691,
-0.131581797046985));
#45732=CARTESIAN_POINT('Ctrl Pts',(-6.00000000001697,-19.591932910674,-0.135482830660537));
#45733=CARTESIAN_POINT('Ctrl Pts',(-5.67775659315864,-19.9920104400695,
0.353201969755379));
#45734=CARTESIAN_POINT('Ctrl Pts',(-3.78517106210576,-19.9513454585501,
1.27015806410654));
#45735=CARTESIAN_POINT('Ctrl Pts',(-2.07350540383511E-10,-19.8989940825525,
2.18677316177469));
#45736=CARTESIAN_POINT('Ctrl Pts',(3.7851710616912,-19.9513454585464,1.27015806419779));
#45737=CARTESIAN_POINT('Ctrl Pts',(5.67775659253729,-19.9920104400553,0.353201970057756));
#45738=CARTESIAN_POINT('Ctrl Pts',(-5.67775659315864,-19.9939858021668,
0.127302152333014));
#45739=CARTESIAN_POINT('Ctrl Pts',(-3.78517106210576,-19.9624099274875,
0.457989911116222));
#45740=CARTESIAN_POINT('Ctrl Pts',(-2.07350540383511E-10,-20.07929286279,
0.79322766033635));
#45741=CARTESIAN_POINT('Ctrl Pts',(3.7851710616912,-19.9624099274969,0.457989911150634));
#45742=CARTESIAN_POINT('Ctrl Pts',(5.67775659253729,-19.9939858021509,0.127302152445153));
#45743=CARTESIAN_POINT('Ctrl Pts',(-5.67775659315864,-19.9940658453786,
-0.0986748542825062));
#45744=CARTESIAN_POINT('Ctrl Pts',(-3.78517106210576,-19.9628582683932,
-0.355018823012134));
#45745=CARTESIAN_POINT('Ctrl Pts',(-2.07350540383511E-10,-20.0865987098241,
-0.615372372365866));
#45746=CARTESIAN_POINT('Ctrl Pts',(3.7851710616912,-19.9628582684084,-0.355018823042515));
#45747=CARTESIAN_POINT('Ctrl Pts',(5.67775659253729,-19.9940658453618,-0.0986748543637739));
#45748=CARTESIAN_POINT('Ctrl Pts',(-5.67775659315864,-19.9922505697091,
-0.324580927234301));
#45749=CARTESIAN_POINT('Ctrl Pts',(-3.78517106210576,-19.95269048127,-1.16725509800203));
#45750=CARTESIAN_POINT('Ctrl Pts',(-2.07350540383511E-10,-19.9209116236529,
-2.01013791647348));
#45751=CARTESIAN_POINT('Ctrl Pts',(3.7851710616912,-19.9526904812655,-1.16725509809374));
#45752=CARTESIAN_POINT('Ctrl Pts',(5.67775659253729,-19.9922505696944,-0.324580927510664));
#45753=CARTESIAN_POINT('Ctrl Pts',(-5.5933616962571,-19.9918770425183,0.136828655319151));
#45754=CARTESIAN_POINT('Ctrl Pts',(-5.58012472919481,-19.99163674265,0.142971485509285));
#45755=CARTESIAN_POINT('Ctrl Pts',(-5.56080272347521,-19.9912875756678,
0.151932544276364));
#45756=CARTESIAN_POINT('Ctrl Pts',(-5.53535952182951,-19.9908363415534,
0.163638016329727));
#45757=CARTESIAN_POINT('Ctrl Pts',(-5.51000522444049,-19.9903866841523,
0.175302586836719));
#45758=CARTESIAN_POINT('Ctrl Pts',(-5.47857227855432,-19.989835793103,0.189692500930799));
#45759=CARTESIAN_POINT('Ctrl Pts',(-5.44100422143108,-19.9891930595044,
0.2066874873172));
#45760=CARTESIAN_POINT('Ctrl Pts',(-5.41357576116322,-19.9887237993318,
0.21909553672266));
#45761=CARTESIAN_POINT('Ctrl Pts',(-5.38287654985487,-19.9882056556176,
0.232891249080397));
#45762=CARTESIAN_POINT('Ctrl Pts',(-5.34887846376692,-19.9876425066992,
0.24801136658331));
#45763=CARTESIAN_POINT('Ctrl Pts',(-5.30328327368837,-19.9868872617741,
0.268289114859251));
#45764=CARTESIAN_POINT('Ctrl Pts',(-5.25175535678456,-19.9860510323723,
0.29095083654136));
#45765=CARTESIAN_POINT('Ctrl Pts',(-5.1942123821824,-19.9851444278923,0.315802052049564));
#45766=CARTESIAN_POINT('Ctrl Pts',(-5.1577545619446,-19.9845700254846,0.331547173916361));
#45767=CARTESIAN_POINT('Ctrl Pts',(-5.11888187229187,-19.9839673843954,
0.34817024080352));
#45768=CARTESIAN_POINT('Ctrl Pts',(-5.07757050665736,-19.9833390403789,
0.365611308779708));
#45769=CARTESIAN_POINT('Ctrl Pts',(-5.0142792917611,-19.982376383842,0.392331954886338));
#45770=CARTESIAN_POINT('Ctrl Pts',(-4.94526457323561,-19.9813533518089,
0.420975101801376));
#45771=CARTESIAN_POINT('Ctrl Pts',(-4.87043008439426,-19.9802806585483,
0.451284577322271));
#45772=CARTESIAN_POINT('Ctrl Pts',(-4.84061248935803,-19.9798532468864,
0.463361303987141));
#45773=CARTESIAN_POINT('Ctrl Pts',(-4.80987082635485,-19.9794179489913,
0.475702019067311));
#45774=CARTESIAN_POINT('Ctrl Pts',(-4.77819856292879,-19.9789754207395,
0.488288233952837));
#45775=CARTESIAN_POINT('Ctrl Pts',(-4.70106309934213,-19.9778976757931,
0.518941032805151));
#45776=CARTESIAN_POINT('Ctrl Pts',(-4.61840846663568,-19.9767770032238,
0.55105350273108));
#45777=CARTESIAN_POINT('Ctrl Pts',(-4.53013413330441,-19.9756247259809,
0.58432325758402));
#45778=CARTESIAN_POINT('Ctrl Pts',(-4.50292955806877,-19.9752696146846,
0.594576402692142));
#45779=CARTESIAN_POINT('Ctrl Pts',(-4.47519119417953,-19.9749115039132,
0.604939096084163));
#45780=CARTESIAN_POINT('Ctrl Pts',(-4.44691597456336,-19.9745507289419,
0.615401484750342));
#45781=CARTESIAN_POINT('Ctrl Pts',(-4.3578107093497,-19.9734137987985,0.648372189470696));
#45782=CARTESIAN_POINT('Ctrl Pts',(-4.26337415693458,-19.9722503419874,
0.682336805905467));
#45783=CARTESIAN_POINT('Ctrl Pts',(-4.16350818045132,-19.9710726185038,
0.716953903297154));
#45784=CARTESIAN_POINT('Ctrl Pts',(-4.13544195145048,-19.9707416323346,
0.726682655940978));
#45785=CARTESIAN_POINT('Ctrl Pts',(-4.1069468718516,-19.9704095241886,0.736462630533679));
#45786=CARTESIAN_POINT('Ctrl Pts',(-4.07802072641322,-19.9700765770652,
0.74628549838169));
#45787=CARTESIAN_POINT('Ctrl Pts',(-3.98959650005386,-19.9690587922426,
0.776312986556394));
#45788=CARTESIAN_POINT('Ctrl Pts',(-3.89714408537845,-19.968033114597,0.806743604209373));
#45789=CARTESIAN_POINT('Ctrl Pts',(-3.80060148807689,-19.9670086332002,
0.837319610561497));
#45790=CARTESIAN_POINT('Ctrl Pts',(-3.75616522180159,-19.9665370887275,
0.851393020619588));
#45791=CARTESIAN_POINT('Ctrl Pts',(-3.71086243987753,-19.9660658070662,
0.865496800800391));
#45792=CARTESIAN_POINT('Ctrl Pts',(-3.66468717719672,-19.965595723055,0.87960351915793));
#45793=CARTESIAN_POINT('Ctrl Pts',(-3.62904937773455,-19.9652329149462,
0.890491002427281));
#45794=CARTESIAN_POINT('Ctrl Pts',(-3.59289187019038,-19.9648708206383,
0.901380206343566));
#45795=CARTESIAN_POINT('Ctrl Pts',(-3.55621207182732,-19.9645098984448,
0.912257972988526));
#45796=CARTESIAN_POINT('Ctrl Pts',(-3.51410949158726,-19.9640956171159,
0.924743920661103));
#45797=CARTESIAN_POINT('Ctrl Pts',(-3.4713187055698,-19.9636828722794,0.937215022091883));
#45798=CARTESIAN_POINT('Ctrl Pts',(-3.42783597968764,-19.9632723869592,
0.949650254350777));
#45799=CARTESIAN_POINT('Ctrl Pts',(-3.40609461674657,-19.9630671442991,
0.955867870480223));
#45800=CARTESIAN_POINT('Ctrl Pts',(-3.38418026883877,-19.9628624663561,
0.962076519309465));
#45801=CARTESIAN_POINT('Ctrl Pts',(-3.36209246653124,-19.9626584445229,
0.968273515281171));
#45802=CARTESIAN_POINT('Ctrl Pts',(-3.35104856537748,-19.9625564336064,
0.971372013267024));
#45803=CARTESIAN_POINT('Ctrl Pts',(-3.33996130062377,-19.9624545867031,
0.974467598037997));
#45804=CARTESIAN_POINT('Ctrl Pts',(-3.32883061483636,-19.9623529153641,
0.977559928309276));
#45805=CARTESIAN_POINT('Ctrl Pts',(-3.32326527194265,-19.9623020796946,
0.979106093444916));
#45806=CARTESIAN_POINT('Ctrl Pts',(-3.31768907379052,-19.9622512879152,
0.980651444955594));
#45807=CARTESIAN_POINT('Ctrl Pts',(-3.31210201325294,-19.9622005414794,
0.982195939788543));
#45808=CARTESIAN_POINT('Ctrl Pts',(-3.30651495271535,-19.9621497950436,
0.983740434621492));
#45809=CARTESIAN_POINT('Ctrl Pts',(-3.30209405065048,-19.9621097238955,
0.984960324852798));
#45810=CARTESIAN_POINT('Ctrl Pts',(-3.29530823737352,-19.9620484396568,
0.986826811081932));
#45811=CARTESIAN_POINT('Ctrl Pts',(-3.26371351551596,-19.9617631004648,
0.995517164154379));
#45812=CARTESIAN_POINT('Ctrl Pts',(-3.23221976327874,-19.9614833155026,
1.00405525712431));
#45813=CARTESIAN_POINT('Ctrl Pts',(-3.20082837943391,-19.9612089854768,
1.01244306424384));
#45814=CARTESIAN_POINT('Ctrl Pts',(-3.02529692306615,-19.9596750120403,
1.05934523353657));
#45815=CARTESIAN_POINT('Ctrl Pts',(-2.85296934932615,-19.9583115521099,
1.10154715968608));
#45816=CARTESIAN_POINT('Ctrl Pts',(-2.68408332990121,-19.957101515053,1.13941645657479));
#45817=CARTESIAN_POINT('Ctrl Pts',(-2.50184473349649,-19.9557958092545,
1.18027980059422));
#45818=CARTESIAN_POINT('Ctrl Pts',(-2.32361410663327,-19.9546686989974,
1.21609906014452));
#45819=CARTESIAN_POINT('Ctrl Pts',(-2.14965775902324,-19.9536981810796,
1.24737014880551));
#45820=CARTESIAN_POINT('Ctrl Pts',(-2.13682704255917,-19.9536265973725,
1.24967664970441));
#45821=CARTESIAN_POINT('Ctrl Pts',(-2.12401955626893,-19.9535558661227,
1.25195841043766));
#45822=CARTESIAN_POINT('Ctrl Pts',(-2.1112353961309,-19.9534859787631,1.25421563135693));
#45823=CARTESIAN_POINT('Ctrl Pts',(-1.93625472138247,-19.952529409288,1.28511089825319));
#45824=CARTESIAN_POINT('Ctrl Pts',(-1.76564842135957,-19.9517307494261,
1.31140933237227));
#45825=CARTESIAN_POINT('Ctrl Pts',(-1.59964960695838,-19.9510660439799,
1.33364778692522));
#45826=CARTESIAN_POINT('Ctrl Pts',(-1.55747659209,-19.9508971714927,1.33929760242477));
#45827=CARTESIAN_POINT('Ctrl Pts',(-1.51560070355459,-19.9507369561823,
1.34468533408111));
#45828=CARTESIAN_POINT('Ctrl Pts',(-1.47402524339339,-19.9505850276501,
1.34981970536911));
#45829=CARTESIAN_POINT('Ctrl Pts',(-1.30954622608724,-19.9499839746354,
1.37013208052167));
#45830=CARTESIAN_POINT('Ctrl Pts',(-1.14977310823239,-19.9495123677062,
1.38648080161668));
#45831=CARTESIAN_POINT('Ctrl Pts',(-0.994888669132556,-19.9491460309321,
1.39942188067988));
#45832=CARTESIAN_POINT('Ctrl Pts',(-0.923054604482982,-19.9489761271015,
1.40542384133819));
#45833=CARTESIAN_POINT('Ctrl Pts',(-0.85227141748989,-19.9488289113757,
1.41069250714498));
#45834=CARTESIAN_POINT('Ctrl Pts',(-0.782553962151891,-19.9487021923061,
1.41528169882576));
#45835=CARTESIAN_POINT('Ctrl Pts',(-0.633225993292338,-19.9484307724559,
1.42511129844432));
#45836=CARTESIAN_POINT('Ctrl Pts',(-0.488789989415151,-19.9482530035993,
1.43182610541899));
#45837=CARTESIAN_POINT('Ctrl Pts',(-0.349367810876151,-19.948143898493,
1.43595869572865));
#45838=CARTESIAN_POINT('Ctrl Pts',(-0.262283845607513,-19.9480757507608,
1.43853993749927));
#45839=CARTESIAN_POINT('Ctrl Pts',(-0.177155096851432,-19.9480344970638,
1.44011308848701));
#45840=CARTESIAN_POINT('Ctrl Pts',(-0.0940037411794105,-19.948015009502,
1.44080102246092));
#45841=CARTESIAN_POINT('Ctrl Pts',(0.0408033074116613,-19.9479834157815,
1.44191631815152));
#45842=CARTESIAN_POINT('Ctrl Pts',(0.170411318462979,-19.9480093421139,
1.44070714992397));
#45843=CARTESIAN_POINT('Ctrl Pts',(0.294749903916067,-19.9480858766655,
1.43767293836567));
#45844=CARTESIAN_POINT('Ctrl Pts',(0.343180995220454,-19.9481156876195,
1.4364910833809));
#45845=CARTESIAN_POINT('Ctrl Pts',(0.390812983906775,-19.9481531567733,
1.43503190092335));
#45846=CARTESIAN_POINT('Ctrl Pts',(0.437643016283311,-19.9481978063411,
1.43332323677407));
#45847=CARTESIAN_POINT('Ctrl Pts',(0.474088859801895,-19.9482325552208,
1.43199345536992));
#45848=CARTESIAN_POINT('Ctrl Pts',(0.510048984651785,-19.9482716524046,
1.43051254789329));
#45849=CARTESIAN_POINT('Ctrl Pts',(0.545522325919625,-19.948314859256,1.42889324789818));
#45850=CARTESIAN_POINT('Ctrl Pts',(0.575342930585281,-19.948351181023,1.42753198608118));
#45851=CARTESIAN_POINT('Ctrl Pts',(0.604819536025602,-19.9483904067925,
1.42607291952875));
#45852=CARTESIAN_POINT('Ctrl Pts',(0.633951737248377,-19.9484323866779,
1.42452357218047));
#45853=CARTESIAN_POINT('Ctrl Pts',(0.665845060554363,-19.9484783453766,
1.42282737917692));
#45854=CARTESIAN_POINT('Ctrl Pts',(0.697325522058463,-19.948527604552,1.42102299411122));
#45855=CARTESIAN_POINT('Ctrl Pts',(0.728392805781448,-19.9485799624068,
1.41912001321096));
#45856=CARTESIAN_POINT('Ctrl Pts',(0.743926447642939,-19.9486061413342,
1.41816852276083));
#45857=CARTESIAN_POINT('Ctrl Pts',(0.759356795058225,-19.9486330945423,
1.41719238332444));
#45858=CARTESIAN_POINT('Ctrl Pts',(0.774683802833065,-19.9486607965246,
1.41619276610858));
#45859=CARTESIAN_POINT('Ctrl Pts',(0.782347306720485,-19.9486746475157,
1.41569295750065));
#45860=CARTESIAN_POINT('Ctrl Pts',(0.78998497569773,-19.948688685677,1.41518727944621));
#45861=CARTESIAN_POINT('Ctrl Pts',(0.797596805412144,-19.94870290775,1.41467587730628));
#45862=CARTESIAN_POINT('Ctrl Pts',(0.805208635126558,-19.948717129823,1.41416447516635));
#45863=CARTESIAN_POINT('Ctrl Pts',(0.81455809586776,-19.9487349382461,1.41352542345741));
#45864=CARTESIAN_POINT('Ctrl Pts',(0.820354772636643,-19.9487461223901,
1.41312464346554));
#45865=CARTESIAN_POINT('Ctrl Pts',(0.913219559701145,-19.9489252962841,
1.40670400797247));
#45866=CARTESIAN_POINT('Ctrl Pts',(1.01097505164935,-19.9491467067125,1.39886195763818));
#45867=CARTESIAN_POINT('Ctrl Pts',(1.1135640324211,-19.9494231953357,1.38924936584772));
#45868=CARTESIAN_POINT('Ctrl Pts',(1.22619399111071,-19.9497267455022,1.37869593400625));
#45869=CARTESIAN_POINT('Ctrl Pts',(1.34465071383681,-19.9500967037675,1.36600849025799));
#45870=CARTESIAN_POINT('Ctrl Pts',(1.46882938107773,-19.9505511703804,1.35069212718216));
#45871=CARTESIAN_POINT('Ctrl Pts',(1.51533015773198,-19.9507213529965,1.34495665913141));
#45872=CARTESIAN_POINT('Ctrl Pts',(1.56263295566258,-19.9509034123575,1.33885215798398));
#45873=CARTESIAN_POINT('Ctrl Pts',(1.6107309717886,-19.9510983971473,1.33235126464855));
#45874=CARTESIAN_POINT('Ctrl Pts',(1.74016072627675,-19.9516230930807,1.31485763193504));
#45875=CARTESIAN_POINT('Ctrl Pts',(1.87535188685385,-19.9522412101344,1.29449569857747));
#45876=CARTESIAN_POINT('Ctrl Pts',(2.01614804957389,-19.9529740117998,1.27071914141072));
#45877=CARTESIAN_POINT('Ctrl Pts',(2.02946099004117,-19.9530433016494,1.2684709559207));
#45878=CARTESIAN_POINT('Ctrl Pts',(2.04282401054921,-19.9531136187254,1.26619222015002));
#45879=CARTESIAN_POINT('Ctrl Pts',(2.05623695835842,-19.9531849821918,1.26388245908358));
#45880=CARTESIAN_POINT('Ctrl Pts',(2.18613474459512,-19.9538761021776,1.24151356198998));
#45881=CARTESIAN_POINT('Ctrl Pts',(2.32071794588983,-19.9546652443161,1.21623591885326));
#45882=CARTESIAN_POINT('Ctrl Pts',(2.45983349748496,-19.9555696850239,1.18761773855746));
#45883=CARTESIAN_POINT('Ctrl Pts',(2.57754555067168,-19.9563349738178,1.16340258272146));
#45884=CARTESIAN_POINT('Ctrl Pts',(2.69850206719957,-19.9571828472084,1.13679523393321));
#45885=CARTESIAN_POINT('Ctrl Pts',(2.82259417732612,-19.958124134521,1.10753308187823));
#45886=CARTESIAN_POINT('Ctrl Pts',(2.92928969165264,-19.958933461833,1.08237321989649));
#45887=CARTESIAN_POINT('Ctrl Pts',(3.03830297462944,-19.9598118612748,1.05525055320977));
#45888=CARTESIAN_POINT('Ctrl Pts',(3.14955604559989,-19.9607663936939,1.02599991467783));
#45889=CARTESIAN_POINT('Ctrl Pts',(3.24644396496343,-19.9615976755565,1.00052615936759));
#45890=CARTESIAN_POINT('Ctrl Pts',(3.34503044467376,-19.9624867037711,0.973438421394531));
#45891=CARTESIAN_POINT('Ctrl Pts',(3.44525913621966,-19.9634382995461,0.944629727965889));
#45892=CARTESIAN_POINT('Ctrl Pts',(3.44870611911616,-19.963471026047,0.943638963026355));
#45893=CARTESIAN_POINT('Ctrl Pts',(3.45215504374027,-19.9635038265659,0.942646162746129));
#45894=CARTESIAN_POINT('Ctrl Pts',(3.45560590773787,-19.963536701306,0.94165132284774));
#45895=CARTESIAN_POINT('Ctrl Pts',(3.53367153282903,-19.9642803953891,0.919146002850343));
#45896=CARTESIAN_POINT('Ctrl Pts',(3.61272983141187,-19.9650620670969,0.895596831425127));
#45897=CARTESIAN_POINT('Ctrl Pts',(3.69275236865053,-19.9658841047799,0.870954669388449));
#45898=CARTESIAN_POINT('Ctrl Pts',(3.69944558974584,-19.9659528614096,0.868893557050984));
#45899=CARTESIAN_POINT('Ctrl Pts',(3.706145556583,-19.9660219004815,0.866824798522152));
#45900=CARTESIAN_POINT('Ctrl Pts',(3.71285225154802,-19.966091223414,0.864748365335758));
#45901=CARTESIAN_POINT('Ctrl Pts',(3.74623737037075,-19.9664363046125,0.854412131316357));
#45902=CARTESIAN_POINT('Ctrl Pts',(3.77978921264104,-19.9667884194618,0.843885722316286));
#45903=CARTESIAN_POINT('Ctrl Pts',(3.81350561990606,-19.9671477526821,0.833165672987393));
#45904=CARTESIAN_POINT('Ctrl Pts',(3.83375044708249,-19.9673635122939,0.82672887963986));
#45905=CARTESIAN_POINT('Ctrl Pts',(3.8540546057761,-19.9675818744595,0.820222271796804));
#45906=CARTESIAN_POINT('Ctrl Pts',(3.87441762676972,-19.967802879636,0.813645104648946));
#45907=CARTESIAN_POINT('Ctrl Pts',(3.88459913726653,-19.9679133822243,0.810356521075018));
#45908=CARTESIAN_POINT('Ctrl Pts',(3.89479536333834,-19.968024545573,0.807050297675153));
#45909=CARTESIAN_POINT('Ctrl Pts',(3.90500624519459,-19.9681363747775,0.803726341583876));
#45910=CARTESIAN_POINT('Ctrl Pts',(3.91011168612271,-19.9681922893797,0.802064363538237));
#45911=CARTESIAN_POINT('Ctrl Pts',(3.91522079099694,-19.9682483704464,0.800397952319758));
#45912=CARTESIAN_POINT('Ctrl Pts',(3.92033355229372,-19.9683046186163,0.798727096350555));
#45913=CARTESIAN_POINT('Ctrl Pts',(3.92544631359051,-19.9683608667862,0.797056240381352));
#45914=CARTESIAN_POINT('Ctrl Pts',(3.93232800683171,-19.9684367905194,0.79480179993151));
#45915=CARTESIAN_POINT('Ctrl Pts',(3.9356827979111,-19.9684738650762,0.793701182621356));
#45916=CARTESIAN_POINT('Ctrl Pts',(3.94201776596352,-19.9685438742444,0.791622848879327));
#45917=CARTESIAN_POINT('Ctrl Pts',(3.94833529221475,-19.9686138847017,0.789545282538373));
#45918=CARTESIAN_POINT('Ctrl Pts',(3.95463539436655,-19.9686838938132,0.787468559316938));
#45919=CARTESIAN_POINT('Ctrl Pts',(4.02984793005298,-19.9695196838803,0.762676005856775));
#45920=CARTESIAN_POINT('Ctrl Pts',(4.10257711980881,-19.9703552659729,0.7380045802307));
#45921=CARTESIAN_POINT('Ctrl Pts',(4.1728536855241,-19.9711864277094,0.713576948003457));
#45922=CARTESIAN_POINT('Ctrl Pts',(4.24078041990787,-19.9719897979641,0.689966100361207));
#45923=CARTESIAN_POINT('Ctrl Pts',(4.30641583373046,-19.9727890443001,0.666582917234265));
#45924=CARTESIAN_POINT('Ctrl Pts',(4.36978780546687,-19.9735806927637,0.643528252680029));
#45925=CARTESIAN_POINT('Ctrl Pts',(4.43123718177006,-19.9743483239894,0.621173026561618));
#45926=CARTESIAN_POINT('Ctrl Pts',(4.49055838824294,-19.9751088167531,0.599126610536702));
#45927=CARTESIAN_POINT('Ctrl Pts',(4.54777651242298,-19.9758592774546,0.577472662590279));
#45928=CARTESIAN_POINT('Ctrl Pts',(4.60352991899979,-19.9765905272327,0.556373030591668));
#45929=CARTESIAN_POINT('Ctrl Pts',(4.65728654863231,-19.9773122570472,0.535645970642595));
#45930=CARTESIAN_POINT('Ctrl Pts',(4.70906899455022,-19.9780220136423,0.515361826729719));
#45931=CARTESIAN_POINT('Ctrl Pts',(4.75988646514747,-19.9787185437938,0.495455681536865));
#45932=CARTESIAN_POINT('Ctrl Pts',(4.80880265137162,-19.9794035476555,0.475976054196603));
#45933=CARTESIAN_POINT('Ctrl Pts',(4.85583810555937,-19.9800748867969,0.45698327080129));
#45934=CARTESIAN_POINT('Ctrl Pts',(4.90206734298214,-19.9807347187704,0.438316035455873));
#45935=CARTESIAN_POINT('Ctrl Pts',(4.94647977271578,-19.9813813550584,0.420119060257995));
#45936=CARTESIAN_POINT('Ctrl Pts',(4.9890939954169,-19.9820129039542,0.402444197157457));
#45937=CARTESIAN_POINT('Ctrl Pts',(4.98946317908515,-19.9820183753092,0.402291072909692));
#45938=CARTESIAN_POINT('Ctrl Pts',(4.98983222778481,-19.9820238455311,0.402137987816611));
#45939=CARTESIAN_POINT('Ctrl Pts',(4.9902011415277,-19.9820293146189,0.401984941910257));
#45940=CARTESIAN_POINT('Ctrl Pts',(5.03326624102464,-19.9826677478928,0.384119147231026));
#45941=CARTESIAN_POINT('Ctrl Pts',(5.0744923583959,-19.9832907382138,0.366787777783412));
#45942=CARTESIAN_POINT('Ctrl Pts',(5.11389765669138,-19.9838964340089,0.350039136630992));
#45943=CARTESIAN_POINT('Ctrl Pts',(5.15370169359892,-19.9845082587844,0.33312101750947));
#45944=CARTESIAN_POINT('Ctrl Pts',(5.19164787976516,-19.9851024422408,0.316797468369802));
#45945=CARTESIAN_POINT('Ctrl Pts',(5.22775373276918,-19.9856771422,0.301113068622864));
#45946=CARTESIAN_POINT('Ctrl Pts',(5.26453890956988,-19.9862626550142,0.285133570294995));
#45947=CARTESIAN_POINT('Ctrl Pts',(5.29941385696856,-19.9868279488227,0.269817495334042));
#45948=CARTESIAN_POINT('Ctrl Pts',(5.33239574607363,-19.9873710979507,0.255206700780277));
#45949=CARTESIAN_POINT('Ctrl Pts',(5.36640991150646,-19.987931246711,0.2401386135196));
#45950=CARTESIAN_POINT('Ctrl Pts',(5.39841067725307,-19.9884678461484,0.225820654257808));
#45951=CARTESIAN_POINT('Ctrl Pts',(5.42841530804753,-19.9889787612015,0.212293095298047));
#45952=CARTESIAN_POINT('Ctrl Pts',(5.4599627399709,-19.9895159468767,0.198069965931917));
#45953=CARTESIAN_POINT('Ctrl Pts',(5.48930350818925,-19.9900247389058,0.184720640340341));
#45954=CARTESIAN_POINT('Ctrl Pts',(5.51645571937383,-19.9905025966942,0.172285432958562));
#45955=CARTESIAN_POINT('Ctrl Pts',(5.54440396445813,-19.9909944640597,0.159485656866014));
#45956=CARTESIAN_POINT('Ctrl Pts',(5.57003347911907,-19.9914535484999,0.147654394959246));
#45957=CARTESIAN_POINT('Ctrl Pts',(5.59336166001797,-19.9918770419854,0.136828574222652));
#45958=CARTESIAN_POINT('Ctrl Pts',(-5.84637332561518,-19.8012032245096,
0.398518228706042));
#45959=CARTESIAN_POINT('Ctrl Pts',(-5.81071186290306,-19.8004233834171,
0.41520737060269));
#45960=CARTESIAN_POINT('Ctrl Pts',(-5.69191724351161,-19.797880036612,0.470271235481794));
#45961=CARTESIAN_POINT('Ctrl Pts',(-5.48049048458094,-19.7936450596294,
0.565146741690545));
#45962=CARTESIAN_POINT('Ctrl Pts',(-5.20214452284485,-19.7884998191918,
0.68405291707163));
#45963=CARTESIAN_POINT('Ctrl Pts',(-4.89413796055143,-19.7832359786177,
0.80835770933709));
#45964=CARTESIAN_POINT('Ctrl Pts',(-4.55276036907155,-19.7778647893813,
0.937269633545895));
#45965=CARTESIAN_POINT('Ctrl Pts',(-4.17237911340894,-19.7724099073617,
1.06997883011475));
#45966=CARTESIAN_POINT('Ctrl Pts',(-3.74657608413542,-19.7669368130706,
1.20488312141804));
#45967=CARTESIAN_POINT('Ctrl Pts',(-3.27004596375486,-19.7615847658559,
1.33873580301228));
#45968=CARTESIAN_POINT('Ctrl Pts',(-2.7387201600104,-19.7565630655646,1.4666394592086));
#45969=CARTESIAN_POINT('Ctrl Pts',(-2.14782149463107,-19.7521260156702,
1.58251297890624));
#45970=CARTESIAN_POINT('Ctrl Pts',(-1.49674277411264,-19.7486061536723,
1.6779232271702));
#45971=CARTESIAN_POINT('Ctrl Pts',(-0.805541188049843,-19.746389950329,
1.7416146737656));
#45972=CARTESIAN_POINT('Ctrl Pts',(-0.113422498758484,-19.7456264454589,
1.76632910849782));
#45973=CARTESIAN_POINT('Ctrl Pts',(0.536119675471227,-19.7459828406868,
1.75439019730121));
#45974=CARTESIAN_POINT('Ctrl Pts',(1.11982241639085,-19.7473094854822,1.71489595544031));
#45975=CARTESIAN_POINT('Ctrl Pts',(1.63691910409778,-19.7493621956864,1.65738874956046));
#45976=CARTESIAN_POINT('Ctrl Pts',(2.09764987887928,-19.7519182415327,1.58837871802467));
#45977=CARTESIAN_POINT('Ctrl Pts',(2.51229038328305,-19.7548277285975,1.51185825784502));
#45978=CARTESIAN_POINT('Ctrl Pts',(2.8862805445336,-19.7579580036799,1.43110355046616));
#45979=CARTESIAN_POINT('Ctrl Pts',(3.22330033713463,-19.7611952123647,1.34881182009632));
#45980=CARTESIAN_POINT('Ctrl Pts',(3.52771849241463,-19.7644627557382,1.26671644234715));
#45981=CARTESIAN_POINT('Ctrl Pts',(3.80296220780623,-19.7677012652864,1.18613702323411));
#45982=CARTESIAN_POINT('Ctrl Pts',(4.05167352309718,-19.7708626842596,1.10813376736068));
#45983=CARTESIAN_POINT('Ctrl Pts',(4.27619687672365,-19.7739112820015,1.03348278511119));
#45984=CARTESIAN_POINT('Ctrl Pts',(4.47888810581092,-19.7768251650753,0.962639383477481));
#45985=CARTESIAN_POINT('Ctrl Pts',(4.66210367547018,-19.7795944348557,0.895783474658922));
#45986=CARTESIAN_POINT('Ctrl Pts',(4.82816201172659,-19.782218972549,0.83287332055465));
#45987=CARTESIAN_POINT('Ctrl Pts',(4.9793040978404,-19.784706262591,0.77369827621928));
#45988=CARTESIAN_POINT('Ctrl Pts',(5.11759466992664,-19.7870683576696,0.717952243040958));
#45989=CARTESIAN_POINT('Ctrl Pts',(5.24463568621137,-19.7893154089871,0.665386419186038));
#45990=CARTESIAN_POINT('Ctrl Pts',(5.3615195899783,-19.7914527440325,0.615872671561029));
#45991=CARTESIAN_POINT('Ctrl Pts',(5.46894761080408,-19.7934811813725,0.569388237748869));
#45992=CARTESIAN_POINT('Ctrl Pts',(5.56755786506634,-19.795402135003,0.525892474641232));
#45993=CARTESIAN_POINT('Ctrl Pts',(5.65799402501198,-19.7972185803945,0.485302861498154));
#45994=CARTESIAN_POINT('Ctrl Pts',(5.74090216955938,-19.7989347556667,0.447500470475536));
#45995=CARTESIAN_POINT('Ctrl Pts',(5.80283684827997,-19.8002553617805,0.418853196576111));
#45996=CARTESIAN_POINT('Ctrl Pts',(5.83721009892043,-19.8010035313691,0.402805975572136));
#45997=CARTESIAN_POINT('Ctrl Pts',(5.84634760404617,-19.8012035243102,0.398529618156887));
#45998=CARTESIAN_POINT('Ctrl Pts',(-5.81214087242335,-19.9271873066255,
0.330204210423679));
#45999=CARTESIAN_POINT('Ctrl Pts',(-5.77669421382378,-19.9264341811936,
0.346835037585213));
#46000=CARTESIAN_POINT('Ctrl Pts',(-5.65860674649306,-19.9239789090011,
0.401710664034115));
#46001=CARTESIAN_POINT('Ctrl Pts',(-5.44839807624833,-19.9198953659561,
0.496281732480572));
#46002=CARTESIAN_POINT('Ctrl Pts',(-5.17161876013454,-19.9149409583558,
0.614825658279969));
#46003=CARTESIAN_POINT('Ctrl Pts',(-4.86533505608267,-19.909878877687,0.7387605376848));
#46004=CARTESIAN_POINT('Ctrl Pts',(-4.52587295649738,-19.9047199784787,
0.867291774518096));
#46005=CARTESIAN_POINT('Ctrl Pts',(-4.14764429923081,-19.8994872295208,
0.99960842331503));
#46006=CARTESIAN_POINT('Ctrl Pts',(-3.72427883488178,-19.8942438262849,
1.13411085093911));
#46007=CARTESIAN_POINT('Ctrl Pts',(-3.25051249031194,-19.8891235326155,
1.26756067629006));
#46008=CARTESIAN_POINT('Ctrl Pts',(-2.72230931503972,-19.8843266474812,
1.39507475420067));
#46009=CARTESIAN_POINT('Ctrl Pts',(-2.1349256811288,-19.8800956328736,1.51059101517757));
#46010=CARTESIAN_POINT('Ctrl Pts',(-1.48775542564675,-19.876746360621,1.60570392250982));
#46011=CARTESIAN_POINT('Ctrl Pts',(-0.800722870452506,-19.8746435601401,
1.66919556666686));
#46012=CARTESIAN_POINT('Ctrl Pts',(-0.112751530308937,-19.8739229914661,
1.69383291987766));
#46013=CARTESIAN_POINT('Ctrl Pts',(0.532923322865208,-19.8742588033861,
1.68193113155805));
#46014=CARTESIAN_POINT('Ctrl Pts',(1.11310674871294,-19.875515597709,1.64256070755316));
#46015=CARTESIAN_POINT('Ctrl Pts',(1.62709029937881,-19.8774656632708,1.58523349554965));
#46016=CARTESIAN_POINT('Ctrl Pts',(2.08505695577575,-19.8798984167727,1.51643825624151));
#46017=CARTESIAN_POINT('Ctrl Pts',(2.49722536838503,-19.8826716687465,1.44015424964475));
#46018=CARTESIAN_POINT('Ctrl Pts',(2.86900237522437,-19.8856590909154,1.35964711728455));
#46019=CARTESIAN_POINT('Ctrl Pts',(3.20404389672357,-19.8887519187439,1.27760569307259));
#46020=CARTESIAN_POINT('Ctrl Pts',(3.50668982756711,-19.8918767530765,1.1957581658858));
#46021=CARTESIAN_POINT('Ctrl Pts',(3.78034401648963,-19.8949765502608,1.11542038234925));
#46022=CARTESIAN_POINT('Ctrl Pts',(4.02762986002984,-19.8980050099384,1.03764968920657));
#46023=CARTESIAN_POINT('Ctrl Pts',(4.25087514579436,-19.9009275845067,0.963220264239793));
#46024=CARTESIAN_POINT('Ctrl Pts',(4.45241937565161,-19.9037229678009,0.89258647044243));
#46025=CARTESIAN_POINT('Ctrl Pts',(4.63460310816801,-19.9063813646969,0.825928096032151));
#46026=CARTESIAN_POINT('Ctrl Pts',(4.79972950250149,-19.9089023917319,0.763203922014176));
#46027=CARTESIAN_POINT('Ctrl Pts',(4.95002508592934,-19.9112930043664,0.704204306591428));
#46028=CARTESIAN_POINT('Ctrl Pts',(5.08754142435965,-19.9135645911091,0.648624430192096));
#46029=CARTESIAN_POINT('Ctrl Pts',(5.21387010188393,-19.9157267527803,0.596216606190617));
#46030=CARTESIAN_POINT('Ctrl Pts',(5.33009618357311,-19.9177844763503,0.546853461908779));
#46031=CARTESIAN_POINT('Ctrl Pts',(5.43691587105589,-19.9197384200799,0.500512656976851));
#46032=CARTESIAN_POINT('Ctrl Pts',(5.53496282016363,-19.9215898205621,0.457153966966406));
#46033=CARTESIAN_POINT('Ctrl Pts',(5.62487650603923,-19.9233414240886,0.416695315435241));
#46034=CARTESIAN_POINT('Ctrl Pts',(5.70729922003086,-19.9249972011021,0.379018161123265));
#46035=CARTESIAN_POINT('Ctrl Pts',(5.76886605586837,-19.9262719866521,0.350468412781502));
#46036=CARTESIAN_POINT('Ctrl Pts',(5.80303331086259,-19.9269944605838,0.33447675633162));
#46037=CARTESIAN_POINT('Ctrl Pts',(5.81211594933361,-19.927187604253,0.330215260750033));
#46038=CARTESIAN_POINT('Ctrl Pts',(-5.7563773441824,-19.9977612734129,0.213435765605445));
#46039=CARTESIAN_POINT('Ctrl Pts',(-5.72124284761157,-19.9970527865212,
0.229944522484756));
#46040=CARTESIAN_POINT('Ctrl Pts',(-5.60419033028892,-19.9947448867347,
0.284419868696954));
#46041=CARTESIAN_POINT('Ctrl Pts',(-5.39580264092759,-19.9909160146533,
0.378311890771256));
#46042=CARTESIAN_POINT('Ctrl Pts',(-5.12141647166683,-19.9862842137298,
0.496009003059121));
#46043=CARTESIAN_POINT('Ctrl Pts',(-4.81780583433225,-19.9815646423287,
0.61905163753994));
#46044=CARTESIAN_POINT('Ctrl Pts',(-4.48135309706814,-19.976767498175,0.746643501707943));
#46045=CARTESIAN_POINT('Ctrl Pts',(-4.10654376060317,-19.9719146709044,
0.877973972287787));
#46046=CARTESIAN_POINT('Ctrl Pts',(-3.68709091834991,-19.9670655738919,
1.01145112966721));
#46047=CARTESIAN_POINT('Ctrl Pts',(-3.21780670805486,-19.9623446304896,
1.14385873471159));
#46048=CARTESIAN_POINT('Ctrl Pts',(-2.69471979114672,-19.9579366090462,
1.27035198639089));
#46049=CARTESIAN_POINT('Ctrl Pts',(-2.113153523698,-19.9540632878202,1.38492123805317));
#46050=CARTESIAN_POINT('Ctrl Pts',(-1.47251555568381,-19.9510111884615,
1.47923787592944));
#46051=CARTESIAN_POINT('Ctrl Pts',(-0.792512707544035,-19.9491065172301,
1.54218975145515));
#46052=CARTESIAN_POINT('Ctrl Pts',(-0.111600877674484,-19.9484611334256,
1.56661679030302));
#46053=CARTESIAN_POINT('Ctrl Pts',(0.527465568453815,-19.9487608876799,
1.55481654016177));
#46054=CARTESIAN_POINT('Ctrl Pts',(1.10169493934809,-19.9498955386969,1.5157817092239));
#46055=CARTESIAN_POINT('Ctrl Pts',(1.61044354822359,-19.9516664740186,1.45893909693094));
#46056=CARTESIAN_POINT('Ctrl Pts',(2.0637940430478,-19.9538845323556,1.39071840306173));
#46057=CARTESIAN_POINT('Ctrl Pts',(2.47186151969891,-19.956421103771,1.31506249690282));
#46058=CARTESIAN_POINT('Ctrl Pts',(2.8399917317103,-19.9591609446546,1.23520815727489));
#46059=CARTESIAN_POINT('Ctrl Pts',(3.17179488226422,-19.9620041439025,1.15382165859323));
#46060=CARTESIAN_POINT('Ctrl Pts',(3.47155832017755,-19.9648828221612,1.07261750478866));
#46061=CARTESIAN_POINT('Ctrl Pts',(3.74264328259959,-19.9677439052293,0.992901886387031));
#46062=CARTESIAN_POINT('Ctrl Pts',(3.98763901532054,-19.9705440558936,0.915725050081919));
#46063=CARTESIAN_POINT('Ctrl Pts',(4.20884309016115,-19.9732506878429,0.841856595879339));
#46064=CARTESIAN_POINT('Ctrl Pts',(4.40856598483163,-19.9758434281717,0.771748892091009));
#46065=CARTESIAN_POINT('Ctrl Pts',(4.58912056827828,-19.9783125889059,0.705581797064866));
#46066=CARTESIAN_POINT('Ctrl Pts',(4.75278392458491,-19.9806572720839,0.643315711772626));
#46067=CARTESIAN_POINT('Ctrl Pts',(4.90175832814151,-19.982883478262,0.584743714215282));
#46068=CARTESIAN_POINT('Ctrl Pts',(5.03807359660553,-19.9850014227761,0.529564249821708));
#46069=CARTESIAN_POINT('Ctrl Pts',(5.16330433238403,-19.9870197378106,0.477532360449496));
#46070=CARTESIAN_POINT('Ctrl Pts',(5.27852354539555,-19.9889428058235,0.428522451677135));
#46071=CARTESIAN_POINT('Ctrl Pts',(5.38441915349035,-19.9907709904362,0.382513134578401));
#46072=CARTESIAN_POINT('Ctrl Pts',(5.48161746205723,-19.992505207299,0.339465166211689));
#46073=CARTESIAN_POINT('Ctrl Pts',(5.57075099051052,-19.9941477956291,0.299297609682865));
#46074=CARTESIAN_POINT('Ctrl Pts',(5.65245559258702,-19.9957022530114,0.26189312047201));
#46075=CARTESIAN_POINT('Ctrl Pts',(5.71348329895462,-19.9969003461367,0.233551396585078));
#46076=CARTESIAN_POINT('Ctrl Pts',(5.74735040689118,-19.9975798766668,0.217676759133368));
#46077=CARTESIAN_POINT('Ctrl Pts',(5.75635321179484,-19.997761577835,0.213446472193785));
#46078=CARTESIAN_POINT('Ctrl Pts',(-5.69417817153309,-19.9936700926002,
0.0798164952284382));
#46079=CARTESIAN_POINT('Ctrl Pts',(-5.65936864913364,-19.993012084528,0.0961724409863023));
#46080=CARTESIAN_POINT('Ctrl Pts',(-5.54339858366178,-19.9908709649436,
0.150143718198236));
#46081=CARTESIAN_POINT('Ctrl Pts',(-5.33694163762173,-19.9873310692217,
0.243165701629514));
#46082=CARTESIAN_POINT('Ctrl Pts',(-5.0651271037478,-19.9830663309066,0.359760385930429));
#46083=CARTESIAN_POINT('Ctrl Pts',(-4.7644159818022,-19.978737314844,0.48162965459219));
#46084=CARTESIAN_POINT('Ctrl Pts',(-4.43125170591844,-19.9743534799028,
0.607977396601455));
#46085=CARTESIAN_POINT('Ctrl Pts',(-4.06020269022993,-19.9699355366651,
0.737994634112659));
#46086=CARTESIAN_POINT('Ctrl Pts',(-3.64507829848936,-19.9655386431136,
0.870100245942965));
#46087=CARTESIAN_POINT('Ctrl Pts',(-3.18078122531583,-19.9612765652182,
1.00110796921292));
#46088=CARTESIAN_POINT('Ctrl Pts',(-2.66341923623205,-19.9573162141937,
1.1262250575769));
#46089=CARTESIAN_POINT('Ctrl Pts',(-2.08839798589795,-19.9538554399291,
1.23951350128208));
#46090=CARTESIAN_POINT('Ctrl Pts',(-1.45514799386454,-19.95114667215,1.33275014651456));
#46091=CARTESIAN_POINT('Ctrl Pts',(-0.783132822868955,-19.9494712370586,
1.39496816565624));
#46092=CARTESIAN_POINT('Ctrl Pts',(-0.110281963156994,-19.9489129397822,
1.41910849568614));
#46093=CARTESIAN_POINT('Ctrl Pts',(0.521223569921493,-19.9491709201523,
1.40744675804296));
#46094=CARTESIAN_POINT('Ctrl Pts',(1.08867568765767,-19.9501641904296,1.36886859839447));
#46095=CARTESIAN_POINT('Ctrl Pts',(1.59148448876097,-19.9517279879307,1.31268422210672));
#46096=CARTESIAN_POINT('Ctrl Pts',(2.03961626718321,-19.9536980517254,1.24524254578414));
#46097=CARTESIAN_POINT('Ctrl Pts',(2.44306402237904,-19.9559615511016,1.17043662862498));
#46098=CARTESIAN_POINT('Ctrl Pts',(2.80710095593827,-19.9584160870507,1.09146386419318));
#46099=CARTESIAN_POINT('Ctrl Pts',(3.13528225918272,-19.9609719694098,1.01095989522807));
#46100=CARTESIAN_POINT('Ctrl Pts',(3.43183324401102,-19.963567664804,0.930620741221009));
#46101=CARTESIAN_POINT('Ctrl Pts',(3.70006480313533,-19.9661546387235,0.851739649889142));
#46102=CARTESIAN_POINT('Ctrl Pts',(3.94252576462863,-19.9686929218185,0.77535744497962));
#46103=CARTESIAN_POINT('Ctrl Pts',(4.16147809566364,-19.9711521364158,0.702237741174908));
#46104=CARTESIAN_POINT('Ctrl Pts',(4.35919841515776,-19.97351293619,0.632830400882521));
#46105=CARTESIAN_POINT('Ctrl Pts',(4.53796761308272,-19.9757657149123,0.567315528008788));
#46106=CARTESIAN_POINT('Ctrl Pts',(4.70003294752602,-19.9779089494471,0.505655806689799));
#46107=CARTESIAN_POINT('Ctrl Pts',(4.8475692076678,-19.9799475179402,0.44764801631894));
#46108=CARTESIAN_POINT('Ctrl Pts',(4.98258177188227,-19.9818902710195,0.392994970754419));
#46109=CARTESIAN_POINT('Ctrl Pts',(5.10662625027061,-19.9837447161293,0.341455316020886));
#46110=CARTESIAN_POINT('Ctrl Pts',(5.220762183999,-19.985514530804,0.292905773024752));
#46111=CARTESIAN_POINT('Ctrl Pts',(5.32566819366107,-19.9871997294046,0.24732617640553));
#46112=CARTESIAN_POINT('Ctrl Pts',(5.42196233400887,-19.9888008499558,0.204678562150652));
#46113=CARTESIAN_POINT('Ctrl Pts',(5.51026929291715,-19.9903197568625,0.164883520156243));
#46114=CARTESIAN_POINT('Ctrl Pts',(5.59121757885841,-19.991759397639,0.127825389454448));
#46115=CARTESIAN_POINT('Ctrl Pts',(5.65168088095001,-19.9928706851653,0.0997459306861807));
#46116=CARTESIAN_POINT('Ctrl Pts',(5.68523498108013,-19.9935016482941,0.0840181187176475));
#46117=CARTESIAN_POINT('Ctrl Pts',(5.69415460745399,-19.9936704109565,0.0798269467380955));
#46118=CARTESIAN_POINT('',(5.73644274981144,-19.808949593799,0.442545696620674));
#46119=CARTESIAN_POINT('Origin',(5.599999999773,-19.591934376757,0.135488061232669));
#46120=CARTESIAN_POINT('Ctrl Pts',(-5.73644387793174,-19.8089519016381,
0.442549068206041));
#46121=CARTESIAN_POINT('Ctrl Pts',(-5.66411038140175,-19.8074370301154,
0.475761117952496));
#46122=CARTESIAN_POINT('Ctrl Pts',(-5.58548128727225,-19.8058476858708,
0.511218927486439));
#46123=CARTESIAN_POINT('Ctrl Pts',(-5.50055659392378,-19.80419803833,0.548567705601548));
#46124=CARTESIAN_POINT('Ctrl Pts',(-5.41741954148235,-19.8025831154059,
0.585130302442944));
#46125=CARTESIAN_POINT('Ctrl Pts',(-5.32824914148616,-19.8009104085098,
0.623504910589953));
#46126=CARTESIAN_POINT('Ctrl Pts',(-5.23304539241587,-19.7991952413925,
0.663306052555013));
#46127=CARTESIAN_POINT('Ctrl Pts',(-5.13477098872149,-19.7974247541235,
0.704390920862915));
#46128=CARTESIAN_POINT('Ctrl Pts',(-5.03006776621619,-19.7956090117036,
0.746996134649694));
#46129=CARTESIAN_POINT('Ctrl Pts',(-4.91893572322883,-19.7937671144692,
0.790639472565173));
#46130=CARTESIAN_POINT('Ctrl Pts',(-4.80780368024147,-19.7919252172349,
0.834282810480652));
#46131=CARTESIAN_POINT('Ctrl Pts',(-4.69024281677204,-19.7900571649709,
0.878964276341194));
#46132=CARTESIAN_POINT('Ctrl Pts',(-4.56625313114939,-19.7881843414101,
0.924142444101347));
#46133=CARTESIAN_POINT('Ctrl Pts',(-4.44622756681731,-19.786371394602,0.96787620351586));
#46134=CARTESIAN_POINT('Ctrl Pts',(-4.3201776876802,-19.7845539879721,1.01207512388596));
#46135=CARTESIAN_POINT('Ctrl Pts',(-4.18810349373807,-19.7827535612779,
1.05619516429525));
#46136=CARTESIAN_POINT('Ctrl Pts',(-4.05161761231589,-19.7808929947511,
1.1017889508171));
#46137=CARTESIAN_POINT('Ctrl Pts',(-3.90869823277936,-19.7790505488329,
1.14729881956836));
#46138=CARTESIAN_POINT('Ctrl Pts',(-3.75934535512849,-19.7772521442393,
1.19206590678836));
#46139=CARTESIAN_POINT('Ctrl Pts',(-3.60999247747762,-19.7754537396457,
1.23683299400836));
#46140=CARTESIAN_POINT('Ctrl Pts',(-3.45420610171241,-19.773699375747,1.28085730551268));
#46141=CARTESIAN_POINT('Ctrl Pts',(-3.29198622783285,-19.7720172785995,
1.32342047204876));
#46142=CARTESIAN_POINT('Ctrl Pts',(-3.21175020715356,-19.7711852918751,
1.34447275762075));
#46143=CARTESIAN_POINT('Ctrl Pts',(-3.12994028410414,-19.7703710201625,
1.36516666911119));
#46144=CARTESIAN_POINT('Ctrl Pts',(-3.04655646337055,-19.7695781029454,
1.38540988355588));
#46145=CARTESIAN_POINT('Ctrl Pts',(-3.00486455300375,-19.7691816443369,
1.39553149077823));
#46146=CARTESIAN_POINT('Ctrl Pts',(-2.96277915948905,-19.7687905006953,
1.40554038637855));
#46147=CARTESIAN_POINT('Ctrl Pts',(-2.92030029408361,-19.7684051710099,
1.41542467313665));
#46148=CARTESIAN_POINT('Ctrl Pts',(-2.89906086138089,-19.7682125061672,
1.4203668165157));
#46149=CARTESIAN_POINT('Ctrl Pts',(-2.87772306013855,-19.7680212933365,
1.42527780536093));
#46150=CARTESIAN_POINT('Ctrl Pts',(-2.85628689020884,-19.7678315911959,
1.43015613482796));
#46151=CARTESIAN_POINT('Ctrl Pts',(-2.84556880524398,-19.7677367401257,
1.43259529956148));
#46152=CARTESIAN_POINT('Ctrl Pts',(-2.83482612807483,-19.7676422666352,
1.43502629930336));
#46153=CARTESIAN_POINT('Ctrl Pts',(-2.8240588586925,-19.7675481781346,1.43744894462185));
#46154=CARTESIAN_POINT('Ctrl Pts',(-2.81867522400134,-19.7675011338842,
1.4386602672811));
#46155=CARTESIAN_POINT('Ctrl Pts',(-2.81328544125487,-19.7674541858755,
1.43986950132529));
#46156=CARTESIAN_POINT('Ctrl Pts',(-2.80788951045314,-19.7674073350413,
1.44107662299125));
#46157=CARTESIAN_POINT('Ctrl Pts',(-2.80249357965141,-19.7673604842071,
1.44228374465721));
#46158=CARTESIAN_POINT('Ctrl Pts',(-2.79531854980412,-19.7672984356932,
1.44388308559887));
#46159=CARTESIAN_POINT('Ctrl Pts',(-2.79168327387814,-19.7672670749844,
1.44469162704568));
#46160=CARTESIAN_POINT('Ctrl Pts',(-2.04596901439503,-19.7608339655671,
1.61054998237992));
#46161=CARTESIAN_POINT('Ctrl Pts',(-1.30026709200512,-19.7571553182439,
1.70987224350879));
#46162=CARTESIAN_POINT('Ctrl Pts',(-0.554547850970883,-19.7562174227089,
1.7426256094221));
#46163=CARTESIAN_POINT('Ctrl Pts',(-0.369699781998668,-19.7559849381906,
1.75074447790271));
#46164=CARTESIAN_POINT('Ctrl Pts',(-0.184850648900509,-19.7559209178912,
1.75477284736426));
#46165=CARTESIAN_POINT('Ctrl Pts',(3.10862446895044E-14,-19.7560252757495,
1.75470973948686));
#46166=CARTESIAN_POINT('Ctrl Pts',(6.95448532179484E-5,-19.7560253150112,
1.7547097157443));
#46167=CARTESIAN_POINT('Ctrl Pts',(0.00013908970661878,-19.7560253542967,
1.75470969142261));
#46168=CARTESIAN_POINT('Ctrl Pts',(0.000208634560234102,-19.7560253936061,
1.7547096665218));
#46169=CARTESIAN_POINT('Ctrl Pts',(0.465533558834944,-19.7562884127967,
1.75454305511928));
#46170=CARTESIAN_POINT('Ctrl Pts',(0.930858482087836,-19.7573599746889,
1.7286044125423));
#46171=CARTESIAN_POINT('Ctrl Pts',(1.39618340431891,-19.759242170924,1.67690524758153));
#46172=CARTESIAN_POINT('Ctrl Pts',(1.62884586543444,-19.7601832690415,1.65105566510115));
#46173=CARTESIAN_POINT('Ctrl Pts',(1.86150832640128,-19.7613268920606,1.61876628003846));
#46174=CARTESIAN_POINT('Ctrl Pts',(2.09417078585734,-19.7626724996003,1.58004052341054));
#46175=CARTESIAN_POINT('Ctrl Pts',(2.21050201558537,-19.7633453033701,1.56067764509659));
#46176=CARTESIAN_POINT('Ctrl Pts',(2.32683324685238,-19.7640686101838,1.53970568504067));
#46177=CARTESIAN_POINT('Ctrl Pts',(2.44316447733886,-19.7648422853926,1.51712520929198));
#46178=CARTESIAN_POINT('Ctrl Pts',(2.5013300925821,-19.7652291229971,1.50583497141763));
#46179=CARTESIAN_POINT('Ctrl Pts',(2.55949570773314,-19.7656285531405,1.49414260533559));
#46180=CARTESIAN_POINT('Ctrl Pts',(2.61766132280996,-19.7660405585964,1.48204818801444));
#46181=CARTESIAN_POINT('Ctrl Pts',(2.64674413034836,-19.7662465613244,1.47600097935386));
#46182=CARTESIAN_POINT('Ctrl Pts',(2.67582693787725,-19.7664557079078,1.46985325792706));
#46183=CARTESIAN_POINT('Ctrl Pts',(2.70490974539835,-19.7666679959892,1.46360503385831));
#46184=CARTESIAN_POINT('Ctrl Pts',(2.73217487744938,-19.7668670160654,1.45774732379385));
#46185=CARTESIAN_POINT('Ctrl Pts',(2.75944000949386,-19.7670687972249,1.45180128133079));
#46186=CARTESIAN_POINT('Ctrl Pts',(2.78670514153807,-19.7672733374521,1.44576691505616));
#46187=CARTESIAN_POINT('Ctrl Pts',(2.78852281700768,-19.7672869734672,1.44536462397119));
#46188=CARTESIAN_POINT('Ctrl Pts',(2.79172281222576,-19.7673110104151,1.44465540587742));
#46189=CARTESIAN_POINT('Ctrl Pts',(2.79215816794666,-19.7673142822828,1.4445588641543));
#46190=CARTESIAN_POINT('Ctrl Pts',(2.80635173261917,-19.7674209524462,1.44141138928538));
#46191=CARTESIAN_POINT('Ctrl Pts',(2.82657059814034,-19.7675848511013,1.43690103084202));
#46192=CARTESIAN_POINT('Ctrl Pts',(2.85281476451015,-19.7678094469751,1.43094042386484));
#46193=CARTESIAN_POINT('Ctrl Pts',(2.87905922487078,-19.7680340453649,1.42497975011611));
#46194=CARTESIAN_POINT('Ctrl Pts',(2.91132912107335,-19.7683193421491,1.41756879525677));
#46195=CARTESIAN_POINT('Ctrl Pts',(2.94962445311786,-19.768670883477,1.40856810271974));
#46196=CARTESIAN_POINT('Ctrl Pts',(2.9879202384843,-19.7690224289664,1.39956730363679));
#46197=CARTESIAN_POINT('Ctrl Pts',(3.03224160234602,-19.769440220275,1.38897672914351));
#46198=CARTESIAN_POINT('Ctrl Pts',(3.08258854470301,-19.7699318846709,1.37660482945053));
#46199=CARTESIAN_POINT('Ctrl Pts',(3.13293647355783,-19.7704235587004,1.36423268734258));
#46200=CARTESIAN_POINT('Ctrl Pts',(3.18931021704058,-19.7709891083087,1.35007915018452));
#46201=CARTESIAN_POINT('Ctrl Pts',(3.25170977515124,-19.77163824743,1.3339005678628));
#46202=CARTESIAN_POINT('Ctrl Pts',(3.31411003816818,-19.7722873938844,1.31772180277722));
#46203=CARTESIAN_POINT('Ctrl Pts',(3.38253625195691,-19.7730201312322,1.29951794664595));
#46204=CARTESIAN_POINT('Ctrl Pts',(3.45698841651743,-19.7738482668148,1.27899325277008));
#46205=CARTESIAN_POINT('Ctrl Pts',(3.53144199947791,-19.7746764181744,1.25846816787501));
#46206=CARTESIAN_POINT('Ctrl Pts',(3.61192176281505,-19.7755999707861,1.2356221567306));
#46207=CARTESIAN_POINT('Ctrl Pts',(3.69842770652883,-19.7766328342588,1.21010736714599));
#46208=CARTESIAN_POINT('Ctrl Pts',(3.77372504312439,-19.7775318692293,1.18789853828361));
#46209=CARTESIAN_POINT('Ctrl Pts',(3.85358810166981,-19.778513755189,1.16366691832388));
#46210=CARTESIAN_POINT('Ctrl Pts',(3.93801688216508,-19.7795889672883,1.13715098203608));
#46211=CARTESIAN_POINT('Ctrl Pts',(3.98561589130771,-19.7801951471981,1.122201905591));
#46212=CARTESIAN_POINT('Ctrl Pts',(4.03466609031313,-19.7808310122523,1.1065262314541));
#46213=CARTESIAN_POINT('Ctrl Pts',(4.0851674847676,-19.7814986223688,1.09007289718878));
#46214=CARTESIAN_POINT('Ctrl Pts',(4.11041818199483,-19.7818324274271,1.08184623005612));
#46215=CARTESIAN_POINT('Ctrl Pts',(4.1360316685357,-19.7821741490636,1.07342511796124));
#46216=CARTESIAN_POINT('Ctrl Pts',(4.16200795649282,-19.7825240823293,1.06480287426906));
#46217=CARTESIAN_POINT('Ctrl Pts',(4.17499610047137,-19.7826990489621,1.06049175242297));
#46218=CARTESIAN_POINT('Ctrl Pts',(4.18807494421639,-19.7828760672703,1.05613034579871));
#46219=CARTESIAN_POINT('Ctrl Pts',(4.20124448757875,-19.7830551710674,1.05171780388577));
#46220=CARTESIAN_POINT('Ctrl Pts',(4.20782925925993,-19.783144722966,1.0495115329293));
#46221=CARTESIAN_POINT('Ctrl Pts',(4.21443670580743,-19.78323479616,1.04729247803444));
#46222=CARTESIAN_POINT('Ctrl Pts',(4.22106682722272,-19.7833253949677,1.04506053174477));
#46223=CARTESIAN_POINT('Ctrl Pts',(4.22769694863801,-19.7834159937755,1.04282858545509));
#46224=CARTESIAN_POINT('Ctrl Pts',(4.23593845356822,-19.7835289311228,1.04004640064536));
#46225=CARTESIAN_POINT('Ctrl Pts',(4.24102521599583,-19.7835987724094,1.03832591063626));
#46226=CARTESIAN_POINT('Ctrl Pts',(4.37039632198203,-19.7853750386718,0.994568865072864));
#46227=CARTESIAN_POINT('Ctrl Pts',(4.49374157185689,-19.7871644886092,0.95084303173788));
#46228=CARTESIAN_POINT('Ctrl Pts',(4.61106096691901,-19.788946139999,0.907680881245061));
#46229=CARTESIAN_POINT('Ctrl Pts',(4.72934383257832,-19.7907424229741,0.86416426708586));
#46230=CARTESIAN_POINT('Ctrl Pts',(4.84150146389165,-19.7925307763442,0.821220700844053));
#46231=CARTESIAN_POINT('Ctrl Pts',(4.94753386218982,-19.7942917673862,0.779342300060695));
#46232=CARTESIAN_POINT('Ctrl Pts',(5.05275938615735,-19.7960393578216,0.737782581181571));
#46233=CARTESIAN_POINT('Ctrl Pts',(5.15195254473685,-19.7977600036065,0.69727180802215));
#46234=CARTESIAN_POINT('Ctrl Pts',(5.24511333922899,-19.799436732092,0.658238623808673));
#46235=CARTESIAN_POINT('Ctrl Pts',(5.33934567583654,-19.8011327464283,0.618756477121113));
#46236=CARTESIAN_POINT('Ctrl Pts',(5.42740608092356,-19.8027838235402,0.58078620540688));
#46237=CARTESIAN_POINT('Ctrl Pts',(5.50929455583613,-19.8043744898071,0.54471720648797));
#46238=CARTESIAN_POINT('Ctrl Pts',(5.5911830307487,-19.805965156074,0.508648207569059));
#46239=CARTESIAN_POINT('Ctrl Pts',(5.66689957548683,-19.807495411507,0.474480479178912));
#46240=CARTESIAN_POINT('Ctrl Pts',(5.73644419139658,-19.8089518848396,0.442548940790224));
#46241=CARTESIAN_POINT('Origin',(5.6,-19.5919343769583,0.135488060981343));
#46242=CARTESIAN_POINT('Origin',(5.59997427801439,-19.5919309020471,0.135464036486979));
#46243=CARTESIAN_POINT('Ctrl Pts',(5.71133811337302,-10.3755286010609,1.73145257720377));
#46244=CARTESIAN_POINT('Ctrl Pts',(5.75152712774209,-10.3630818178758,1.71508837504171));
#46245=CARTESIAN_POINT('Ctrl Pts',(5.83253386184225,-10.339510644463,1.66946189472995));
#46246=CARTESIAN_POINT('Ctrl Pts',(5.93556513369406,-10.3144216017685,1.56983798684213));
#46247=CARTESIAN_POINT('Ctrl Pts',(6.0101868944103,-10.3020933870588,1.44730328144741));
#46248=CARTESIAN_POINT('Ctrl Pts',(6.0464526344208,-10.3029959215501,1.32878328478311));
#46249=CARTESIAN_POINT('Ctrl Pts',(6.05178037288678,-10.3097270187875,1.25604070393047));
#46250=CARTESIAN_POINT('Ctrl Pts',(6.05105514091469,-10.3135670567819,1.22629617474195));
#46251=CARTESIAN_POINT('Ctrl Pts',(5.59496958662951,-10.0914744550291,1.65476262870179));
#46252=CARTESIAN_POINT('Ctrl Pts',(5.6324300295316,-10.079786670298,1.63972737512157));
#46253=CARTESIAN_POINT('Ctrl Pts',(5.70803679797223,-10.0575373066719,1.59779561973394));
#46254=CARTESIAN_POINT('Ctrl Pts',(5.8042440459682,-10.0335959394155,1.50625015057469));
#46255=CARTESIAN_POINT('Ctrl Pts',(5.87377408174617,-10.0215572105226,1.39395818247593));
#46256=CARTESIAN_POINT('Ctrl Pts',(5.90737675075672,-10.0219742604469,1.28598673146488));
#46257=CARTESIAN_POINT('Ctrl Pts',(5.91225807786315,-10.0279912265321,1.22030099419056));
#46258=CARTESIAN_POINT('Ctrl Pts',(5.91159342033835,-10.0314515024023,1.19357093143111));
#46259=CARTESIAN_POINT('Ctrl Pts',(5.57745794489003,-9.81893181439426,1.81452368423867));
#46260=CARTESIAN_POINT('Ctrl Pts',(5.63078003213836,-9.80260188831539,1.7933090225621));
#46261=CARTESIAN_POINT('Ctrl Pts',(5.73752235044812,-9.77206798166216,1.73458079337837));
#46262=CARTESIAN_POINT('Ctrl Pts',(5.87296120872625,-9.74001612997592,1.60722602071493));
#46263=CARTESIAN_POINT('Ctrl Pts',(5.97215523450811,-9.72435725886636,1.44946063567694));
#46264=CARTESIAN_POINT('Ctrl Pts',(6.02175241241746,-9.7257043359174,1.29349598934462));
#46265=CARTESIAN_POINT('Ctrl Pts',(6.02944537147473,-9.73486110115558,1.19446719239946));
#46266=CARTESIAN_POINT('Ctrl Pts',(6.02839959740249,-9.74017965350145,1.15322607941975));
#46267=CARTESIAN_POINT('Ctrl Pts',(5.67031557196363,-9.7370756153637,2.10570536871782));
#46268=CARTESIAN_POINT('Ctrl Pts',(5.74766173694799,-9.71375425056511,2.07486541692242));
#46269=CARTESIAN_POINT('Ctrl Pts',(5.90160594775961,-9.67077588277422,1.98989187537063));
#46270=CARTESIAN_POINT('Ctrl Pts',(6.09654035518264,-9.62668739149764,1.80638185716079));
#46271=CARTESIAN_POINT('Ctrl Pts',(6.24065234784129,-9.60587870824828,1.577322095495));
#46272=CARTESIAN_POINT('Ctrl Pts',(6.31438648424582,-9.60895990411399,1.34637426317501));
#46273=CARTESIAN_POINT('Ctrl Pts',(6.32630069195067,-9.6230462278461,1.19552294162878));
#46274=CARTESIAN_POINT('Ctrl Pts',(6.32468266445671,-9.63123942470839,1.13178513551015));
#46275=CARTESIAN_POINT('',(5.99999999999901,-10.0933615553116,1.21101376485454));
#46276=CARTESIAN_POINT('',(5.99999927107837,-9.65439083358236,1.8624630218698));
#46277=CARTESIAN_POINT('Ctrl Pts',(5.99998770355867,-10.0933615554491,1.21101376294399));
#46278=CARTESIAN_POINT('Ctrl Pts',(5.99998389443016,-10.0741186879649,1.2256833335264));
#46279=CARTESIAN_POINT('Ctrl Pts',(5.99998390164969,-10.0552448950568,1.2406862381206));
#46280=CARTESIAN_POINT('Ctrl Pts',(5.99999784523119,-10.0368574489198,1.25602792947848));
#46281=CARTESIAN_POINT('Ctrl Pts',(6.00000835464427,-10.0229986518209,1.26759111155923));
#46282=CARTESIAN_POINT('Ctrl Pts',(6.0000254843442,-10.009416316904,1.27934608106548));
#46283=CARTESIAN_POINT('Ctrl Pts',(6.00004217340985,-9.99615755794859,1.29127967956365));
#46284=CARTESIAN_POINT('Ctrl Pts',(6.00006539524908,-9.97770878583298,1.30788456995736));
#46285=CARTESIAN_POINT('Ctrl Pts',(6.00008857477621,-9.95988747126659,1.32483689381485));
#46286=CARTESIAN_POINT('Ctrl Pts',(6.00010759262717,-9.94279223481774,1.34206757541617));
#46287=CARTESIAN_POINT('Ctrl Pts',(6.00011528625985,-9.93587639189722,1.34903821239592));
#46288=CARTESIAN_POINT('Ctrl Pts',(6.00012209870678,-9.92907912135122,1.356053879453));
#46289=CARTESIAN_POINT('Ctrl Pts',(6.00012731958345,-9.92240574123668,1.36310798860156));
#46290=CARTESIAN_POINT('Ctrl Pts',(6.0001405716832,-9.90546676629374,1.38101336429743));
#46291=CARTESIAN_POINT('Ctrl Pts',(6.00014254779794,-9.8893288051776,1.39916896132706));
#46292=CARTESIAN_POINT('Ctrl Pts',(6.000126590469,-9.87405375348299,1.41743989761469));
#46293=CARTESIAN_POINT('Ctrl Pts',(6.00011864155799,-9.86644470894263,1.42654129843389));
#46294=CARTESIAN_POINT('Ctrl Pts',(6.0001064336008,-9.8590491939023,1.4356707588169));
#46295=CARTESIAN_POINT('Ctrl Pts',(6.00009082199952,-9.85187121335682,1.44480893859278));
#46296=CARTESIAN_POINT('Ctrl Pts',(6.00008441100787,-9.84892353537432,1.44856158338677));
#46297=CARTESIAN_POINT('Ctrl Pts',(6.0000781550863,-9.84599792430372,1.45233257340954));
#46298=CARTESIAN_POINT('Ctrl Pts',(6.00007171917567,-9.84310110032392,1.45611438476854));
#46299=CARTESIAN_POINT('Ctrl Pts',(6.00005349850847,-9.83489991967,1.46682104777966));
#46300=CARTESIAN_POINT('Ctrl Pts',(6.00003298876159,-9.8269318828134,1.47761727587867));
#46301=CARTESIAN_POINT('Ctrl Pts',(6.00001091572104,-9.81932764534066,1.4883072411331));
#46302=CARTESIAN_POINT('Ctrl Pts',(5.99998852113744,-9.81161263519312,1.49915292956805));
#46303=CARTESIAN_POINT('Ctrl Pts',(5.99996411956146,-9.80427237022355,1.50988876190026));
#46304=CARTESIAN_POINT('Ctrl Pts',(5.99995391373301,-9.79740660411635,1.52027358190028));
#46305=CARTESIAN_POINT('Ctrl Pts',(5.99995171009857,-9.79592415331001,1.52251586404948));
#46306=CARTESIAN_POINT('Ctrl Pts',(5.99995023593322,-9.79446368393491,1.52474166500346));
#46307=CARTESIAN_POINT('Ctrl Pts',(5.9999497685552,-9.79302597069511,1.52694837772846));
#46308=CARTESIAN_POINT('Ctrl Pts',(5.99994527145316,-9.77919232251255,1.54818132365431));
#46309=CARTESIAN_POINT('Ctrl Pts',(5.99996424179167,-9.76607610181729,1.56992337199025));
#46310=CARTESIAN_POINT('Ctrl Pts',(5.99998963853606,-9.75381433254361,1.59208686252081));
#46311=CARTESIAN_POINT('Ctrl Pts',(6.0000149372747,-9.74159988130341,1.61416482438388));
#46312=CARTESIAN_POINT('Ctrl Pts',(6.00004588401721,-9.73023410458729,1.63666047488403));
#46313=CARTESIAN_POINT('Ctrl Pts',(6.0000667455618,-9.71982413701758,1.65944401473347));
#46314=CARTESIAN_POINT('Ctrl Pts',(6.00008321614764,-9.71160526982082,1.67743205235613));
#46315=CARTESIAN_POINT('Ctrl Pts',(6.00009334879337,-9.70398170771886,1.69559852861912));
#46316=CARTESIAN_POINT('Ctrl Pts',(6.00009392184178,-9.696989358003,1.71386448439385));
#46317=CARTESIAN_POINT('Ctrl Pts',(6.00009465088789,-9.68809352076062,1.7371028772448));
#46318=CARTESIAN_POINT('Ctrl Pts',(6.00007926180274,-9.68022089597653,1.76050251695918));
#46319=CARTESIAN_POINT('Ctrl Pts',(6.00005735438713,-9.67340477113262,1.78388361762506));
#46320=CARTESIAN_POINT('Ctrl Pts',(6.00003516239185,-9.66650010409649,1.80756844129435));
#46321=CARTESIAN_POINT('Ctrl Pts',(6.00000603608545,-9.66067964436474,1.83123317213234));
#46322=CARTESIAN_POINT('Ctrl Pts',(5.99999995656782,-9.65592999578,1.85467974452393));
#46323=CARTESIAN_POINT('Ctrl Pts',(5.99999928313501,-9.65540387358089,1.85727693924436));
#46324=CARTESIAN_POINT('Ctrl Pts',(5.99999891415755,-9.65489084251379,1.85987145558861));
#46325=CARTESIAN_POINT('Ctrl Pts',(5.99999890661755,-9.6543908489942,1.86246302484216));
#46326=CARTESIAN_POINT('',(5.72001518115902,-9.72697656272786,2.0594344008613));
#46327=CARTESIAN_POINT('Ctrl Pts',(5.72001578478243,-9.72697810542107,2.05943472749027));
#46328=CARTESIAN_POINT('Ctrl Pts',(5.74831100472407,-9.71874550010011,2.04602639308294));
#46329=CARTESIAN_POINT('Ctrl Pts',(5.77568625593793,-9.71101591981585,2.03140417355019));
#46330=CARTESIAN_POINT('Ctrl Pts',(5.80217318781282,-9.70375779008786,2.01566912583796));
#46331=CARTESIAN_POINT('Ctrl Pts',(5.82514840580841,-9.69746196414892,2.00202027616873));
#46332=CARTESIAN_POINT('Ctrl Pts',(5.84745545926059,-9.6915209690025,1.9875330189415));
#46333=CARTESIAN_POINT('Ctrl Pts',(5.86910927423317,-9.68592085153798,1.97224290234583));
#46334=CARTESIAN_POINT('Ctrl Pts',(5.87213457678101,-9.68513844669823,1.97010668622169));
#46335=CARTESIAN_POINT('Ctrl Pts',(5.8751470713802,-9.68436271319161,1.9679548108044));
#46336=CARTESIAN_POINT('Ctrl Pts',(5.87814679973064,-9.6835936198623,1.96578732373684));
#46337=CARTESIAN_POINT('Ctrl Pts',(5.90308793908996,-9.6771990195299,1.94776582622233));
#46338=CARTESIAN_POINT('Ctrl Pts',(5.92714861735105,-9.67126222158962,1.92866869327927));
#46339=CARTESIAN_POINT('Ctrl Pts',(5.9503530048751,-9.6657663374122,1.90851108261494));
#46340=CARTESIAN_POINT('Ctrl Pts',(5.96736235160321,-9.66173772862197,1.8937350930033));
#46341=CARTESIAN_POINT('Ctrl Pts',(5.9839111813902,-9.65794632524712,1.87838828078923));
#46342=CARTESIAN_POINT('Ctrl Pts',(5.99999890661755,-9.65439084899398,1.86246302484326));
#46343=CARTESIAN_POINT('',(5.73278448927459,-10.3449549114295,1.71289216038973));
#46344=CARTESIAN_POINT('Origin',(5.89877390157852,-10.1838134841955,2.15616635811418));
#46345=CARTESIAN_POINT('Ctrl Pts',(5.73278343850714,-10.3449559315799,1.71288935424927));
#46346=CARTESIAN_POINT('Ctrl Pts',(5.74706594025812,-10.3340579318584,1.70357912933021));
#46347=CARTESIAN_POINT('Ctrl Pts',(5.7606924637996,-10.3236084956166,1.69367908770345));
#46348=CARTESIAN_POINT('Ctrl Pts',(5.7736157350861,-10.3135974006678,1.68336145275714));
#46349=CARTESIAN_POINT('Ctrl Pts',(5.78686204651708,-10.3033360606001,1.6727859101797));
#46350=CARTESIAN_POINT('Ctrl Pts',(5.79937022147026,-10.2935348620722,1.66177263797491));
#46351=CARTESIAN_POINT('Ctrl Pts',(5.81114106549577,-10.2841865752441,1.65048704321575));
#46352=CARTESIAN_POINT('Ctrl Pts',(5.82340063156014,-10.2744501502512,1.63873287382688));
#46353=CARTESIAN_POINT('Ctrl Pts',(5.83486131813222,-10.2652047124572,1.62668404740507));
#46354=CARTESIAN_POINT('Ctrl Pts',(5.84556649895441,-10.2564517360702,1.61449197344315));
#46355=CARTESIAN_POINT('Ctrl Pts',(5.84821827311156,-10.254283541346,1.61147188184532));
#46356=CARTESIAN_POINT('Ctrl Pts',(5.85082384535926,-10.2521456204111,1.60844280935656));
#46357=CARTESIAN_POINT('Ctrl Pts',(5.8533841464279,-10.2500381107383,1.60540667504513));
#46358=CARTESIAN_POINT('Ctrl Pts',(5.86462142145881,-10.2407881572411,1.59208094679144));
#46359=CARTESIAN_POINT('Ctrl Pts',(5.87496485395669,-10.2321098068509,1.57863342454987));
#46360=CARTESIAN_POINT('Ctrl Pts',(5.88446757402116,-10.2239747888587,1.5652369199639));
#46361=CARTESIAN_POINT('Ctrl Pts',(5.88870736401695,-10.2203452209387,1.55925985595098));
#46362=CARTESIAN_POINT('Ctrl Pts',(5.89278028921961,-10.2168239588668,1.55329243262826));
#46363=CARTESIAN_POINT('Ctrl Pts',(5.89669301056068,-10.2134092586863,1.54734745152633));
#46364=CARTESIAN_POINT('Ctrl Pts',(5.90303419873817,-10.2078751931276,1.53771266269452));
#46365=CARTESIAN_POINT('Ctrl Pts',(5.90895335839127,-10.2026197175057,1.52813789901526));
#46366=CARTESIAN_POINT('Ctrl Pts',(5.91447772628224,-10.1976310571052,1.51867479271051));
#46367=CARTESIAN_POINT('Ctrl Pts',(5.91723991022772,-10.195136726905,1.51394323955814));
#46368=CARTESIAN_POINT('Ctrl Pts',(5.91990336636591,-10.1927090997186,1.50923960424323));
#46369=CARTESIAN_POINT('Ctrl Pts',(5.92247184573428,-10.1903465860769,1.5045695429203));
#46370=CARTESIAN_POINT('Ctrl Pts',(5.92381837363261,-10.1891080359184,1.50212125856353));
#46371=CARTESIAN_POINT('Ctrl Pts',(5.92487882671067,-10.1881259571778,1.50016163694302));
#46372=CARTESIAN_POINT('Ctrl Pts',(5.9260665578843,-10.1870235681627,1.49794011890751));
#46373=CARTESIAN_POINT('Ctrl Pts',(5.92714440399162,-10.186023168632,1.49592412857225));
#46374=CARTESIAN_POINT('Ctrl Pts',(5.92832754104918,-10.1849235979202,1.49369260689465));
#46375=CARTESIAN_POINT('Ctrl Pts',(5.92989598840333,-10.1834528208751,1.49066569306805));
#46376=CARTESIAN_POINT('Ctrl Pts',(5.93909904534128,-10.1748228564377,1.47290490548488));
#46377=CARTESIAN_POINT('Ctrl Pts',(5.94727709077157,-10.1668954013321,1.45510029582112));
#46378=CARTESIAN_POINT('Ctrl Pts',(5.95446910596299,-10.159602320606,1.43744398035853));
#46379=CARTESIAN_POINT('Ctrl Pts',(5.96185599887856,-10.1521116236435,1.41930924230051));
#46380=CARTESIAN_POINT('Ctrl Pts',(5.96820359292578,-10.1452898169574,1.40133156463171));
#46381=CARTESIAN_POINT('Ctrl Pts',(5.97359534977732,-10.1390731519335,1.38368381110519));
#46382=CARTESIAN_POINT('Ctrl Pts',(5.97925150630115,-10.1325516355892,1.36517065129693));
#46383=CARTESIAN_POINT('Ctrl Pts',(5.98385679554753,-10.1266957972089,1.34702100805308));
#46384=CARTESIAN_POINT('Ctrl Pts',(5.98753741331365,-10.1214478149248,1.32938740197709));
#46385=CARTESIAN_POINT('Ctrl Pts',(5.99132844747022,-10.1160423962271,1.31122479798355));
#46386=CARTESIAN_POINT('Ctrl Pts',(5.99413962519572,-10.1112817793758,1.29360957474132));
#46387=CARTESIAN_POINT('Ctrl Pts',(5.9961226619511,-10.1071217563007,1.27665700852777));
#46388=CARTESIAN_POINT('Ctrl Pts',(5.99820305528237,-10.10275749818,1.25887216132167));
#46389=CARTESIAN_POINT('Ctrl Pts',(5.99937303010722,-10.0990542664404,1.24181635888134));
#46390=CARTESIAN_POINT('Ctrl Pts',(5.99980556935907,-10.0959821632958,1.22556956840182));
#46391=CARTESIAN_POINT('Ctrl Pts',(5.99993672661163,-10.0950506209991,1.2206431151534));
#46392=CARTESIAN_POINT('Ctrl Pts',(6.00000000770566,-10.094177247548,1.2157907116249));
#46393=CARTESIAN_POINT('Ctrl Pts',(5.99999999999901,-10.0933615553116,1.21101376485454));
#46394=CARTESIAN_POINT('Ctrl Pts',(5.99968359779795,-10.0074384078293,1.15797266224462));
#46395=CARTESIAN_POINT('Ctrl Pts',(5.99968359779795,-10.4048995152158,1.32597657845856));
#46396=CARTESIAN_POINT('Ctrl Pts',(5.99968359779795,-11.3019001480193,1.63774436815911));
#46397=CARTESIAN_POINT('Ctrl Pts',(5.99968359779795,-12.7412947791966,1.91665429258608));
#46398=CARTESIAN_POINT('Ctrl Pts',(5.99968359779795,-14.29016833524,1.9708926670458));
#46399=CARTESIAN_POINT('Ctrl Pts',(5.99968359779795,-15.8279016039224,1.7842043053716));
#46400=CARTESIAN_POINT('Ctrl Pts',(5.99968359779795,-17.3191350716031,1.36096628041763));
#46401=CARTESIAN_POINT('Ctrl Pts',(5.99968359779795,-18.6017699378808,0.768028796234896));
#46402=CARTESIAN_POINT('Ctrl Pts',(5.99968359779795,-19.3570916146985,0.286012646059891));
#46403=CARTESIAN_POINT('Ctrl Pts',(5.99968359779795,-19.663819703818,0.0645701956650116));
#46404=CARTESIAN_POINT('Ctrl Pts',(6.00710253473281,-9.93485458739443,1.32967571533749));
#46405=CARTESIAN_POINT('Ctrl Pts',(6.00710253473281,-10.3398263101573,1.50085626859094));
#46406=CARTESIAN_POINT('Ctrl Pts',(6.00710253473281,-11.2536100219151,1.81845838195038));
#46407=CARTESIAN_POINT('Ctrl Pts',(6.00710253473281,-12.7202225074092,2.10263700633451));
#46408=CARTESIAN_POINT('Ctrl Pts',(6.00710253473281,-14.2981186671284,2.1578944512487));
#46409=CARTESIAN_POINT('Ctrl Pts',(6.00710253473281,-15.8649160622648,1.96767950897587));
#46410=CARTESIAN_POINT('Ctrl Pts',(6.00710253473281,-17.3841034287348,1.53650155762526));
#46411=CARTESIAN_POINT('Ctrl Pts',(6.00710253473281,-18.6909640914977,0.932370814900383));
#46412=CARTESIAN_POINT('Ctrl Pts',(6.00710253473281,-19.460427013042,0.441331865624406));
#46413=CARTESIAN_POINT('Ctrl Pts',(6.00710253473281,-19.7729404670082,0.215710140185089));
#46414=CARTESIAN_POINT('Ctrl Pts',(5.90028450533773,-9.87522756015876,1.47072839845487));
#46415=CARTESIAN_POINT('Ctrl Pts',(5.90028450533773,-10.2863691933082,1.64451853359839));
#46416=CARTESIAN_POINT('Ctrl Pts',(5.90028450533773,-11.2139400700279,1.96691349712163));
#46417=CARTESIAN_POINT('Ctrl Pts',(5.90028450533773,-12.7029118048803,2.25542031632971));
#46418=CARTESIAN_POINT('Ctrl Pts',(5.90028450533773,-14.304649801108,2.3115149194609));
#46419=CARTESIAN_POINT('Ctrl Pts',(5.90028450533773,-15.8953231433789,2.11840291946901));
#46420=CARTESIAN_POINT('Ctrl Pts',(5.90028450533773,-17.4374744138533,1.68070238216881));
#46421=CARTESIAN_POINT('Ctrl Pts',(5.90028450533773,-18.7642363744345,1.0673764671802));
#46422=CARTESIAN_POINT('Ctrl Pts',(5.90028450533773,-19.5453162152736,0.568925360697917));
#46423=CARTESIAN_POINT('Ctrl Pts',(5.90028450533773,-19.8625823001286,0.339870394288303));
#46424=CARTESIAN_POINT('Ctrl Pts',(5.72238425036396,-9.85296650859829,1.52338876401701));
#46425=CARTESIAN_POINT('Ctrl Pts',(5.72238425036396,-10.2664116054559,1.69815315596464));
#46426=CARTESIAN_POINT('Ctrl Pts',(5.72238425036396,-11.1991297585749,2.02233747390619));
#46427=CARTESIAN_POINT('Ctrl Pts',(5.72238425036396,-12.6964490570393,2.31246017390902));
#46428=CARTESIAN_POINT('Ctrl Pts',(5.72238425036396,-14.307088123404,2.36886732024849));
#46429=CARTESIAN_POINT('Ctrl Pts',(5.72238425036396,-15.906675270626,2.17467373771829));
#46430=CARTESIAN_POINT('Ctrl Pts',(5.72238425036396,-17.4573998454323,1.73453806943007));
#46431=CARTESIAN_POINT('Ctrl Pts',(5.72238425036396,-18.7915917222315,1.11777924467817));
#46432=CARTESIAN_POINT('Ctrl Pts',(5.72238425036396,-19.5770086037039,0.616560896193298));
#46433=CARTESIAN_POINT('Ctrl Pts',(5.72238425036396,-19.8960490275765,0.38622416951656));
#46434=CARTESIAN_POINT('Ctrl Pts',(5.73278343850724,-10.3449559316229,1.71288935426486));
#46435=CARTESIAN_POINT('Ctrl Pts',(5.73338951373976,-10.6015227247303,1.80593970663245));
#46436=CARTESIAN_POINT('Ctrl Pts',(5.73395354980591,-10.8620213512442,1.88890386447321));
#46437=CARTESIAN_POINT('Ctrl Pts',(5.7344755567973,-11.125573150665,1.96144081361503));
#46438=CARTESIAN_POINT('Ctrl Pts',(5.73532468768319,-11.5542838319682,2.07943418324701));
#46439=CARTESIAN_POINT('Ctrl Pts',(5.73606260779809,-11.9910756848763,2.16983732042539));
#46440=CARTESIAN_POINT('Ctrl Pts',(5.73668937956405,-12.4324023067721,2.23164721150446));
#46441=CARTESIAN_POINT('Ctrl Pts',(5.73681687420498,-12.5221746645008,2.24422025690401));
#46442=CARTESIAN_POINT('Ctrl Pts',(5.73693976982774,-12.6121344962671,2.25561012995919));
#46443=CARTESIAN_POINT('Ctrl Pts',(5.73705806698001,-12.7022516999475,2.26580830619289));
#46444=CARTESIAN_POINT('Ctrl Pts',(5.73707478318901,-12.7149858865471,2.26724937930471));
#46445=CARTESIAN_POINT('Ctrl Pts',(5.73709140757734,-12.7277232153531,2.26866665698201));
#46446=CARTESIAN_POINT('Ctrl Pts',(5.73710794014652,-12.7404635980934,2.27006013275583));
#46447=CARTESIAN_POINT('Ctrl Pts',(5.73767502819834,-13.177474854341,2.31785811582091));
#46448=CARTESIAN_POINT('Ctrl Pts',(5.73813408904666,-13.6180836599348,2.33765181685216));
#46449=CARTESIAN_POINT('Ctrl Pts',(5.73848518400464,-14.0587011175929,2.3291771912748));
#46450=CARTESIAN_POINT('Ctrl Pts',(5.73855071735787,-14.140944222582,2.32759536670342));
#46451=CARTESIAN_POINT('Ctrl Pts',(5.73861248915111,-14.223187483881,2.32502866307856));
#46452=CARTESIAN_POINT('Ctrl Pts',(5.73867049970327,-14.3054073624453,2.32147534064942));
#46453=CARTESIAN_POINT('Ctrl Pts',(5.73897977956717,-14.7437578332544,2.30253101006965));
#46454=CARTESIAN_POINT('Ctrl Pts',(5.73918215133214,-15.1814478225317,2.25554262168904));
#46455=CARTESIAN_POINT('Ctrl Pts',(5.73927764637247,-15.6148698966946,2.18075633105717));
#46456=CARTESIAN_POINT('Ctrl Pts',(5.73929840890395,-15.709104523217,2.16449629589329));
#46457=CARTESIAN_POINT('Ctrl Pts',(5.73931411909929,-15.8031372038809,2.14692221903379));
#46458=CARTESIAN_POINT('Ctrl Pts',(5.73932477707789,-15.8969305343161,2.12803663990889));
#46459=CARTESIAN_POINT('Ctrl Pts',(5.73937358607066,-16.3264639532701,2.04154874857584));
#46460=CARTESIAN_POINT('Ctrl Pts',(5.73931644016915,-16.7509816658227,1.9275547088644));
#46461=CARTESIAN_POINT('Ctrl Pts',(5.73915333029904,-17.1669777326464,1.7867581306035));
#46462=CARTESIAN_POINT('Ctrl Pts',(5.73911747341489,-17.2584272737588,1.75580643778949));
#46463=CARTESIAN_POINT('Ctrl Pts',(5.73907649554377,-17.3494647971327,1.72355950598733));
#46464=CARTESIAN_POINT('Ctrl Pts',(5.739030396378,-17.4400527221644,1.69002486412558));
#46465=CARTESIAN_POINT('Ctrl Pts',(5.73900084492746,-17.4981232868037,1.66852778725571));
#46466=CARTESIAN_POINT('Ctrl Pts',(5.73896918896426,-17.5560090938688,1.646501547335));
#46467=CARTESIAN_POINT('Ctrl Pts',(5.73893542839204,-17.6137011364924,1.62395006942777));
#46468=CARTESIAN_POINT('Ctrl Pts',(5.73869640176937,-18.0221638252673,1.46428442260826));
#46469=CARTESIAN_POINT('Ctrl Pts',(5.73835187053754,-18.4209177953517,1.27828845729314));
#46470=CARTESIAN_POINT('Ctrl Pts',(5.73790179920334,-18.8067387748802,1.06736605898228));
#46471=CARTESIAN_POINT('Ctrl Pts',(5.73786596836643,-18.8374545471248,1.05057421848748));
#46472=CARTESIAN_POINT('Ctrl Pts',(5.73782946860637,-18.868088324797,1.03362440477691));
#46473=CARTESIAN_POINT('Ctrl Pts',(5.73779229989976,-18.898638467726,1.01651733151422));
#46474=CARTESIAN_POINT('Ctrl Pts',(5.73741169653613,-19.211468485665,0.841342830757322));
#46475=CARTESIAN_POINT('Ctrl Pts',(5.73696095091125,-19.5155308117973,0.649677901256858));
#46476=CARTESIAN_POINT('Ctrl Pts',(5.73644003521419,-19.8089444558075,0.442538425468125));
#46477=CARTESIAN_POINT('Ctrl Pts',(5.99999999999901,-10.0933615553116,1.21101376485454));
#46478=CARTESIAN_POINT('Ctrl Pts',(5.99999999999902,-10.2342115358103,1.26888262128331));
#46479=CARTESIAN_POINT('Ctrl Pts',(6.00000000007117,-10.3759192504903,1.32333077848203));
#46480=CARTESIAN_POINT('Ctrl Pts',(5.9999999982386,-10.5185579008191,1.37443737920613));
#46481=CARTESIAN_POINT('Ctrl Pts',(5.99999999639773,-10.6618425531298,1.42577543869178));
#46482=CARTESIAN_POINT('Ctrl Pts',(5.99999999249222,-10.8060670351755,1.47374173423722));
#46483=CARTESIAN_POINT('Ctrl Pts',(5.99999999189388,-10.9513242537834,1.51836744200924));
#46484=CARTESIAN_POINT('Ctrl Pts',(5.99999999151874,-11.042396086891,1.54634639582287));
#46485=CARTESIAN_POINT('Ctrl Pts',(5.9999999928441,-11.1338742268903,1.57301121591701));
#46486=CARTESIAN_POINT('Ctrl Pts',(5.99999999533728,-11.2257841171048,1.59835945117828));
#46487=CARTESIAN_POINT('Ctrl Pts',(5.99999999728275,-11.2975031128956,1.61813915033543));
#46488=CARTESIAN_POINT('Ctrl Pts',(5.99999999999971,-11.3694850404562,1.63711702887793));
#46489=CARTESIAN_POINT('Ctrl Pts',(5.99999999999971,-11.4417456110861,1.65529145736262));
#46490=CARTESIAN_POINT('Ctrl Pts',(5.99999999999971,-11.6167974858284,1.69931917193611));
#46491=CARTESIAN_POINT('Ctrl Pts',(5.99999998490599,-11.7934508492852,1.73870094298862));
#46492=CARTESIAN_POINT('Ctrl Pts',(5.99999998011058,-11.9712350857339,1.77327579437879));
#46493=CARTESIAN_POINT('Ctrl Pts',(5.9999999753187,-12.1488888962661,1.80782528099663));
#46494=CARTESIAN_POINT('Ctrl Pts',(5.99999998033521,-12.3276714858777,1.8375747837877));
#46495=CARTESIAN_POINT('Ctrl Pts',(5.99999998873906,-12.5070997365936,1.86241385083192));
#46496=CARTESIAN_POINT('Ctrl Pts',(5.99999999244222,-12.5861646634751,1.87335916747977));
#46497=CARTESIAN_POINT('Ctrl Pts',(5.9999999964315,-12.6653548222305,1.88335168086257));
#46498=CARTESIAN_POINT('Ctrl Pts',(5.99999999855252,-12.7446283783657,1.89238511809521));
#46499=CARTESIAN_POINT('Ctrl Pts',(5.99999999944807,-12.7780997308221,1.89619926970197));
#46500=CARTESIAN_POINT('Ctrl Pts',(5.99999999999971,-12.8115859483216,1.89984246629865));
#46501=CARTESIAN_POINT('Ctrl Pts',(5.99999999999971,-12.8450837113497,1.90331467554893));
#46502=CARTESIAN_POINT('Ctrl Pts',(5.99999999999971,-13.0549406604288,1.92506738898285));
#46503=CARTESIAN_POINT('Ctrl Pts',(5.99999998498977,-13.2652658520439,1.94004065756617));
#46504=CARTESIAN_POINT('Ctrl Pts',(5.99999998424828,-13.4758154446101,1.94828024097899));
#46505=CARTESIAN_POINT('Ctrl Pts',(5.9999999835058,-13.686645927915,1.95653081668414));
#46506=CARTESIAN_POINT('Ctrl Pts',(5.99999999341929,-13.8977019825745,1.95802978030323));
#46507=CARTESIAN_POINT('Ctrl Pts',(5.99999999806903,-14.108744973676,1.95277140513812));
#46508=CARTESIAN_POINT('Ctrl Pts',(5.99999999924309,-14.162033264823,1.9514436670062));
#46509=CARTESIAN_POINT('Ctrl Pts',(5.99999999999972,-14.2153207296733,1.94968484831666));
#46510=CARTESIAN_POINT('Ctrl Pts',(5.99999999999972,-14.2686035217176,1.94749433026555));
#46511=CARTESIAN_POINT('Ctrl Pts',(5.99999999999972,-14.2755281186275,1.94720965196801));
#46512=CARTESIAN_POINT('Ctrl Pts',(5.99999999998697,-14.2824526370692,1.94691772879533));
#46513=CARTESIAN_POINT('Ctrl Pts',(5.99999999996268,-14.2893770551291,1.94661855921418));
#46514=CARTESIAN_POINT('Ctrl Pts',(5.99999999919951,-14.5068769322331,1.93722147391849));
#46515=CARTESIAN_POINT('Ctrl Pts',(5.99999999014405,-14.7242778297529,1.92067056310208));
#46516=CARTESIAN_POINT('Ctrl Pts',(5.99999998974401,-14.9409228014816,1.89701138721353));
#46517=CARTESIAN_POINT('Ctrl Pts',(5.99999998934372,-15.1577057951409,1.87333713834586));
#46518=CARTESIAN_POINT('Ctrl Pts',(5.99999999677977,-15.3737313428998,1.84254561761958));
#46519=CARTESIAN_POINT('Ctrl Pts',(5.99999999936865,-15.5883455253423,1.80473432426097));
#46520=CARTESIAN_POINT('Ctrl Pts',(5.99999999976083,-15.6208564573964,1.79900646240549));
#46521=CARTESIAN_POINT('Ctrl Pts',(5.99999999999972,-15.6533350188477,1.79311760774684));
#46522=CARTESIAN_POINT('Ctrl Pts',(5.99999999999972,-15.6857789575284,1.78706820160289));
#46523=CARTESIAN_POINT('Ctrl Pts',(5.99999999999972,-15.7315477507526,1.77853428031619));
#46524=CARTESIAN_POINT('Ctrl Pts',(5.99999999951876,-15.777247151839,1.76967947395661));
#46525=CARTESIAN_POINT('Ctrl Pts',(5.99999999869846,-15.8228747191234,1.76050412644273));
#46526=CARTESIAN_POINT('Ctrl Pts',(5.99999999491949,-16.0330725133978,1.7182349912707));
#46527=CARTESIAN_POINT('Ctrl Pts',(5.99999998426348,-16.2417469407301,1.66916709667107));
#46528=CARTESIAN_POINT('Ctrl Pts',(5.9999999840381,-16.4486448314297,1.61336408257583));
#46529=CARTESIAN_POINT('Ctrl Pts',(5.99999998381272,-16.6555427221293,1.5575610684806));
#46530=CARTESIAN_POINT('Ctrl Pts',(5.99999999999972,-16.8606646284446,1.49502273906511));
#46531=CARTESIAN_POINT('Ctrl Pts',(5.99999999999972,-17.0637382052462,1.42576403766304));
#46532=CARTESIAN_POINT('Ctrl Pts',(5.99999999999972,-17.1461081213509,1.39767159198959));
#46533=CARTESIAN_POINT('Ctrl Pts',(5.9999999959448,-17.228147456194,1.36848536385057));
#46534=CARTESIAN_POINT('Ctrl Pts',(5.99999999152483,-17.3098017704308,1.33821950546152));
#46535=CARTESIAN_POINT('Ctrl Pts',(5.99999998224927,-17.4811578307823,1.27470494036867));
#46536=CARTESIAN_POINT('Ctrl Pts',(5.99999997346263,-17.6508169321434,1.20643267167925));
#46537=CARTESIAN_POINT('Ctrl Pts',(5.99999997653249,-17.8183278080572,1.13361882186231));
#46538=CARTESIAN_POINT('Ctrl Pts',(5.99999997960618,-17.9860479662972,1.06071400092609));
#46539=CARTESIAN_POINT('Ctrl Pts',(5.99999999486857,-18.15161412349,0.983256456991716));
#46540=CARTESIAN_POINT('Ctrl Pts',(5.99999999914226,-18.3145968762394,0.901509651121568));
#46541=CARTESIAN_POINT('Ctrl Pts',(5.9999999996837,-18.335245252142,0.89115310266497));
#46542=CARTESIAN_POINT('Ctrl Pts',(5.99999999999972,-18.3558521987823,0.880727768035456));
#46543=CARTESIAN_POINT('Ctrl Pts',(5.99999999999972,-18.376416875006,0.870234233398874));
#46544=CARTESIAN_POINT('Ctrl Pts',(5.99999999999972,-18.4906080449267,0.811965920116257));
#46545=CARTESIAN_POINT('Ctrl Pts',(5.99999999304432,-18.6034685434981,0.751564739808506));
#46546=CARTESIAN_POINT('Ctrl Pts',(5.99999999143185,-18.7150743302283,0.689018754849032));
#46547=CARTESIAN_POINT('Ctrl Pts',(5.999999989508,-18.8482324949303,0.614394411338742));
#46548=CARTESIAN_POINT('Ctrl Pts',(5.99999999273616,-18.9796053836656,0.536717940997866));
#46549=CARTESIAN_POINT('Ctrl Pts',(5.99999999547183,-19.1092808530767,0.455953080560843));
#46550=CARTESIAN_POINT('Ctrl Pts',(5.99999999819522,-19.238374241603,0.375550753466731));
#46551=CARTESIAN_POINT('Ctrl Pts',(5.99999999961476,-19.3657858118951,0.292087468462894));
#46552=CARTESIAN_POINT('Ctrl Pts',(5.99999999985073,-19.4915752850365,0.205483546894013));
#46553=CARTESIAN_POINT('Ctrl Pts',(5.99999999991369,-19.5251424039942,0.182373154069339));
#46554=CARTESIAN_POINT('Ctrl Pts',(5.99999999993326,-19.5585938461359,0.15903888480154));
#46555=CARTESIAN_POINT('Ctrl Pts',(5.99999999993295,-19.591930363142,0.135478724431447));
#46556=CARTESIAN_POINT('Ctrl Pts',(-5.8435303439,-10.0864263463971,1.57297215988872));
#46557=CARTESIAN_POINT('Ctrl Pts',(-3.895686895933,-10.6220924815581,2.52887995839878));
#46558=CARTESIAN_POINT('Ctrl Pts',(0.0001666015754012,-11.1575607682146,
3.48561785406667));
#46559=CARTESIAN_POINT('Ctrl Pts',(3.896020099084,-10.6220466822612,2.5287981273656));
#46560=CARTESIAN_POINT('Ctrl Pts',(5.844030148626,-10.0862888918595,1.57272686930798));
#46561=CARTESIAN_POINT('Ctrl Pts',(-5.8435303439,-10.8186462754844,1.86224935014598));
#46562=CARTESIAN_POINT('Ctrl Pts',(-3.895686895933,-11.3231586997723,2.74792625098423));
#46563=CARTESIAN_POINT('Ctrl Pts',(0.0001666015754012,-11.8270683815162,
3.63586015557252));
#46564=CARTESIAN_POINT('Ctrl Pts',(3.896020099084,-11.3231155997237,2.74785030484635));
#46565=CARTESIAN_POINT('Ctrl Pts',(5.844030148626,-10.8185168151363,1.86202208116965));
#46566=CARTESIAN_POINT('Ctrl Pts',(-5.8435303439,-12.4568735769095,2.30089098965536));
#46567=CARTESIAN_POINT('Ctrl Pts',(-3.895686895933,-12.8710977176598,3.06727942798209));
#46568=CARTESIAN_POINT('Ctrl Pts',(0.0001666015754012,-13.2856328777696,
3.8324424554894));
#46569=CARTESIAN_POINT('Ctrl Pts',(3.896020099084,-12.8710622619296,3.067213982596));
#46570=CARTESIAN_POINT('Ctrl Pts',(5.844030148626,-12.4567672849836,2.3006943306413));
#46571=CARTESIAN_POINT('Ctrl Pts',(-5.8435303439,-15.0614254536644,2.34071384846666));
#46572=CARTESIAN_POINT('Ctrl Pts',(-3.895686895933,-15.2991206270769,3.03320173188209));
#46573=CARTESIAN_POINT('Ctrl Pts',(0.0001666015754012,-15.5368879417648,
3.72636712889203));
#46574=CARTESIAN_POINT('Ctrl Pts',(3.896020099084,-15.2991002905297,3.03314244454918));
#46575=CARTESIAN_POINT('Ctrl Pts',(5.844030148626,-15.0613644599276,2.34053615271556));
#46576=CARTESIAN_POINT('Ctrl Pts',(-5.8435303439,-17.685813504417,1.67939836341819));
#46577=CARTESIAN_POINT('Ctrl Pts',(-3.895686895933,-17.7477953301944,2.42360808198115));
#46578=CARTESIAN_POINT('Ctrl Pts',(0.0001666015754012,-17.8092308921404,
3.16660406935368));
#46579=CARTESIAN_POINT('Ctrl Pts',(3.896020099084,-17.747790075531,2.42354453257711));
#46580=CARTESIAN_POINT('Ctrl Pts',(5.844030148626,-17.6857975995771,1.67920739556743));
#46581=CARTESIAN_POINT('Ctrl Pts',(-5.8435303439,-19.259293374411,0.803936086515145));
#46582=CARTESIAN_POINT('Ctrl Pts',(-3.895686895933,-19.2409363781689,1.65690460410087));
#46583=CARTESIAN_POINT('Ctrl Pts',(0.0001666015754012,-19.2238042759609,
2.51236030102749));
#46584=CARTESIAN_POINT('Ctrl Pts',(3.896020099084,-19.2409378435011,1.65683143587068));
#46585=CARTESIAN_POINT('Ctrl Pts',(5.844030148626,-19.2592980849162,0.803717210669497));
#46586=CARTESIAN_POINT('Ctrl Pts',(-5.8435303439,-19.9729830806857,0.275591947000292));
#46587=CARTESIAN_POINT('Ctrl Pts',(-3.895686895933,-19.9313477701919,1.19822030152823));
#46588=CARTESIAN_POINT('Ctrl Pts',(0.0001666015754012,-19.8897492247631,
2.12096520787675));
#46589=CARTESIAN_POINT('Ctrl Pts',(3.896020099084,-19.9313513281736,1.1981413779533));
#46590=CARTESIAN_POINT('Ctrl Pts',(5.844030148626,-19.9729937645153,0.275355196075999));
#46591=CARTESIAN_POINT('Ctrl Pts',(-5.73278975426698,-10.3449510844138,
1.7128961701427));
#46592=CARTESIAN_POINT('Ctrl Pts',(-5.37911661672383,-10.4448068797057,
1.88163075288831));
#46593=CARTESIAN_POINT('Ctrl Pts',(-5.01642977825625,-10.5335803034939,
2.03722749340925));
#46594=CARTESIAN_POINT('Ctrl Pts',(-4.64634172525782,-10.611675775621,2.17794544599532));
#46595=CARTESIAN_POINT('Ctrl Pts',(-4.3719281748242,-10.6695821457552,2.28228524477033));
#46596=CARTESIAN_POINT('Ctrl Pts',(-4.09344547188132,-10.7216176124039,
2.37844082849794));
#46597=CARTESIAN_POINT('Ctrl Pts',(-3.81155096772038,-10.7679708202799,
2.46571664042017));
#46598=CARTESIAN_POINT('Ctrl Pts',(-3.57259918982531,-10.8072627584682,
2.53969719030044));
#46599=CARTESIAN_POINT('Ctrl Pts',(-3.33119591680233,-10.8424716474326,
2.60729655139232));
#46600=CARTESIAN_POINT('Ctrl Pts',(-3.08774152507161,-10.8737346886791,
2.66812502300776));
#46601=CARTESIAN_POINT('Ctrl Pts',(-3.04398962084052,-10.8793530617011,
2.67905668641183));
#46602=CARTESIAN_POINT('Ctrl Pts',(-3.00017147216096,-10.88484406648,2.68976978813144));
#46603=CARTESIAN_POINT('Ctrl Pts',(-2.95628940287459,-10.8902085973293,
2.70026223126147));
#46604=CARTESIAN_POINT('Ctrl Pts',(-2.75785502552652,-10.9144669642695,
2.74770897780801));
#46605=CARTESIAN_POINT('Ctrl Pts',(-2.55810778692668,-10.9362004020262,
2.79065903858132));
#46606=CARTESIAN_POINT('Ctrl Pts',(-2.35731447366229,-10.955388545368,2.82889657577336));
#46607=CARTESIAN_POINT('Ctrl Pts',(-2.16336116913836,-10.9739230460858,
2.86583155420807));
#46608=CARTESIAN_POINT('Ctrl Pts',(-1.96843184497064,-10.9900826889669,
2.89836954757001));
#46609=CARTESIAN_POINT('Ctrl Pts',(-1.77276694175945,-11.0038727784303,
2.92635796653381));
#46610=CARTESIAN_POINT('Ctrl Pts',(-1.58019158343941,-11.0174451226581,
2.9539044489244));
#46611=CARTESIAN_POINT('Ctrl Pts',(-1.38690369223543,-11.0287220802415,
2.97704375250748));
#46612=CARTESIAN_POINT('Ctrl Pts',(-1.19313249798695,-11.0377328161332,
2.99567340172542));
#46613=CARTESIAN_POINT('Ctrl Pts',(-0.994964448639617,-11.0469480143043,
3.01472577563405));
#46614=CARTESIAN_POINT('Ctrl Pts',(-0.796290914181298,-11.0537927389847,
3.02906107575225));
#46615=CARTESIAN_POINT('Ctrl Pts',(-0.597357085544801,-11.0583261912699,
3.0386198665503));
#46616=CARTESIAN_POINT('Ctrl Pts',(-0.408582158378835,-11.0626281349404,
3.04769052109439));
#46617=CARTESIAN_POINT('Ctrl Pts',(-0.219572842985093,-11.0648489562389,
3.05246026215182));
#46618=CARTESIAN_POINT('Ctrl Pts',(-0.0305386525764808,-11.0650644686467,
3.05292360453938));
#46619=CARTESIAN_POINT('Ctrl Pts',(-0.0203657988837101,-11.0650760664227,
3.05294853925784));
#46620=CARTESIAN_POINT('Ctrl Pts',(-0.0101928731518484,-11.0650818628657,
3.05296101346823));
#46621=CARTESIAN_POINT('Ctrl Pts',(-1.99080335683277E-5,-11.0650818718951,
3.05296103009418));
#46622=CARTESIAN_POINT('Ctrl Pts',(-1.32720223513428E-5,-11.065081871901,
3.05296103010502));
#46623=CARTESIAN_POINT('Ctrl Pts',(-6.63601115180548E-6,-11.0650818719044,
3.05296103011057));
#46624=CARTESIAN_POINT('Ctrl Pts',(3.19744231092045E-14,-11.0650818719054,
3.05296103011081));
#46625=CARTESIAN_POINT('Ctrl Pts',(0.189388142373251,-11.0650818994384,
3.05296103706175));
#46626=CARTESIAN_POINT('Ctrl Pts',(0.378762758287906,-11.0630739549068,
3.04863958591605));
#46627=CARTESIAN_POINT('Ctrl Pts',(0.567913157339342,-11.0589804436018,
3.03999975310335));
#46628=CARTESIAN_POINT('Ctrl Pts',(0.769315340839379,-11.0546217844652,
3.03080029488239));
#46629=CARTESIAN_POINT('Ctrl Pts',(0.970463320504467,-11.0478984432597,
3.01670457339992));
#46630=CARTESIAN_POINT('Ctrl Pts',(1.17110275584932,-11.0387476846565,2.99777185791181));
#46631=CARTESIAN_POINT('Ctrl Pts',(1.36689625026887,-11.0298179396119,2.97929641454797));
#46632=CARTESIAN_POINT('Ctrl Pts',(1.56220546893065,-11.018576867138,2.95621526529146));
#46633=CARTESIAN_POINT('Ctrl Pts',(1.75679405869412,-11.0049935453993,2.92863254316764));
#46634=CARTESIAN_POINT('Ctrl Pts',(1.95860682728074,-10.9909059374361,2.90002580150961));
#46635=CARTESIAN_POINT('Ctrl Pts',(2.15964446646054,-10.9742989289985,2.8665770390857));
#46636=CARTESIAN_POINT('Ctrl Pts',(2.3596433095925,-10.9551663818215,2.82845300631155));
#46637=CARTESIAN_POINT('Ctrl Pts',(2.55964215272445,-10.9360338346445,2.7903289735374));
#46638=CARTESIAN_POINT('Ctrl Pts',(2.75860219980856,-10.9143759250434,2.74753000555756));
#46639=CARTESIAN_POINT('Ctrl Pts',(2.95625978420382,-10.8902128218895,2.70026948337304));
#46640=CARTESIAN_POINT('Ctrl Pts',(3.19866256794929,-10.8605797395752,2.64231024961106));
#46641=CARTESIAN_POINT('Ctrl Pts',(3.43911507177877,-10.8270851551401,2.5776139620524));
#46642=CARTESIAN_POINT('Ctrl Pts',(3.67722557626171,-10.7895899938813,2.50655383829733));
#46643=CARTESIAN_POINT('Ctrl Pts',(3.96182040203707,-10.7447749660477,2.42162124120941));
#46644=CARTESIAN_POINT('Ctrl Pts',(4.2430695535221,-10.6942449885152,2.32759836386369));
#46645=CARTESIAN_POINT('Ctrl Pts',(4.52030419347271,-10.6378030703474,2.22518608067058));
#46646=CARTESIAN_POINT('Ctrl Pts',(4.88748869107178,-10.5630483522153,2.08954573371057));
#46647=CARTESIAN_POINT('Ctrl Pts',(5.24763102041744,-10.4779235063923,1.93919512435998));
#46648=CARTESIAN_POINT('Ctrl Pts',(5.59917725319807,-10.3820335990965,1.77581546490113));
#46649=CARTESIAN_POINT('Ctrl Pts',(5.64385361771994,-10.3698473998065,1.75505230904618));
#46650=CARTESIAN_POINT('Ctrl Pts',(5.68839114945533,-10.3574873916263,1.73407867881818));
#46651=CARTESIAN_POINT('Ctrl Pts',(5.73278665894458,-10.3449528049755,1.71289795467394));
#46652=CARTESIAN_POINT('Ctrl Pts',(-5.84445822842855,-10.3331482537831,
1.66691354819033));
#46653=CARTESIAN_POINT('Ctrl Pts',(-5.38771312971971,-10.4717359418486,
1.89165575395626));
#46654=CARTESIAN_POINT('Ctrl Pts',(-4.3554965874562,-10.7317200894033,2.33408242690297));
#46655=CARTESIAN_POINT('Ctrl Pts',(-2.68987671632907,-10.9928689957095,
2.82006056998998));
#46656=CARTESIAN_POINT('Ctrl Pts',(-0.896046561860736,-11.1236914322874,
3.0802434618201));
#46657=CARTESIAN_POINT('Ctrl Pts',(0.899212367975122,-11.1235788104192,
3.08001404244163));
#46658=CARTESIAN_POINT('Ctrl Pts',(2.69302899897811,-10.9925148949045,2.81937246391085));
#46659=CARTESIAN_POINT('Ctrl Pts',(4.35754598382318,-10.7312667792372,2.33328151229503));
#46660=CARTESIAN_POINT('Ctrl Pts',(5.38875361144458,-10.4714240747359,1.8911487048757));
#46661=CARTESIAN_POINT('Ctrl Pts',(5.84456702674697,-10.3331152084568,1.66686006128739));
#46662=CARTESIAN_POINT('Ctrl Pts',(-5.72526670899364,-10.051662855528,1.59453804482822));
#46663=CARTESIAN_POINT('Ctrl Pts',(-5.27774229481278,-10.1879516186282,
1.81303528671515));
#46664=CARTESIAN_POINT('Ctrl Pts',(-4.26639310686917,-10.4437163668707,
2.24334241603749));
#46665=CARTESIAN_POINT('Ctrl Pts',(-2.63466707886049,-10.7007617776932,
2.71620795356878));
#46666=CARTESIAN_POINT('Ctrl Pts',(-0.877615543970877,-10.8295728779202,
2.96940634106978));
#46667=CARTESIAN_POINT('Ctrl Pts',(0.880716270486781,-10.8294619741478,
2.96918307565484));
#46668=CARTESIAN_POINT('Ctrl Pts',(2.63775495090047,-10.7004131618419,2.71553833995515));
#46669=CARTESIAN_POINT('Ctrl Pts',(4.26840102530109,-10.4432703029748,2.24256325387882));
#46670=CARTESIAN_POINT('Ctrl Pts',(5.27876176978872,-10.1876449150383,1.81254230777516));
#46671=CARTESIAN_POINT('Ctrl Pts',(5.72537331154816,-10.0516303572414,1.59448604041269));
#46672=CARTESIAN_POINT('Ctrl Pts',(-5.71930850295601,-9.77801082274168,
1.74867595839893));
#46673=CARTESIAN_POINT('Ctrl Pts',(-5.27308497670522,-9.91296458113766,
1.96485547901025));
#46674=CARTESIAN_POINT('Ctrl Pts',(-4.26441701469436,-10.1663983984807,
2.39093719126511));
#46675=CARTESIAN_POINT('Ctrl Pts',(-2.63505179740053,-10.4215122664498,
2.86008785287843));
#46676=CARTESIAN_POINT('Ctrl Pts',(-0.878095819546688,-10.5495459780576,
3.1117583958528));
#46677=CARTESIAN_POINT('Ctrl Pts',(0.881197899559866,-10.5494356793196,
3.11153631405035));
#46678=CARTESIAN_POINT('Ctrl Pts',(2.63813754839394,-10.4211659428768,2.85942274077247));
#46679=CARTESIAN_POINT('Ctrl Pts',(4.26642002857102,-10.1659561458811,2.39016514377892));
#46680=CARTESIAN_POINT('Ctrl Pts',(5.27410150328015,-9.91266085860032,1.96436771771184));
#46681=CARTESIAN_POINT('Ctrl Pts',(5.71941478998875,-9.77797863935038,1.74862451318204));
#46682=CARTESIAN_POINT('Ctrl Pts',(-5.8304606616367,-9.69020667453587,2.02906075227467));
#46683=CARTESIAN_POINT('Ctrl Pts',(-5.37677190025951,-9.82565779738564,
2.24835754410253));
#46684=CARTESIAN_POINT('Ctrl Pts',(-4.35085467555363,-10.0801654743651,
2.68085673877077));
#46685=CARTESIAN_POINT('Ctrl Pts',(-2.69078117464156,-10.3367762696711,
3.15810692828297));
#46686=CARTESIAN_POINT('Ctrl Pts',(-0.89717515569234,-10.4657722550533,
3.41470022626425));
#46687=CARTESIAN_POINT('Ctrl Pts',(0.900344142508115,-10.4656610546937,
3.41447358771451));
#46688=CARTESIAN_POINT('Ctrl Pts',(2.69392847455747,-10.3364275545085,3.15742939829163));
#46689=CARTESIAN_POINT('Ctrl Pts',(4.35289254910898,-10.0797211187514,2.68007253983937));
#46690=CARTESIAN_POINT('Ctrl Pts',(5.3778054549422,-9.82535293419236,2.24786275370891));
#46691=CARTESIAN_POINT('Ctrl Pts',(5.83056871866019,-9.69017436905015,2.02900857919085));
#46692=CARTESIAN_POINT('Ctrl Pts',(-5.72001725923566,-9.72697394243655,
2.05943194359944));
#46693=CARTESIAN_POINT('Ctrl Pts',(-5.48693272988403,-9.79479243900217,
2.1698632189192));
#46694=CARTESIAN_POINT('Ctrl Pts',(-5.24893985465217,-9.8578898842069,2.27505821719543));
#46695=CARTESIAN_POINT('Ctrl Pts',(-5.00626021853139,-9.91632228116233,
2.37435968097908));
#46696=CARTESIAN_POINT('Ctrl Pts',(-4.81288427723629,-9.96288333566201,
2.45348669113162));
#46697=CARTESIAN_POINT('Ctrl Pts',(-4.61653254429665,-10.0064820069781,
2.5288708354457));
#46698=CARTESIAN_POINT('Ctrl Pts',(-4.41732289584036,-10.0471397417556,
2.60015753014603));
#46699=CARTESIAN_POINT('Ctrl Pts',(-4.40009339203155,-10.0506562009313,
2.60632306674215));
#46700=CARTESIAN_POINT('Ctrl Pts',(-4.38284251386637,-10.0541506570791,
2.6124579399829));
#46701=CARTESIAN_POINT('Ctrl Pts',(-4.36557037135436,-10.0576231265581,
2.61856191382665));
#46702=CARTESIAN_POINT('Ctrl Pts',(-4.13177327318589,-10.1046267502896,
2.70118579045179));
#46703=CARTESIAN_POINT('Ctrl Pts',(-3.89408346669447,-10.1475966538231,
2.77817366986499));
#46704=CARTESIAN_POINT('Ctrl Pts',(-3.65276146729705,-10.1865292264382,
2.84906061991673));
#46705=CARTESIAN_POINT('Ctrl Pts',(-3.53210046759834,-10.2059955127458,
2.8845040949426));
#46706=CARTESIAN_POINT('Ctrl Pts',(-3.41053208906834,-10.2244515842033,
2.9184231578225));
#46707=CARTESIAN_POINT('Ctrl Pts',(-3.28809316452347,-10.2418917665002,
2.95076478016178));
#46708=CARTESIAN_POINT('Ctrl Pts',(-3.22687370225103,-10.2506118576487,
2.96693559133142));
#46709=CARTESIAN_POINT('Ctrl Pts',(-3.16543659837793,-10.2590779517068,
2.98271203496152));
#46710=CARTESIAN_POINT('Ctrl Pts',(-3.10378680031152,-10.2672889927752,
2.99808788577522));
#46711=CARTESIAN_POINT('Ctrl Pts',(-3.07296190127832,-10.2713945133094,
3.00577581118207));
#46712=CARTESIAN_POINT('Ctrl Pts',(-3.04208382849723,-10.2754362692712,
3.01336358796922));
#46713=CARTESIAN_POINT('Ctrl Pts',(-3.01115321055681,-10.2794141145398,
3.02085044997317));
#46714=CARTESIAN_POINT('Ctrl Pts',(-2.98624862142243,-10.2826169798121,
3.02687869106661));
#46715=CARTESIAN_POINT('Ctrl Pts',(-2.96051439371824,-10.2858783416408,
3.03303033589897));
#46716=CARTESIAN_POINT('Ctrl Pts',(-2.93587242134819,-10.2889564309938,
3.03884835934926));
#46717=CARTESIAN_POINT('Ctrl Pts',(-2.929909936501,-10.2897012196353,3.04025611503302));
#46718=CARTESIAN_POINT('Ctrl Pts',(-2.92401146545564,-10.2904353978881,
3.04164453878627));
#46719=CARTESIAN_POINT('Ctrl Pts',(-2.91820435563567,-10.2911557637968,
3.04300753181412));
#46720=CARTESIAN_POINT('Ctrl Pts',(-2.83088075353848,-10.3019881654436,
3.06350334892712));
#46721=CARTESIAN_POINT('Ctrl Pts',(-2.74333417703633,-10.3123017606963,
3.08311072788639));
#46722=CARTESIAN_POINT('Ctrl Pts',(-2.65557894832266,-10.3221031860875,
3.10181531402008));
#46723=CARTESIAN_POINT('Ctrl Pts',(-2.39760263918788,-10.3509166890975,
3.15680166828517));
#46724=CARTESIAN_POINT('Ctrl Pts',(-2.13782516201486,-10.3753059013279,
3.20398885075858));
#46725=CARTESIAN_POINT('Ctrl Pts',(-1.8767291264866,-10.3953879991318,3.24316256673323));
#46726=CARTESIAN_POINT('Ctrl Pts',(-1.61583159188067,-10.4154548293161,
3.28230650049101));
#46727=CARTESIAN_POINT('Ctrl Pts',(-1.35361695580228,-10.431221027104,3.31344948606628));
#46728=CARTESIAN_POINT('Ctrl Pts',(-1.09054431580665,-10.4427785152057,
3.3363382803531));
#46729=CARTESIAN_POINT('Ctrl Pts',(-1.02152917496517,-10.445810535826,3.34234298445849));
#46730=CARTESIAN_POINT('Ctrl Pts',(-0.952454888250652,-10.4485527672398,
3.34777937920162));
#46731=CARTESIAN_POINT('Ctrl Pts',(-0.883329562900901,-10.4510065925464,
3.35264239616797));
#46732=CARTESIAN_POINT('Ctrl Pts',(-0.621402695948059,-10.4603045274398,
3.37106914195888));
#46733=CARTESIAN_POINT('Ctrl Pts',(-0.358743620959177,-10.465463405017,
3.38126706659519));
#46734=CARTESIAN_POINT('Ctrl Pts',(-0.0958570272718549,-10.4664724902806,
3.38326282124112));
#46735=CARTESIAN_POINT('Ctrl Pts',(-0.0639000864720908,-10.466595156399,
3.38350542856536));
#46736=CARTESIAN_POINT('Ctrl Pts',(-0.0319397761689494,-10.4666564718144,
3.38362677429207));
#46737=CARTESIAN_POINT('Ctrl Pts',(2.300178284668E-5,-10.4666563938114,
3.38362685957177));
#46738=CARTESIAN_POINT('Ctrl Pts',(0.260337415711732,-10.4666557585314,
3.38362755411516));
#46739=CARTESIAN_POINT('Ctrl Pts',(0.520480755586545,-10.4625880719849,
3.37557893746241));
#46740=CARTESIAN_POINT('Ctrl Pts',(0.77997268513999,-10.4544603514888,3.35948138375795));
#46741=CARTESIAN_POINT('Ctrl Pts',(0.81547805772961,-10.4533482639375,3.35727881182039));
#46742=CARTESIAN_POINT('Ctrl Pts',(0.850971231436825,-10.452160130752,3.3549254805135));
#46743=CARTESIAN_POINT('Ctrl Pts',(0.886450970381633,-10.4508959359216,
3.35242132307833));
#46744=CARTESIAN_POINT('Ctrl Pts',(1.08153280298439,-10.4439448857833,3.33865246129671));
#46745=CARTESIAN_POINT('Ctrl Pts',(1.27620873109396,-10.4346949219051,3.32032490351649));
#46746=CARTESIAN_POINT('Ctrl Pts',(1.47030049461408,-10.4231094685303,3.29755584435938));
#46747=CARTESIAN_POINT('Ctrl Pts',(1.71399050157766,-10.408563466359,3.268968375814));
#46748=CARTESIAN_POINT('Ctrl Pts',(1.95674662779223,-10.3903532933778,3.23333124378285));
#46749=CARTESIAN_POINT('Ctrl Pts',(2.19819766295024,-10.368396071073,3.19083022181142));
#46750=CARTESIAN_POINT('Ctrl Pts',(2.31892318052924,-10.3574174599205,3.1695797108257));
#46751=CARTESIAN_POINT('Ctrl Pts',(2.43932260395416,-10.345501247044,3.14661428567981));
#46752=CARTESIAN_POINT('Ctrl Pts',(2.55935059295051,-10.3326319233828,3.12196359574265));
#46753=CARTESIAN_POINT('Ctrl Pts',(2.59249782324256,-10.3290778987035,3.11515599942251));
#46754=CARTESIAN_POINT('Ctrl Pts',(2.62561677822834,-10.3254511436961,3.10821993941185));
#46755=CARTESIAN_POINT('Ctrl Pts',(2.65870640247661,-10.3217513385284,3.10115598276616));
#46756=CARTESIAN_POINT('Ctrl Pts',(2.68552647536097,-10.3187525421834,3.09543044684989));
#46757=CARTESIAN_POINT('Ctrl Pts',(2.71232727914222,-10.3157057549886,3.08962088827545));
#46758=CARTESIAN_POINT('Ctrl Pts',(2.73910840455801,-10.3126107653246,3.08372779963449));
#46759=CARTESIAN_POINT('Ctrl Pts',(2.76901975340948,-10.3091540280107,3.0771459167817));
#46760=CARTESIAN_POINT('Ctrl Pts',(2.79890649941338,-10.305637192199,3.07045976831403));
#46761=CARTESIAN_POINT('Ctrl Pts',(2.82876795903543,-10.3020600177251,3.06366991148607));
#46762=CARTESIAN_POINT('Ctrl Pts',(2.85294750930066,-10.2991634925353,3.05817199924254));
#46763=CARTESIAN_POINT('Ctrl Pts',(2.8763080945304,-10.2963257491386,3.05279238073469));
#46764=CARTESIAN_POINT('Ctrl Pts',(2.90079864213134,-10.2933080492701,3.0470793056848));
#46765=CARTESIAN_POINT('Ctrl Pts',(2.90655363219694,-10.2925989253645,3.04573680037655));
#46766=CARTESIAN_POINT('Ctrl Pts',(2.9123709587508,-10.2918797545079,3.04437569618811));
#46767=CARTESIAN_POINT('Ctrl Pts',(2.9182757973104,-10.2911472306701,3.04298978108805));
#46768=CARTESIAN_POINT('Ctrl Pts',(3.17624357856515,-10.2591450773108,2.98244258072667));
#46769=CARTESIAN_POINT('Ctrl Pts',(3.43059704783037,-10.2227651596086,2.91473261962076));
#46770=CARTESIAN_POINT('Ctrl Pts',(3.68103189504611,-10.1820138635033,2.84048532916211));
#46771=CARTESIAN_POINT('Ctrl Pts',(3.93146674226184,-10.141262567398,2.76623803870345));
#46772=CARTESIAN_POINT('Ctrl Pts',(4.17798321528555,-10.0961399671612,2.68545293148422));
#46773=CARTESIAN_POINT('Ctrl Pts',(4.42027976008899,-10.0466389069888,2.59870198645564));
#46774=CARTESIAN_POINT('Ctrl Pts',(4.67259159069087,-9.99509172905041,2.50836520610923));
#46775=CARTESIAN_POINT('Ctrl Pts',(4.92032803560847,-9.93879687513458,2.41155906436459));
#46776=CARTESIAN_POINT('Ctrl Pts',(5.16324371845964,-9.87774347039952,2.30887781548181));
#46777=CARTESIAN_POINT('Ctrl Pts',(5.35177735600155,-9.83035821991295,2.22918403395236));
#46778=CARTESIAN_POINT('Ctrl Pts',(5.53740701620603,-9.78010618807128,2.1459500771757));
#46779=CARTESIAN_POINT('Ctrl Pts',(5.72001441299688,-9.72697459952105,2.05943398518195));
#46780=CARTESIAN_POINT('Origin',(5.6,9.91330329119712,16.8993688492374));
#46781=CARTESIAN_POINT('',(5.99999999995608,9.91329603789449,16.8993703023573));
#46782=CARTESIAN_POINT('',(5.59336167795831,10.1144355810365,17.2450590896867));
#46783=CARTESIAN_POINT('Origin',(5.6,9.91330329119712,16.8993688492374));
#46784=CARTESIAN_POINT('',(5.736443493912,10.2877312271804,16.9337809062588));
#46785=CARTESIAN_POINT('Origin',(5.59997427807905,9.91328074797341,16.8993778521222));
#46786=CARTESIAN_POINT('Origin',(5.599999999773,9.91330329131382,16.8993688489353));
#46787=CARTESIAN_POINT('Ctrl Pts',(5.99999999997507,9.91330135657847,16.8993650110572));
#46788=CARTESIAN_POINT('Ctrl Pts',(5.99999999997507,9.83522888887418,16.9447895967211));
#46789=CARTESIAN_POINT('Ctrl Pts',(5.99999999997507,9.75700380943156,16.989952878335));
#46790=CARTESIAN_POINT('Ctrl Pts',(5.99999999997507,9.67862816205461,17.0348534691249));
#46791=CARTESIAN_POINT('Ctrl Pts',(6.00000263486327,10.032695805171,17.1045706743813));
#46792=CARTESIAN_POINT('Ctrl Pts',(6.00000263486327,9.95416474484471,17.1502620775629));
#46793=CARTESIAN_POINT('Ctrl Pts',(6.00000263486327,9.87548026973953,17.1956905916351));
#46794=CARTESIAN_POINT('Ctrl Pts',(6.00000263486327,9.79664425061367,17.240854924572));
#46795=CARTESIAN_POINT('Ctrl Pts',(5.83074066841791,10.1164175341797,17.2484649101538));
#46796=CARTESIAN_POINT('Ctrl Pts',(5.83074066841791,10.0375648997121,17.2943434110114));
#46797=CARTESIAN_POINT('Ctrl Pts',(5.83074066841791,9.95855828735685,17.339957911285));
#46798=CARTESIAN_POINT('Ctrl Pts',(5.83074066841791,9.87939944652955,17.3853071853885));
#46799=CARTESIAN_POINT('Ctrl Pts',(5.59336110044213,10.1144359114724,17.2450590549684));
#46800=CARTESIAN_POINT('Ctrl Pts',(5.59336110044213,10.0355908883956,17.2909331273823));
#46801=CARTESIAN_POINT('Ctrl Pts',(5.59336110044213,9.95659190076084,17.3365432255189));
#46802=CARTESIAN_POINT('Ctrl Pts',(5.59336110044213,9.8774407008502,17.3818881222188));
#46803=CARTESIAN_POINT('',(5.59336169566021,9.87744142947385,17.3818877157234));
#46804=CARTESIAN_POINT('Origin',(5.59336169595361,7.4927251628836,13.0987219083732));
#46805=CARTESIAN_POINT('',(6.,9.67863108609234,17.0348569101268));
#46806=CARTESIAN_POINT('Origin',(5.6,9.67863108611231,17.0348569102122));
#46807=CARTESIAN_POINT('Ctrl Pts',(5.99999999999163,9.91329301289976,16.8993720623907));
#46808=CARTESIAN_POINT('Ctrl Pts',(5.99999999999168,9.88722393978031,16.9145397247202));
#46809=CARTESIAN_POINT('Ctrl Pts',(5.9999999999997,9.86114407693772,16.9296767195884));
#46810=CARTESIAN_POINT('Ctrl Pts',(5.9999999999997,9.83508082014215,16.9447638792478));
#46811=CARTESIAN_POINT('Ctrl Pts',(5.9999999999997,9.80901756334656,16.9598510389072));
#46812=CARTESIAN_POINT('Ctrl Pts',(5.9999999999997,9.78297091259799,16.9748883633578));
#46813=CARTESIAN_POINT('Ctrl Pts',(5.9999999999997,9.75690044719229,16.9899010654912));
#46814=CARTESIAN_POINT('Ctrl Pts',(5.9999999999997,9.73082998178661,17.0049137676245));
#46815=CARTESIAN_POINT('Ctrl Pts',(5.9999999999997,9.7047357017238,17.0199018474406));
#46816=CARTESIAN_POINT('Ctrl Pts',(5.9999999999997,9.67863108609234,17.0348569101268));
#46817=CARTESIAN_POINT('Origin',(5.6,9.67863108603356,17.0348569100686));
#46818=CARTESIAN_POINT('',(5.73644276526939,9.52121697668264,17.3763304375098));
#46819=CARTESIAN_POINT('Origin',(5.6,9.67863108603356,17.0348569100686));
#46820=CARTESIAN_POINT('Origin',(5.600000004204,9.67863108709891,17.0348569087034));
#46821=CARTESIAN_POINT('Ctrl Pts',(5.99928507671022,9.77920217854224,17.0543525003981));
#46822=CARTESIAN_POINT('Ctrl Pts',(5.99928507671022,9.74894839966019,17.0407709830063));
#46823=CARTESIAN_POINT('Ctrl Pts',(5.99928507671022,9.27203920735655,16.8237867818179));
#46824=CARTESIAN_POINT('Ctrl Pts',(5.99928507671022,8.38193522943825,16.330354291202));
#46825=CARTESIAN_POINT('Ctrl Pts',(5.99928507671022,7.21246426313331,15.4323267873748));
#46826=CARTESIAN_POINT('Ctrl Pts',(5.99928507671022,6.18849730659679,14.3709116157364));
#46827=CARTESIAN_POINT('Ctrl Pts',(5.99928507671022,5.3327105314028,13.1688951809427));
#46828=CARTESIAN_POINT('Ctrl Pts',(5.99928507671022,4.66383020186651,11.8527237226933));
#46829=CARTESIAN_POINT('Ctrl Pts',(5.99928507671022,4.224790911033,10.5321726316798));
#46830=CARTESIAN_POINT('Ctrl Pts',(5.99928507671022,4.05899861711237,9.64833292798276));
#46831=CARTESIAN_POINT('Ctrl Pts',(5.99928507671022,4.00882230478759,9.24471639752885));
#46832=CARTESIAN_POINT('Ctrl Pts',(6.0106308763342,9.70160290773497,17.2272498486038));
#46833=CARTESIAN_POINT('Ctrl Pts',(6.0106308763342,9.67076783714877,17.2134071734354));
#46834=CARTESIAN_POINT('Ctrl Pts',(6.0106308763342,9.18470187459673,16.9922547580898));
#46835=CARTESIAN_POINT('Ctrl Pts',(6.0106308763342,8.27768603745146,16.4894560547017));
#46836=CARTESIAN_POINT('Ctrl Pts',(6.0106308763342,7.08568030104689,15.5741219743995));
#46837=CARTESIAN_POINT('Ctrl Pts',(6.0106308763342,6.04221997992615,14.4924954167108));
#46838=CARTESIAN_POINT('Ctrl Pts',(6.0106308763342,5.16996731271864,13.2673652494844));
#46839=CARTESIAN_POINT('Ctrl Pts',(6.0106308763342,4.4883276541397,11.9260693537073));
#46840=CARTESIAN_POINT('Ctrl Pts',(6.0106308763342,4.04084623666606,10.5801434939708));
#46841=CARTESIAN_POINT('Ctrl Pts',(6.0106308763342,3.87189639823667,9.67946934988362));
#46842=CARTESIAN_POINT('Ctrl Pts',(6.0106308763342,3.82075680084142,9.26809143104854));
#46843=CARTESIAN_POINT('Ctrl Pts',(5.90351527979004,9.63722337780829,17.3706925625164));
#46844=CARTESIAN_POINT('Ctrl Pts',(5.90351527979004,9.60590604384287,17.3566332201771));
#46845=CARTESIAN_POINT('Ctrl Pts',(5.90351527979004,9.11224325005284,17.1320226838286));
#46846=CARTESIAN_POINT('Ctrl Pts',(5.90351527979004,8.19119664256615,16.6214533871243));
#46847=CARTESIAN_POINT('Ctrl Pts',(5.90351527979004,6.98049513891304,15.6917610629));
#46848=CARTESIAN_POINT('Ctrl Pts',(5.90351527979004,5.92086232498848,14.5933663124247));
#46849=CARTESIAN_POINT('Ctrl Pts',(5.90351527979004,5.03494888009271,13.3490600471091));
#46850=CARTESIAN_POINT('Ctrl Pts',(5.90351527979004,4.34272356011029,11.9869198900282));
#46851=CARTESIAN_POINT('Ctrl Pts',(5.90351527979004,3.88823820897759,10.6199420839871));
#46852=CARTESIAN_POINT('Ctrl Pts',(5.90351527979004,3.71666874243767,9.70530139939471));
#46853=CARTESIAN_POINT('Ctrl Pts',(5.90351527979004,3.66472996433574,9.28748431521313));
#46854=CARTESIAN_POINT('Ctrl Pts',(5.72195022899939,9.61342435717959,17.42371867364));
#46855=CARTESIAN_POINT('Ctrl Pts',(5.72195022899939,9.5819287461083,17.4095792364841));
#46856=CARTESIAN_POINT('Ctrl Pts',(5.72195022899939,9.08545765061893,17.1836903451488));
#46857=CARTESIAN_POINT('Ctrl Pts',(5.72195022899939,8.15922432316945,16.6702485125462));
#46858=CARTESIAN_POINT('Ctrl Pts',(5.72195022899939,6.94161160176299,15.7352484120208));
#46859=CARTESIAN_POINT('Ctrl Pts',(5.72195022899939,5.87600034267062,14.6306550054462));
#46860=CARTESIAN_POINT('Ctrl Pts',(5.72195022899939,4.98503695207054,13.379259959662));
#46861=CARTESIAN_POINT('Ctrl Pts',(5.72195022899939,4.28889845698094,12.0094143563736));
#46862=CARTESIAN_POINT('Ctrl Pts',(5.72195022899939,3.83182397912037,10.634654329726));
#46863=CARTESIAN_POINT('Ctrl Pts',(5.72195022899939,3.65928612117585,9.71485066885913));
#46864=CARTESIAN_POINT('Ctrl Pts',(5.72195022899939,3.60705191193102,9.2946532344466));
#46865=CARTESIAN_POINT('',(5.999995708873,3.99788407334609,9.34660788812901));
#46866=CARTESIAN_POINT('Ctrl Pts',(5.99999999999973,9.67863108609234,17.0348569101268));
#46867=CARTESIAN_POINT('Ctrl Pts',(5.99999999999973,9.53996482697851,16.9709229523272));
#46868=CARTESIAN_POINT('Ctrl Pts',(6.00000000003745,9.40322990797334,16.9040238345851));
#46869=CARTESIAN_POINT('Ctrl Pts',(5.99999999795223,9.26832001839706,16.8341585314163));
#46870=CARTESIAN_POINT('Ctrl Pts',(5.99999999586008,9.13296247354946,16.7640614026095));
#46871=CARTESIAN_POINT('Ctrl Pts',(5.99999999148617,8.99944169513547,16.6909781287824));
#46872=CARTESIAN_POINT('Ctrl Pts',(5.99999999087358,8.86767321977893,16.614860483692));
#46873=CARTESIAN_POINT('Ctrl Pts',(5.99999999026198,8.73611954089724,16.5388669183695));
#46874=CARTESIAN_POINT('Ctrl Pts',(5.99999999695625,8.60631206863277,16.4598486138468));
#46875=CARTESIAN_POINT('Ctrl Pts',(5.99999999953313,8.47819538350943,16.3777143843333));
#46876=CARTESIAN_POINT('Ctrl Pts',(5.99999999982103,8.46388161372689,16.368537980406));
#46877=CARTESIAN_POINT('Ctrl Pts',(5.99999999999973,8.44958898200459,16.359322640206));
#46878=CARTESIAN_POINT('Ctrl Pts',(5.99999999999973,8.43531743665976,16.3500682051006));
#46879=CARTESIAN_POINT('Ctrl Pts',(5.99999999999973,8.41951507644111,16.3398211075634));
#46880=CARTESIAN_POINT('Ctrl Pts',(5.99999999977974,8.40373799579134,16.3295268932048));
#46881=CARTESIAN_POINT('Ctrl Pts',(5.99999999940211,8.38798676299758,16.3191857879634));
#46882=CARTESIAN_POINT('Ctrl Pts',(5.99999999572733,8.23470703683931,16.218553551723));
#46883=CARTESIAN_POINT('Ctrl Pts',(5.99999998184256,8.08387696920508,16.1134769902102));
#46884=CARTESIAN_POINT('Ctrl Pts',(5.99999998033334,7.93593246473448,16.0042029928132));
#46885=CARTESIAN_POINT('Ctrl Pts',(5.99999997882271,7.78785045815604,15.8948274343273));
#46886=CARTESIAN_POINT('Ctrl Pts',(5.99999998731003,7.64265976295762,15.7812468735777));
#46887=CARTESIAN_POINT('Ctrl Pts',(5.99999999411985,7.5007707703766,15.6637536647565));
#46888=CARTESIAN_POINT('Ctrl Pts',(5.99999999739301,7.43257160181644,15.6072803682216));
#46889=CARTESIAN_POINT('Ctrl Pts',(5.99999999999973,7.36513478078999,15.5499037886171));
#46890=CARTESIAN_POINT('Ctrl Pts',(5.99999999999973,7.29850328839949,15.4916598064483));
#46891=CARTESIAN_POINT('Ctrl Pts',(5.99999999999973,7.27238327152499,15.4688277529777));
#46892=CARTESIAN_POINT('Ctrl Pts',(5.99999999960413,7.24638785264082,15.4458614503161));
#46893=CARTESIAN_POINT('Ctrl Pts',(5.99999999898864,7.22051776537669,15.4227616312461));
#46894=CARTESIAN_POINT('Ctrl Pts',(5.99999999507859,7.05617055376932,15.276013349571));
#46895=CARTESIAN_POINT('Ctrl Pts',(5.99999998615654,6.89687872218253,15.1238800776715));
#46896=CARTESIAN_POINT('Ctrl Pts',(5.99999998771983,6.74283048209746,14.9666009211881));
#46897=CARTESIAN_POINT('Ctrl Pts',(5.99999998928313,6.58878224201239,14.8093217647046));
#46898=CARTESIAN_POINT('Ctrl Pts',(5.99999999999973,6.43997714680652,14.6468962856073));
#46899=CARTESIAN_POINT('Ctrl Pts',(5.99999999999973,6.29664110038306,14.4795249794001));
#46900=CARTESIAN_POINT('Ctrl Pts',(5.99999999999973,6.26385436913115,14.4412404154483));
#46901=CARTESIAN_POINT('Ctrl Pts',(5.99999999934668,6.23135170199707,14.4026986427203));
#46902=CARTESIAN_POINT('Ctrl Pts',(5.99999999845572,6.19913907434236,14.363905280557));
#46903=CARTESIAN_POINT('Ctrl Pts',(5.99999999449761,6.05603309717716,14.1915641086601));
#46904=CARTESIAN_POINT('Ctrl Pts',(5.99999998895131,5.91865446118546,14.0142547237431));
#46905=CARTESIAN_POINT('Ctrl Pts',(5.99999999115152,5.78742187753508,13.8325315583979));
#46906=CARTESIAN_POINT('Ctrl Pts',(5.99999999312719,5.66958213385772,13.6693540103466));
#46907=CARTESIAN_POINT('Ctrl Pts',(5.99999999999973,5.55669768563095,13.5026183339827));
#46908=CARTESIAN_POINT('Ctrl Pts',(5.99999999999973,5.44904317681685,13.3327476292601));
#46909=CARTESIAN_POINT('Ctrl Pts',(5.99999999999973,5.41325256681909,13.2762727429805));
#46910=CARTESIAN_POINT('Ctrl Pts',(5.99999999913626,5.37804226723512,13.2194505286227));
#46911=CARTESIAN_POINT('Ctrl Pts',(5.99999999780773,5.34341678808384,13.1622879102264));
#46912=CARTESIAN_POINT('Ctrl Pts',(5.99999999336881,5.22772507043026,12.971294408622));
#46913=CARTESIAN_POINT('Ctrl Pts',(5.99999998477713,5.11855861819962,12.7765024096211));
#46914=CARTESIAN_POINT('Ctrl Pts',(5.99999998688352,5.01608477820067,12.5781968544433));
#46915=CARTESIAN_POINT('Ctrl Pts',(5.99999998863007,4.93111681483905,12.4137683608206));
#46916=CARTESIAN_POINT('Ctrl Pts',(5.99999999999973,4.85075089138975,12.2469236106697));
#46917=CARTESIAN_POINT('Ctrl Pts',(5.99999999999973,4.77510784589458,12.0778154581379));
#46918=CARTESIAN_POINT('Ctrl Pts',(5.99999999999973,4.74092204835138,12.001389436056));
#46919=CARTESIAN_POINT('Ctrl Pts',(5.99999999683353,4.70768988233517,11.924503809641));
#46920=CARTESIAN_POINT('Ctrl Pts',(5.99999999319074,4.67543337998425,11.8471991538665));
#46921=CARTESIAN_POINT('Ctrl Pts',(5.99999998466666,4.59995360841245,11.6663073232577));
#46922=CARTESIAN_POINT('Ctrl Pts',(5.99999997595978,4.52981981238128,11.4831198183697));
#46923=CARTESIAN_POINT('Ctrl Pts',(5.99999997954453,4.4651956975605,11.2981805868859));
#46924=CARTESIAN_POINT('Ctrl Pts',(5.99999998312928,4.40057158273971,11.1132413554021));
#46925=CARTESIAN_POINT('Ctrl Pts',(5.99999999999973,4.34145727180275,10.9265509189428));
#46926=CARTESIAN_POINT('Ctrl Pts',(5.99999999999973,4.2879615125261,10.7386680750648));
#46927=CARTESIAN_POINT('Ctrl Pts',(5.99999999999973,4.2606285677341,10.6426718415593));
#46928=CARTESIAN_POINT('Ctrl Pts',(5.99999999545167,4.23478514967479,10.5463642320464));
#46929=CARTESIAN_POINT('Ctrl Pts',(5.99999999307292,4.2104123041608,10.4497165385551));
#46930=CARTESIAN_POINT('Ctrl Pts',(5.99999998940938,4.17287556936319,10.3008689681184));
#46931=CARTESIAN_POINT('Ctrl Pts',(5.99999999031161,4.13882446531637,10.151215309579));
#46932=CARTESIAN_POINT('Ctrl Pts',(5.99999999276242,4.10822755632143,10.0006714395986));
#46933=CARTESIAN_POINT('Ctrl Pts',(5.99999999520027,4.0777923342782,9.85092310682235));
#46934=CARTESIAN_POINT('Ctrl Pts',(5.99999999786782,4.05077479935226,9.70029349538257));
#46935=CARTESIAN_POINT('Ctrl Pts',(5.99999999875693,4.02719432996178,9.54868945906619));
#46936=CARTESIAN_POINT('Ctrl Pts',(5.99999999915083,4.01674728370481,9.48152309550002));
#46937=CARTESIAN_POINT('Ctrl Pts',(5.99999999931875,4.00697554674536,9.4141653731669));
#46938=CARTESIAN_POINT('Ctrl Pts',(5.99999999931447,3.99788407309719,9.34660788816251));
#46939=CARTESIAN_POINT('',(5.732785250275,3.68906751028189,9.81543787979773));
#46940=CARTESIAN_POINT('Ctrl Pts',(5.73644276397758,9.52121697613018,17.3763304378322));
#46941=CARTESIAN_POINT('Ctrl Pts',(5.73708792253423,9.11866917743972,17.1904707590909));
#46942=CARTESIAN_POINT('Ctrl Pts',(5.7376256311299,8.72821037826326,16.9787094793335));
#46943=CARTESIAN_POINT('Ctrl Pts',(5.73805595545524,8.35333662058844,16.7430677587439));
#46944=CARTESIAN_POINT('Ctrl Pts',(5.73812189676484,8.29589235108936,16.7069588921571));
#46945=CARTESIAN_POINT('Ctrl Pts',(5.7381853165236,8.23881395572367,16.6702892265697));
#46946=CARTESIAN_POINT('Ctrl Pts',(5.73824621493853,8.18211392296712,16.6330659762314));
#46947=CARTESIAN_POINT('Ctrl Pts',(5.7386514731337,7.80479453019456,16.3853579321291));
#46948=CARTESIAN_POINT('Ctrl Pts',(5.73894507723332,7.44423382954565,16.1131376200729));
#46949=CARTESIAN_POINT('Ctrl Pts',(5.73912707304862,7.10336506027343,15.8189084737335));
#46950=CARTESIAN_POINT('Ctrl Pts',(5.73915087280096,7.05878935244757,15.7804318702914));
#46951=CARTESIAN_POINT('Ctrl Pts',(5.73917276389451,7.01455034381636,15.7415788431653));
#46952=CARTESIAN_POINT('Ctrl Pts',(5.73919274639104,6.97065454663181,15.7023549458792));
#46953=CARTESIAN_POINT('Ctrl Pts',(5.73934700322414,6.63179665406559,15.3995622407664));
#46954=CARTESIAN_POINT('Ctrl Pts',(5.73938752574635,6.31339410984921,15.0746719519374));
#46955=CARTESIAN_POINT('Ctrl Pts',(5.73931432087574,6.01802949013874,14.7306311257563));
#46956=CARTESIAN_POINT('Ctrl Pts',(5.73930537009204,5.98191516059527,14.688565140381));
#46957=CARTESIAN_POINT('Ctrl Pts',(5.73929471903226,5.94614520943738,14.646212803436));
#46958=CARTESIAN_POINT('Ctrl Pts',(5.73928236766916,5.91072432464435,14.6035794599326));
#46959=CARTESIAN_POINT('Ctrl Pts',(5.7391813575988,5.62105054233214,14.2549218265221));
#46960=CARTESIAN_POINT('Ctrl Pts',(5.73896663328804,5.35472454602451,13.8874741273139));
#46961=CARTESIAN_POINT('Ctrl Pts',(5.73863815938408,5.11384108228221,13.5046257890557));
#46962=CARTESIAN_POINT('Ctrl Pts',(5.73859603620214,5.08295041533258,13.4555296812299));
#46963=CARTESIAN_POINT('Ctrl Pts',(5.73855204233368,5.05247812384846,13.4061802442968));
#46964=CARTESIAN_POINT('Ctrl Pts',(5.73850617766587,5.02242859618563,13.3565845722194));
#46965=CARTESIAN_POINT('Ctrl Pts',(5.73815298353459,4.7910235228329,12.9746587641395));
#46966=CARTESIAN_POINT('Ctrl Pts',(5.73768884855725,4.58469079279698,12.5781343479219));
#46967=CARTESIAN_POINT('Ctrl Pts',(5.73711370893166,4.40507707792291,12.1703805322858));
#46968=CARTESIAN_POINT('Ctrl Pts',(5.73703020600002,4.37899945939716,12.1111798834711));
#46969=CARTESIAN_POINT('Ctrl Pts',(5.73694436300226,4.35348502659766,12.0517424478515));
#46970=CARTESIAN_POINT('Ctrl Pts',(5.73685617975238,4.32853878647124,11.9920784594305));
#46971=CARTESIAN_POINT('Ctrl Pts',(5.73622837166435,4.15093758284581,11.5673091914781));
#46972=CARTESIAN_POINT('Ctrl Pts',(5.73548194665821,4.00213608247109,11.1310612655917));
#46973=CARTESIAN_POINT('Ctrl Pts',(5.73461683945432,3.88305444394366,10.6872940893152));
#46974=CARTESIAN_POINT('Ctrl Pts',(5.73452245510481,3.87006247839285,10.6388784986493));
#46975=CARTESIAN_POINT('Ctrl Pts',(5.73442665808298,3.85742426259303,10.5903733553511));
#46976=CARTESIAN_POINT('Ctrl Pts',(5.73432944831777,3.84514098508373,10.5417837646067));
#46977=CARTESIAN_POINT('Ctrl Pts',(5.73384873488381,3.78439876953865,10.3015026676433));
#46978=CARTESIAN_POINT('Ctrl Pts',(5.73333347371323,3.73233632290025,10.05915688844));
#46979=CARTESIAN_POINT('Ctrl Pts',(5.73278365815454,3.68907196536841,9.81543709253676));
#46980=CARTESIAN_POINT('Ctrl Pts',(5.99999999931447,3.99788407309719,9.3466078881625));
#46981=CARTESIAN_POINT('Ctrl Pts',(5.99999921905452,3.98578558819822,9.35665170909537));
#46982=CARTESIAN_POINT('Ctrl Pts',(5.99933245555486,3.97325817756116,9.36759536657576));
#46983=CARTESIAN_POINT('Ctrl Pts',(5.99783142449878,3.96039551133393,9.37944935506896));
#46984=CARTESIAN_POINT('Ctrl Pts',(5.99639504223158,3.94808683483931,9.39079279716379));
#46985=CARTESIAN_POINT('Ctrl Pts',(5.99419378268927,3.93547109215435,9.40296993155199));
#46986=CARTESIAN_POINT('Ctrl Pts',(5.99108408909626,3.92267709122614,9.41598364189161));
#46987=CARTESIAN_POINT('Ctrl Pts',(5.98929042384455,3.91529753622859,9.42348992485284));
#46988=CARTESIAN_POINT('Ctrl Pts',(5.98719466025372,3.90785956790051,9.43127440764121));
#46989=CARTESIAN_POINT('Ctrl Pts',(5.98477186618435,3.90039536693395,9.43933646513942));
#46990=CARTESIAN_POINT('Ctrl Pts',(5.98071484714981,3.88789640724855,9.4528365480154));
#46991=CARTESIAN_POINT('Ctrl Pts',(5.97573805800257,3.87531381301812,9.46710865485213));
#46992=CARTESIAN_POINT('Ctrl Pts',(5.96972968522987,3.86280213529356,9.48211836184687));
#46993=CARTESIAN_POINT('Ctrl Pts',(5.96758326184623,3.85833247958935,9.48748041032386));
#46994=CARTESIAN_POINT('Ctrl Pts',(5.96530538179708,3.85387229884052,9.49293650756601));
#46995=CARTESIAN_POINT('Ctrl Pts',(5.96289174885348,3.84943004700347,9.49848479322591));
#46996=CARTESIAN_POINT('Ctrl Pts',(5.95830675299446,3.84099143734185,9.50902445164523));
#46997=CARTESIAN_POINT('Ctrl Pts',(5.95323089635072,3.83261536357627,9.51989644938458));
#46998=CARTESIAN_POINT('Ctrl Pts',(5.94763509895936,3.82435832537359,9.53108169525198));
#46999=CARTESIAN_POINT('Ctrl Pts',(5.94483720026369,3.82022980627226,9.53667431818568));
#47000=CARTESIAN_POINT('Ctrl Pts',(5.94190933196359,3.81613107762387,9.54234524794495));
#47001=CARTESIAN_POINT('Ctrl Pts',(5.93884846234065,3.81207003683764,9.54809147636354));
#47002=CARTESIAN_POINT('Ctrl Pts',(5.93731802752919,3.81003951644452,9.55096459057283));
#47003=CARTESIAN_POINT('Ctrl Pts',(5.93575434414046,3.80801841801275,9.55385652942552));
#47004=CARTESIAN_POINT('Ctrl Pts',(5.93415706120959,3.80600775380745,9.55676689546259));
#47005=CARTESIAN_POINT('Ctrl Pts',(5.93309249680217,3.80466767716424,9.55870660948305));
#47006=CARTESIAN_POINT('Ctrl Pts',(5.93174397974193,3.80300201583821,9.56113909554917));
#47007=CARTESIAN_POINT('Ctrl Pts',(5.93064736237428,3.80167271211161,9.56309525086169));
#47008=CARTESIAN_POINT('Ctrl Pts',(5.93009860423359,3.80100751542319,9.5640741302629));
#47009=CARTESIAN_POINT('Ctrl Pts',(5.92961384298516,3.80042591251214,9.56493376387943));
#47010=CARTESIAN_POINT('Ctrl Pts',(5.92926407743291,3.80000808667201,9.56555286688789));
#47011=CARTESIAN_POINT('Ctrl Pts',(5.9237222231917,3.79338785237691,9.57536223379416));
#47012=CARTESIAN_POINT('Ctrl Pts',(5.91756027126521,3.78661920970786,9.58594208419168));
#47013=CARTESIAN_POINT('Ctrl Pts',(5.91064191769737,3.77975689027944,9.59724510500674));
#47014=CARTESIAN_POINT('Ctrl Pts',(5.90401867363957,3.77318729016703,9.60806598380606));
#47015=CARTESIAN_POINT('Ctrl Pts',(5.89670135644846,3.76653153860572,9.61954976307286));
#47016=CARTESIAN_POINT('Ctrl Pts',(5.88856867051108,3.75988379433895,9.63164686285785));
#47017=CARTESIAN_POINT('Ctrl Pts',(5.88075741804393,3.75349879322067,9.64326584104889));
#47018=CARTESIAN_POINT('Ctrl Pts',(5.87219301358668,3.74712115240292,9.65545068612455));
#47019=CARTESIAN_POINT('Ctrl Pts',(5.86277924073904,3.74088016718042,9.66814856503587));
#47020=CARTESIAN_POINT('Ctrl Pts',(5.8538529024773,3.73496233316379,9.68018896203755));
#47021=CARTESIAN_POINT('Ctrl Pts',(5.844162003248,3.72916776719875,9.69269062627937));
#47022=CARTESIAN_POINT('Ctrl Pts',(5.83364789820362,3.72364591984021,9.70559998642325));
#47023=CARTESIAN_POINT('Ctrl Pts',(5.82342631893895,3.71827770255262,9.71815017946487));
#47024=CARTESIAN_POINT('Ctrl Pts',(5.8124258371083,3.71316782542568,9.73108564878583));
#47025=CARTESIAN_POINT('Ctrl Pts',(5.80062802127563,3.70848480610254,9.74434929261022));
#47026=CARTESIAN_POINT('Ctrl Pts',(5.78926063509769,3.70397264131883,9.75712902774231));
#47027=CARTESIAN_POINT('Ctrl Pts',(5.77715249409862,3.69985766044913,9.77021329910403));
#47028=CARTESIAN_POINT('Ctrl Pts',(5.76433060935114,3.69630904301238,9.78354493083899));
#47029=CARTESIAN_POINT('Ctrl Pts',(5.75424393196645,3.69351742852269,9.79403261427793));
#47030=CARTESIAN_POINT('Ctrl Pts',(5.74371633829686,3.69107690256356,9.80467322214807));
#47031=CARTESIAN_POINT('Ctrl Pts',(5.73278365815454,3.68907196536841,9.81543709253676));
#47032=CARTESIAN_POINT('Ctrl Pts',(6.05076794927297,4.09458203878362,9.54441225412628));
#47033=CARTESIAN_POINT('Ctrl Pts',(6.05141961089931,4.06988665095652,9.55471205249664));
#47034=CARTESIAN_POINT('Ctrl Pts',(6.04716305939897,4.00788049666569,9.58295885528607));
#47035=CARTESIAN_POINT('Ctrl Pts',(6.01566649547382,3.90953592463721,9.63753455351153));
#47036=CARTESIAN_POINT('Ctrl Pts',(5.94752439895274,3.8106474887844,9.70652326956244));
#47037=CARTESIAN_POINT('Ctrl Pts',(5.84910136934098,3.73282443315672,9.77805722652396));
#47038=CARTESIAN_POINT('Ctrl Pts',(5.76414048183063,3.69951678478747,9.8252049164694));
#47039=CARTESIAN_POINT('Ctrl Pts',(5.71687785318494,3.68927674302881,9.84788773253446));
#47040=CARTESIAN_POINT('Ctrl Pts',(5.71192604303504,3.68828956961732,9.85022763652081));
#47041=CARTESIAN_POINT('Ctrl Pts',(5.91195109670203,3.98202506659494,9.28408186263919));
#47042=CARTESIAN_POINT('Ctrl Pts',(5.91254930560179,3.95979988492668,9.29334225786693));
#47043=CARTESIAN_POINT('Ctrl Pts',(5.9086455165599,3.9037959614243,9.3189084546854));
#47044=CARTESIAN_POINT('Ctrl Pts',(5.87945207765067,3.81435590889244,9.36894703351106));
#47045=CARTESIAN_POINT('Ctrl Pts',(5.81592785132783,3.724038797409,9.43278746526276));
#47046=CARTESIAN_POINT('Ctrl Pts',(5.72395388473843,3.65290980473349,9.4993131445599));
#47047=CARTESIAN_POINT('Ctrl Pts',(5.64456392614967,3.62258130620308,9.54323751898402));
#47048=CARTESIAN_POINT('Ctrl Pts',(5.6004601945523,3.61331530819896,9.56435979366266));
#47049=CARTESIAN_POINT('Ctrl Pts',(5.59584005632463,3.61242305635906,9.56653858267162));
#47050=CARTESIAN_POINT('Ctrl Pts',(6.02852321580189,3.87156862597752,9.01219535140232));
#47051=CARTESIAN_POINT('Ctrl Pts',(6.02946140921585,3.83732372353067,9.02648434185954));
#47052=CARTESIAN_POINT('Ctrl Pts',(6.02330612970468,3.7527205708333,9.0650283490567));
#47053=CARTESIAN_POINT('Ctrl Pts',(5.98006479999682,3.62281406661669,9.13695627061525));
#47054=CARTESIAN_POINT('Ctrl Pts',(5.88925135176173,3.49510413587073,9.22578449759683));
#47055=CARTESIAN_POINT('Ctrl Pts',(5.75973990848393,3.39553695641023,9.31721776716681));
#47056=CARTESIAN_POINT('Ctrl Pts',(5.64791312656201,3.35283377232076,9.37793571390397));
#47057=CARTESIAN_POINT('Ctrl Pts',(5.58525613648115,3.33967210674828,9.40750191109257));
#47058=CARTESIAN_POINT('Ctrl Pts',(5.57868611740273,3.33840311444834,9.41055623991342));
#47059=CARTESIAN_POINT('Ctrl Pts',(6.32407110292224,3.8356169056028,8.9069743206792));
#47060=CARTESIAN_POINT('Ctrl Pts',(6.32551985797543,3.78274129227489,8.92906365643331));
#47061=CARTESIAN_POINT('Ctrl Pts',(6.31598468883757,3.65368426869858,8.98773692499536));
#47062=CARTESIAN_POINT('Ctrl Pts',(6.25155285603629,3.46046613433746,9.09363216926371));
#47063=CARTESIAN_POINT('Ctrl Pts',(6.1194312004155,3.27391026506049,9.22120475071504));
#47064=CARTESIAN_POINT('Ctrl Pts',(5.93300158659274,3.12941390447521,9.35113453270944));
#47065=CARTESIAN_POINT('Ctrl Pts',(5.77199259259683,3.06709381628777,9.43765473932759));
#47066=CARTESIAN_POINT('Ctrl Pts',(5.68123186418643,3.04772038523933,9.48013432491254));
#47067=CARTESIAN_POINT('Ctrl Pts',(5.67170855993161,3.04584994414088,9.48452693128353));
#47068=CARTESIAN_POINT('',(5.72001553113216,3.07996593912288,9.45352621454216));
#47069=CARTESIAN_POINT('Origin',(5.89875807498483,3.22462412373647,9.89750210812564));
#47070=CARTESIAN_POINT('',(5.99999998860547,3.2142420421365,9.29218348100167));
#47071=CARTESIAN_POINT('Ctrl Pts',(6.00000005199697,3.21424211020075,9.29218367777145));
#47072=CARTESIAN_POINT('Ctrl Pts',(5.95914560526162,3.18372948881454,9.32022546602934));
#47073=CARTESIAN_POINT('Ctrl Pts',(5.91541907063108,3.15725519634921,9.34766265780539));
#47074=CARTESIAN_POINT('Ctrl Pts',(5.86878902309948,3.13479935800112,9.37455777546322));
#47075=CARTESIAN_POINT('Ctrl Pts',(5.82215897557027,3.11234351965418,9.40145289311967));
#47076=CARTESIAN_POINT('Ctrl Pts',(5.77262518198777,3.09390594889867,9.42780540507949));
#47077=CARTESIAN_POINT('Ctrl Pts',(5.72001606109867,3.0799663679684,9.45352753087965));
#47078=CARTESIAN_POINT('Ctrl Pts',(5.99998738510668,3.99788407452638,9.34660788723015));
#47079=CARTESIAN_POINT('Ctrl Pts',(5.99998486187692,3.97178788320407,9.33570712756464));
#47080=CARTESIAN_POINT('Ctrl Pts',(5.99998575125159,3.94579597545338,9.32564379782521));
#47081=CARTESIAN_POINT('Ctrl Pts',(5.9999822017208,3.91991001575388,9.31645115807804));
#47082=CARTESIAN_POINT('Ctrl Pts',(5.9999810788976,3.91172150915836,9.31354325000456));
#47083=CARTESIAN_POINT('Ctrl Pts',(5.99997928834179,3.90354373511738,9.31072213040201));
#47084=CARTESIAN_POINT('Ctrl Pts',(5.99997621692483,3.89537702176094,9.30798798286405));
#47085=CARTESIAN_POINT('Ctrl Pts',(5.99996211490638,3.85788060115839,9.29543449389021));
#47086=CARTESIAN_POINT('Ctrl Pts',(5.99992503046496,3.82061959459092,9.28471765012796));
#47087=CARTESIAN_POINT('Ctrl Pts',(5.99991423108138,3.78357227620041,9.27578205250742));
#47088=CARTESIAN_POINT('Ctrl Pts',(5.99990487784501,3.75148597024292,9.26804302221802));
#47089=CARTESIAN_POINT('Ctrl Pts',(5.99990278201534,3.71956006053042,9.26166526912885));
#47090=CARTESIAN_POINT('Ctrl Pts',(5.99990421744023,3.68780888196962,9.25664785673608));
#47091=CARTESIAN_POINT('Ctrl Pts',(5.99990515161368,3.66714523844375,9.25338252846148));
#47092=CARTESIAN_POINT('Ctrl Pts',(5.9999079344194,3.64655501788334,9.25069311330917));
#47093=CARTESIAN_POINT('Ctrl Pts',(5.9999154152975,3.62603165865102,9.24858460933612));
#47094=CARTESIAN_POINT('Ctrl Pts',(5.99991831505916,3.6180763291548,9.24776730434917));
#47095=CARTESIAN_POINT('Ctrl Pts',(5.99992637047819,3.60986152187724,9.24700704859185));
#47096=CARTESIAN_POINT('Ctrl Pts',(5.99993172018324,3.60175615292464,9.2463534189002));
#47097=CARTESIAN_POINT('Ctrl Pts',(5.99993713803719,3.59354753118767,9.24569146274173));
#47098=CARTESIAN_POINT('Ctrl Pts',(5.99993950798768,3.58545148438002,9.24513890584738));
#47099=CARTESIAN_POINT('Ctrl Pts',(5.99994451737532,3.57786718423949,9.24469687939468));
#47100=CARTESIAN_POINT('Ctrl Pts',(5.9999453511632,3.57660481486588,9.24462330627048));
#47101=CARTESIAN_POINT('Ctrl Pts',(5.99994629295721,3.57535665077325,9.24455268656537));
#47102=CARTESIAN_POINT('Ctrl Pts',(5.99994741064896,3.57412456268449,9.24448490010183));
#47103=CARTESIAN_POINT('Ctrl Pts',(5.99997420500839,3.54458778655221,9.24285985915166));
#47104=CARTESIAN_POINT('Ctrl Pts',(5.99996028565624,3.51545795299334,9.24253338015036));
#47105=CARTESIAN_POINT('Ctrl Pts',(5.99993572430989,3.48674258613422,9.2434249525757));
#47106=CARTESIAN_POINT('Ctrl Pts',(5.99991395264873,3.46128871938452,9.24421525993356));
#47107=CARTESIAN_POINT('Ctrl Pts',(5.99988491856864,3.43615941743387,9.24596289046136));
#47108=CARTESIAN_POINT('Ctrl Pts',(5.99986830472523,3.4113487813846,9.2486445826423));
#47109=CARTESIAN_POINT('Ctrl Pts',(5.99985059014699,3.38489433959829,9.25150394785762));
#47110=CARTESIAN_POINT('Ctrl Pts',(5.99984847396056,3.35880084002476,9.2554250847677));
#47111=CARTESIAN_POINT('Ctrl Pts',(5.99986814609541,3.33305940975811,9.26042190483073));
#47112=CARTESIAN_POINT('Ctrl Pts',(5.99988721410813,3.30810848685332,9.26526527487156));
#47113=CARTESIAN_POINT('Ctrl Pts',(5.99992732030962,3.28348762440651,9.2711201492481));
#47114=CARTESIAN_POINT('Ctrl Pts',(5.99996104571581,3.25920753570425,9.27802936166073));
#47115=CARTESIAN_POINT('Ctrl Pts',(5.99998205295688,3.24408369483654,9.28233304565181));
#47116=CARTESIAN_POINT('Ctrl Pts',(5.99999988351111,3.22909250348764,9.28704637806825));
#47117=CARTESIAN_POINT('Ctrl Pts',(5.99999988746152,3.2142419772354,9.29218329337644));
#47118=CARTESIAN_POINT('Ctrl Pts',(5.84420570955861,3.72282131685335,9.78165001835963));
#47119=CARTESIAN_POINT('Ctrl Pts',(5.38996562765094,3.59817429287799,10.0127664874412));
#47120=CARTESIAN_POINT('Ctrl Pts',(4.3608413144944,3.34562052197065,10.4582067183885));
#47121=CARTESIAN_POINT('Ctrl Pts',(2.69718314813897,3.05501779598387,10.9280508734159));
#47122=CARTESIAN_POINT('Ctrl Pts',(0.90123277416832,2.89428850134492,11.17270495048));
#47123=CARTESIAN_POINT('Ctrl Pts',(-0.898128982031577,2.8941485408364,11.1729135901656));
#47124=CARTESIAN_POINT('Ctrl Pts',(-2.69409800732445,3.05460699185379,10.9286891589027));
#47125=CARTESIAN_POINT('Ctrl Pts',(-4.35891886514342,3.3451779127716,10.4589598300149));
#47126=CARTESIAN_POINT('Ctrl Pts',(-5.38910342437971,3.59793551935265,10.0132112031376));
#47127=CARTESIAN_POINT('Ctrl Pts',(-5.84432165449578,3.72285318444294,9.78159102714844));
#47128=CARTESIAN_POINT('Ctrl Pts',(5.7253835366412,3.64453122286361,9.50229947997997));
#47129=CARTESIAN_POINT('Ctrl Pts',(5.28028699998817,3.52410865238856,9.72834256843305));
#47130=CARTESIAN_POINT('Ctrl Pts',(4.27190667605031,3.27990049730564,10.1641115674878));
#47131=CARTESIAN_POINT('Ctrl Pts',(2.64199881102779,2.99858776068898,10.6238561265337));
#47132=CARTESIAN_POINT('Ctrl Pts',(0.882754176675387,2.84291319818067,10.8632628192133));
#47133=CARTESIAN_POINT('Ctrl Pts',(-0.87971398644993,2.84277761987843,10.8634669836749));
#47134=CARTESIAN_POINT('Ctrl Pts',(-2.63897651280263,2.99818993802861,10.6244807187979));
#47135=CARTESIAN_POINT('Ctrl Pts',(-4.27002301198306,3.27947228142262,10.1648484281922));
#47136=CARTESIAN_POINT('Ctrl Pts',(-5.27944214962427,3.52387798467926,9.72877751971192));
#47137=CARTESIAN_POINT('Ctrl Pts',(-5.72549714712437,3.64456200849647,9.50224178643512));
#47138=CARTESIAN_POINT('Ctrl Pts',(5.71943787886701,3.37475784113534,9.34269929423411));
#47139=CARTESIAN_POINT('Ctrl Pts',(5.2756326248328,3.25566510720836,9.56644456769944));
#47140=CARTESIAN_POINT('Ctrl Pts',(4.26992144284517,3.01394111402995,9.99809686394945));
#47141=CARTESIAN_POINT('Ctrl Pts',(2.64237893294683,2.73488110526287,10.4543085477678));
#47142=CARTESIAN_POINT('Ctrl Pts',(0.88323656858176,2.58014446259695,10.6922727548935));
#47143=CARTESIAN_POINT('Ctrl Pts',(-0.880195053418905,2.58000959282474,
10.6924758250735));
#47144=CARTESIAN_POINT('Ctrl Pts',(-2.63935872061311,2.73448597878072,10.4549289906926));
#47145=CARTESIAN_POINT('Ctrl Pts',(-4.26804245262757,3.0135169461685,9.99882719418305));
#47146=CARTESIAN_POINT('Ctrl Pts',(-5.27479024948778,3.25543701995469,9.56687507681326));
#47147=CARTESIAN_POINT('Ctrl Pts',(-5.71955116480935,3.37478829409326,9.34264218643082));
#47148=CARTESIAN_POINT('Ctrl Pts',(5.83022605357272,3.08847457867854,9.40636717847527));
#47149=CARTESIAN_POINT('Ctrl Pts',(5.37902222649196,2.96695450753855,9.63208058929464));
#47150=CARTESIAN_POINT('Ctrl Pts',(4.35617397923863,2.72024194468582,10.0678408530508));
#47151=CARTESIAN_POINT('Ctrl Pts',(2.69807744090008,2.43493622270342,10.5293778616329));
#47152=CARTESIAN_POINT('Ctrl Pts',(0.902367232240108,2.27641231756555,10.7706401107682));
#47153=CARTESIAN_POINT('Ctrl Pts',(-0.899260324091646,2.27627402306329,
10.7708461773899));
#47154=CARTESIAN_POINT('Ctrl Pts',(-2.69499720433024,2.43453175827675,10.5300063904455));
#47155=CARTESIAN_POINT('Ctrl Pts',(-4.35426251968476,2.71980885391328,10.0685786090101));
#47156=CARTESIAN_POINT('Ctrl Pts',(-5.37816584285293,2.96672180164854,9.63251485973078));
#47157=CARTESIAN_POINT('Ctrl Pts',(-5.83034123540271,3.08850566402354,9.40630956456854));
#47158=CARTESIAN_POINT('',(-5.73278815913615,3.68906842472479,9.8154377369168));
#47159=CARTESIAN_POINT('',(-5.72001815309143,3.07996731954463,9.4535247212504));
#47160=CARTESIAN_POINT('Origin',(-5.89877627455651,3.22461269371084,9.89752154741546));
#47161=CARTESIAN_POINT('Ctrl Pts',(5.72001489176857,3.07996542174506,9.45352462645422));
#47162=CARTESIAN_POINT('Ctrl Pts',(5.48799480950505,3.01852056718121,9.56695266265951));
#47163=CARTESIAN_POINT('Ctrl Pts',(5.25105331740395,2.95922638303655,9.6737593363739));
#47164=CARTESIAN_POINT('Ctrl Pts',(5.0094050840325,2.90266822363824,9.77366018116699));
#47165=CARTESIAN_POINT('Ctrl Pts',(4.81759303552342,2.8577743038163,9.85295803251148));
#47166=CARTESIAN_POINT('Ctrl Pts',(4.62281550529396,2.81460478293779,9.92790410854663));
#47167=CARTESIAN_POINT('Ctrl Pts',(4.42518538965302,2.7734680793389,9.99833953918084));
#47168=CARTESIAN_POINT('Ctrl Pts',(4.40774373489348,2.76983759933948,10.0045557500047));
#47169=CARTESIAN_POINT('Ctrl Pts',(4.39027986594403,2.76622296211083,10.0107368187201));
#47170=CARTESIAN_POINT('Ctrl Pts',(4.37279389617178,2.76262438737662,10.0168826343622));
#47171=CARTESIAN_POINT('Ctrl Pts',(4.14017952315663,2.71475285285797,10.0986398986647));
#47172=CARTESIAN_POINT('Ctrl Pts',(3.90365739658418,2.66969955791451,10.1741666705095));
#47173=CARTESIAN_POINT('Ctrl Pts',(3.66348127988705,2.62785752322128,10.2432234915449));
#47174=CARTESIAN_POINT('Ctrl Pts',(3.54339322153849,2.60693650587466,10.2777519020626));
#47175=CARTESIAN_POINT('Ctrl Pts',(3.42239233379337,2.58681718649473,10.3106624654352));
#47176=CARTESIAN_POINT('Ctrl Pts',(3.3005145956988,2.56754188749553,10.3419232420058));
#47177=CARTESIAN_POINT('Ctrl Pts',(3.23957572665152,2.55790423799593,10.357553630291));
#47178=CARTESIAN_POINT('Ctrl Pts',(3.17841763997856,2.54847758767506,10.3727715469446));
#47179=CARTESIAN_POINT('Ctrl Pts',(3.11704519208393,2.53926669940264,10.3875729011152));
#47180=CARTESIAN_POINT('Ctrl Pts',(3.07988353782467,2.53368941094271,10.3965352747067));
#47181=CARTESIAN_POINT('Ctrl Pts',(3.04193898898731,2.52808742398809,10.4055108688518));
#47182=CARTESIAN_POINT('Ctrl Pts',(3.00449108092427,2.52265192508638,10.4141944648429));
#47183=CARTESIAN_POINT('Ctrl Pts',(2.98009379312151,2.51911070107907,10.4198518219962));
#47184=CARTESIAN_POINT('Ctrl Pts',(2.95590762246372,2.51563964095862,10.4253861653091));
#47185=CARTESIAN_POINT('Ctrl Pts',(2.93228963345293,2.51228602752607,10.4307231081398));
#47186=CARTESIAN_POINT('Ctrl Pts',(2.84332746939896,2.4996539313631,10.4508258350669));
#47187=CARTESIAN_POINT('Ctrl Pts',(2.7541295169341,2.48755127785995,10.4700011812909));
#47188=CARTESIAN_POINT('Ctrl Pts',(2.66471106197608,2.47599474546089,10.4882474435908));
#47189=CARTESIAN_POINT('Ctrl Pts',(2.40601906227546,2.44256112734122,10.5410347802055));
#47190=CARTESIAN_POINT('Ctrl Pts',(2.14548351135197,2.41369694976508,10.5860489111368));
#47191=CARTESIAN_POINT('Ctrl Pts',(1.8835937526012,2.38964917037043,10.6232802084062));
#47192=CARTESIAN_POINT('Ctrl Pts',(1.62209049315631,2.36563688090897,10.660456559386));
#47193=CARTESIAN_POINT('Ctrl Pts',(1.35923647871264,2.34642645776671,10.6898731463566));
#47194=CARTESIAN_POINT('Ctrl Pts',(1.09549640146985,2.33228549305395,10.7114791845455));
#47195=CARTESIAN_POINT('Ctrl Pts',(1.02640032222961,2.32858076516981,10.7171396535284));
#47196=CARTESIAN_POINT('Ctrl Pts',(0.95724333138418,2.32522411743047,10.7222638094589));
#47197=CARTESIAN_POINT('Ctrl Pts',(0.888033601990727,2.32222065282843,10.7268502548576));
#47198=CARTESIAN_POINT('Ctrl Pts',(0.625306294401089,2.31081918983688,10.744260877057));
#47199=CARTESIAN_POINT('Ctrl Pts',(0.361819606584868,2.30450503961765,10.7539262208446));
#47200=CARTESIAN_POINT('Ctrl Pts',(0.0980851516409874,2.30324908729893,
10.7558476291474));
#47201=CARTESIAN_POINT('Ctrl Pts',(0.0653985927216461,2.30309342785173,
10.7560857634697));
#47202=CARTESIAN_POINT('Ctrl Pts',(0.0327082200821129,2.30301550054985,
10.7562048927606));
#47203=CARTESIAN_POINT('Ctrl Pts',(1.50025002827934E-5,2.30301528050426,
10.7562049732159));
#47204=CARTESIAN_POINT('Ctrl Pts',(-0.260402583971723,2.30301352773274,
10.7562056140815));
#47205=CARTESIAN_POINT('Ctrl Pts',(-0.520628077614817,2.30794945072763,
10.7486542432409));
#47206=CARTESIAN_POINT('Ctrl Pts',(-0.780180801991693,2.31782837820034,
10.7335597513319));
#47207=CARTESIAN_POINT('Ctrl Pts',(-0.81512385878719,2.31915835816717,10.7315276105045));
#47208=CARTESIAN_POINT('Ctrl Pts',(-0.850054718196095,2.32057797102278,
10.7293586884452));
#47209=CARTESIAN_POINT('Ctrl Pts',(-0.884972201923496,2.3220872693386,10.7270529467002));
#47210=CARTESIAN_POINT('Ctrl Pts',(-1.08302033513938,2.33064784364132,10.7139750327288));
#47211=CARTESIAN_POINT('Ctrl Pts',(-1.2806384511707,2.34209289818217,10.6964967557869));
#47212=CARTESIAN_POINT('Ctrl Pts',(-1.47763989231892,2.3562977959534,10.674647479821));
#47213=CARTESIAN_POINT('Ctrl Pts',(-1.72250309886319,2.37395379276554,10.6474898928383));
#47214=CARTESIAN_POINT('Ctrl Pts',(-1.966400611854,2.3959245489063,10.6135703251249));
#47215=CARTESIAN_POINT('Ctrl Pts',(-2.20895642300066,2.4220042870364,10.5729124602434));
#47216=CARTESIAN_POINT('Ctrl Pts',(-2.33023432857398,2.43504415610144,10.5525835278027));
#47217=CARTESIAN_POINT('Ctrl Pts',(-2.45117699628968,2.44910990931528,10.530569817162));
#47218=CARTESIAN_POINT('Ctrl Pts',(-2.57173853619459,2.46416754251723,10.5068730018646));
#47219=CARTESIAN_POINT('Ctrl Pts',(-2.6017328859219,2.46791371162457,10.500977501807));
#47220=CARTESIAN_POINT('Ctrl Pts',(-2.63170369420663,2.47172120300045,10.4949778228535));
#47221=CARTESIAN_POINT('Ctrl Pts',(-2.66165016511053,2.47558955193389,10.4888739720703));
#47222=CARTESIAN_POINT('Ctrl Pts',(-2.6918882402914,2.4794955689818,10.4827106849347));
#47223=CARTESIAN_POINT('Ctrl Pts',(-2.7221015017876,2.48346363461805,10.4764411873324));
#47224=CARTESIAN_POINT('Ctrl Pts',(-2.75228934779513,2.48749300356865,10.4700655732347));
#47225=CARTESIAN_POINT('Ctrl Pts',(-2.78882912694254,2.4923702065172,10.4623484432678));
#47226=CARTESIAN_POINT('Ctrl Pts',(-2.82462118325018,2.49724024702851,10.4546297236668));
#47227=CARTESIAN_POINT('Ctrl Pts',(-2.86096121657739,2.5022776069016,10.446631522554));
#47228=CARTESIAN_POINT('Ctrl Pts',(-2.88437730122785,2.50552348298931,10.4414777971124));
#47229=CARTESIAN_POINT('Ctrl Pts',(-2.908020652911,2.50883932056307,10.4362071803145));
#47230=CARTESIAN_POINT('Ctrl Pts',(-2.93223485551304,2.51227720699284,10.4307356970442));
#47231=CARTESIAN_POINT('Ctrl Pts',(-3.18816992375771,2.54861438119102,10.3729041645668));
#47232=CARTESIAN_POINT('Ctrl Pts',(-3.44048848520818,2.58887347579288,10.3078290569615));
#47233=CARTESIAN_POINT('Ctrl Pts',(-3.68889603981782,2.63253044431277,10.2358289104327));
#47234=CARTESIAN_POINT('Ctrl Pts',(-3.93730359442746,2.67618741283266,10.1638287639039));
#47235=CARTESIAN_POINT('Ctrl Pts',(-4.18180036782967,2.72324271279475,10.0849034043995));
#47236=CARTESIAN_POINT('Ctrl Pts',(-4.42209432422583,2.77321168723325,9.99933375784427));
#47237=CARTESIAN_POINT('Ctrl Pts',(-4.67323483047252,2.8254361947711,9.90990161116226));
#47238=CARTESIAN_POINT('Ctrl Pts',(-4.91978515228066,2.88084356156688,9.81321196147461));
#47239=CARTESIAN_POINT('Ctrl Pts',(-5.16150816290815,2.93892462402289,9.70955603679204));
#47240=CARTESIAN_POINT('Ctrl Pts',(-5.35067345013844,2.98437714769289,9.62843797229831));
#47241=CARTESIAN_POINT('Ctrl Pts',(-5.53688233523973,3.03146792259273,9.54305277196725));
#47242=CARTESIAN_POINT('Ctrl Pts',(-5.72001751640012,3.07996680432955,9.4535231397943));
#47243=CARTESIAN_POINT('Ctrl Pts',(5.7327878508998,3.68906023344589,9.8154391656489));
#47244=CARTESIAN_POINT('Ctrl Pts',(5.30941801079182,3.57389352473303,10.0199549438219));
#47245=CARTESIAN_POINT('Ctrl Pts',(4.87321266289563,3.46710832616739,10.2012597279903));
#47246=CARTESIAN_POINT('Ctrl Pts',(4.42676988928123,3.37162421611693,10.3585398299166));
#47247=CARTESIAN_POINT('Ctrl Pts',(3.97538576906854,3.27508326270317,10.5175607495749));
#47248=CARTESIAN_POINT('Ctrl Pts',(3.51353578308825,3.19009467841088,10.6520220699274));
#47249=CARTESIAN_POINT('Ctrl Pts',(3.04423925012539,3.11963046164668,10.7611848420038));
#47250=CARTESIAN_POINT('Ctrl Pts',(3.01496106880174,3.11523438375063,10.7679952213911));
#47251=CARTESIAN_POINT('Ctrl Pts',(2.98565389961434,3.11089484111177,10.7747071184131));
#47252=CARTESIAN_POINT('Ctrl Pts',(2.95631847406784,3.10661255698121,10.7813203473808));
#47253=CARTESIAN_POINT('Ctrl Pts',(2.85795171409622,3.09225331700585,10.8034956488935));
#47254=CARTESIAN_POINT('Ctrl Pts',(2.75926725078899,3.07853787660286,10.8245615546286));
#47255=CARTESIAN_POINT('Ctrl Pts',(2.66029265310875,3.06549352193883,10.8445110040261));
#47256=CARTESIAN_POINT('Ctrl Pts',(2.18170270998425,3.00241777216995,10.9409762191043));
#47257=CARTESIAN_POINT('Ctrl Pts',(1.69632932885789,2.95503173038643,11.0113404250582));
#47258=CARTESIAN_POINT('Ctrl Pts',(1.2078115150959,2.9253399419601,11.0551347613053));
#47259=CARTESIAN_POINT('Ctrl Pts',(1.10052561963786,2.91881917645405,11.0647526594615));
#47260=CARTESIAN_POINT('Ctrl Pts',(0.993088047838054,2.91315189485321,11.0730888880343));
#47261=CARTESIAN_POINT('Ctrl Pts',(0.885537321098461,2.90835946256806,11.080138173233));
#47262=CARTESIAN_POINT('Ctrl Pts',(0.395429725259918,2.88652039614146,11.1122616960193));
#47263=CARTESIAN_POINT('Ctrl Pts',(-0.0970276312894777,2.88284672761108,
11.1176640421829));
#47264=CARTESIAN_POINT('Ctrl Pts',(-0.587926624973332,2.89733815422664,
11.096349233134));
#47265=CARTESIAN_POINT('Ctrl Pts',(-0.686185169594239,2.90023876414242,
11.0920828521819));
#47266=CARTESIAN_POINT('Ctrl Pts',(-0.784381279689713,2.90386721875651,
11.0867459208781));
#47267=CARTESIAN_POINT('Ctrl Pts',(-0.882483612659545,2.90822362826941,
11.0803382472665));
#47268=CARTESIAN_POINT('Ctrl Pts',(-1.37227578455157,2.92997372546261,11.0483468737689));
#47269=CARTESIAN_POINT('Ctrl Pts',(-1.85973068428807,2.96986769642306,10.989669217233));
#47270=CARTESIAN_POINT('Ctrl Pts',(-2.34120806414937,3.02589889861017,10.9047837983762));
#47271=CARTESIAN_POINT('Ctrl Pts',(-2.44684847556357,3.03819264178203,10.8861591839162));
#47272=CARTESIAN_POINT('Ctrl Pts',(-2.55220111103462,3.05126331203751,10.8662727383614));
#47273=CARTESIAN_POINT('Ctrl Pts',(-2.65722748483552,3.06508983926093,10.845129205313));
#47274=CARTESIAN_POINT('Ctrl Pts',(-2.75721742290147,3.07825332906549,10.8249995894508));
#47275=CARTESIAN_POINT('Ctrl Pts',(-2.85691164015495,3.09210192194813,10.8037305593992));
#47276=CARTESIAN_POINT('Ctrl Pts',(-2.9562817073028,3.10660749829929,10.7813293867526));
#47277=CARTESIAN_POINT('Ctrl Pts',(-3.42652729613442,3.17525174387923,10.6753210793812));
#47278=CARTESIAN_POINT('Ctrl Pts',(-3.88951476256729,3.25860776287227,10.5439630996004));
#47279=CARTESIAN_POINT('Ctrl Pts',(-4.3422241853442,3.35370329731909,10.3879967801771));
#47280=CARTESIAN_POINT('Ctrl Pts',(-4.36944131534789,3.35942049116041,10.3786200025392));
#47281=CARTESIAN_POINT('Ctrl Pts',(-4.39662129094512,3.36518012041666,10.3691542639388));
#47282=CARTESIAN_POINT('Ctrl Pts',(-4.42376345396193,3.37098154034238,10.3595997198319));
#47283=CARTESIAN_POINT('Ctrl Pts',(-4.8712542026576,3.46662910330382,10.2020746879022));
#47284=CARTESIAN_POINT('Ctrl Pts',(-5.30846866553962,3.57363557563167,10.0204148208704));
#47285=CARTESIAN_POINT('Ctrl Pts',(-5.73279070742533,3.68906129430703,9.81543899687841));
#47286=CARTESIAN_POINT('Ctrl Pts',(-5.843530256068,9.74782190829776,17.4349067435944));
#47287=CARTESIAN_POINT('Ctrl Pts',(-3.895686837379,8.92798468161957,17.8601636720695));
#47288=CARTESIAN_POINT('Ctrl Pts',(0.0001633689302756,8.10806558103108,
18.285510362917));
#47289=CARTESIAN_POINT('Ctrl Pts',(3.896013575239,8.92805344962997,17.8601279975215));
#47290=CARTESIAN_POINT('Ctrl Pts',(5.844020362859,9.74802820036948,17.434799738045));
#47291=CARTESIAN_POINT('Ctrl Pts',(-5.843530256068,8.93341759983096,17.0810053948035));
#47292=CARTESIAN_POINT('Ctrl Pts',(-3.895686837379,8.18554671757756,17.4915920160191));
#47293=CARTESIAN_POINT('Ctrl Pts',(0.0001633689302756,7.43613494371508,
17.9044826735906));
#47294=CARTESIAN_POINT('Ctrl Pts',(3.896013575239,8.18560957201543,17.4915573861792));
#47295=CARTESIAN_POINT('Ctrl Pts',(5.844020362859,8.93360578330469,17.0809020807058));
#47296=CARTESIAN_POINT('Ctrl Pts',(-5.843530256068,7.38850508713007,16.1560629905898));
#47297=CARTESIAN_POINT('Ctrl Pts',(-3.895686837379,6.77499149589132,16.5818456722199));
#47298=CARTESIAN_POINT('Ctrl Pts',(0.0001633689302756,6.16225640317841,
17.0065480575296));
#47299=CARTESIAN_POINT('Ctrl Pts',(3.896013575239,6.77504288702132,16.5818100517117));
#47300=CARTESIAN_POINT('Ctrl Pts',(5.844020362859,7.38865946288593,16.1559558527372));
#47301=CARTESIAN_POINT('Ctrl Pts',(-5.843530256068,5.5035950496088,14.2139340091217));
#47302=CARTESIAN_POINT('Ctrl Pts',(-3.895686837379,5.02273055192306,14.7660279927807));
#47303=CARTESIAN_POINT('Ctrl Pts',(0.0001633689302756,4.54131578037147,
15.3185227509534));
#47304=CARTESIAN_POINT('Ctrl Pts',(3.896013575239,5.02277092898996,14.7659816541094));
#47305=CARTESIAN_POINT('Ctrl Pts',(5.844020362859,5.50371604744243,14.2137950881263));
#47306=CARTESIAN_POINT('Ctrl Pts',(-5.843530256068,4.23580635710636,11.9384138467925));
#47307=CARTESIAN_POINT('Ctrl Pts',(-3.895686837379,3.77920659141981,12.6803367266932));
#47308=CARTESIAN_POINT('Ctrl Pts',(0.0001633689302756,3.32382395062254,
13.4219156363165));
#47309=CARTESIAN_POINT('Ctrl Pts',(3.896013575239,3.77924478513343,12.6802745292127));
#47310=CARTESIAN_POINT('Ctrl Pts',(5.844020362859,4.23592124932683,11.9382271599712));
#47311=CARTESIAN_POINT('Ctrl Pts',(-5.843530256068,3.79656748423947,10.3003457878546));
#47312=CARTESIAN_POINT('Ctrl Pts',(-3.895686837379,3.28180496518032,11.180104908631));
#47313=CARTESIAN_POINT('Ctrl Pts',(0.0001633689302756,2.76478687832676,
12.0604698112373));
#47314=CARTESIAN_POINT('Ctrl Pts',(3.896013575239,3.28184832836377,11.1800310709341));
#47315=CARTESIAN_POINT('Ctrl Pts',(5.844020362859,3.79669701166332,10.3001244179095));
#47316=CARTESIAN_POINT('Ctrl Pts',(-5.843530256068,3.68097897297366,9.52158538067259));
#47317=CARTESIAN_POINT('Ctrl Pts',(-3.895686837379,3.1209714929087,10.4634399073288));
#47318=CARTESIAN_POINT('Ctrl Pts',(0.0001633689302756,2.56014667279914,
11.4055373579833));
#47319=CARTESIAN_POINT('Ctrl Pts',(3.896013575239,3.12101853023684,10.4633608920186));
#47320=CARTESIAN_POINT('Ctrl Pts',(5.844020362859,3.68111988520519,9.52134838592816));
#47321=CARTESIAN_POINT('',(-5.73644346265606,9.52121765609472,17.3763289909641));
#47322=CARTESIAN_POINT('Ctrl Pts',(-5.7364438776242,9.52121721553873,17.3763301032173));
#47323=CARTESIAN_POINT('Ctrl Pts',(-5.68283410133726,9.49933861028788,17.3876652899307));
#47324=CARTESIAN_POINT('Ctrl Pts',(-5.62362602122325,9.47550628802813,17.4000397186838));
#47325=CARTESIAN_POINT('Ctrl Pts',(-5.55871833523674,9.44988973305887,17.413361706295));
#47326=CARTESIAN_POINT('Ctrl Pts',(-5.49483785882197,9.42467857800582,17.4264728641257));
#47327=CARTESIAN_POINT('Ctrl Pts',(-5.42543674955886,9.39773917888359,17.4405018460537));
#47328=CARTESIAN_POINT('Ctrl Pts',(-5.35041843921672,9.36927739071634,17.4553379787743));
#47329=CARTESIAN_POINT('Ctrl Pts',(-5.28279634620865,9.34362171175151,17.4687113851085));
#47330=CARTESIAN_POINT('Ctrl Pts',(-5.21061007458706,9.31672951463994,17.4827403793437));
#47331=CARTESIAN_POINT('Ctrl Pts',(-5.13378889523013,9.28878373746725,17.497327002931));
#47332=CARTESIAN_POINT('Ctrl Pts',(-5.05114656189602,9.25872035843925,17.5130189334483));
#47333=CARTESIAN_POINT('Ctrl Pts',(-4.96313255951284,9.22743587270336,17.529358901209));
#47334=CARTESIAN_POINT('Ctrl Pts',(-4.86963668391357,9.19519757921132,17.5462092461735));
#47335=CARTESIAN_POINT('Ctrl Pts',(-4.82248599479802,9.17893955986752,17.5547070047305));
#47336=CARTESIAN_POINT('Ctrl Pts',(-4.77394112144133,9.16243967649653,17.5633341890093));
#47337=CARTESIAN_POINT('Ctrl Pts',(-4.72398792920224,9.14573668509423,17.5720707845653));
#47338=CARTESIAN_POINT('Ctrl Pts',(-4.64948483055452,9.12082487144674,17.585101051729));
#47339=CARTESIAN_POINT('Ctrl Pts',(-4.57184842120784,9.09546050181848,17.5983752821524));
#47340=CARTESIAN_POINT('Ctrl Pts',(-4.49102962369258,9.06978519776136,17.6118209922886));
#47341=CARTESIAN_POINT('Ctrl Pts',(-4.45062022493494,9.05694754573281,17.6185438473567));
#47342=CARTESIAN_POINT('Ctrl Pts',(-4.40941525324104,9.04403240896086,17.6253094358827));
#47343=CARTESIAN_POINT('Ctrl Pts',(-4.36740858903266,9.03105903615374,17.6321079195241));
#47344=CARTESIAN_POINT('Ctrl Pts',(-4.34640525692848,9.02457234975017,17.6355071613449));
#47345=CARTESIAN_POINT('Ctrl Pts',(-4.32520149790406,9.0180711103512,17.6389146148433));
#47346=CARTESIAN_POINT('Ctrl Pts',(-4.3037965478717,9.01155783669579,17.6423290072939));
#47347=CARTESIAN_POINT('Ctrl Pts',(-4.29309407285551,9.00830119986808,17.6440362035192));
#47348=CARTESIAN_POINT('Ctrl Pts',(-4.2823412998427,9.00504155485615,17.645745133715));
#47349=CARTESIAN_POINT('Ctrl Pts',(-4.27153813267531,9.00177922108494,17.6474556350356));
#47350=CARTESIAN_POINT('Ctrl Pts',(-4.26343575729977,8.99933247075653,17.648738511026));
#47351=CARTESIAN_POINT('Ctrl Pts',(-4.25530503519258,8.99688420803268,17.6500222707106));
#47352=CARTESIAN_POINT('Ctrl Pts',(-4.24714592572875,8.99443456916128,17.6513068446019));
#47353=CARTESIAN_POINT('Ctrl Pts',(-4.24442622257414,8.99361802287081,17.6517350358991));
#47354=CARTESIAN_POINT('Ctrl Pts',(-4.24040661896544,8.99241275500541,17.6523670902657));
#47355=CARTESIAN_POINT('Ctrl Pts',(-4.23897735232055,8.99198447672772,17.652591687306));
#47356=CARTESIAN_POINT('Ctrl Pts',(-4.15849608766392,8.96786834868632,17.665238630342));
#47357=CARTESIAN_POINT('Ctrl Pts',(-4.07249650548149,8.94277842041226,17.6783932118544));
#47358=CARTESIAN_POINT('Ctrl Pts',(-3.98088600231545,8.91699602800316,17.6919117243921));
#47359=CARTESIAN_POINT('Ctrl Pts',(-3.89040600132535,8.89153179835609,17.7052634142697));
#47360=CARTESIAN_POINT('Ctrl Pts',(-3.79445270593128,8.86539204381246,17.7189701335298));
#47361=CARTESIAN_POINT('Ctrl Pts',(-3.69293689881025,8.83889286121126,17.7328696811413));
#47362=CARTESIAN_POINT('Ctrl Pts',(-3.66359282295988,8.83123302924741,17.7368874729607));
#47363=CARTESIAN_POINT('Ctrl Pts',(-3.63378397028016,8.8235434582015,17.7409212220854));
#47364=CARTESIAN_POINT('Ctrl Pts',(-3.60350818595862,8.81583250498245,17.744966629995));
#47365=CARTESIAN_POINT('Ctrl Pts',(-3.49990877451926,8.78944672396864,17.7588094382941));
#47366=CARTESIAN_POINT('Ctrl Pts',(-3.39084132813128,8.76280714218299,17.7727908127734));
#47367=CARTESIAN_POINT('Ctrl Pts',(-3.27622403179247,8.73628098812355,17.7867233140545));
#47368=CARTESIAN_POINT('Ctrl Pts',(-3.25749145032406,8.7319456621489,17.7890003849997));
#47369=CARTESIAN_POINT('Ctrl Pts',(-3.23861062517755,8.72761346586328,17.7912760977316));
#47370=CARTESIAN_POINT('Ctrl Pts',(-3.21958119918262,8.7232861203216,17.7935495717162));
#47371=CARTESIAN_POINT('Ctrl Pts',(-3.15184970057834,8.7078837850859,17.801641555156));
#47372=CARTESIAN_POINT('Ctrl Pts',(-3.08223598429778,8.69254251698729,17.8097053219785));
#47373=CARTESIAN_POINT('Ctrl Pts',(-3.01072583053028,8.67734391900242,17.8176992250224));
#47374=CARTESIAN_POINT('Ctrl Pts',(-2.96889170568906,8.66845259361696,17.8223757348645));
#47375=CARTESIAN_POINT('Ctrl Pts',(-2.92568006515535,8.65945929280977,17.8271077760883));
#47376=CARTESIAN_POINT('Ctrl Pts',(-2.88236683521321,8.6506496230998,17.8317452466546));
#47377=CARTESIAN_POINT('Ctrl Pts',(-2.85164156799341,8.64440027489098,17.8350349464198));
#47378=CARTESIAN_POINT('Ctrl Pts',(-2.82086517985766,8.63824239100087,17.8382775516242));
#47379=CARTESIAN_POINT('Ctrl Pts',(-2.79049313147201,8.63226377058535,17.8414269193232));
#47380=CARTESIAN_POINT('Ctrl Pts',(-2.49774374027982,8.5746371836463,17.8717829712043));
#47381=CARTESIAN_POINT('Ctrl Pts',(-2.21879412928721,8.52884151832713,17.8959619875009));
#47382=CARTESIAN_POINT('Ctrl Pts',(-1.95462250685991,8.49248912601094,17.9151940729285));
#47383=CARTESIAN_POINT('Ctrl Pts',(-1.73091164750199,8.46170449876731,17.9314805548706));
#47384=CARTESIAN_POINT('Ctrl Pts',(-1.51779862260439,8.43769072216954,17.9442201273955));
#47385=CARTESIAN_POINT('Ctrl Pts',(-1.3158774973236,8.41902980884336,17.9541436669417));
#47386=CARTESIAN_POINT('Ctrl Pts',(-1.27935766618023,8.41565476127117,17.9559384568037));
#47387=CARTESIAN_POINT('Ctrl Pts',(-1.24320393342112,8.41245493284762,17.9576410685465));
#47388=CARTESIAN_POINT('Ctrl Pts',(-1.20741981363967,8.40942211174052,17.9592557342648));
#47389=CARTESIAN_POINT('Ctrl Pts',(-1.05114003191732,8.39617688945994,17.9663074546243));
#47390=CARTESIAN_POINT('Ctrl Pts',(-0.901869672502831,8.38610981159634,
17.9716853664282));
#47391=CARTESIAN_POINT('Ctrl Pts',(-0.759755495368958,8.37855170967793,
17.9757326033567));
#47392=CARTESIAN_POINT('Ctrl Pts',(-0.689409738587004,8.37481048969545,
17.9777359639669));
#47393=CARTESIAN_POINT('Ctrl Pts',(-0.620817387436509,8.37168470694852,
17.9794129221181));
#47394=CARTESIAN_POINT('Ctrl Pts',(-0.553996241471728,8.36909742699286,
17.9808028777138));
#47395=CARTESIAN_POINT('Ctrl Pts',(-0.453088831378307,8.36519034465025,
17.9829018662492));
#47396=CARTESIAN_POINT('Ctrl Pts',(-0.356216007876087,8.36251015480873,
17.9843469301776));
#47397=CARTESIAN_POINT('Ctrl Pts',(-0.263414058300233,8.36080599351406,
17.9852672871028));
#47398=CARTESIAN_POINT('Ctrl Pts',(-0.217013083512306,8.35995391286673,
17.9857274655654));
#47399=CARTESIAN_POINT('Ctrl Pts',(-0.171629597781392,8.3593461703712,17.9860563598658));
#47400=CARTESIAN_POINT('Ctrl Pts',(-0.127266766540642,8.35895266383208,
17.9862689842807));
#47401=CARTESIAN_POINT('Ctrl Pts',(-0.105085350920267,8.35875591056252,
17.9863752964882));
#47402=CARTESIAN_POINT('Ctrl Pts',(-0.0831590989529071,8.35861272470365,
17.9864525259354));
#47403=CARTESIAN_POINT('Ctrl Pts',(-0.0614883185709054,8.358519476498,17.9865025015845));
#47404=CARTESIAN_POINT('Ctrl Pts',(-0.040712076886637,8.35843007744438,
17.9865504143105));
#47405=CARTESIAN_POINT('Ctrl Pts',(-0.0212663475724724,8.35838682250874,
17.9865732018906));
#47406=CARTESIAN_POINT('Ctrl Pts',(1.636912875435E-12,8.35838583196835,
17.9865726564898));
#47407=CARTESIAN_POINT('Ctrl Pts',(0.000915640623919675,8.3583857893198,
17.9865726330071));
#47408=CARTESIAN_POINT('Ctrl Pts',(0.00183465631929605,8.3583858335768,
17.98657256177));
#47409=CARTESIAN_POINT('Ctrl Pts',(0.00275729860215538,8.35838596679082,
17.9865724416797));
#47410=CARTESIAN_POINT('Ctrl Pts',(0.129186119377432,8.35840422098474,17.9865559858236));
#47411=CARTESIAN_POINT('Ctrl Pts',(0.262648467165869,8.36008917059176,17.9856368970372));
#47412=CARTESIAN_POINT('Ctrl Pts',(0.403015392074524,8.3640381883428,17.9835101130247));
#47413=CARTESIAN_POINT('Ctrl Pts',(0.546996654915845,8.36808889019544,17.9813285659963));
#47414=CARTESIAN_POINT('Ctrl Pts',(0.698242647626174,8.37452182263524,17.9778762910046));
#47415=CARTESIAN_POINT('Ctrl Pts',(0.856614200546237,8.3840309130267,17.9727981879443));
#47416=CARTESIAN_POINT('Ctrl Pts',(0.980582325233258,8.39147432114877,17.9688232132614));
#47417=CARTESIAN_POINT('Ctrl Pts',(1.10891645992642,8.40080359578708,17.963851511902));
#47418=CARTESIAN_POINT('Ctrl Pts',(1.24154985587638,8.41237122005545,17.9577024643033));
#47419=CARTESIAN_POINT('Ctrl Pts',(1.46301935575659,8.43168668689672,17.9474348655085));
#47420=CARTESIAN_POINT('Ctrl Pts',(1.69642619692483,8.45723519738743,17.933885327057));
#47421=CARTESIAN_POINT('Ctrl Pts',(1.9411391977435,8.49068447227641,17.916196228235));
#47422=CARTESIAN_POINT('Ctrl Pts',(1.95457768306835,8.49252134889604,17.9152248262493));
#47423=CARTESIAN_POINT('Ctrl Pts',(1.96805026425494,8.49438206284401,17.9142409349655));
#47424=CARTESIAN_POINT('Ctrl Pts',(1.98155683677488,8.49626689386396,17.9132444105436));
#47425=CARTESIAN_POINT('Ctrl Pts',(2.11128655275263,8.51437056839158,17.9036728608387));
#47426=CARTESIAN_POINT('Ctrl Pts',(2.2441485498313,8.53469810982091,17.8929357036826));
#47427=CARTESIAN_POINT('Ctrl Pts',(2.38002393604269,8.55749304688889,17.8809078074937));
#47428=CARTESIAN_POINT('Ctrl Pts',(2.44796162914838,8.56889051542288,17.8748938593993));
#47429=CARTESIAN_POINT('Ctrl Pts',(2.51665241842725,8.5809047741614,17.8685572531071));
#47430=CARTESIAN_POINT('Ctrl Pts',(2.58608015528761,8.59356557582336,17.86188244989));
#47431=CARTESIAN_POINT('Ctrl Pts',(2.6207940237178,8.59989597665434,17.8585450482815));
#47432=CARTESIAN_POINT('Ctrl Pts',(2.65569212925892,8.60638801177433,17.8551231000482));
#47433=CARTESIAN_POINT('Ctrl Pts',(2.69077230290425,8.61304536776699,17.8516147019052));
#47434=CARTESIAN_POINT('Ctrl Pts',(2.70831238972691,8.61637404576332,17.8498605028337));
#47435=CARTESIAN_POINT('Ctrl Pts',(2.72589799362908,8.61974405384018,17.848084691545));
#47436=CARTESIAN_POINT('Ctrl Pts',(2.74352883870858,8.6231558510227,17.846287032341));
#47437=CARTESIAN_POINT('Ctrl Pts',(2.75878964495409,8.62610901495311,17.8447310247484));
#47438=CARTESIAN_POINT('Ctrl Pts',(2.77549105180195,8.6293697107186,17.8430131339223));
#47439=CARTESIAN_POINT('Ctrl Pts',(2.78998005552623,8.63222120238673,17.8415109419287));
#47440=CARTESIAN_POINT('Ctrl Pts',(2.79223023162701,8.63266404569917,17.8412776480055));
#47441=CARTESIAN_POINT('Ctrl Pts',(2.79442704718602,8.63309692748931,17.8410496048427));
#47442=CARTESIAN_POINT('Ctrl Pts',(2.79655681911697,8.63351706784238,17.8408282768086));
#47443=CARTESIAN_POINT('Ctrl Pts',(3.06216252883609,8.68591313665962,17.813226265189));
#47444=CARTESIAN_POINT('Ctrl Pts',(3.32574192769713,8.74545004698172,17.7819422058441));
#47445=CARTESIAN_POINT('Ctrl Pts',(3.58705296384314,8.81170933478502,17.7471902317705));
#47446=CARTESIAN_POINT('Ctrl Pts',(3.85046129536175,8.87850042292769,17.7121593366245));
#47447=CARTESIAN_POINT('Ctrl Pts',(4.1115647060592,8.95212217125134,17.6736046824906));
#47448=CARTESIAN_POINT('Ctrl Pts',(4.37011526901556,9.03209869294817,17.6317706874632));
#47449=CARTESIAN_POINT('Ctrl Pts',(4.63268827870015,9.11331946371704,17.5892858525593));
#47450=CARTESIAN_POINT('Ctrl Pts',(4.89262838997619,9.20109425021854,17.5434188750952));
#47451=CARTESIAN_POINT('Ctrl Pts',(5.14967592346197,9.29487661277545,17.4944509967036));
#47452=CARTESIAN_POINT('Ctrl Pts',(5.3470087682887,9.36687240338649,17.4568588415987));
#47453=CARTESIAN_POINT('Ctrl Pts',(5.54263687795273,9.44240774729819,17.4174397040541));
#47454=CARTESIAN_POINT('Ctrl Pts',(5.73644276397646,9.52121697613148,17.3763304378294));
#47455=CARTESIAN_POINT('Ctrl Pts',(-5.73644356954166,9.52121823625822,17.3763277345534));
#47456=CARTESIAN_POINT('Ctrl Pts',(-5.73766037024742,8.76684683000269,17.0280907334631));
#47457=CARTESIAN_POINT('Ctrl Pts',(-5.73849618482897,8.0551635985718,16.5887330587425));
#47458=CARTESIAN_POINT('Ctrl Pts',(-5.73940756701334,6.75884967989494,15.5535369773042));
#47459=CARTESIAN_POINT('Ctrl Pts',(-5.73948313454875,6.1741609243319,14.9577815461622));
#47460=CARTESIAN_POINT('Ctrl Pts',(-5.73887402246562,5.16463991420442,13.6459927306558));
#47461=CARTESIAN_POINT('Ctrl Pts',(-5.73818934284707,4.74008688875323,12.9297575973714));
#47462=CARTESIAN_POINT('Ctrl Pts',(-5.73605973645603,4.07387565941445,11.4195453010467));
#47463=CARTESIAN_POINT('Ctrl Pts',(-5.73461480968354,3.83284551922558,10.6253394017529));
#47464=CARTESIAN_POINT('Ctrl Pts',(-5.732787930129,3.6890690658187,9.81543762359093));
#47465=CARTESIAN_POINT('Ctrl Pts',(-5.69266556774236,9.93047362171998,17.3532063511374));
#47466=CARTESIAN_POINT('Ctrl Pts',(-5.6579015041144,9.91591389121002,17.3608578763875));
#47467=CARTESIAN_POINT('Ctrl Pts',(-5.54372918028431,9.86855194591315,17.3857823389823));
#47468=CARTESIAN_POINT('Ctrl Pts',(-5.34117686668635,9.78714465878113,17.4287935841603));
#47469=CARTESIAN_POINT('Ctrl Pts',(-5.07577939191893,9.68537211231267,17.4827627766661));
#47470=CARTESIAN_POINT('Ctrl Pts',(-4.78282515662344,9.57897707244638,17.5393277358742));
#47471=CARTESIAN_POINT('Ctrl Pts',(-4.45930905771319,9.46872628426622,17.5980540214943));
#47472=CARTESIAN_POINT('Ctrl Pts',(-4.10061553946611,9.35538603621517,17.6585190484757));
#47473=CARTESIAN_POINT('Ctrl Pts',(-3.70134298965158,9.240249772823,17.7200282654163));
#47474=CARTESIAN_POINT('Ctrl Pts',(-3.25666212546635,9.12573356196013,17.7812939172411));
#47475=CARTESIAN_POINT('Ctrl Pts',(-2.76257283843288,9.01548172265967,17.8403746545893));
#47476=CARTESIAN_POINT('Ctrl Pts',(-2.21448293063478,8.91409697651722,17.8948143734171));
#47477=CARTESIAN_POINT('Ctrl Pts',(-1.60537183769643,8.82721888555496,17.9415936924642));
#47478=CARTESIAN_POINT('Ctrl Pts',(-0.938804294879647,8.76361682732247,
17.9759748015788));
#47479=CARTESIAN_POINT('Ctrl Pts',(-0.236508776851559,8.73273231277665,
17.9927966994848));
#47480=CARTESIAN_POINT('Ctrl Pts',(0.464364601057791,8.7390534224892,17.9893367439343));
#47481=CARTESIAN_POINT('Ctrl Pts',(1.12896559560388,8.77908287968296,17.9676008051861));
#47482=CARTESIAN_POINT('Ctrl Pts',(1.73422006975932,8.84413599471573,17.9324762362283));
#47483=CARTESIAN_POINT('Ctrl Pts',(2.27384587622857,8.92486790916139,17.8890293045475));
#47484=CARTESIAN_POINT('Ctrl Pts',(2.75210517025956,9.01417457107673,17.8410806225033));
#47485=CARTESIAN_POINT('Ctrl Pts',(3.17956446862062,9.10813528834538,17.790722121323));
#47486=CARTESIAN_POINT('Ctrl Pts',(3.56234892002592,9.2036241030006,17.7396175800791));
#47487=CARTESIAN_POINT('Ctrl Pts',(3.90388903432242,9.29788224441845,17.6892335714503));
#47488=CARTESIAN_POINT('Ctrl Pts',(4.20698277150655,9.38866585517398,17.6407615423958));
#47489=CARTESIAN_POINT('Ctrl Pts',(4.47552350916443,9.47468692044263,17.5948833416307));
#47490=CARTESIAN_POINT('Ctrl Pts',(4.71437364865999,9.55559720416526,17.5517812500452));
#47491=CARTESIAN_POINT('Ctrl Pts',(4.92834373472514,9.63159157290231,17.5113505406579));
#47492=CARTESIAN_POINT('Ctrl Pts',(5.12117579191109,9.70292314754304,17.473458081615));
#47493=CARTESIAN_POINT('Ctrl Pts',(5.29544459285597,9.7697118950186,17.4380436592871));
#47494=CARTESIAN_POINT('Ctrl Pts',(5.45302136069345,9.83200747379042,17.4050853286124));
#47495=CARTESIAN_POINT('Ctrl Pts',(5.58355472894296,9.88505281103088,17.3770970955391));
#47496=CARTESIAN_POINT('Ctrl Pts',(5.66171727448349,9.91751314502851,17.3600175469933));
#47497=CARTESIAN_POINT('Ctrl Pts',(5.69263920831806,9.93046917053698,17.3532089777586));
#47498=CARTESIAN_POINT('Ctrl Pts',(-5.75649916779056,9.81444719502755,17.4266144013715));
#47499=CARTESIAN_POINT('Ctrl Pts',(-5.7214030273039,9.79970756314098,17.4342702770646));
#47500=CARTESIAN_POINT('Ctrl Pts',(-5.60614021198355,9.751757100279,17.4592032236821));
#47501=CARTESIAN_POINT('Ctrl Pts',(-5.40164894963342,9.66931649258382,17.5021948859192));
#47502=CARTESIAN_POINT('Ctrl Pts',(-5.13368112666671,9.5661995361647,17.5560703775035));
#47503=CARTESIAN_POINT('Ctrl Pts',(-4.83783506996195,9.45834443418207,17.612479415478));
#47504=CARTESIAN_POINT('Ctrl Pts',(-4.51104954847754,9.34652609944795,17.6709960258764));
#47505=CARTESIAN_POINT('Ctrl Pts',(-4.14863414602988,9.23151944235374,17.7312040879216));
#47506=CARTESIAN_POINT('Ctrl Pts',(-3.7450998233873,9.11463384419983,17.7924131442713));
#47507=CARTESIAN_POINT('Ctrl Pts',(-3.29553136104131,8.99831906675384,17.8533393247946));
#47508=CARTESIAN_POINT('Ctrl Pts',(-2.79585032997637,8.88627539459825,17.9120464571609));
#47509=CARTESIAN_POINT('Ctrl Pts',(-2.2413830036986,8.78318279794773,17.9660866201541));
#47510=CARTESIAN_POINT('Ctrl Pts',(-1.62500802087657,8.69478332220193,18.0124555046676));
#47511=CARTESIAN_POINT('Ctrl Pts',(-0.950336100124751,8.63001825070586,
18.046463119548));
#47512=CARTESIAN_POINT('Ctrl Pts',(-0.239411452652046,8.59853301614872,
18.0630351699963));
#47513=CARTESIAN_POINT('Ctrl Pts',(0.470068367886107,8.60498147064549,18.0596354408429));
#47514=CARTESIAN_POINT('Ctrl Pts',(1.14282032180368,8.64577151992081,18.0381873663481));
#47515=CARTESIAN_POINT('Ctrl Pts',(1.75540154176908,8.71200012569824,18.0034225013884));
#47516=CARTESIAN_POINT('Ctrl Pts',(2.30143868154968,8.79413603665911,17.9603447467543));
#47517=CARTESIAN_POINT('Ctrl Pts',(2.78525552176593,8.884943982301,17.9127452134487));
#47518=CARTESIAN_POINT('Ctrl Pts',(3.21756459439386,8.98043601974661,17.8627089971835));
#47519=CARTESIAN_POINT('Ctrl Pts',(3.60458630020787,9.07743638428598,17.8118963803323));
#47520=CARTESIAN_POINT('Ctrl Pts',(3.94981603920815,9.17314581293368,17.761771322737));
#47521=CARTESIAN_POINT('Ctrl Pts',(4.25610869089316,9.26529062369714,17.7135235168905));
#47522=CARTESIAN_POINT('Ctrl Pts',(4.52742310264509,9.35256886962024,17.6678347552335));
#47523=CARTESIAN_POINT('Ctrl Pts',(4.76869242281635,9.43463232895327,17.6248884916112));
#47524=CARTESIAN_POINT('Ctrl Pts',(4.98479244422413,9.51168301727899,17.5845813156777));
#47525=CARTESIAN_POINT('Ctrl Pts',(5.17951571606055,9.58398125229581,17.5467807593111));
#47526=CARTESIAN_POINT('Ctrl Pts',(5.35547336783225,9.65165209884505,17.5114269323108));
#47527=CARTESIAN_POINT('Ctrl Pts',(5.51456429154051,9.714749875375,17.4784991695837));
#47528=CARTESIAN_POINT('Ctrl Pts',(5.64634618110254,9.76846300224162,17.4505149960062));
#47529=CARTESIAN_POINT('Ctrl Pts',(5.72525518795606,9.80132673659468,17.4334297817267));
#47530=CARTESIAN_POINT('Ctrl Pts',(5.75647210570228,9.81444369343647,17.4266190648295));
#47531=CARTESIAN_POINT('Ctrl Pts',(-5.8136196818267,9.67439307521046,17.423196759913));
#47532=CARTESIAN_POINT('Ctrl Pts',(-5.77819705101768,9.65952057934147,17.4308417919519));
#47533=CARTESIAN_POINT('Ctrl Pts',(-5.66186629691354,9.61113998799483,17.4557318756997));
#47534=CARTESIAN_POINT('Ctrl Pts',(-5.45549726793896,9.5279688855426,17.49860525688));
#47535=CARTESIAN_POINT('Ctrl Pts',(-5.18506580571852,9.42394225964876,17.5522463207665));
#47536=CARTESIAN_POINT('Ctrl Pts',(-4.8864742352847,9.31513196562998,17.60833774815));
#47537=CARTESIAN_POINT('Ctrl Pts',(-4.55661570512959,9.20231551898028,17.6664644876122));
#47538=CARTESIAN_POINT('Ctrl Pts',(-4.19074002650286,9.08627222891287,17.7262188124506));
#47539=CARTESIAN_POINT('Ctrl Pts',(-3.78329010947872,8.96832213491303,17.7869166097969));
#47540=CARTESIAN_POINT('Ctrl Pts',(-3.3292874134522,8.85093759828555,17.8472819386104));
#47541=CARTESIAN_POINT('Ctrl Pts',(-2.82459972125377,8.73785509947674,17.9053904110669));
#47542=CARTESIAN_POINT('Ctrl Pts',(-2.26449815904256,8.63380219603441,17.9588116307512));
#47543=CARTESIAN_POINT('Ctrl Pts',(-1.641790113482,8.54458023606658,18.0045692580133));
#47544=CARTESIAN_POINT('Ctrl Pts',(-0.960140287992341,8.47921865788041,
18.0380445444115));
#47545=CARTESIAN_POINT('Ctrl Pts',(-0.241865765967301,8.44745231309993,
18.0542799882141));
#47546=CARTESIAN_POINT('Ctrl Pts',(0.47489962410608,8.45395708095796,18.0509594735994));
#47547=CARTESIAN_POINT('Ctrl Pts',(1.15461838952617,8.49511618875115,18.0299067692742));
#47548=CARTESIAN_POINT('Ctrl Pts',(1.77352632071982,8.56195700003843,17.9956606052727));
#47549=CARTESIAN_POINT('Ctrl Pts',(2.32516508944598,8.64485754784285,17.9531364356432));
#47550=CARTESIAN_POINT('Ctrl Pts',(2.81389481841379,8.7365111091626,17.9060786654344));
#47551=CARTESIAN_POINT('Ctrl Pts',(3.25054101924557,8.8328888560205,17.856557408933));
#47552=CARTESIAN_POINT('Ctrl Pts',(3.64139477649633,8.93078312520244,17.8062236353288));
#47553=CARTESIAN_POINT('Ctrl Pts',(3.98999701973634,9.02736771692221,17.7565340796509));
#47554=CARTESIAN_POINT('Ctrl Pts',(4.29924266837349,9.12034820868826,17.70867337501));
#47555=CARTESIAN_POINT('Ctrl Pts',(4.57314066591343,9.20841173545414,17.6633218271144));
#47556=CARTESIAN_POINT('Ctrl Pts',(4.81668173982086,9.29120827097723,17.6206641928624));
#47557=CARTESIAN_POINT('Ctrl Pts',(5.03479661627034,9.36894315808525,17.5805992095702));
#47558=CARTESIAN_POINT('Ctrl Pts',(5.23132099554413,9.44188068092139,17.542995771987));
#47559=CARTESIAN_POINT('Ctrl Pts',(5.40889737384632,9.51014887211331,17.5077946817537));
#47560=CARTESIAN_POINT('Ctrl Pts',(5.56944911388493,9.57380459823179,17.4749769061113));
#47561=CARTESIAN_POINT('Ctrl Pts',(5.70244460066286,9.62799566795384,17.4470585904865));
#47562=CARTESIAN_POINT('Ctrl Pts',(5.78208503328795,9.66115432803744,17.4300028520173));
#47563=CARTESIAN_POINT('Ctrl Pts',(5.81359216861889,9.6743893639485,17.4232038071368));
#47564=CARTESIAN_POINT('Ctrl Pts',(-5.8478684852305,9.55010345183306,17.3442497677672));
#47565=CARTESIAN_POINT('Ctrl Pts',(-5.8122174502477,9.53518258073926,17.3518718998449));
#47566=CARTESIAN_POINT('Ctrl Pts',(-5.6951438548994,9.48665146739425,17.3766801397573));
#47567=CARTESIAN_POINT('Ctrl Pts',(-5.48749011694532,9.40325841727438,17.4193704823528));
#47568=CARTESIAN_POINT('Ctrl Pts',(-5.21539943495581,9.29901279673593,17.4727034262668));
#47569=CARTESIAN_POINT('Ctrl Pts',(-4.91498607989269,9.19002071642843,17.528406250694));
#47570=CARTESIAN_POINT('Ctrl Pts',(-4.58312097072923,9.07705601563583,17.586074177172));
#47571=CARTESIAN_POINT('Ctrl Pts',(-4.21502610849078,8.96089695073282,17.6453074158685));
#47572=CARTESIAN_POINT('Ctrl Pts',(-3.80511493093653,8.8428659429201,17.705428641255));
#47573=CARTESIAN_POINT('Ctrl Pts',(-3.34838603991078,8.72544050156519,17.765171621273));
#47574=CARTESIAN_POINT('Ctrl Pts',(-2.84069310071325,8.61236336019298,17.8226269922694));
#47575=CARTESIAN_POINT('Ctrl Pts',(-2.27729398891054,8.50836664329447,17.8753862184402));
#47576=CARTESIAN_POINT('Ctrl Pts',(-1.65097445000958,8.4192511995751,17.9205058456566));
#47577=CARTESIAN_POINT('Ctrl Pts',(-0.965445840894169,8.35402624679165,
17.95344150259));
#47578=CARTESIAN_POINT('Ctrl Pts',(-0.243178106984612,8.32237670105204,
17.9693493410763));
#47579=CARTESIAN_POINT('Ctrl Pts',(0.477492972615759,8.32885109541683,17.9661044996576));
#47580=CARTESIAN_POINT('Ctrl Pts',(1.16102514354678,8.36988481208941,17.9454421695092));
#47581=CARTESIAN_POINT('Ctrl Pts',(1.78347110439172,8.43660345553906,17.9117260313382));
#47582=CARTESIAN_POINT('Ctrl Pts',(2.33831781818648,8.51941531978428,17.8697821884199));
#47583=CARTESIAN_POINT('Ctrl Pts',(2.82992627541635,8.61102198917264,17.8233044445839));
#47584=CARTESIAN_POINT('Ctrl Pts',(3.26917005567782,8.70739159011194,17.7743440670996));
#47585=CARTESIAN_POINT('Ctrl Pts',(3.66236643292317,8.80531143237798,17.7245395595451));
#47586=CARTESIAN_POINT('Ctrl Pts',(4.01306968578505,8.90194951063851,17.6753378872775));
#47587=CARTESIAN_POINT('Ctrl Pts',(4.32418661918743,8.99500558484918,17.6279167669807));
#47588=CARTESIAN_POINT('Ctrl Pts',(4.59974676804594,9.08316196710642,17.5829540145801));
#47589=CARTESIAN_POINT('Ctrl Pts',(4.8447690100173,9.16606552695142,17.5406354503353));
#47590=CARTESIAN_POINT('Ctrl Pts',(5.06421316646418,9.2439201861955,17.500862178041));
#47591=CARTESIAN_POINT('Ctrl Pts',(5.26193851816834,9.31698985470052,17.4635047652742));
#47592=CARTESIAN_POINT('Ctrl Pts',(5.44060507020823,9.38540257085393,17.4285048762992));
#47593=CARTESIAN_POINT('Ctrl Pts',(5.60215053677798,9.44921492438462,17.3958449989642));
#47594=CARTESIAN_POINT('Ctrl Pts',(5.73598092677608,9.50355945699389,17.3680354126988));
#47595=CARTESIAN_POINT('Ctrl Pts',(5.81613053647907,9.53682145263586,17.3510357885404));
#47596=CARTESIAN_POINT('Ctrl Pts',(5.84784089921826,9.55009843600966,17.3442588686793));
#47597=CARTESIAN_POINT('',(-5.593361696257,9.87744143006053,17.3818877156668));
#47598=CARTESIAN_POINT('Ctrl Pts',(-5.593361696257,9.87744143006053,17.3818877156668));
#47599=CARTESIAN_POINT('Ctrl Pts',(-5.53989250492938,9.85546719473476,17.3934537221547));
#47600=CARTESIAN_POINT('Ctrl Pts',(-5.47940098467193,9.83101975551148,17.4063389204174));
#47601=CARTESIAN_POINT('Ctrl Pts',(-5.37813021089118,9.79076334881011,17.4276019464024));
#47602=CARTESIAN_POINT('Ctrl Pts',(-5.34261770406517,9.77675424696755,17.4350079149863));
#47603=CARTESIAN_POINT('Ctrl Pts',(-5.28671557047751,9.75493420233089,17.4465521226116));
#47604=CARTESIAN_POINT('Ctrl Pts',(-5.25810616034651,9.74382322934089,17.4524326696608));
#47605=CARTESIAN_POINT('Ctrl Pts',(-5.22850923520978,9.73243139520307,17.4584647215534));
#47606=CARTESIAN_POINT('Ctrl Pts',(-5.20855850400624,9.72477709790203,17.4625183010151));
#47607=CARTESIAN_POINT('Ctrl Pts',(-5.19652326399056,9.72017680466359,17.4649549275125));
#47608=CARTESIAN_POINT('Ctrl Pts',(-5.12232129828262,9.69189636800157,17.4799357695392));
#47609=CARTESIAN_POINT('Ctrl Pts',(-5.04967091216259,9.66472261805258,17.4943429868338));
#47610=CARTESIAN_POINT('Ctrl Pts',(-4.93065570807978,9.62125919422881,17.5174112254402));
#47611=CARTESIAN_POINT('Ctrl Pts',(-4.86863819981268,9.59885699467281,17.5293067125793));
#47612=CARTESIAN_POINT('Ctrl Pts',(-4.79189210427276,9.57167794713725,17.5437478377285));
#47613=CARTESIAN_POINT('Ctrl Pts',(-4.75242097252906,9.55784774956845,17.5510983793266));
#47614=CARTESIAN_POINT('Ctrl Pts',(-4.73526946950167,9.5518711876235,17.5542752647172));
#47615=CARTESIAN_POINT('Ctrl Pts',(-4.72378284443704,9.54787610858598,17.5563989725316));
#47616=CARTESIAN_POINT('Ctrl Pts',(-4.71687145441156,9.54547754923709,17.5576740663135));
#47617=CARTESIAN_POINT('Ctrl Pts',(-4.56330035732465,9.49226685040711,17.5859623330004));
#47618=CARTESIAN_POINT('Ctrl Pts',(-4.38742083376464,9.43392133780629,17.6170101124104));
#47619=CARTESIAN_POINT('Ctrl Pts',(-4.08315840430196,9.34023826849138,17.6669296812749));
#47620=CARTESIAN_POINT('Ctrl Pts',(-3.97499707046061,9.30801566536103,17.6841092574927));
#47621=CARTESIAN_POINT('Ctrl Pts',(-3.80264428366793,9.25895958677314,17.7102778110509));
#47622=CARTESIAN_POINT('Ctrl Pts',(-3.71394019376392,9.23425373108708,17.7234604296094));
#47623=CARTESIAN_POINT('Ctrl Pts',(-3.60602861998748,9.20531488374581,17.7389081362217));
#47624=CARTESIAN_POINT('Ctrl Pts',(-3.55096696587716,9.19084300277489,17.746634997581));
#47625=CARTESIAN_POINT('Ctrl Pts',(-3.527132142568,9.18464310672296,17.7499456364573));
#47626=CARTESIAN_POINT('Ctrl Pts',(-3.51118960001799,9.18051068563473,17.7521523639014));
#47627=CARTESIAN_POINT('Ctrl Pts',(-3.50199535539259,9.17813690347825,17.7534200272329));
#47628=CARTESIAN_POINT('Ctrl Pts',(-3.2766948368566,9.12014890156824,17.7843882334437));
#47629=CARTESIAN_POINT('Ctrl Pts',(-3.0302774314496,9.06193661034056,17.815508643134));
#47630=CARTESIAN_POINT('Ctrl Pts',(-2.61873506037185,8.97833393532695,17.8602667918085));
#47631=CARTESIAN_POINT('Ctrl Pts',(-2.47456822618473,8.95110744004314,17.8748540188011));
#47632=CARTESIAN_POINT('Ctrl Pts',(-2.24783890916224,8.91224181782533,17.8956959311803));
#47633=CARTESIAN_POINT('Ctrl Pts',(-2.17051595919777,8.89961674957794,17.9024694686771));
#47634=CARTESIAN_POINT('Ctrl Pts',(-2.0123770373549,8.87520800329911,17.915571987208));
#47635=CARTESIAN_POINT('Ctrl Pts',(-1.93359205714849,8.86370156201463,17.9217519816094));
#47636=CARTESIAN_POINT('Ctrl Pts',(-1.51062468461165,8.8059715377584,17.9527772412711));
#47637=CARTESIAN_POINT('Ctrl Pts',(-1.1559767799876,8.77006019485985,17.9721409225942));
#47638=CARTESIAN_POINT('Ctrl Pts',(-0.599593913159634,8.73782855337055,
17.9895832486352));
#47639=CARTESIAN_POINT('Ctrl Pts',(-0.410064455901665,8.73068661704158,
17.9934643165518));
#47640=CARTESIAN_POINT('Ctrl Pts',(-0.119667517541742,8.7260893818246,17.9959679935218));
#47641=CARTESIAN_POINT('Ctrl Pts',(-0.0218514126762748,8.72557544902211,
17.9962493029249));
#47642=CARTESIAN_POINT('Ctrl Pts',(0.126398432740171,8.72641563924098,17.9957913442492));
#47643=CARTESIAN_POINT('Ctrl Pts',(0.200904777477956,8.72723861905749,17.9953427384674));
#47644=CARTESIAN_POINT('Ctrl Pts',(0.275983255260081,8.72868170504874,17.9945570124753));
#47645=CARTESIAN_POINT('Ctrl Pts',(0.326162714458018,8.72978326875773,17.9939574444567));
#47646=CARTESIAN_POINT('Ctrl Pts',(0.353068789745851,8.73045184547564,17.9935936527374));
#47647=CARTESIAN_POINT('Ctrl Pts',(0.751958403468875,8.74138449395115,17.9876467348906));
#47648=CARTESIAN_POINT('Ctrl Pts',(1.10849134973418,8.76677112538586,17.9738993830128));
#47649=CARTESIAN_POINT('Ctrl Pts',(1.61495191033288,8.82094465101678,17.9447265285685));
#47650=CARTESIAN_POINT('Ctrl Pts',(1.86109747593242,8.8520477561408,17.9280012002593));
#47651=CARTESIAN_POINT('Ctrl Pts',(2.13586905174054,8.89390623756821,17.905531504999));
#47652=CARTESIAN_POINT('Ctrl Pts',(2.25097153050302,8.91288546000701,17.8953504939764));
#47653=CARTESIAN_POINT('Ctrl Pts',(2.32711612345302,8.92575243891898,17.8884497539916));
#47654=CARTESIAN_POINT('Ctrl Pts',(2.36665276247385,8.93260467126174,17.8847756054096));
#47655=CARTESIAN_POINT('Ctrl Pts',(2.68815404379909,8.98955276178681,17.85424606372));
#47656=CARTESIAN_POINT('Ctrl Pts',(2.94945525844658,9.04484068918616,17.8246561887078));
#47657=CARTESIAN_POINT('Ctrl Pts',(3.30469052728873,9.12823135723393,17.7800773475732));
#47658=CARTESIAN_POINT('Ctrl Pts',(3.41698285804794,9.15611908146275,17.7651777008726));
#47659=CARTESIAN_POINT('Ctrl Pts',(3.57624221590447,9.19741366093029,17.7431262720328));
#47660=CARTESIAN_POINT('Ctrl Pts',(3.65357711026217,9.21792832465172,17.7321741939344));
#47661=CARTESIAN_POINT('Ctrl Pts',(3.739785280681,9.24150050145565,17.7195943535128));
#47662=CARTESIAN_POINT('Ctrl Pts',(3.77587109521795,9.25151267978903,17.7142520545844));
#47663=CARTESIAN_POINT('Ctrl Pts',(3.79973707286171,9.2581660471466,17.7107021529559));
#47664=CARTESIAN_POINT('Ctrl Pts',(3.8098321625265,9.26099167213174,17.7091946138522));
#47665=CARTESIAN_POINT('Ctrl Pts',(4.03906084095668,9.32550557489382,17.6747771483891));
#47666=CARTESIAN_POINT('Ctrl Pts',(4.23305855283995,9.38535894097414,17.6428776600593));
#47667=CARTESIAN_POINT('Ctrl Pts',(4.49143473070597,9.46908457807708,17.5983018997288));
#47668=CARTESIAN_POINT('Ctrl Pts',(4.57212339166817,9.49600414147767,17.5839784369806));
#47669=CARTESIAN_POINT('Ctrl Pts',(4.68500128562173,9.53450066553663,17.5635072343031));
#47670=CARTESIAN_POINT('Ctrl Pts',(4.73940145822609,9.55328036811316,17.5535239435117));
#47671=CARTESIAN_POINT('Ctrl Pts',(4.79930047111274,9.57430584208441,17.5423515809152));
#47672=CARTESIAN_POINT('Ctrl Pts',(4.82420693624594,9.58312192570992,17.5376678794198));
#47673=CARTESIAN_POINT('Ctrl Pts',(4.84064134847036,9.58895546402193,17.5345689006767));
#47674=CARTESIAN_POINT('Ctrl Pts',(4.8471229973513,9.59126108436074,17.5333441340759));
#47675=CARTESIAN_POINT('Ctrl Pts',(4.93440424627371,9.62241797040445,17.5167945121165));
#47676=CARTESIAN_POINT('Ctrl Pts',(5.00681738695592,9.64894999419244,17.5027116938825));
#47677=CARTESIAN_POINT('Ctrl Pts',(5.10768181043932,9.68655270637007,17.4827706331314));
#47678=CARTESIAN_POINT('Ctrl Pts',(5.15617520029604,9.70480850706302,17.4730940902559));
#47679=CARTESIAN_POINT('Ctrl Pts',(5.20935788349684,9.72508928042515,17.4623520315752));
#47680=CARTESIAN_POINT('Ctrl Pts',(5.23142340380461,9.73355857970071,17.4578677257988));
#47681=CARTESIAN_POINT('Ctrl Pts',(5.24597218218603,9.739154921829,17.4549049317256));
#47682=CARTESIAN_POINT('Ctrl Pts',(5.25210470602221,9.74151819612761,17.4536539000924));
#47683=CARTESIAN_POINT('Ctrl Pts',(5.39106103678595,9.79520571035242,17.4252374298913));
#47684=CARTESIAN_POINT('Ctrl Pts',(5.5020887329495,9.83993097584024,17.4016311175229));
#47685=CARTESIAN_POINT('Ctrl Pts',(5.593361696325,9.87744142971438,17.3818877156863));
#47686=CARTESIAN_POINT('Origin',(-5.599999999997,9.6786310860259,17.0348569100619));
#47687=CARTESIAN_POINT('Origin',(-5.599999999997,9.6786310860259,17.0348569100619));
#47688=CARTESIAN_POINT('',(-5.99999997117386,9.67863337111575,17.0348538908756));
#47689=CARTESIAN_POINT('Origin',(-5.6,9.67863108604804,17.0348569101035));
#47690=CARTESIAN_POINT('Origin',(-5.59998164336875,9.67863961983816,17.0348438488187));
#47691=CARTESIAN_POINT('Ctrl Pts',(-5.72202473568975,9.61344955698967,17.4236870330605));
#47692=CARTESIAN_POINT('Ctrl Pts',(-5.72274567064853,9.1758914447973,17.227024855994));
#47693=CARTESIAN_POINT('Ctrl Pts',(-5.72404121715671,8.29086220798215,16.7525775913613));
#47694=CARTESIAN_POINT('Ctrl Pts',(-5.72530537911657,7.0637852157259,15.8436323328137));
#47695=CARTESIAN_POINT('Ctrl Pts',(-5.72546529150377,5.9593366094895,14.7303948942631));
#47696=CARTESIAN_POINT('Ctrl Pts',(-5.72471353061148,5.03570888986459,13.4633046841625));
#47697=CARTESIAN_POINT('Ctrl Pts',(-5.72306572655457,4.31359098850255,12.0712170637154));
#47698=CARTESIAN_POINT('Ctrl Pts',(-5.72038901589368,3.83840721059553,10.6678390325755));
#47699=CARTESIAN_POINT('Ctrl Pts',(-5.71829740700494,3.65952909703187,9.72608608981356));
#47700=CARTESIAN_POINT('Ctrl Pts',(-5.71724182049107,3.60559725899456,9.2948909596003));
#47701=CARTESIAN_POINT('Ctrl Pts',(-5.90002849745086,9.63679782292734,17.3716661896694));
#47702=CARTESIAN_POINT('Ctrl Pts',(-5.90064146364177,9.20180721910066,17.1757869809176));
#47703=CARTESIAN_POINT('Ctrl Pts',(-5.9017416993345,8.32198023867081,16.7034321811413));
#47704=CARTESIAN_POINT('Ctrl Pts',(-5.9028112502954,7.10225243166773,15.7991880815107));
#47705=CARTESIAN_POINT('Ctrl Pts',(-5.90294650836853,6.00412626997486,14.6922156321237));
#47706=CARTESIAN_POINT('Ctrl Pts',(-5.90231053688296,5.085487591936,13.4325712074677));
#47707=CARTESIAN_POINT('Ctrl Pts',(-5.90091484041538,4.36673081244574,12.0486614223905));
#47708=CARTESIAN_POINT('Ctrl Pts',(-5.89863714804845,3.89298856491527,10.6534828562829));
#47709=CARTESIAN_POINT('Ctrl Pts',(-5.89685281246244,3.71409999207949,9.71696536617335));
#47710=CARTESIAN_POINT('Ctrl Pts',(-5.89594634491586,3.65996428723496,9.28813332545949));
#47711=CARTESIAN_POINT('Ctrl Pts',(-6.00728099553466,9.69953390946991,17.2318878304503));
#47712=CARTESIAN_POINT('Ctrl Pts',(-6.00760395673598,9.27115450686099,17.0387535402842));
#47713=CARTESIAN_POINT('Ctrl Pts',(-6.00818201774359,8.40460392931769,16.5730884304966));
#47714=CARTESIAN_POINT('Ctrl Pts',(-6.00873883246761,7.20353730477516,15.6822211593903));
#47715=CARTESIAN_POINT('Ctrl Pts',(-6.00880920187504,6.12189909393815,14.5918025726931));
#47716=CARTESIAN_POINT('Ctrl Pts',(-6.00847818758616,5.21697168858999,13.3513274687463));
#47717=CARTESIAN_POINT('Ctrl Pts',(-6.00774958520186,4.50853451476516,11.9883501791246));
#47718=CARTESIAN_POINT('Ctrl Pts',(-6.00654715789313,4.04115926875987,10.6143701706271));
#47719=CARTESIAN_POINT('Ctrl Pts',(-6.00559944219796,3.86430275187011,9.69181559903544));
#47720=CARTESIAN_POINT('Ctrl Pts',(-6.00511045427861,3.81066035891786,9.26940225083461));
#47721=CARTESIAN_POINT('Ctrl Pts',(-5.99966790181819,9.77609467523413,17.0613075954953));
#47722=CARTESIAN_POINT('Ctrl Pts',(-5.99963699057152,9.35567597393494,16.8717624111685));
#47723=CARTESIAN_POINT('Ctrl Pts',(-5.99957878702131,8.50506541600627,16.414659546472));
#47724=CARTESIAN_POINT('Ctrl Pts',(-5.99951367676562,7.32636687298965,15.5403949299101));
#47725=CARTESIAN_POINT('Ctrl Pts',(-5.99950536491651,6.26466320051636,14.4700735480911));
#47726=CARTESIAN_POINT('Ctrl Pts',(-5.99954420752702,5.37658269142921,13.2526794263663));
#47727=CARTESIAN_POINT('Ctrl Pts',(-5.99962585271713,4.68122009686565,11.9148587494722));
#47728=CARTESIAN_POINT('Ctrl Pts',(-5.99973680126801,4.22254572368814,10.5664376666286));
#47729=CARTESIAN_POINT('Ctrl Pts',(-5.99981416583464,4.04893806171432,9.66088387769014));
#47730=CARTESIAN_POINT('Ctrl Pts',(-5.99984092598252,3.99628630515258,9.24632947018055));
#47731=CARTESIAN_POINT('',(-5.99999618081983,3.99788654355748,9.34661202484151));
#47732=CARTESIAN_POINT('Ctrl Pts',(-6.,9.67863396518287,17.0348526023092));
#47733=CARTESIAN_POINT('Ctrl Pts',(-6.,9.24640194836271,16.8355809089051));
#47734=CARTESIAN_POINT('Ctrl Pts',(-6.,8.83275508448163,16.6077872907197));
#47735=CARTESIAN_POINT('Ctrl Pts',(-6.,8.43516131847461,16.3499544364876));
#47736=CARTESIAN_POINT('Ctrl Pts',(-6.,8.03756727126096,16.0921213998978));
#47737=CARTESIAN_POINT('Ctrl Pts',(-6.,7.65602634462916,15.8042490847697));
#47738=CARTESIAN_POINT('Ctrl Pts',(-6.,7.29796322038041,15.4912222280303));
#47739=CARTESIAN_POINT('Ctrl Pts',(-6.,6.93990009613191,15.1781953712911));
#47740=CARTESIAN_POINT('Ctrl Pts',(-6.,6.60531477426643,14.8400139729407));
#47741=CARTESIAN_POINT('Ctrl Pts',(-6.,6.29607548230007,14.4788351240543));
#47742=CARTESIAN_POINT('Ctrl Pts',(-6.,5.98683619033349,14.1176562751676));
#47743=CARTESIAN_POINT('Ctrl Pts',(-6.,5.70294292826608,13.7334799757447));
#47744=CARTESIAN_POINT('Ctrl Pts',(-6.,5.44842667074869,13.3317962248934));
#47745=CARTESIAN_POINT('Ctrl Pts',(-6.,5.19391041323149,12.9301124740424));
#47746=CARTESIAN_POINT('Ctrl Pts',(-6.,4.96877116026427,12.5109212717628));
#47747=CARTESIAN_POINT('Ctrl Pts',(-6.,4.7746677150985,12.076828535284));
#47748=CARTESIAN_POINT('Ctrl Pts',(-6.,4.58056426993259,11.6427357988049));
#47749=CARTESIAN_POINT('Ctrl Pts',(-6.,4.41749663256818,11.1937415281265));
#47750=CARTESIAN_POINT('Ctrl Pts',(-6.,4.28772377553626,10.7378297754049));
#47751=CARTESIAN_POINT('Ctrl Pts',(-6.,4.15795091850444,10.2819180226836));
#47752=CARTESIAN_POINT('Ctrl Pts',(-6.,4.06147284180507,9.81908878791919));
#47753=CARTESIAN_POINT('Ctrl Pts',(-6.,3.99788654321422,9.34661202516592));
#47754=CARTESIAN_POINT('Ctrl Pts',(-5.73278606918832,3.68907427304369,9.81543670344895));
#47755=CARTESIAN_POINT('Ctrl Pts',(-5.74643892975411,3.69157874331479,9.80199766513387));
#47756=CARTESIAN_POINT('Ctrl Pts',(-5.75940527740446,3.69473932546515,9.78873354297374));
#47757=CARTESIAN_POINT('Ctrl Pts',(-5.7716485988922,3.69839100959473,9.77571635192827));
#47758=CARTESIAN_POINT('Ctrl Pts',(-5.78419257321745,3.70213236622016,9.76237950453559));
#47759=CARTESIAN_POINT('Ctrl Pts',(-5.79597832116455,3.70638821389214,9.74930201408252));
#47760=CARTESIAN_POINT('Ctrl Pts',(-5.80701828852253,3.71100259495989,9.73655425995103));
#47761=CARTESIAN_POINT('Ctrl Pts',(-5.8185606921694,3.71582697959233,9.72322634701382));
#47762=CARTESIAN_POINT('Ctrl Pts',(-5.82928881694117,3.72104247748579,9.71025896007629));
#47763=CARTESIAN_POINT('Ctrl Pts',(-5.83925970990793,3.72650871517201,9.6977229197899));
#47764=CARTESIAN_POINT('Ctrl Pts',(-5.84579318371984,3.73009049274115,9.68950862131239));
#47765=CARTESIAN_POINT('Ctrl Pts',(-5.85200237370557,3.73378078310869,9.68147931558694));
#47766=CARTESIAN_POINT('Ctrl Pts',(-5.85790960796569,3.73755009977863,9.67365268746806));
#47767=CARTESIAN_POINT('Ctrl Pts',(-5.86794796082459,3.74395542062822,9.66035264699343));
#47768=CARTESIAN_POINT('Ctrl Pts',(-5.87708910768384,3.75056572619156,9.64762920607599));
#47769=CARTESIAN_POINT('Ctrl Pts',(-5.88541230482037,3.75721385440797,9.63553178398123));
#47770=CARTESIAN_POINT('Ctrl Pts',(-5.89033927120756,3.76114925371699,9.62837064252864));
#47771=CARTESIAN_POINT('Ctrl Pts',(-5.89498027758906,3.76509875741602,9.62142867264591));
#47772=CARTESIAN_POINT('Ctrl Pts',(-5.89935566970285,3.76903508538686,9.61471458108651));
#47773=CARTESIAN_POINT('Ctrl Pts',(-5.90523907304197,3.77432809788155,9.60568642825533));
#47774=CARTESIAN_POINT('Ctrl Pts',(-5.91064087265227,3.779595289029,9.59706928178317));
#47775=CARTESIAN_POINT('Ctrl Pts',(-5.91560821859055,3.78477485647406,9.58887630999103));
#47776=CARTESIAN_POINT('Ctrl Pts',(-5.91809189155969,3.78736464019659,9.58477982409497));
#47777=CARTESIAN_POINT('Ctrl Pts',(-5.92046687519904,3.78993256795288,9.58078937429346));
#47778=CARTESIAN_POINT('Ctrl Pts',(-5.9227391226194,3.79247183393863,9.57690601577689));
#47779=CARTESIAN_POINT('Ctrl Pts',(-5.92387524632958,3.7937414669315,9.5749643365186));
#47780=CARTESIAN_POINT('Ctrl Pts',(-5.92498568057128,3.79500393752615,9.57304942962578));
#47781=CARTESIAN_POINT('Ctrl Pts',(-5.92607115753564,3.79625843901833,9.57116141170833));
#47782=CARTESIAN_POINT('Ctrl Pts',(-5.92683305117489,3.79713897056225,9.56983621652749));
#47783=CARTESIAN_POINT('Ctrl Pts',(-5.92726953125371,3.79764818979171,9.56907222952432));
#47784=CARTESIAN_POINT('Ctrl Pts',(-5.92804136074465,3.79855856119187,9.56771569930345));
#47785=CARTESIAN_POINT('Ctrl Pts',(-5.92836916391853,3.79894520440501,9.56713956828348));
#47786=CARTESIAN_POINT('Ctrl Pts',(-5.92875713505322,3.79940444874364,9.56645654115736));
#47787=CARTESIAN_POINT('Ctrl Pts',(-5.92925343459007,3.79999725005728,9.5655781323251));
#47788=CARTESIAN_POINT('Ctrl Pts',(-5.93848645652589,3.8110255648672,9.54923645272486));
#47789=CARTESIAN_POINT('Ctrl Pts',(-5.94669689114229,3.8224449053479,9.53347789300259));
#47790=CARTESIAN_POINT('Ctrl Pts',(-5.95392299422338,3.83405494850678,9.51833954729964));
#47791=CARTESIAN_POINT('Ctrl Pts',(-5.96134516857754,3.84598001567197,9.50279044151191));
#47792=CARTESIAN_POINT('Ctrl Pts',(-5.96772976030061,3.85810556804016,9.48789569112109));
#47793=CARTESIAN_POINT('Ctrl Pts',(-5.97315960569138,3.87025001855399,9.47368658169972));
#47794=CARTESIAN_POINT('Ctrl Pts',(-5.97885729588574,3.88299353363197,9.45877656169101));
#47795=CARTESIAN_POINT('Ctrl Pts',(-5.98350473838865,3.89575733437832,9.44462148359316));
#47796=CARTESIAN_POINT('Ctrl Pts',(-5.98722767349291,3.90838022749538,9.43124761886934));
#47797=CARTESIAN_POINT('Ctrl Pts',(-5.99106252997875,3.92138259852372,9.4174717000202));
#47798=CARTESIAN_POINT('Ctrl Pts',(-5.9939175880687,3.93423549544542,9.40452456817365));
#47799=CARTESIAN_POINT('Ctrl Pts',(-5.99594423417257,3.94681679063525,9.39242564731228));
#47800=CARTESIAN_POINT('Ctrl Pts',(-5.99807144897294,3.96002241014849,9.37972633909279));
#47801=CARTESIAN_POINT('Ctrl Pts',(-5.99928703414559,3.97292904470642,9.36796138653384));
#47802=CARTESIAN_POINT('Ctrl Pts',(-5.99976393734273,3.98545223150753,9.35714494908657));
#47803=CARTESIAN_POINT('Ctrl Pts',(-5.99992341808622,3.98964009846637,9.35352783455197));
#47804=CARTESIAN_POINT('Ctrl Pts',(-6.00000020849968,3.99378551625259,9.35001673465345));
#47805=CARTESIAN_POINT('Ctrl Pts',(-6.00000045072924,3.99788654296547,9.34661202516627));
#47806=CARTESIAN_POINT('Ctrl Pts',(-5.71201400288887,3.68829715163933,9.85011170501378));
#47807=CARTESIAN_POINT('Ctrl Pts',(-5.71753251403363,3.68939869751833,9.84750341117836));
#47808=CARTESIAN_POINT('Ctrl Pts',(-5.76529487390022,3.69985385925291,9.82453497351882));
#47809=CARTESIAN_POINT('Ctrl Pts',(-5.85056111518657,3.73367616562962,9.77704813744305));
#47810=CARTESIAN_POINT('Ctrl Pts',(-5.94855988658026,3.81178308395445,9.70555474539447));
#47811=CARTESIAN_POINT('Ctrl Pts',(-6.01625395589241,3.91079812614269,9.63668369038972));
#47812=CARTESIAN_POINT('Ctrl Pts',(-6.04733191412374,4.00898590408443,9.5823388230584));
#47813=CARTESIAN_POINT('Ctrl Pts',(-6.05141294660998,4.07077663899963,9.55425433710709));
#47814=CARTESIAN_POINT('Ctrl Pts',(-6.0507177793919,4.09530166542757,9.54404505445509));
#47815=CARTESIAN_POINT('Ctrl Pts',(-5.59595655141215,3.61240315183009,9.56649342059599));
#47816=CARTESIAN_POINT('Ctrl Pts',(-5.60110598069255,3.61339890679393,9.56406447589219));
#47817=CARTESIAN_POINT('Ctrl Pts',(-5.6456815434348,3.62286184211323,9.54267394188476));
#47818=CARTESIAN_POINT('Ctrl Pts',(-5.72536604180584,3.65366544424186,9.49842961777456));
#47819=CARTESIAN_POINT('Ctrl Pts',(-5.81695119687203,3.72506232608075,9.4319382918881));
#47820=CARTESIAN_POINT('Ctrl Pts',(-5.88006121814607,3.81550180528306,9.36820597259601));
#47821=CARTESIAN_POINT('Ctrl Pts',(-5.90886715308718,3.90480301610222,9.31838067552393));
#47822=CARTESIAN_POINT('Ctrl Pts',(-5.91260953843266,3.96061446345423,9.2929624946597));
#47823=CARTESIAN_POINT('Ctrl Pts',(-5.91197130778005,3.98268771189454,9.28378361798423));
#47824=CARTESIAN_POINT('Ctrl Pts',(-5.57885092685922,3.33845035983965,9.41052417590997));
#47825=CARTESIAN_POINT('Ctrl Pts',(-5.5861727528405,3.33986641830796,9.40711957037098));
#47826=CARTESIAN_POINT('Ctrl Pts',(-5.64948567484334,3.35330499147511,9.37718630234053));
#47827=CARTESIAN_POINT('Ctrl Pts',(-5.7617056670393,3.39666414699678,9.31604358749384));
#47828=CARTESIAN_POINT('Ctrl Pts',(-5.89067084915357,3.49660116044179,9.22466059496501));
#47829=CARTESIAN_POINT('Ctrl Pts',(-5.98091140797734,3.62450296347671,9.13596530973809));
#47830=CARTESIAN_POINT('Ctrl Pts',(-6.02359980578094,3.75425184877456,9.06431252548699));
#47831=CARTESIAN_POINT('Ctrl Pts',(-6.02950843301525,3.83859796744313,9.02597213171389));
#47832=CARTESIAN_POINT('Ctrl Pts',(-6.02850758242405,3.8726184681507,9.01180311927841));
#47833=CARTESIAN_POINT('Ctrl Pts',(-5.67190623754282,3.04595868814745,9.4844095814992));
#47834=CARTESIAN_POINT('Ctrl Pts',(-5.68251837688113,3.04804572148206,9.47951365138588));
#47835=CARTESIAN_POINT('Ctrl Pts',(-5.77421430622641,3.06782257858551,9.43651502745686));
#47836=CARTESIAN_POINT('Ctrl Pts',(-5.93576666433574,3.13108394579195,9.34940645997486));
#47837=CARTESIAN_POINT('Ctrl Pts',(-6.12141055110656,3.2761090354012,9.21954946744644));
#47838=CARTESIAN_POINT('Ctrl Pts',(-6.25271771234329,3.46296215222781,9.09214763633029));
#47839=CARTESIAN_POINT('Ctrl Pts',(-6.31634594300365,3.65598776994707,8.98662376375804));
#47840=CARTESIAN_POINT('Ctrl Pts',(-6.32550617250183,3.78468387418799,8.92824050832422));
#47841=CARTESIAN_POINT('Ctrl Pts',(-6.32396076869737,3.83722167560608,8.90633083239327));
#47842=CARTESIAN_POINT('',(-5.99999999616514,3.21424233716894,9.29218337155546));
#47843=CARTESIAN_POINT('Ctrl Pts',(-5.99998809173024,3.99788654423531,9.34661202443565));
#47844=CARTESIAN_POINT('Ctrl Pts',(-5.99998614033841,3.9756966407273,9.33734346540929));
#47845=CARTESIAN_POINT('Ctrl Pts',(-5.99998781129199,3.95340271551789,9.32855288994148));
#47846=CARTESIAN_POINT('Ctrl Pts',(-6.00000062824778,3.93105674294894,9.32034398865034));
#47847=CARTESIAN_POINT('Ctrl Pts',(-6.00000707142181,3.91982326500558,9.3162173161008));
#47848=CARTESIAN_POINT('Ctrl Pts',(-6.00001566897004,3.90857713712436,9.31223733327578));
#47849=CARTESIAN_POINT('Ctrl Pts',(-6.0000244752767,3.89732800865246,9.30841467970623));
#47850=CARTESIAN_POINT('Ctrl Pts',(-6.00004292770395,3.87375697795109,9.30040482499851));
#47851=CARTESIAN_POINT('Ctrl Pts',(-6.00006398859164,3.85017088480974,9.29308821818177));
#47852=CARTESIAN_POINT('Ctrl Pts',(-6.00008526219979,3.82667220549539,9.28652704165603));
#47853=CARTESIAN_POINT('Ctrl Pts',(-6.00009914087016,3.81134192291226,9.28224660151418));
#47854=CARTESIAN_POINT('Ctrl Pts',(-6.00011245325881,3.79604956090522,9.27828690817963));
#47855=CARTESIAN_POINT('Ctrl Pts',(-6.00012171175511,3.78082955043215,9.27465535168952));
#47856=CARTESIAN_POINT('Ctrl Pts',(-6.00013624555717,3.75693748280786,9.26895460704177));
#47857=CARTESIAN_POINT('Ctrl Pts',(-6.00013967180186,3.73322340031339,9.26406506925698));
#47858=CARTESIAN_POINT('Ctrl Pts',(-6.00012396232745,3.70983392607146,9.25997440600767));
#47859=CARTESIAN_POINT('Ctrl Pts',(-6.00011958298683,3.70331362679944,9.25883404909624));
#47860=CARTESIAN_POINT('Ctrl Pts',(-6.00011380591141,3.69681861084596,9.25775547962216));
#47861=CARTESIAN_POINT('Ctrl Pts',(-6.00010670568716,3.69035213901702,9.25673776074387));
#47862=CARTESIAN_POINT('Ctrl Pts',(-6.00010098822708,3.6851450084649,9.25591824196999));
#47863=CARTESIAN_POINT('Ctrl Pts',(-6.0000944168878,3.67995638621582,9.25513817470758));
#47864=CARTESIAN_POINT('Ctrl Pts',(-6.000087197726,3.67478785822803,9.25439696282023));
#47865=CARTESIAN_POINT('Ctrl Pts',(-6.0000686539007,3.66151148589301,9.25249301550313));
#47866=CARTESIAN_POINT('Ctrl Pts',(-6.00005102575909,3.64818629218426,9.25081443241227));
#47867=CARTESIAN_POINT('Ctrl Pts',(-6.00003057014899,3.6350436628381,9.24939478068352));
#47868=CARTESIAN_POINT('Ctrl Pts',(-6.00000992967953,3.62178226225679,9.24796229942235));
#47869=CARTESIAN_POINT('Ctrl Pts',(-5.99998595813632,3.6087072522888,9.24679357696966));
#47870=CARTESIAN_POINT('Ctrl Pts',(-5.99996791547271,3.59607265740729,9.24587342005326));
#47871=CARTESIAN_POINT('Ctrl Pts',(-5.99995722328277,3.58858532121565,9.24532812958318));
#47872=CARTESIAN_POINT('Ctrl Pts',(-5.99994890967927,3.58125292365108,9.24486915457422));
#47873=CARTESIAN_POINT('Ctrl Pts',(-5.99994782973441,3.57412979372052,9.24448538624468));
#47874=CARTESIAN_POINT('Ctrl Pts',(-5.99994380484314,3.54758230563794,9.24305510415602));
#47875=CARTESIAN_POINT('Ctrl Pts',(-5.99996594985709,3.52094333406006,9.24258915158953));
#47876=CARTESIAN_POINT('Ctrl Pts',(-5.99999369856026,3.49438163998381,9.24317248831033));
#47877=CARTESIAN_POINT('Ctrl Pts',(-6.00002003739072,3.46916950834885,9.24372618651007));
#47878=CARTESIAN_POINT('Ctrl Pts',(-6.00005067895185,3.44402809178869,9.24522532892716));
#47879=CARTESIAN_POINT('Ctrl Pts',(-6.00007008721575,3.41912457662145,9.24769520019424));
#47880=CARTESIAN_POINT('Ctrl Pts',(-6.00007112610705,3.41779153389374,9.24782740819415));
#47881=CARTESIAN_POINT('Ctrl Pts',(-6.00007213476198,3.41645917622918,9.24796238580117));
#47882=CARTESIAN_POINT('Ctrl Pts',(-6.00007311154347,3.41512753029382,9.24810013286172));
#47883=CARTESIAN_POINT('Ctrl Pts',(-6.00009137615634,3.39022738858315,9.25067583353174));
#47884=CARTESIAN_POINT('Ctrl Pts',(-6.00009744663443,3.36557569992992,9.25422408903788));
#47885=CARTESIAN_POINT('Ctrl Pts',(-6.00008943235848,3.34134509983179,9.25871858948095));
#47886=CARTESIAN_POINT('Ctrl Pts',(-6.00008131870418,3.3168140362713,9.26326882247539));
#47887=CARTESIAN_POINT('Ctrl Pts',(-6.00005836465279,3.29271560150319,9.26878868405213));
#47888=CARTESIAN_POINT('Ctrl Pts',(-6.00003565609221,3.26922449003499,9.27519998313362));
#47889=CARTESIAN_POINT('Ctrl Pts',(-6.00001753957257,3.2504836640485,9.28031481308094));
#47890=CARTESIAN_POINT('Ctrl Pts',(-5.99999991840366,3.23212942824875,9.28599586008373));
#47891=CARTESIAN_POINT('Ctrl Pts',(-5.99999992132208,3.21424226856843,9.29218317323549));
#47892=CARTESIAN_POINT('Ctrl Pts',(-5.72001867923018,3.0799677452912,9.45352602807886));
#47893=CARTESIAN_POINT('Ctrl Pts',(-5.77263456943365,3.09390922256596,9.42780054399856));
#47894=CARTESIAN_POINT('Ctrl Pts',(-5.82217073197134,3.11234983333796,9.40144596360093));
#47895=CARTESIAN_POINT('Ctrl Pts',(-5.86880003058743,3.13480613498432,9.37455093300828));
#47896=CARTESIAN_POINT('Ctrl Pts',(-5.91542932732122,3.15726243572417,9.34765590350132));
#47897=CARTESIAN_POINT('Ctrl Pts',(-5.95915199503964,3.18373461472357,9.32022095924429));
#47898=CARTESIAN_POINT('Ctrl Pts',(-6.00000008250755,3.21424239912979,9.29218356476923));
#47899=CARTESIAN_POINT('Ctrl Pts',(6.05073416954824,-6.21799316481487,8.31849901783411));
#47900=CARTESIAN_POINT('Ctrl Pts',(6.05138851905234,-6.23846348656192,8.30285784976043));
#47901=CARTESIAN_POINT('Ctrl Pts',(6.04748115695756,-6.29320366773436,8.26366670974756));
#47902=CARTESIAN_POINT('Ctrl Pts',(6.01688298770343,-6.38906583647729,8.20581144498912));
#47903=CARTESIAN_POINT('Ctrl Pts',(5.94901053102531,-6.49891818272934,8.15405555171379));
#47904=CARTESIAN_POINT('Ctrl Pts',(5.85047649675774,-6.60050118995466,8.12193834043125));
#47905=CARTESIAN_POINT('Ctrl Pts',(5.76680004331251,-6.65737095906819,8.11655682688315));
#47906=CARTESIAN_POINT('Ctrl Pts',(5.72097979789639,-6.6816926781363,8.11871977358638));
#47907=CARTESIAN_POINT('Ctrl Pts',(5.71762411915974,-6.68343928363121,8.11890412240399));
#47908=CARTESIAN_POINT('Ctrl Pts',(5.91195465679019,-6.04887183299702,8.09084333278917));
#47909=CARTESIAN_POINT('Ctrl Pts',(5.91255544435238,-6.06728713996125,8.07676162461918));
#47910=CARTESIAN_POINT('Ctrl Pts',(5.90897244737554,-6.11676498715629,8.04139360101593));
#47911=CARTESIAN_POINT('Ctrl Pts',(5.8806167381171,-6.20428020149151,7.9889774803304));
#47912=CARTESIAN_POINT('Ctrl Pts',(5.81734518076637,-6.3053298833833,7.94212151691093));
#47913=CARTESIAN_POINT('Ctrl Pts',(5.72526412879784,-6.39917473945531,7.91333790687482));
#47914=CARTESIAN_POINT('Ctrl Pts',(5.64706911429235,-6.45181161411251,7.90892600936277));
#47915=CARTESIAN_POINT('Ctrl Pts',(5.60430646326424,-6.47432847354459,7.91117108524512));
#47916=CARTESIAN_POINT('Ctrl Pts',(5.60117502174684,-6.47594550881959,7.91135914934469));
#47917=CARTESIAN_POINT('Ctrl Pts',(6.02850429655224,-5.86846171619569,7.8594200448853));
#47918=CARTESIAN_POINT('Ctrl Pts',(6.0294458481419,-5.89685901208869,7.83772995718211));
#47919=CARTESIAN_POINT('Ctrl Pts',(6.02378949073807,-5.9716166886548,7.78420864811893));
#47920=CARTESIAN_POINT('Ctrl Pts',(5.98173069054818,-6.09820219289116,7.70765349338715));
#47921=CARTESIAN_POINT('Ctrl Pts',(5.89124051535816,-6.23988002999824,7.64065795139567));
#47922=CARTESIAN_POINT('Ctrl Pts',(5.76157170010822,-6.36977135011668,7.59951888803959));
#47923=CARTESIAN_POINT('Ctrl Pts',(5.65144406230163,-6.44290468661577,7.59275046404611));
#47924=CARTESIAN_POINT('Ctrl Pts',(5.5907186306291,-6.47449766812669,7.59572432625113));
#47925=CARTESIAN_POINT('Ctrl Pts',(5.58626901549766,-6.47676845393569,7.59597617732597));
#47926=CARTESIAN_POINT('Ctrl Pts',(6.32399708752164,-5.79500234059736,7.77590234717818));
#47927=CARTESIAN_POINT('Ctrl Pts',(6.32545039447524,-5.83887649506691,7.74242252558534));
#47928=CARTESIAN_POINT('Ctrl Pts',(6.31668181867899,-5.95288791984639,7.66066908075003));
#47929=CARTESIAN_POINT('Ctrl Pts',(6.25395529759717,-6.14035453070281,7.54621728843544));
#47930=CARTESIAN_POINT('Ctrl Pts',(6.12226590114595,-6.34546389958309,7.44724201576168));
#47931=CARTESIAN_POINT('Ctrl Pts',(5.93560336462689,-6.53156166818348,7.38615613310121));
#47932=CARTESIAN_POINT('Ctrl Pts',(5.77705748510178,-6.63648756796766,7.37524949342088));
#47933=CARTESIAN_POINT('Ctrl Pts',(5.68912159307504,-6.68208921880697,7.37912115719306));
#47934=CARTESIAN_POINT('Ctrl Pts',(5.68267531632909,-6.68536861183381,7.37945506135755));
#47935=CARTESIAN_POINT('',(5.73278512538254,-6.6558845698369,8.10254539185841));
#47936=CARTESIAN_POINT('',(5.72001596702532,-6.64701164882605,7.39409270018585));
#47937=CARTESIAN_POINT('Origin',(5.89875799467743,-6.95917611500265,7.74135837685731));
#47938=CARTESIAN_POINT('',(5.99999998587216,-6.44014763970973,7.42970560850941));
#47939=CARTESIAN_POINT('Ctrl Pts',(6.00000001391262,-6.44014774286491,7.4297057275149));
#47940=CARTESIAN_POINT('Ctrl Pts',(5.95924742401491,-6.47958993893993,7.4173332049442));
#47941=CARTESIAN_POINT('Ctrl Pts',(5.91558896907838,-6.51654787976713,7.40812577084738));
#47942=CARTESIAN_POINT('Ctrl Pts',(5.86896519300227,-6.55107434372493,7.40211809013247));
#47943=CARTESIAN_POINT('Ctrl Pts',(5.82234141692615,-6.58560080768272,7.39611040941757));
#47944=CARTESIAN_POINT('Ctrl Pts',(5.77275207242162,-6.61769538986344,7.39330201919218));
#47945=CARTESIAN_POINT('Ctrl Pts',(5.72001606109157,-6.64701181310764,7.39409288292955));
#47946=CARTESIAN_POINT('',(5.99998098390851,-6.09545783085286,8.13557311429686));
#47947=CARTESIAN_POINT('Ctrl Pts',(5.99998098390851,-6.09545783085286,8.13557311429686));
#47948=CARTESIAN_POINT('Ctrl Pts',(5.99997795080516,-6.09912681471699,8.10718396161426));
#47949=CARTESIAN_POINT('Ctrl Pts',(5.99997856657729,-6.10348550211984,8.07931777015222));
#47950=CARTESIAN_POINT('Ctrl Pts',(5.99997355844376,-6.10855067239734,8.05200283568773));
#47951=CARTESIAN_POINT('Ctrl Pts',(5.99997239516563,-6.10972719889876,8.04565818338163));
#47952=CARTESIAN_POINT('Ctrl Pts',(5.9999707973073,-6.1109416624435,8.0393432201366));
#47953=CARTESIAN_POINT('Ctrl Pts',(5.99996848874586,-6.11219397191406,8.0330581951774));
#47954=CARTESIAN_POINT('Ctrl Pts',(5.99995522862971,-6.1193870960483,7.9969577217872));
#47955=CARTESIAN_POINT('Ctrl Pts',(5.99992305431804,-6.12783083555669,7.96184754052742));
#47956=CARTESIAN_POINT('Ctrl Pts',(5.9999092524274,-6.13751521093299,7.92768174892519));
#47957=CARTESIAN_POINT('Ctrl Pts',(5.99990745008773,-6.13877985897252,7.92322016005754));
#47958=CARTESIAN_POINT('Ctrl Pts',(5.99990591277677,-6.14006565105881,7.91877462908017));
#47959=CARTESIAN_POINT('Ctrl Pts',(5.99990469357332,-6.14137257067106,7.91434501280618));
#47960=CARTESIAN_POINT('Ctrl Pts',(5.99989649855682,-6.15015718143404,7.88457083661982));
#47961=CARTESIAN_POINT('Ctrl Pts',(5.9998958870529,-6.15990751700441,7.85553451876249));
#47962=CARTESIAN_POINT('Ctrl Pts',(5.99989864392041,-6.17061785514147,7.82724658889151));
#47963=CARTESIAN_POINT('Ctrl Pts',(5.99990072599376,-6.17870664055037,7.8058826514079));
#47964=CARTESIAN_POINT('Ctrl Pts',(5.99990523562835,-6.18734279182029,7.78494486521122));
#47965=CARTESIAN_POINT('Ctrl Pts',(5.99991500873739,-6.19653415230066,7.7644298683282));
#47966=CARTESIAN_POINT('Ctrl Pts',(5.99991850715718,-6.19982432713193,7.75708624095635));
#47967=CARTESIAN_POINT('Ctrl Pts',(5.99992700898706,-6.20329286828286,7.74955169037503));
#47968=CARTESIAN_POINT('Ctrl Pts',(5.99993271621318,-6.20679880098116,7.74216830770547));
#47969=CARTESIAN_POINT('Ctrl Pts',(5.99993849506638,-6.21034873398374,7.73469226179561));
#47970=CARTESIAN_POINT('Ctrl Pts',(5.99994113580615,-6.21393686387291,7.72737150855663));
#47971=CARTESIAN_POINT('Ctrl Pts',(5.99994639777485,-6.21736531306685,7.72054982169873));
#47972=CARTESIAN_POINT('Ctrl Pts',(5.99994718576889,-6.21787873260638,7.71952825564151));
#47973=CARTESIAN_POINT('Ctrl Pts',(5.99994806094423,-6.21838848348708,7.71851785694636));
#47974=CARTESIAN_POINT('Ctrl Pts',(5.99994907258546,-6.21889381249274,7.71751975375738));
#47975=CARTESIAN_POINT('Ctrl Pts',(5.99997579529468,-6.23224218120401,7.69115465452693));
#47976=CARTESIAN_POINT('Ctrl Pts',(5.99996192119624,-6.24651037187084,7.66578871787388));
#47977=CARTESIAN_POINT('Ctrl Pts',(5.9999372794125,-6.26162446045842,7.64138874328849));
#47978=CARTESIAN_POINT('Ctrl Pts',(5.99991690557245,-6.27412079703479,7.62121483117286));
#47979=CARTESIAN_POINT('Ctrl Pts',(5.999890038424,-6.28719634665374,7.60170065612216));
#47980=CARTESIAN_POINT('Ctrl Pts',(5.99987287327607,-6.30083610829983,7.5828324562705));
#47981=CARTESIAN_POINT('Ctrl Pts',(5.99985320162157,-6.31646758899985,7.5612090650795));
#47982=CARTESIAN_POINT('Ctrl Pts',(5.99984785764865,-6.33284019468986,7.54043265309109));
#47983=CARTESIAN_POINT('Ctrl Pts',(5.99986495093018,-6.34996887007247,7.52050046833024));
#47984=CARTESIAN_POINT('Ctrl Pts',(5.99988150843523,-6.36656065957162,7.50119304341716));
#47985=CARTESIAN_POINT('Ctrl Pts',(5.99991970425662,-6.38386297476151,7.48267754176755));
#47986=CARTESIAN_POINT('Ctrl Pts',(5.99995446206205,-6.4019071796299,7.4649826235714));
#47987=CARTESIAN_POINT('Ctrl Pts',(5.99997833382845,-6.41429999437422,7.45282969997515));
#47988=CARTESIAN_POINT('Ctrl Pts',(5.99999989103997,-6.42704314418577,7.44106453666026));
#47989=CARTESIAN_POINT('Ctrl Pts',(5.9999998934196,-6.44014754776427,7.42970550243612));
#47990=CARTESIAN_POINT('Ctrl Pts',(5.99998098390851,-6.09545783085286,8.13557311429686));
#47991=CARTESIAN_POINT('Ctrl Pts',(5.99997772867445,-6.11094053579484,8.12985643031688));
#47992=CARTESIAN_POINT('Ctrl Pts',(5.99924872607125,-6.12747879190542,8.12421726742495));
#47993=CARTESIAN_POINT('Ctrl Pts',(5.997604829686,-6.14501797924142,8.11878177647199));
#47994=CARTESIAN_POINT('Ctrl Pts',(5.99698611775157,-6.15161918879596,8.11673602519944));
#47995=CARTESIAN_POINT('Ctrl Pts',(5.99623762779396,-6.15836181538866,8.11471942401007));
#47996=CARTESIAN_POINT('Ctrl Pts',(5.99534851590325,-6.16524155001333,8.11273984489372));
#47997=CARTESIAN_POINT('Ctrl Pts',(5.99290206688184,-6.18417158594679,8.10729290459006));
#47998=CARTESIAN_POINT('Ctrl Pts',(5.98939069302446,-6.20414337978211,8.1021243085497));
#47999=CARTESIAN_POINT('Ctrl Pts',(5.98464484566116,-6.22504366912051,8.09738742436529));
#48000=CARTESIAN_POINT('Ctrl Pts',(5.98034782442747,-6.24396736813623,8.09309851864123));
#48001=CARTESIAN_POINT('Ctrl Pts',(5.97503916761414,-6.26365224354456,8.08916334415599));
#48002=CARTESIAN_POINT('Ctrl Pts',(5.96858845952096,-6.2839738607091,8.08571964003558));
#48003=CARTESIAN_POINT('Ctrl Pts',(5.96735211223312,-6.28786871626649,8.08505961726167));
#48004=CARTESIAN_POINT('Ctrl Pts',(5.96607378803647,-6.29178683360547,8.08441772769999));
#48005=CARTESIAN_POINT('Ctrl Pts',(5.96475252746431,-6.29572714730741,8.0837950604321));
#48006=CARTESIAN_POINT('Ctrl Pts',(5.96410107363795,-6.29766993777001,8.08348805136608));
#48007=CARTESIAN_POINT('Ctrl Pts',(5.96343918144502,-6.29961812320199,8.08318571602489));
#48008=CARTESIAN_POINT('Ctrl Pts',(5.96276677815532,-6.30157158264049,8.08288816314251));
#48009=CARTESIAN_POINT('Ctrl Pts',(5.9581909831883,-6.31486513727338,8.08086327569404));
#48010=CARTESIAN_POINT('Ctrl Pts',(5.95312831785123,-6.32840360031641,8.07905954701971));
#48011=CARTESIAN_POINT('Ctrl Pts',(5.94755665828282,-6.34214417495224,8.07751341825763));
#48012=CARTESIAN_POINT('Ctrl Pts',(5.94477082849862,-6.34901446227015,8.07674035387659));
#48013=CARTESIAN_POINT('Ctrl Pts',(5.94185770909024,-6.35593526246158,8.07603170829155));
#48014=CARTESIAN_POINT('Ctrl Pts',(5.93881470100109,-6.36290026499228,8.07539249392606));
#48015=CARTESIAN_POINT('Ctrl Pts',(5.93729319695651,-6.36638276625764,8.07507288674331));
#48016=CARTESIAN_POINT('Ctrl Pts',(5.93573921753015,-6.3698763169927,8.07477063876403));
#48017=CARTESIAN_POINT('Ctrl Pts',(5.93415243365218,-6.37338008924375,8.0744863991385));
#48018=CARTESIAN_POINT('Ctrl Pts',(5.93309118143456,-6.37572343676769,8.07429629767785));
#48019=CARTESIAN_POINT('Ctrl Pts',(5.93174669274984,-6.378654997998,8.07407033155907));
#48020=CARTESIAN_POINT('Ctrl Pts',(5.93065585008325,-6.38100281960402,8.07389808521894));
#48021=CARTESIAN_POINT('Ctrl Pts',(5.93011566524478,-6.38216545989472,8.07381278890237));
#48022=CARTESIAN_POINT('Ctrl Pts',(5.92963855434378,-6.38318525846102,8.07374007905873));
#48023=CARTESIAN_POINT('Ctrl Pts',(5.9292933318568,-6.38392121979147,8.07368836917371));
#48024=CARTESIAN_POINT('Ctrl Pts',(5.92334489559235,-6.39660237247523,8.07279736998656));
#48025=CARTESIAN_POINT('Ctrl Pts',(5.91661161124661,-6.41017628257469,8.07209947444279));
#48026=CARTESIAN_POINT('Ctrl Pts',(5.90895442130354,-6.42453791539892,8.07172163154264));
#48027=CARTESIAN_POINT('Ctrl Pts',(5.90810063408666,-6.42613925722406,8.07167950153926));
#48028=CARTESIAN_POINT('Ctrl Pts',(5.90723535216071,-6.42775034845592,8.07164138054929));
#48029=CARTESIAN_POINT('Ctrl Pts',(5.90635837684122,-6.42937100889063,8.07160746788664));
#48030=CARTESIAN_POINT('Ctrl Pts',(5.89875324496737,-6.44342537969755,8.07131337720253));
#48031=CARTESIAN_POINT('Ctrl Pts',(5.89026820006472,-6.45820265893285,8.07133406150863));
#48032=CARTESIAN_POINT('Ctrl Pts',(5.88078908081662,-6.47357436698548,8.0717985590752));
#48033=CARTESIAN_POINT('Ctrl Pts',(5.87367899091882,-6.48510436500285,8.07214696902439));
#48034=CARTESIAN_POINT('Ctrl Pts',(5.8660096694548,-6.49696817421058,8.072745410005));
#48035=CARTESIAN_POINT('Ctrl Pts',(5.85773624959864,-6.50909451012828,8.07365714025404));
#48036=CARTESIAN_POINT('Ctrl Pts',(5.84731781891584,-6.52436478437901,8.07480525053566));
#48037=CARTESIAN_POINT('Ctrl Pts',(5.83594081812807,-6.54005343178411,8.07644904341306));
#48038=CARTESIAN_POINT('Ctrl Pts',(5.82352550448333,-6.55597597045343,8.07873664042811));
#48039=CARTESIAN_POINT('Ctrl Pts',(5.81177708120982,-6.57104322765119,8.08090135883807));
#48040=CARTESIAN_POINT('Ctrl Pts',(5.79909789939182,-6.58631935505125,8.0836433580915));
#48041=CARTESIAN_POINT('Ctrl Pts',(5.78545577118372,-6.60162414051487,8.087086205805));
#48042=CARTESIAN_POINT('Ctrl Pts',(5.7726902189806,-6.61594551580274,8.09030783307193));
#48043=CARTESIAN_POINT('Ctrl Pts',(5.75908137506514,-6.63029216541615,8.09414298561802));
#48044=CARTESIAN_POINT('Ctrl Pts',(5.74462482502411,-6.6444786197375,8.0987080025764));
#48045=CARTESIAN_POINT('Ctrl Pts',(5.74073850671199,-6.64829232889056,8.09993520470623));
#48046=CARTESIAN_POINT('Ctrl Pts',(5.73679106169321,-6.65209422866094,8.10121524939007));
#48047=CARTESIAN_POINT('Ctrl Pts',(5.73278271922475,-6.65588017670764,8.10255062446566));
#48048=CARTESIAN_POINT('Ctrl Pts',(5.99928507441383,-9.87990138305988,16.996213761673));
#48049=CARTESIAN_POINT('Ctrl Pts',(5.99928507441383,-9.88326633338716,16.9632224620409));
#48050=CARTESIAN_POINT('Ctrl Pts',(5.99928507441383,-9.93380725827969,16.441713240187));
#48051=CARTESIAN_POINT('Ctrl Pts',(5.99928507441383,-9.95153396276962,15.4241420274085));
#48052=CARTESIAN_POINT('Ctrl Pts',(5.99928507441383,-9.7585538486203,13.962336164721));
#48053=CARTESIAN_POINT('Ctrl Pts',(5.99928507441383,-9.35132498744714,12.5448501172522));
#48054=CARTESIAN_POINT('Ctrl Pts',(5.99928507441383,-8.73824353394044,11.2027127608678));
#48055=CARTESIAN_POINT('Ctrl Pts',(5.99928507441383,-7.93284774114545,9.96536136565117));
#48056=CARTESIAN_POINT('Ctrl Pts',(5.99928507441383,-7.00873643877852,8.92486523185514));
#48057=CARTESIAN_POINT('Ctrl Pts',(5.99928507441383,-6.3262035229329,8.33936349584419));
#48058=CARTESIAN_POINT('Ctrl Pts',(5.99928507441383,-6.00174807522006,8.09410018447627));
#48059=CARTESIAN_POINT('Ctrl Pts',(6.01063753142534,-10.0685448362718,17.0154707577556));
#48060=CARTESIAN_POINT('Ctrl Pts',(6.01063753142534,-10.0719743009096,16.9818450948751));
#48061=CARTESIAN_POINT('Ctrl Pts',(6.01063753142534,-10.1234844014194,16.4503158788653));
#48062=CARTESIAN_POINT('Ctrl Pts',(6.01063753142534,-10.141555854936,15.4134041054537));
#48063=CARTESIAN_POINT('Ctrl Pts',(6.01063753142534,-9.94485299521173,13.9234127767083));
#48064=CARTESIAN_POINT('Ctrl Pts',(6.01063753142534,-9.52986270675546,12.4789235515721));
#48065=CARTESIAN_POINT('Ctrl Pts',(6.01063753142534,-8.90499026070635,11.1109544163187));
#48066=CARTESIAN_POINT('Ctrl Pts',(6.01063753142534,-8.08420677078012,9.84997711608917));
#48067=CARTESIAN_POINT('Ctrl Pts',(6.01063753142534,-7.14233094405397,8.78947077084895));
#48068=CARTESIAN_POINT('Ctrl Pts',(6.01063753142534,-6.44679011346318,8.19281074633989));
#48069=CARTESIAN_POINT('Ctrl Pts',(6.01063753142534,-6.11609106980937,7.94282973159906));
#48070=CARTESIAN_POINT('Ctrl Pts',(5.90340740959394,-10.2250068268442,17.0314426236621));
#48071=CARTESIAN_POINT('Ctrl Pts',(5.90340740959394,-10.2284898000314,16.9972908161699));
#48072=CARTESIAN_POINT('Ctrl Pts',(5.90340740959394,-10.2808037405078,16.4574509580307));
#48073=CARTESIAN_POINT('Ctrl Pts',(5.90340740959394,-10.2991611308929,15.4044980097731));
#48074=CARTESIAN_POINT('Ctrl Pts',(5.90340740959394,-10.0993706040784,13.8911294895681));
#48075=CARTESIAN_POINT('Ctrl Pts',(5.90340740959394,-9.67794294214227,12.4242436699105));
#48076=CARTESIAN_POINT('Ctrl Pts',(5.90340740959394,-9.04329097746749,11.0348495051978));
#48077=CARTESIAN_POINT('Ctrl Pts',(5.90340740959394,-8.20974484096032,9.7542767402771));
#48078=CARTESIAN_POINT('Ctrl Pts',(5.90340740959394,-7.25313501315403,8.67717380786529));
#48079=CARTESIAN_POINT('Ctrl Pts',(5.90340740959394,-6.54680534150376,8.07125903319736));
#48080=CARTESIAN_POINT('Ctrl Pts',(5.90340740959394,-6.21092782262036,7.8173651275034));
#48081=CARTESIAN_POINT('Ctrl Pts',(5.72171463267843,-10.2827457696937,17.0373366983171));
#48082=CARTESIAN_POINT('Ctrl Pts',(5.72171463267843,-10.2862484890613,17.002990728433));
#48083=CARTESIAN_POINT('Ctrl Pts',(5.72171463267843,-10.3388590694426,16.4600840060095));
#48084=CARTESIAN_POINT('Ctrl Pts',(5.72171463267843,-10.3573219786997,15.4012114061234));
#48085=CARTESIAN_POINT('Ctrl Pts',(5.72171463267843,-10.1563920145498,13.8792160346507));
#48086=CARTESIAN_POINT('Ctrl Pts',(5.72171463267843,-9.73258877795812,12.4040652320039));
#48087=CARTESIAN_POINT('Ctrl Pts',(5.72171463267843,-9.09432789162046,11.0067646195493));
#48088=CARTESIAN_POINT('Ctrl Pts',(5.72171463267843,-8.2560719740424,9.71896056854079));
#48089=CARTESIAN_POINT('Ctrl Pts',(5.72171463267843,-7.29402487905501,8.63573302148622));
#48090=CARTESIAN_POINT('Ctrl Pts',(5.72171463267843,-6.58371381693797,8.02640297970358));
#48091=CARTESIAN_POINT('Ctrl Pts',(5.72171463267843,-6.24592529280697,7.77106510550619));
#48092=CARTESIAN_POINT('',(6.,-9.9133032909571,16.8993688494793));
#48093=CARTESIAN_POINT('Ctrl Pts',(5.99999999999973,-9.9133032909571,16.8993688494793));
#48094=CARTESIAN_POINT('Ctrl Pts',(5.99999999999973,-9.92726798483485,16.7473134109464));
#48095=CARTESIAN_POINT('Ctrl Pts',(6.00000000003746,-9.93769910712317,16.595447980401));
#48096=CARTESIAN_POINT('Ctrl Pts',(5.99999999795221,-9.94464892471596,16.4436799771047));
#48097=CARTESIAN_POINT('Ctrl Pts',(5.99999999586004,-9.95162180286593,16.2914083843728));
#48098=CARTESIAN_POINT('Ctrl Pts',(5.99999999148609,-9.95509022250395,16.1392344036198));
#48099=CARTESIAN_POINT('Ctrl Pts',(5.99999999087348,-9.95505464980814,15.9870607740922));
#48100=CARTESIAN_POINT('Ctrl Pts',(5.99999999026188,-9.95501913510092,15.8351352093599));
#48101=CARTESIAN_POINT('Ctrl Pts',(5.99999999695621,-9.9514910181508,15.6832095322195));
#48102=CARTESIAN_POINT('Ctrl Pts',(5.99999999953312,-9.94441903913389,15.5311901549495));
#48103=CARTESIAN_POINT('Ctrl Pts',(5.99999999982103,-9.94362892143478,15.5142057718932));
#48104=CARTESIAN_POINT('Ctrl Pts',(5.99999999999973,-9.94279451441727,15.4972202267563));
#48105=CARTESIAN_POINT('Ctrl Pts',(5.99999999999973,-9.94191570654023,15.4802333954616));
#48106=CARTESIAN_POINT('Ctrl Pts',(5.99999999999973,-9.94094255237386,15.4614229067532));
#48107=CARTESIAN_POINT('Ctrl Pts',(5.9999999997797,-9.93991594443028,15.4426107520415));
#48108=CARTESIAN_POINT('Ctrl Pts',(5.99999999940201,-9.93883579420981,15.4237975366115));
#48109=CARTESIAN_POINT('Ctrl Pts',(5.99999999572692,-9.92832550450536,15.2407374948734));
#48110=CARTESIAN_POINT('Ctrl Pts',(5.99999998184225,-9.91274149826588,15.057576758604));
#48111=CARTESIAN_POINT('Ctrl Pts',(5.99999998033318,-9.89207963590134,14.8748162763473));
#48112=CARTESIAN_POINT('Ctrl Pts',(5.99999997882271,-9.87139856928759,14.6918859266418));
#48113=CARTESIAN_POINT('Ctrl Pts',(5.9999999873102,-9.84563021940766,14.5093570258918));
#48114=CARTESIAN_POINT('Ctrl Pts',(5.99999999411999,-9.8148225770521,14.3277311598507));
#48115=CARTESIAN_POINT('Ctrl Pts',(5.99999999739309,-9.8000150339968,14.2404335730922));
#48116=CARTESIAN_POINT('Ctrl Pts',(5.99999999999973,-9.78404408500407,14.1533445516174));
#48117=CARTESIAN_POINT('Ctrl Pts',(5.99999999999973,-9.76691931257516,14.0665192561223));
#48118=CARTESIAN_POINT('Ctrl Pts',(5.99999999999973,-9.7602057349753,14.032480359468));
#48119=CARTESIAN_POINT('Ctrl Pts',(5.99999999960408,-9.75331357134629,13.9984822486694));
#48120=CARTESIAN_POINT('Ctrl Pts',(5.99999999898853,-9.74624308953661,13.9645259256645));
#48121=CARTESIAN_POINT('Ctrl Pts',(5.99999999507832,-9.70132904128378,13.7488240865275));
#48122=CARTESIAN_POINT('Ctrl Pts',(5.99999998615653,-9.6492238410253,13.5348078243482));
#48123=CARTESIAN_POINT('Ctrl Pts',(5.99999998771989,-9.59004045253633,13.3227596842198));
#48124=CARTESIAN_POINT('Ctrl Pts',(5.99999998928325,-9.53085706404735,13.1107115440914));
#48125=CARTESIAN_POINT('Ctrl Pts',(5.99999999999973,-9.46459533129902,12.9006309202312));
#48126=CARTESIAN_POINT('Ctrl Pts',(5.99999999999973,-9.39131593584195,12.6928136949694));
#48127=CARTESIAN_POINT('Ctrl Pts',(5.99999999999973,-9.37455367135169,12.6452766311913));
#48128=CARTESIAN_POINT('Ctrl Pts',(5.99999999934667,-9.35742661566423,12.5978569729541));
#48129=CARTESIAN_POINT('Ctrl Pts',(5.99999999845569,-9.33993664766838,12.5505627050574));
#48130=CARTESIAN_POINT('Ctrl Pts',(5.99999999449755,-9.26223771587858,12.3404585987361));
#48131=CARTESIAN_POINT('Ctrl Pts',(5.99999998895131,-9.17737250715791,12.1328304142742));
#48132=CARTESIAN_POINT('Ctrl Pts',(5.99999999115155,-9.08561181914581,11.9283179829288));
#48133=CARTESIAN_POINT('Ctrl Pts',(5.99999999312724,-9.00321607235455,11.7446777457656));
#48134=CARTESIAN_POINT('Ctrl Pts',(5.99999999999973,-8.91526129320293,11.5635498380372));
#48135=CARTESIAN_POINT('Ctrl Pts',(5.99999999999973,-8.82197657218222,11.3853836525694));
#48136=CARTESIAN_POINT('Ctrl Pts',(5.99999999999973,-8.79096372712254,11.3261516556857));
#48137=CARTESIAN_POINT('Ctrl Pts',(5.9999999991363,-8.75935995230306,11.2672485469129));
#48138=CARTESIAN_POINT('Ctrl Pts',(5.99999999780781,-8.72716898892441,11.2086816936824));
#48139=CARTESIAN_POINT('Ctrl Pts',(5.99999999336895,-8.61960963189566,11.0129928289979));
#48140=CARTESIAN_POINT('Ctrl Pts',(5.99999998477723,-8.50549803860959,10.8210557635332));
#48141=CARTESIAN_POINT('Ctrl Pts',(5.99999998688355,-8.38499730264774,10.6331578953627));
#48142=CARTESIAN_POINT('Ctrl Pts',(5.99999998863004,-8.28508151746534,10.477358323829));
#48143=CARTESIAN_POINT('Ctrl Pts',(5.99999999999973,-8.18077212285937,10.324336137916));
#48144=CARTESIAN_POINT('Ctrl Pts',(5.99999999999973,-8.07214107678254,10.1742724167866));
#48145=CARTESIAN_POINT('Ctrl Pts',(5.99999999999973,-8.02304831449606,10.1064553161024));
#48146=CARTESIAN_POINT('Ctrl Pts',(5.99999999683371,-7.97308075075413,10.039234252959));
#48147=CARTESIAN_POINT('Ctrl Pts',(5.99999999319106,-7.92226250667201,9.97264859238534));
#48148=CARTESIAN_POINT('Ctrl Pts',(5.99999998466704,-7.80334493725567,9.81683437533751));
#48149=CARTESIAN_POINT('Ctrl Pts',(5.99999997595993,-7.67976621500289,9.66450210452235));
#48150=CARTESIAN_POINT('Ctrl Pts',(5.99999997954458,-7.5519155657467,9.5160655345673));
#48151=CARTESIAN_POINT('Ctrl Pts',(5.99999998312923,-7.4240649164905,9.36762896461225));
#48152=CARTESIAN_POINT('Ctrl Pts',(5.99999999999973,-7.29194273064179,9.22308846257705));
#48153=CARTESIAN_POINT('Ctrl Pts',(5.99999999999973,-7.15597857436782,9.0828176121166));
#48154=CARTESIAN_POINT('Ctrl Pts',(5.99999999999973,-7.08651113747799,9.01114977907237));
#48155=CARTESIAN_POINT('Ctrl Pts',(5.99999999545184,-7.01602931504084,8.94061618500218));
#48156=CARTESIAN_POINT('Ctrl Pts',(5.99999999307309,-6.94451772313367,8.87118606265322));
#48157=CARTESIAN_POINT('Ctrl Pts',(5.9999999894095,-6.83438040522495,8.7642544833994));
#48158=CARTESIAN_POINT('Ctrl Pts',(5.99999999031162,-6.72180218208047,8.65993850515689));
#48159=CARTESIAN_POINT('Ctrl Pts',(5.99999999276239,-6.60672591906142,8.5581688414802));
#48160=CARTESIAN_POINT('Ctrl Pts',(5.99999999520021,-6.49225775995384,8.45693696491031));
#48161=CARTESIAN_POINT('Ctrl Pts',(5.9999999978678,-6.37531755059047,8.35822425283109));
#48162=CARTESIAN_POINT('Ctrl Pts',(5.99999999875692,-6.25581493514787,8.26200091361462));
#48163=CARTESIAN_POINT('Ctrl Pts',(5.99999999915085,-6.20286922387451,8.21936910077066));
#48164=CARTESIAN_POINT('Ctrl Pts',(5.99999999931877,-6.14942010854285,8.1772264711099));
#48165=CARTESIAN_POINT('Ctrl Pts',(5.99999999931449,-6.09545783333519,8.13557311294732));
#48166=CARTESIAN_POINT('',(5.73644276520453,-10.2877350949113,16.9337809954847));
#48167=CARTESIAN_POINT('Origin',(5.6,-9.91330329093393,16.8993688493888));
#48168=CARTESIAN_POINT('Ctrl Pts',(5.7364427639771,-10.2877350956467,16.9337809951854));
#48169=CARTESIAN_POINT('Ctrl Pts',(5.73708792260912,-10.3280497960652,16.4922344854671));
#48170=CARTESIAN_POINT('Ctrl Pts',(5.73762563125427,-10.3398885462273,16.0482065524611));
#48171=CARTESIAN_POINT('Ctrl Pts',(5.7380559556032,-10.323253700388,15.6057354409328));
#48172=CARTESIAN_POINT('Ctrl Pts',(5.7381218985348,-10.3207045755147,15.5379311386264));
#48173=CARTESIAN_POINT('Ctrl Pts',(5.73818531979119,-10.3174868144141,15.4701632949043));
#48174=CARTESIAN_POINT('Ctrl Pts',(5.73824621957937,-10.313600420569,15.4024463333027));
#48175=CARTESIAN_POINT('Ctrl Pts',(5.73865147700528,-10.2877384264188,14.951824050896));
#48176=CARTESIAN_POINT('Ctrl Pts',(5.73894508028782,-10.2322688266212,14.5034591043037));
#48177=CARTESIAN_POINT('Ctrl Pts',(5.73912707523813,-10.1478930445972,14.0611434726086));
#48178=CARTESIAN_POINT('Ctrl Pts',(5.73915087509495,-10.1368590487234,14.0033009408067));
#48179=CARTESIAN_POINT('Ctrl Pts',(5.73917276625726,-10.1253307016213,13.9455617894377));
#48180=CARTESIAN_POINT('Ctrl Pts',(5.73919274878682,-10.1133095567134,13.8879344352759));
#48181=CARTESIAN_POINT('Ctrl Pts',(5.73934700450547,-10.0205119786601,13.443078397285));
#48182=CARTESIAN_POINT('Ctrl Pts',(5.73938752580425,-9.89834963657934,13.004888446781));
#48183=CARTESIAN_POINT('Ctrl Pts',(5.73931431960101,-9.74808346097681,12.5770746854827));
#48184=CARTESIAN_POINT('Ctrl Pts',(5.7393053689643,-9.7297110022455,12.5247675668472));
#48185=CARTESIAN_POINT('Ctrl Pts',(5.73929471816761,-9.71091839539337,12.472615502568));
#48186=CARTESIAN_POINT('Ctrl Pts',(5.73928236718371,-9.69170792511209,12.4206252243643));
#48187=CARTESIAN_POINT('Ctrl Pts',(5.73918135673792,-9.53459832292005,11.9954314728928));
#48188=CARTESIAN_POINT('Ctrl Pts',(5.73896663198965,-9.34954214044669,11.5810624745185));
#48189=CARTESIAN_POINT('Ctrl Pts',(5.73863815758599,-9.13842733572597,11.1810270495251));
#48190=CARTESIAN_POINT('Ctrl Pts',(5.73859603581172,-9.11135511929459,11.1297286783854));
#48191=CARTESIAN_POINT('Ctrl Pts',(5.73855204348063,-9.08385435544975,11.0786659502261));
#48192=CARTESIAN_POINT('Ctrl Pts',(5.7385061804799,-9.05592899315542,11.027846211693));
#48193=CARTESIAN_POINT('Ctrl Pts',(5.73815298599507,-8.84087363714812,10.6364795090074));
#48194=CARTESIAN_POINT('Ctrl Pts',(5.73768885006914,-8.60063920364099,10.2595268562011));
#48195=CARTESIAN_POINT('Ctrl Pts',(5.73711370889943,-8.33732019141297,9.90009894299511));
#48196=CARTESIAN_POINT('Ctrl Pts',(5.73703020872958,-8.29909099934179,9.84791646436043));
#48197=CARTESIAN_POINT('Ctrl Pts',(5.73694436865899,-8.2603751832675,9.79610330116616));
#48198=CARTESIAN_POINT('Ctrl Pts',(5.73685618849917,-8.22117910196827,9.74466890558282));
#48199=CARTESIAN_POINT('Ctrl Pts',(5.73622838502973,-7.94212045794209,9.37847891382779));
#48200=CARTESIAN_POINT('Ctrl Pts',(5.73548196633125,-7.63872140676405,9.03149064911417));
#48201=CARTESIAN_POINT('Ctrl Pts',(5.73461686622672,-7.31395075498618,8.70648064284032));
#48202=CARTESIAN_POINT('Ctrl Pts',(5.73452247697748,-7.27851571361542,8.67101948600494));
#48203=CARTESIAN_POINT('Ctrl Pts',(5.73442667489549,-7.24282621420437,8.63581993734851));
#48204=CARTESIAN_POINT('Ctrl Pts',(5.73432945990849,-7.20688608431088,8.6008855793511));
#48205=CARTESIAN_POINT('Ctrl Pts',(5.73384874333807,-7.02916640840315,8.42813932607534));
#48206=CARTESIAN_POINT('Ctrl Pts',(5.73333347833963,-6.84531868177435,8.26187772439676));
#48207=CARTESIAN_POINT('Ctrl Pts',(5.73278365812027,-6.65588188879718,8.10254858488964));
#48208=CARTESIAN_POINT('Ctrl Pts',(5.99999999997511,-9.67862872910786,17.0348533156911));
#48209=CARTESIAN_POINT('Ctrl Pts',(5.99999999997511,-9.75700380810197,16.9899528681551));
#48210=CARTESIAN_POINT('Ctrl Pts',(5.99999999997511,-9.83522889702052,16.9447896029531));
#48211=CARTESIAN_POINT('Ctrl Pts',(5.99999999997511,-9.91330177297901,16.8993645966839));
#48212=CARTESIAN_POINT('Ctrl Pts',(6.00000263486451,-9.79664482225296,17.2408547729115));
#48213=CARTESIAN_POINT('Ctrl Pts',(6.00000263486451,-9.87548026830557,17.1956905812713));
#48214=CARTESIAN_POINT('Ctrl Pts',(6.00000263486451,-9.95416475310039,17.1502620839818));
#48215=CARTESIAN_POINT('Ctrl Pts',(6.00000263486451,-10.0326962223327,17.1045702551533));
#48216=CARTESIAN_POINT('Ctrl Pts',(5.83074066841747,-9.87940002138524,17.3853070349674));
#48217=CARTESIAN_POINT('Ctrl Pts',(5.83074066841747,-9.95855828585064,17.3399579007926));
#48218=CARTESIAN_POINT('Ctrl Pts',(5.83074066841747,-10.0375649080453,17.2943434175637));
#48219=CARTESIAN_POINT('Ctrl Pts',(5.83074066841747,-10.1164179518766,17.2484644875256));
#48220=CARTESIAN_POINT('Ctrl Pts',(5.59336110043933,-9.87744127562476,17.3818879717683));
#48221=CARTESIAN_POINT('Ctrl Pts',(5.59336110043933,-9.95659189925084,17.3365432150276));
#48222=CARTESIAN_POINT('Ctrl Pts',(5.59336110043933,-10.0355908967271,17.2909331339327));
#48223=CARTESIAN_POINT('Ctrl Pts',(5.59336110043933,-10.1144363291588,17.2450586324221));
#48224=CARTESIAN_POINT('',(5.9999999999561,-9.67863597085289,17.0348513552246));
#48225=CARTESIAN_POINT('',(5.59336167787126,-9.87744147108621,17.381887702864));
#48226=CARTESIAN_POINT('Origin',(5.6,-9.67863108576213,17.0348569102136));
#48227=CARTESIAN_POINT('',(5.59336169565921,-10.1144356128051,17.2450590601813));
#48228=CARTESIAN_POINT('Origin',(5.59336169595271,-7.59798961603702,13.03919108114));
#48229=CARTESIAN_POINT('Origin',(5.6,-9.9133032910197,16.8993688495356));
#48230=CARTESIAN_POINT('Ctrl Pts',(5.99999999999168,-9.67863900758509,17.0348496155183));
#48231=CARTESIAN_POINT('Ctrl Pts',(5.99999999999173,-9.704809124558,17.0198569673818));
#48232=CARTESIAN_POINT('Ctrl Pts',(5.99999999999975,-9.73095807774519,17.00483964126));
#48233=CARTESIAN_POINT('Ctrl Pts',(5.99999999999975,-9.75705556964899,16.9898117786181));
#48234=CARTESIAN_POINT('Ctrl Pts',(5.99999999999975,-9.7831530615528,16.9747839159761));
#48235=CARTESIAN_POINT('Ctrl Pts',(5.99999999999975,-9.80919909217321,16.959745516814));
#48236=CARTESIAN_POINT('Ctrl Pts',(5.99999999999975,-9.83523570648505,16.9446741824461));
#48237=CARTESIAN_POINT('Ctrl Pts',(5.99999999999975,-9.86127232079687,16.9296028480782));
#48238=CARTESIAN_POINT('Ctrl Pts',(5.99999999999975,-9.88729951880012,16.9144985785046));
#48239=CARTESIAN_POINT('Ctrl Pts',(5.99999999999975,-9.9133032909571,16.8993688494793));
#48240=CARTESIAN_POINT('Origin',(5.6,-9.91330329093393,16.8993688493888));
#48241=CARTESIAN_POINT('Origin',(5.600000004206,-9.91330328921746,16.8993688496408));
#48242=CARTESIAN_POINT('Ctrl Pts',(-5.69266253961901,-10.0630749584107,
17.2766486289707));
#48243=CARTESIAN_POINT('Ctrl Pts',(-5.65789849165985,-10.0769812343233,
17.2678653025353));
#48244=CARTESIAN_POINT('Ctrl Pts',(-5.54372221655544,-10.1222489973318,
17.2393099090453));
#48245=CARTESIAN_POINT('Ctrl Pts',(-5.34116379992913,-10.2002037509081,
17.1903133546863));
#48246=CARTESIAN_POINT('Ctrl Pts',(-5.07576041681189,-10.2978306297997,
17.1291591915671));
#48247=CARTESIAN_POINT('Ctrl Pts',(-4.78280587130533,-10.4000145999421,
17.065301068575));
#48248=CARTESIAN_POINT('Ctrl Pts',(-4.45929391303252,-10.5059967628546,
16.9991853363862));
#48249=CARTESIAN_POINT('Ctrl Pts',(-4.10060720841936,-10.6150288379794,
16.9312638063993));
#48250=CARTESIAN_POINT('Ctrl Pts',(-3.70134405537019,-10.7258628654771,
16.862309194946));
#48251=CARTESIAN_POINT('Ctrl Pts',(-3.25667833810229,-10.8361751048301,
16.7937702956078));
#48252=CARTESIAN_POINT('Ctrl Pts',(-2.76261624754771,-10.9424615311872,
16.7278328779196));
#48253=CARTESIAN_POINT('Ctrl Pts',(-2.2145737102596,-11.0402939926339,16.6672547928867));
#48254=CARTESIAN_POINT('Ctrl Pts',(-1.60552241530544,-11.1242420353307,
16.6154077498866));
#48255=CARTESIAN_POINT('Ctrl Pts',(-0.939003279753059,-11.1858223338615,
16.5775146241924));
#48256=CARTESIAN_POINT('Ctrl Pts',(-0.236719809617086,-11.2158434081714,
16.5591722813375));
#48257=CARTESIAN_POINT('Ctrl Pts',(0.464182390050123,-11.2096967358559,
16.5629102770733));
#48258=CARTESIAN_POINT('Ctrl Pts',(1.12883546536813,-11.170862628158,16.5867059961451));
#48259=CARTESIAN_POINT('Ctrl Pts',(1.73414248783393,-11.1079160719739,16.6254820470085));
#48260=CARTESIAN_POINT('Ctrl Pts',(2.27380839700242,-11.0299200690652,16.6736768114977));
#48261=CARTESIAN_POINT('Ctrl Pts',(2.75209280343738,-10.9437380722387,16.7270466558039));
#48262=CARTESIAN_POINT('Ctrl Pts',(3.179567188373,-10.8531427618628,16.7832417082349));
#48263=CARTESIAN_POINT('Ctrl Pts',(3.56235976801865,-10.7611382589682,16.8403865311068));
#48264=CARTESIAN_POINT('Ctrl Pts',(3.90390329062717,-10.6703740483985,16.8968252371846));
#48265=CARTESIAN_POINT('Ctrl Pts',(4.20699758400573,-10.5830036834202,16.9512104351589));
#48266=CARTESIAN_POINT('Ctrl Pts',(4.47553728859529,-10.5002614434386,17.0027677360216));
#48267=CARTESIAN_POINT('Ctrl Pts',(4.7143855071493,-10.4224791464794,17.0512867978894));
#48268=CARTESIAN_POINT('Ctrl Pts',(4.92835317176294,-10.3494685548629,17.0968840833541));
#48269=CARTESIAN_POINT('Ctrl Pts',(5.12118235045995,-10.2809878012257,17.1397122419037));
#48270=CARTESIAN_POINT('Ctrl Pts',(5.29544761530358,-10.2169248336399,17.1798450111274));
#48271=CARTESIAN_POINT('Ctrl Pts',(5.45302040146602,-10.157235748825,17.2173144652497));
#48272=CARTESIAN_POINT('Ctrl Pts',(5.58355164973166,-10.106475377781,17.2492584257149));
#48273=CARTESIAN_POINT('Ctrl Pts',(5.66171355133499,-10.0754541448553,17.2688299523486));
#48274=CARTESIAN_POINT('Ctrl Pts',(5.69263618025467,-10.0630794583498,17.2766460876169));
#48275=CARTESIAN_POINT('Ctrl Pts',(-5.75649720686471,-10.1846648990153,
17.2128720584055));
#48276=CARTESIAN_POINT('Ctrl Pts',(-5.72140107752118,-10.1986648957518,
17.2039351049194));
#48277=CARTESIAN_POINT('Ctrl Pts',(-5.60613425768153,-10.2442342837783,
17.174874254139));
#48278=CARTESIAN_POINT('Ctrl Pts',(-5.40163680541364,-10.3226887670576,
17.1249729790431));
#48279=CARTESIAN_POINT('Ctrl Pts',(-5.13366297613342,-10.4209067331027,
17.0626076171722));
#48280=CARTESIAN_POINT('Ctrl Pts',(-4.83781655802612,-10.5236857216695,
16.9974070511417));
#48281=CARTESIAN_POINT('Ctrl Pts',(-4.51103516393409,-10.6302700871289,
16.9298289327573));
#48282=CARTESIAN_POINT('Ctrl Pts',(-4.14862658342972,-10.7399128406559,
16.860335762575));
#48283=CARTESIAN_POINT('Ctrl Pts',(-3.74510168729925,-10.851361600653,16.7897161027685));
#48284=CARTESIAN_POINT('Ctrl Pts',(-3.29554845890987,-10.9622791410709,
16.7194498781575));
#48285=CARTESIAN_POINT('Ctrl Pts',(-2.79589484443845,-11.069137934311,16.6517739280095));
#48286=CARTESIAN_POINT('Ctrl Pts',(-2.24147534651171,-11.1674782931378,
16.5895170965467));
#48287=CARTESIAN_POINT('Ctrl Pts',(-1.62516077627618,-11.2518315982921,
16.5361473155307));
#48288=CARTESIAN_POINT('Ctrl Pts',(-0.950537739291694,-11.3136699997299,
16.497060155779));
#48289=CARTESIAN_POINT('Ctrl Pts',(-0.239625133653724,-11.3437751162513,
16.4780724300291));
#48290=CARTESIAN_POINT('Ctrl Pts',(0.469884024736187,-11.3376169473577,
16.4819505930994));
#48291=CARTESIAN_POINT('Ctrl Pts',(1.14268886717138,-11.2986518605244,16.5065488874252));
#48292=CARTESIAN_POINT('Ctrl Pts',(1.75532342712682,-11.2354290547684,16.5465228616901));
#48293=CARTESIAN_POINT('Ctrl Pts',(2.30140127461001,-11.1570507323928,16.5961182236132));
#48294=CARTESIAN_POINT('Ctrl Pts',(2.78524362272039,-11.0704204226496,16.650962897641));
#48295=CARTESIAN_POINT('Ctrl Pts',(3.21756803710182,-10.9793385182868,16.7086453435522));
#48296=CARTESIAN_POINT('Ctrl Pts',(3.60459802992447,-10.8868310186806,16.7672452384226));
#48297=CARTESIAN_POINT('Ctrl Pts',(3.94983127105897,-10.7955653931699,16.8250703222752));
#48298=CARTESIAN_POINT('Ctrl Pts',(4.25612453257301,-10.7077085873143,16.88074650159));
#48299=CARTESIAN_POINT('Ctrl Pts',(4.52743794110943,-10.6245017968007,16.9334872976845));
#48300=CARTESIAN_POINT('Ctrl Pts',(4.76870535582295,-10.5462778473736,16.9830829704242));
#48301=CARTESIAN_POINT('Ctrl Pts',(4.98480296232433,-10.4728460664202,17.0296568340121));
#48302=CARTESIAN_POINT('Ctrl Pts',(5.1795233546998,-10.4039615628841,17.0733681030989));
#48303=CARTESIAN_POINT('Ctrl Pts',(5.35547746058191,-10.3395100165887,17.1142950914743));
#48304=CARTESIAN_POINT('Ctrl Pts',(5.51456438643061,-10.2794463026207,17.1524745505953));
#48305=CARTESIAN_POINT('Ctrl Pts',(5.64634415384641,-10.2283555481259,17.1849988667016));
#48306=CARTESIAN_POINT('Ctrl Pts',(5.72525252118978,-10.1971277043966,17.2049169199058));
#48307=CARTESIAN_POINT('Ctrl Pts',(5.75647014480878,-10.184670688155,17.2128713579864));
#48308=CARTESIAN_POINT('Ctrl Pts',(-5.81361907770973,-10.2517346582615,
17.0898712656509));
#48309=CARTESIAN_POINT('Ctrl Pts',(-5.77819645091898,-10.2657916980671,
17.0808138235748));
#48310=CARTESIAN_POINT('Ctrl Pts',(-5.66186163142478,-10.3115390424439,
17.0513590148227));
#48311=CARTESIAN_POINT('Ctrl Pts',(-5.4554863139952,-10.3902563547935,17.0007659322332));
#48312=CARTESIAN_POINT('Ctrl Pts',(-5.18504873353398,-10.4887261479065,
16.9374955140954));
#48313=CARTESIAN_POINT('Ctrl Pts',(-4.88645673350072,-10.5917076816743,
16.8713088940619));
#48314=CARTESIAN_POINT('Ctrl Pts',(-4.55660229647095,-10.6984534721325,
16.802671434488));
#48315=CARTESIAN_POINT('Ctrl Pts',(-4.19073342277236,-10.808221602351,16.7320536351322));
#48316=CARTESIAN_POINT('Ctrl Pts',(-3.78329293118505,-10.9197598564323,
16.6602564585697));
#48317=CARTESIAN_POINT('Ctrl Pts',(-3.32930551518025,-11.0307265753496,
16.5887833721865));
#48318=CARTESIAN_POINT('Ctrl Pts',(-2.82464539782738,-11.1375863407278,
16.5199084631354));
#48319=CARTESIAN_POINT('Ctrl Pts',(-2.26459202118377,-11.235870852726,16.4565105508145));
#48320=CARTESIAN_POINT('Ctrl Pts',(-1.64194486442485,-11.320106064408,16.4021228636622));
#48321=CARTESIAN_POINT('Ctrl Pts',(-0.960344264318984,-11.3817817301385,
16.3622528822177));
#48322=CARTESIAN_POINT('Ctrl Pts',(-0.242081705222581,-11.4117358685156,
16.3428532574355));
#48323=CARTESIAN_POINT('Ctrl Pts',(0.474713498383719,-11.4056180786119,
16.3468196523771));
#48324=CARTESIAN_POINT('Ctrl Pts',(1.15448587132591,-11.3668108697193,16.3719352137425));
#48325=CARTESIAN_POINT('Ctrl Pts',(1.77344785678181,-11.3037311804594,16.4126987703441));
#48326=CARTESIAN_POINT('Ctrl Pts',(2.32512789356553,-11.2254499630162,16.4632331992705));
#48327=CARTESIAN_POINT('Ctrl Pts',(2.8138835116069,-11.1388660220307,16.5190811568224));
#48328=CARTESIAN_POINT('Ctrl Pts',(3.25054531281605,-11.0477872223285,16.5777881968641));
#48329=CARTESIAN_POINT('Ctrl Pts',(3.64140752922088,-10.95524744967,16.6374017121183));
#48330=CARTESIAN_POINT('Ctrl Pts',(3.99001338647845,-10.8639213867097,16.6962025023282));
#48331=CARTESIAN_POINT('Ctrl Pts',(4.2992597178733,-10.7759819686143,16.7527959847812));
#48332=CARTESIAN_POINT('Ctrl Pts',(4.57315676078164,-10.6926745629042,16.8063854846301));
#48333=CARTESIAN_POINT('Ctrl Pts',(4.81669596217747,-10.6143340261694,16.8567603524753));
#48334=CARTESIAN_POINT('Ctrl Pts',(5.03480844630179,-10.5407698820821,16.904047859267));
#48335=CARTESIAN_POINT('Ctrl Pts',(5.23132995987367,-10.4717364368529,16.948411336553));
#48336=CARTESIAN_POINT('Ctrl Pts',(5.40890279612314,-10.4071184861256,16.9899320138223));
#48337=CARTESIAN_POINT('Ctrl Pts',(5.56945053459471,-10.3468710450711,17.0286496664754));
#48338=CARTESIAN_POINT('Ctrl Pts',(5.70244390694285,-10.2955983500078,17.0616208273054));
#48339=CARTESIAN_POINT('Ctrl Pts',(5.7820837103127,-10.2642485670913,17.0818090366983));
#48340=CARTESIAN_POINT('Ctrl Pts',(5.81359156453149,-10.2517426167626,17.0898715756317));
#48341=CARTESIAN_POINT('Ctrl Pts',(-5.84786853141265,-10.2455091741718,
16.9427568836198));
#48342=CARTESIAN_POINT('Ctrl Pts',(-5.81221749608519,-10.2595705697258,
16.9336460964131));
#48343=CARTESIAN_POINT('Ctrl Pts',(-5.69513979505893,-10.3053222964001,
16.9040200007179));
#48344=CARTESIAN_POINT('Ctrl Pts',(-5.4874797057468,-10.3839920616726,16.8531431733464));
#48345=CARTESIAN_POINT('Ctrl Pts',(-5.21538283686595,-10.482304500486,16.7895290278166));
#48346=CARTESIAN_POINT('Ctrl Pts',(-4.91496901490327,-10.58504037815,16.7229906696414));
#48347=CARTESIAN_POINT('Ctrl Pts',(-4.58310798543357,-10.6914629472664,
16.6539954113149));
#48348=CARTESIAN_POINT('Ctrl Pts',(-4.21501992700169,-10.8008376894694,
16.5830168063254));
#48349=CARTESIAN_POINT('Ctrl Pts',(-3.80511818472374,-10.9119170755123,
16.5108612726519));
#48350=CARTESIAN_POINT('Ctrl Pts',(-3.34840461299257,-11.0223652836609,
16.4390415920042));
#48351=CARTESIAN_POINT('Ctrl Pts',(-2.84073935392859,-11.1286567864201,
16.3698447805026));
#48352=CARTESIAN_POINT('Ctrl Pts',(-2.2773886440694,-11.2263399371374,16.3061645413724));
#48353=CARTESIAN_POINT('Ctrl Pts',(-1.65113026598497,-11.3099693976257,
16.2515501009313));
#48354=CARTESIAN_POINT('Ctrl Pts',(-0.965651068761255,-11.3711094017989,
16.2115286076516));
#48355=CARTESIAN_POINT('Ctrl Pts',(-0.243395249204597,-11.4007213303408,
16.1920663039319));
#48356=CARTESIAN_POINT('Ctrl Pts',(0.477305864509668,-11.394684130552,16.1960442118997));
#48357=CARTESIAN_POINT('Ctrl Pts',(1.16089199366367,-11.3562776831491,16.2212463556512));
#48358=CARTESIAN_POINT('Ctrl Pts',(1.78339237472185,-11.2937181300105,16.2621691278305));
#48359=CARTESIAN_POINT('Ctrl Pts',(2.33828065309362,-11.2159838790585,16.3129169306687));
#48360=CARTESIAN_POINT('Ctrl Pts',(2.82991520548475,-11.1299257391801,16.3690143067492));
#48361=CARTESIAN_POINT('Ctrl Pts',(3.26917472852458,-11.0393367756593,16.4279947460898));
#48362=CARTESIAN_POINT('Ctrl Pts',(3.6623796608692,-10.9472425933416,16.4878950535873));
#48363=CARTESIAN_POINT('Ctrl Pts',(4.01308659024824,-10.8563123186887,16.5469861157905));
#48364=CARTESIAN_POINT('Ctrl Pts',(4.3242042468058,-10.7687158078831,16.6038648539006));
#48365=CARTESIAN_POINT('Ctrl Pts',(4.59976346742793,-10.6856986852594,16.6577291719566));
#48366=CARTESIAN_POINT('Ctrl Pts',(4.84478385417697,-10.6075982814546,16.7083662643601));
#48367=CARTESIAN_POINT('Ctrl Pts',(5.06422562949391,-10.5342268808267,16.7559033549902));
#48368=CARTESIAN_POINT('Ctrl Pts',(5.26194812135429,-10.4653404258265,16.8005042877178));
#48369=CARTESIAN_POINT('Ctrl Pts',(5.44061113093055,-10.4008244566688,16.8422507280134));
#48370=CARTESIAN_POINT('Ctrl Pts',(5.6021525906504,-10.3406354448213,16.8811829719989));
#48371=CARTESIAN_POINT('Ctrl Pts',(5.73598086912627,-10.2893801809809,16.9143414007394));
#48372=CARTESIAN_POINT('Ctrl Pts',(5.81612985524781,-10.2580273269292,16.934647159681));
#48373=CARTESIAN_POINT('Ctrl Pts',(5.84784094545612,-10.2455195636508,16.9427570906608));
#48374=CARTESIAN_POINT('',(-5.593361696257,-10.114435612469,17.2450590606623));
#48375=CARTESIAN_POINT('Ctrl Pts',(-5.593361696257,-10.114435612469,17.2450590606623));
#48376=CARTESIAN_POINT('Ctrl Pts',(-5.53985803395109,-10.1354527263307,
17.2318032775356));
#48377=CARTESIAN_POINT('Ctrl Pts',(-5.47932176399903,-10.1588523176192,
17.2170630927394));
#48378=CARTESIAN_POINT('Ctrl Pts',(-5.377968447602,-10.1974253312631,17.1928124140373));
#48379=CARTESIAN_POINT('Ctrl Pts',(-5.34242585689151,-10.2108546235383,
17.1843762811573));
#48380=CARTESIAN_POINT('Ctrl Pts',(-5.28647474295853,-10.2317797500377,
17.1712407072089));
#48381=CARTESIAN_POINT('Ctrl Pts',(-5.25783987902523,-10.2424369641257,
17.164552952931));
#48382=CARTESIAN_POINT('Ctrl Pts',(-5.22821605464172,-10.2533661581861,
17.1576975073026));
#48383=CARTESIAN_POINT('Ctrl Pts',(-5.20824706939711,-10.2607101238115,
17.1530915356416));
#48384=CARTESIAN_POINT('Ctrl Pts',(-5.19619845864606,-10.2651250909784,
17.150322977261));
#48385=CARTESIAN_POINT('Ctrl Pts',(-5.12194820685333,-10.2922550768492,
17.1333118578821));
#48386=CARTESIAN_POINT('Ctrl Pts',(-5.04924772603904,-10.3183350163019,
17.1169723072663));
#48387=CARTESIAN_POINT('Ctrl Pts',(-4.93014661931982,-10.3600705978436,
17.0908496926532));
#48388=CARTESIAN_POINT('Ctrl Pts',(-4.86808346958576,-10.3815871067203,
17.0773880893416));
#48389=CARTESIAN_POINT('Ctrl Pts',(-4.79127941790741,-10.4076995780588,
17.0610606025377));
#48390=CARTESIAN_POINT('Ctrl Pts',(-4.75177813115442,-10.4209888516975,
17.0527533358605));
#48391=CARTESIAN_POINT('Ctrl Pts',(-4.73461345235018,-10.4267320296099,
17.0491636650573));
#48392=CARTESIAN_POINT('Ctrl Pts',(-4.72311798738954,-10.4305711815526,
17.046764169854));
#48393=CARTESIAN_POINT('Ctrl Pts',(-4.71619978461696,-10.4328766746857,
17.0453232896371));
#48394=CARTESIAN_POINT('Ctrl Pts',(-4.56255901740035,-10.483996393471,17.0133757063631));
#48395=CARTESIAN_POINT('Ctrl Pts',(-4.3865990321201,-10.540073840317,16.978360696291));
#48396=CARTESIAN_POINT('Ctrl Pts',(-4.0821965558671,-10.6301690061502,16.9221750041953));
#48397=CARTESIAN_POINT('Ctrl Pts',(-3.97398531406067,-10.6611651185234,
16.9028549809191));
#48398=CARTESIAN_POINT('Ctrl Pts',(-3.80155282676788,-10.7083647078009,
16.8734499833083));
#48399=CARTESIAN_POINT('Ctrl Pts',(-3.71280767697568,-10.7321382323889,
16.8586428785537));
#48400=CARTESIAN_POINT('Ctrl Pts',(-3.60484608312967,-10.7599898039259,
16.8413024969385));
#48401=CARTESIAN_POINT('Ctrl Pts',(-3.54975888976788,-10.7739192136909,
16.8326318138909));
#48402=CARTESIAN_POINT('Ctrl Pts',(-3.52591300766166,-10.7798869881474,
16.8289174252434));
#48403=CARTESIAN_POINT('Ctrl Pts',(-3.50996306737948,-10.7838647560478,
16.8264417203206));
#48404=CARTESIAN_POINT('Ctrl Pts',(-3.50076307772626,-10.7861501079709,
16.8250194080026));
#48405=CARTESIAN_POINT('Ctrl Pts',(-3.27540677250763,-10.8419576514817,
16.7902881080184));
#48406=CARTESIAN_POINT('Ctrl Pts',(-3.02893969710884,-10.8980033528736,
16.7554422862958));
#48407=CARTESIAN_POINT('Ctrl Pts',(-2.6173294603214,-10.978539531806,16.7054362266149));
#48408=CARTESIAN_POINT('Ctrl Pts',(-2.47314111077737,-11.0047751539418,
16.6891576239548));
#48409=CARTESIAN_POINT('Ctrl Pts',(-2.24638118053902,-11.0422394556187,
16.6659313380236));
#48410=CARTESIAN_POINT('Ctrl Pts',(-2.16904830280584,-11.0544116122549,
16.6583885082993));
#48411=CARTESIAN_POINT('Ctrl Pts',(-2.01089007869873,-11.0779494736167,
16.6438097033959));
#48412=CARTESIAN_POINT('Ctrl Pts',(-1.93207851175822,-11.0890500154442,
16.6369377924131));
#48413=CARTESIAN_POINT('Ctrl Pts',(-1.50915171111936,-11.1447334756106,
16.602486057467));
#48414=CARTESIAN_POINT('Ctrl Pts',(-1.15456312141725,-11.179414968581,16.581094880351));
#48415=CARTESIAN_POINT('Ctrl Pts',(-0.598309513077577,-11.2105762749662,
16.5619397177837));
#48416=CARTESIAN_POINT('Ctrl Pts',(-0.408829856333268,-11.2174892628756,
16.557706909214));
#48417=CARTESIAN_POINT('Ctrl Pts',(-0.118517690270173,-11.2219303194708,
16.5549932439991));
#48418=CARTESIAN_POINT('Ctrl Pts',(0.0281615629980323,-11.2226689944669,
16.5545440520554));
#48419=CARTESIAN_POINT('Ctrl Pts',(0.201952906391755,-11.2207893532392,
16.555691075836));
#48420=CARTESIAN_POINT('Ctrl Pts',(0.277006099542097,-11.2193823030147,
16.556551060769));
#48421=CARTESIAN_POINT('Ctrl Pts',(0.32716849249538,-11.2183090012549,16.5572072730465));
#48422=CARTESIAN_POINT('Ctrl Pts',(0.354069491480004,-11.2176578450654,
16.5576054971895));
#48423=CARTESIAN_POINT('Ctrl Pts',(0.75274992570008,-11.2070187026837,16.5641139248419));
#48424=CARTESIAN_POINT('Ctrl Pts',(1.1090999952353,-11.1824152262659,16.5792286931375));
#48425=CARTESIAN_POINT('Ctrl Pts',(1.61530723788318,-11.1300744467122,16.6115515562428));
#48426=CARTESIAN_POINT('Ctrl Pts',(1.86133139379339,-11.1000478603117,16.6301191065388));
#48427=CARTESIAN_POINT('Ctrl Pts',(2.13597051121459,-11.0596761937399,16.6551243093524));
#48428=CARTESIAN_POINT('Ctrl Pts',(2.25101819057925,-11.0413778628387,16.6664651533834));
#48429=CARTESIAN_POINT('Ctrl Pts',(2.32712668803787,-11.0289738997268,16.6741543546353));
#48430=CARTESIAN_POINT('Ctrl Pts',(2.36663752496652,-11.0223702200823,16.6782487949033));
#48431=CARTESIAN_POINT('Ctrl Pts',(2.68805207114582,-10.967472195256,16.7122929768115));
#48432=CARTESIAN_POINT('Ctrl Pts',(2.94928878969231,-10.9142187883781,16.7453687479245));
#48433=CARTESIAN_POINT('Ctrl Pts',(3.3044462170927,-10.8339400967379,16.7952833992631));
#48434=CARTESIAN_POINT('Ctrl Pts',(3.41671575115627,-10.8071002673444,16.8119803720291));
#48435=CARTESIAN_POINT('Ctrl Pts',(3.57594563964679,-10.7673664139986,16.8367102355905));
#48436=CARTESIAN_POINT('Ctrl Pts',(3.65326698074084,-10.7476293920049,16.8489972383141));
#48437=CARTESIAN_POINT('Ctrl Pts',(3.73946140650262,-10.7249543835214,16.8631179578464));
#48438=CARTESIAN_POINT('Ctrl Pts',(3.77554177350454,-10.7153240107291,16.8691161813833));
#48439=CARTESIAN_POINT('Ctrl Pts',(3.79940421790988,-10.7089245228322,16.8731022769998));
#48440=CARTESIAN_POINT('Ctrl Pts',(3.80949575899816,-10.7062073375777,16.8747948247689));
#48441=CARTESIAN_POINT('Ctrl Pts',(4.03872720869192,-10.6441486480237,16.9134538283418));
#48442=CARTESIAN_POINT('Ctrl Pts',(4.23272945063578,-10.5865995058161,16.9493365218276));
#48443=CARTESIAN_POINT('Ctrl Pts',(4.49111530631149,-10.5061357349937,16.9995553690905));
#48444=CARTESIAN_POINT('Ctrl Pts',(4.57180767366338,-10.4802720452767,17.0157062827));
#48445=CARTESIAN_POINT('Ctrl Pts',(4.68469184788119,-10.4432955350863,17.0388094058357));
#48446=CARTESIAN_POINT('Ctrl Pts',(4.73909534078758,-10.4252599357605,17.0500814197759));
#48447=CARTESIAN_POINT('Ctrl Pts',(4.79899854265733,-10.4050714702017,17.0627039233768));
#48448=CARTESIAN_POINT('Ctrl Pts',(4.82390687063271,-10.3966071017749,17.0679970922034));
#48449=CARTESIAN_POINT('Ctrl Pts',(4.84034253976609,-10.3910064469563,17.0714996462197));
#48450=CARTESIAN_POINT('Ctrl Pts',(4.84682231416707,-10.3887937335801,17.0728835010604));
#48451=CARTESIAN_POINT('Ctrl Pts',(4.93413194828082,-10.3588749603406,17.0915962762918));
#48452=CARTESIAN_POINT('Ctrl Pts',(5.00656807785455,-10.3334060550506,17.1075365103738));
#48453=CARTESIAN_POINT('Ctrl Pts',(5.10746362109077,-10.2973256799759,17.1301368266871));
#48454=CARTESIAN_POINT('Ctrl Pts',(5.15597172992778,-10.2798130361603,17.1411114118487));
#48455=CARTESIAN_POINT('Ctrl Pts',(5.20917011370403,-10.2603647102356,17.1533071871831));
#48456=CARTESIAN_POINT('Ctrl Pts',(5.23124204749381,-10.252244452158,17.1584009613105));
#48457=CARTESIAN_POINT('Ctrl Pts',(5.24579503145523,-10.246879052893,17.1617669938564));
#48458=CARTESIAN_POINT('Ctrl Pts',(5.25192688210893,-10.2446143149913,17.1631879272938));
#48459=CARTESIAN_POINT('Ctrl Pts',(5.39096436493034,-10.1931327539252,17.1954922143067));
#48460=CARTESIAN_POINT('Ctrl Pts',(5.50204974451482,-10.1503044424321,17.2224360957622));
#48461=CARTESIAN_POINT('Ctrl Pts',(5.593361696325,-10.1144356126512,17.2450590603724));
#48462=CARTESIAN_POINT('',(-5.7364434626539,-10.2877335026487,16.9337808606147));
#48463=CARTESIAN_POINT('Origin',(-5.599999999997,-9.91330329093349,16.899368849389));
#48464=CARTESIAN_POINT('Ctrl Pts',(-5.73644387761981,-10.2877346861599,
16.933781035207));
#48465=CARTESIAN_POINT('Ctrl Pts',(-5.73644352459171,-10.2877348228402,
16.9337809477574));
#48466=CARTESIAN_POINT('Ctrl Pts',(-5.73644317156337,-10.2877349595205,
16.9337808603077));
#48467=CARTESIAN_POINT('Ctrl Pts',(-5.73644281853479,-10.287735096201,16.933780772858));
#48468=CARTESIAN_POINT('Ctrl Pts',(-5.67992342214019,-10.3096174512513,
16.9197801907616));
#48469=CARTESIAN_POINT('Ctrl Pts',(-5.61717135766351,-10.3335901883676,
16.9044748730959));
#48470=CARTESIAN_POINT('Ctrl Pts',(-5.54808404764097,-10.3594533564795,
16.8879873983964));
#48471=CARTESIAN_POINT('Ctrl Pts',(-5.52951893949722,-10.3664032943593,
16.8835568922627));
#48472=CARTESIAN_POINT('Ctrl Pts',(-5.51049626897038,-10.3734894845319,
16.8790411222862));
#48473=CARTESIAN_POINT('Ctrl Pts',(-5.49101384545753,-10.3807074712925,
16.8744426778672));
#48474=CARTESIAN_POINT('Ctrl Pts',(-5.42195250385916,-10.4062938080743,
16.858142101061));
#48475=CARTESIAN_POINT('Ctrl Pts',(-5.34711523904944,-10.4335394878555,
16.8408006378256));
#48476=CARTESIAN_POINT('Ctrl Pts',(-5.26639250305688,-10.4622194147446,
16.8225604772693));
#48477=CARTESIAN_POINT('Ctrl Pts',(-5.25084323281781,-10.4677439045695,
16.8190469543169));
#48478=CARTESIAN_POINT('Ctrl Pts',(-5.23507554015899,-10.473321484367,16.8155001622011));
#48479=CARTESIAN_POINT('Ctrl Pts',(-5.21908857950422,-10.4789503599815,
16.8119212284932));
#48480=CARTESIAN_POINT('Ctrl Pts',(-5.19131863628201,-10.4887279255611,
16.8057044879875));
#48481=CARTESIAN_POINT('Ctrl Pts',(-5.16288710415933,-10.4986602990195,
16.7993907444015));
#48482=CARTESIAN_POINT('Ctrl Pts',(-5.13378950707246,-10.5087375916594,
16.7929863248323));
#48483=CARTESIAN_POINT('Ctrl Pts',(-5.06602372686519,-10.5322067322924,
16.7780709870609));
#48484=CARTESIAN_POINT('Ctrl Pts',(-4.9946456086541,-10.5564631357043,16.7626630286108));
#48485=CARTESIAN_POINT('Ctrl Pts',(-4.91959547546881,-10.5813691667781,
16.7468506385375));
#48486=CARTESIAN_POINT('Ctrl Pts',(-4.82890430343498,-10.6114658108868,
16.7277428218351));
#48487=CARTESIAN_POINT('Ctrl Pts',(-4.73285110657451,-10.6425123616857,
16.7080435478597));
#48488=CARTESIAN_POINT('Ctrl Pts',(-4.63132572878703,-10.6742283680998,
16.6879338713862));
#48489=CARTESIAN_POINT('Ctrl Pts',(-4.61737858186911,-10.6785853851408,
16.6851712851407));
#48490=CARTESIAN_POINT('Ctrl Pts',(-4.60332815346294,-10.6829549696038,
16.6824009979981));
#48491=CARTESIAN_POINT('Ctrl Pts',(-4.58917414913846,-10.6873363297421,
16.679623522341));
#48492=CARTESIAN_POINT('Ctrl Pts',(-4.55699556861907,-10.6972971822869,
16.6733090390312));
#48493=CARTESIAN_POINT('Ctrl Pts',(-4.52428164451092,-10.7073189284579,
16.6669573814176));
#48494=CARTESIAN_POINT('Ctrl Pts',(-4.49102899371767,-10.7173919554314,
16.6605747653606));
#48495=CARTESIAN_POINT('Ctrl Pts',(-4.4506194813747,-10.729632967745,16.652818439288));
#48496=CARTESIAN_POINT('Ctrl Pts',(-4.40941439087031,-10.741949738429,16.6450163758549));
#48497=CARTESIAN_POINT('Ctrl Pts',(-4.36740760327574,-10.7543241258112,
16.6371803260442));
#48498=CARTESIAN_POINT('Ctrl Pts',(-4.34640420947845,-10.7605113195023,
16.6332623011389));
#48499=CARTESIAN_POINT('Ctrl Pts',(-4.32520038750531,-10.766712903505,16.6293357787708));
#48500=CARTESIAN_POINT('Ctrl Pts',(-4.30379537259903,-10.7729265138952,
16.6254023037402));
#48501=CARTESIAN_POINT('Ctrl Pts',(-4.29309286514589,-10.7760333190904,
16.6234355662249));
#48502=CARTESIAN_POINT('Ctrl Pts',(-4.28234005920634,-10.7791431299959,
16.6214670904874));
#48503=CARTESIAN_POINT('Ctrl Pts',(-4.27153685848547,-10.782255645371,16.6194970717074));
#48504=CARTESIAN_POINT('Ctrl Pts',(-4.26343445794482,-10.7845900319024,
16.6180195576223));
#48505=CARTESIAN_POINT('Ctrl Pts',(-4.25530371031925,-10.7869259396242,
16.6165411755713));
#48506=CARTESIAN_POINT('Ctrl Pts',(-4.24714457491206,-10.7892632399678,
16.6150620087903));
#48507=CARTESIAN_POINT('Ctrl Pts',(-4.24442486310967,-10.7900423400823,
16.6145689531966));
#48508=CARTESIAN_POINT('Ctrl Pts',(-4.24040522469893,-10.7911923588804,
16.6138411817243));
#48509=CARTESIAN_POINT('Ctrl Pts',(-4.23897597541557,-10.7916009996867,
16.6135825836003));
#48510=CARTESIAN_POINT('Ctrl Pts',(-4.2336371240715,-10.7931274461529,16.6126166100938));
#48511=CARTESIAN_POINT('Ctrl Pts',(-4.22827398300798,-10.7946579551636,
16.6116480535346));
#48512=CARTESIAN_POINT('Ctrl Pts',(-4.22288652589826,-10.7961924549587,
16.610676960236));
#48513=CARTESIAN_POINT('Ctrl Pts',(-4.14210580925051,-10.8192010823345,
16.5961161737666));
#48514=CARTESIAN_POINT('Ctrl Pts',(-4.05585859609673,-10.8431104347092,
16.5809827770254));
#48515=CARTESIAN_POINT('Ctrl Pts',(-3.96405497827556,-10.8676567011821,
16.5654470656392));
#48516=CARTESIAN_POINT('Ctrl Pts',(-3.91582512166372,-10.8805523031251,
16.5572852398822));
#48517=CARTESIAN_POINT('Ctrl Pts',(-3.86606160406621,-10.8936229969566,
16.5490128309054));
#48518=CARTESIAN_POINT('Ctrl Pts',(-3.81475097641875,-10.9068256811941,
16.5406577091471));
#48519=CARTESIAN_POINT('Ctrl Pts',(-3.71992040764233,-10.931226436223,16.5252160553442));
#48520=CARTESIAN_POINT('Ctrl Pts',(-3.61980520893666,-10.9560805656995,
16.5094902210422));
#48521=CARTESIAN_POINT('Ctrl Pts',(-3.51432294869463,-10.9810848930795,
16.4936763458349));
#48522=CARTESIAN_POINT('Ctrl Pts',(-3.46379932858498,-10.9930614011174,
16.4861018568013));
#48523=CARTESIAN_POINT('Ctrl Pts',(-3.41204441572844,-11.0050717436431,
16.4785075780106));
#48524=CARTESIAN_POINT('Ctrl Pts',(-3.3590493348187,-11.0170790331133,16.4709174043337));
#48525=CARTESIAN_POINT('Ctrl Pts',(-3.24837455319146,-11.0421550235115,
16.4550661064437));
#48526=CARTESIAN_POINT('Ctrl Pts',(-3.13229029342362,-11.0672207271769,
16.4392307259755));
#48527=CARTESIAN_POINT('Ctrl Pts',(-3.01072492044189,-11.091908246093,16.4236497593753));
#48528=CARTESIAN_POINT('Ctrl Pts',(-2.96856982425133,-11.1004691109929,
16.4182467640185));
#48529=CARTESIAN_POINT('Ctrl Pts',(-2.92501792022023,-11.1091301709932,
16.4127824523541));
#48530=CARTESIAN_POINT('Ctrl Pts',(-2.88137035979109,-11.1176132503999,
16.40743270236));
#48531=CARTESIAN_POINT('Ctrl Pts',(-2.87181730524371,-11.1194699250802,
16.4062618132426));
#48532=CARTESIAN_POINT('Ctrl Pts',(-2.86225971698664,-11.1213182353447,
16.4050963077141));
#48533=CARTESIAN_POINT('Ctrl Pts',(-2.85271131793043,-11.1231555396757,
16.4039378520687));
#48534=CARTESIAN_POINT('Ctrl Pts',(-2.83187965633902,-11.1271639710198,
16.4014104591695));
#48535=CARTESIAN_POINT('Ctrl Pts',(-2.81109169289071,-11.1311198674688,
16.3989167185575));
#48536=CARTESIAN_POINT('Ctrl Pts',(-2.79049042164608,-11.1349974785239,
16.3964728476892));
#48537=CARTESIAN_POINT('Ctrl Pts',(-2.6197081214259,-11.1671424528552,16.3762134237264));
#48538=CARTESIAN_POINT('Ctrl Pts',(-2.45358689126072,-11.1954600801453,
16.3583851565426));
#48539=CARTESIAN_POINT('Ctrl Pts',(-2.29236877426872,-11.2203892871839,
16.3427065217999));
#48540=CARTESIAN_POINT('Ctrl Pts',(-2.13001959335807,-11.2454933909842,
16.3269178898783));
#48541=CARTESIAN_POINT('Ctrl Pts',(-1.9726425728085,-11.2671622061084,16.313308628385));
#48542=CARTESIAN_POINT('Ctrl Pts',(-1.82044574964147,-11.2858528440568,
16.301585213352));
#48543=CARTESIAN_POINT('Ctrl Pts',(-1.76989122124497,-11.2920612284846,
16.2976910997572));
#48544=CARTESIAN_POINT('Ctrl Pts',(-1.71990782410642,-11.2979409267194,
16.2940051090325));
#48545=CARTESIAN_POINT('Ctrl Pts',(-1.67050197927261,-11.3035083877696,
16.2905166532439));
#48546=CARTESIAN_POINT('Ctrl Pts',(-1.52125898565814,-11.3203263281722,
16.279978880097));
#48547=CARTESIAN_POINT('Ctrl Pts',(-1.37728964501425,-11.3342968914911,
16.2712425364788));
#48548=CARTESIAN_POINT('Ctrl Pts',(-1.23874958120321,-11.3458747262349,
16.2640146511266));
#48549=CARTESIAN_POINT('Ctrl Pts',(-1.14911391351094,-11.3533656059064,
16.2593381964482));
#48550=CARTESIAN_POINT('Ctrl Pts',(-1.06175000190717,-11.3598544133719,
16.2552934670782));
#48551=CARTESIAN_POINT('Ctrl Pts',(-0.97669034347626,-11.3654588671785,
16.2518044106196));
#48552=CARTESIAN_POINT('Ctrl Pts',(-0.844793817754813,-11.374149332192,
16.246394155824));
#48553=CARTESIAN_POINT('Ctrl Pts',(-0.718439524656626,-11.3807153182433,
16.2423188713657));
#48554=CARTESIAN_POINT('Ctrl Pts',(-0.597721599451305,-11.3855832138007,
16.2393040884794));
#48555=CARTESIAN_POINT('Ctrl Pts',(-0.480995492516642,-11.3902901410976,
16.2363889963837));
#48556=CARTESIAN_POINT('Ctrl Pts',(-0.369538556420161,-11.3934093157848,
16.2344654664392));
#48557=CARTESIAN_POINT('Ctrl Pts',(-0.263406647333268,-11.3952954750715,
16.2333039464515));
#48558=CARTESIAN_POINT('Ctrl Pts',(-0.255824396465324,-11.3954302256193,
16.233220965414));
#48559=CARTESIAN_POINT('Ctrl Pts',(-0.248269313533065,-11.3955586699161,
16.2331418815967));
#48560=CARTESIAN_POINT('Ctrl Pts',(-0.240741414122083,-11.3956809312728,
16.2330666150223));
#48561=CARTESIAN_POINT('Ctrl Pts',(-0.202201236844007,-11.3963068660922,
16.2326812768341));
#48562=CARTESIAN_POINT('Ctrl Pts',(-0.16437359065513,-11.3967707924497,
16.2323959571174));
#48563=CARTESIAN_POINT('Ctrl Pts',(-0.127260292915424,-11.3970892300575,
16.2321998046146));
#48564=CARTESIAN_POINT('Ctrl Pts',(-0.105079047690209,-11.3972795484366,
16.2320825715194));
#48565=CARTESIAN_POINT('Ctrl Pts',(-0.0831529736488741,-11.3974178860524,
16.2319971868112));
#48566=CARTESIAN_POINT('Ctrl Pts',(-0.0614823788571396,-11.3975076611715,
16.2319414219955));
#48567=CARTESIAN_POINT('Ctrl Pts',(-0.0416874740895889,-11.3975896658395,
16.2318904838821));
#48568=CARTESIAN_POINT('Ctrl Pts',(-0.0231011596291624,-11.3976306161978,
16.2318646679704));
#48569=CARTESIAN_POINT('Ctrl Pts',(-0.00299587767511127,-11.3976346106805,
16.2318611125498));
#48570=CARTESIAN_POINT('Ctrl Pts',(-0.00109077748708527,-11.3976349891825,
16.2318607756517));
#48571=CARTESIAN_POINT('Ctrl Pts',(0.000827961144775839,-11.3976350036236,
16.2318606597262));
#48572=CARTESIAN_POINT('Ctrl Pts',(0.00276265878407632,-11.3976346367673,
16.2318607758997));
#48573=CARTESIAN_POINT('Ctrl Pts',(0.115384922859647,-11.3976132813997,
16.2318675385748));
#48574=CARTESIAN_POINT('Ctrl Pts',(0.233561096316357,-11.3963109193049,
16.2326602932816));
#48575=CARTESIAN_POINT('Ctrl Pts',(0.35723705049632,-11.3933310334508,16.2344974049638));
#48576=CARTESIAN_POINT('Ctrl Pts',(0.4006677928433,-11.3922846000062,16.2351425354151));
#48577=CARTESIAN_POINT('Ctrl Pts',(0.444776498966903,-11.3910309712916,
16.2359166635083));
#48578=CARTESIAN_POINT('Ctrl Pts',(0.489559944492275,-11.3895519147881,
16.2368316586877));
#48579=CARTESIAN_POINT('Ctrl Pts',(0.616826132084439,-11.3853487124614,
16.2394319040858));
#48580=CARTESIAN_POINT('Ctrl Pts',(0.749544200108315,-11.3793270294523,
16.2431685683526));
#48581=CARTESIAN_POINT('Ctrl Pts',(0.887615196589414,-11.3710593224922,
16.2483172112831));
#48582=CARTESIAN_POINT('Ctrl Pts',(0.982140754091479,-11.3653991213669,
16.25184205253));
#48583=CARTESIAN_POINT('Ctrl Pts',(1.07917451717098,-11.3586855955954,16.2560290586568));
#48584=CARTESIAN_POINT('Ctrl Pts',(1.1786736826074,-11.3507739191701,16.260971147143));
#48585=CARTESIAN_POINT('Ctrl Pts',(1.32346414485075,-11.3392609051491,16.2681628383822));
#48586=CARTESIAN_POINT('Ctrl Pts',(1.47347738408703,-11.3252111773464,16.2769531843729));
#48587=CARTESIAN_POINT('Ctrl Pts',(1.62855152014101,-11.3081749134555,16.2876319525441));
#48588=CARTESIAN_POINT('Ctrl Pts',(1.68651040446399,-11.3018076179588,16.2916231370505));
#48589=CARTESIAN_POINT('Ctrl Pts',(1.74517577213395,-11.2950229558544,16.2958782200467));
#48590=CARTESIAN_POINT('Ctrl Pts',(1.80453741563049,-11.2877968278436,16.3004126889885));
#48591=CARTESIAN_POINT('Ctrl Pts',(1.96227499440047,-11.2685953389839,16.3124618188603));
#48592=CARTESIAN_POINT('Ctrl Pts',(2.12493249599591,-11.2462771144358,16.3264834789877));
#48593=CARTESIAN_POINT('Ctrl Pts',(2.29229484978981,-11.2203986250669,16.3427622938076));
#48594=CARTESIAN_POINT('Ctrl Pts',(2.31267645412228,-11.2172471090953,16.3447447489723));
#48595=CARTESIAN_POINT('Ctrl Pts',(2.33312777143621,-11.2140427844923,16.3467606826937));
#48596=CARTESIAN_POINT('Ctrl Pts',(2.35364835962339,-11.2107848446272,16.3488106114143));
#48597=CARTESIAN_POINT('Ctrl Pts',(2.36243285324297,-11.209390179343,16.3496881489197));
#48598=CARTESIAN_POINT('Ctrl Pts',(2.37123004088339,-11.2079856888241,16.3505719161559));
#48599=CARTESIAN_POINT('Ctrl Pts',(2.38003988911401,-11.2065713117456,16.3514619524672));
#48600=CARTESIAN_POINT('Ctrl Pts',(2.44797664373784,-11.195664405518,16.3583254280799));
#48601=CARTESIAN_POINT('Ctrl Pts',(2.51666639180399,-11.1841695738006,16.3655617099716));
#48602=CARTESIAN_POINT('Ctrl Pts',(2.5860930260163,-11.1720587322928,16.3731888014931));
#48603=CARTESIAN_POINT('Ctrl Pts',(2.62080634312245,-11.1660033115389,16.3770023472539));
#48604=CARTESIAN_POINT('Ctrl Pts',(2.65570388132704,-11.1597938857993,16.3809135953313));
#48605=CARTESIAN_POINT('Ctrl Pts',(2.6907834711816,-11.1534269579017,16.3849247863288));
#48606=CARTESIAN_POINT('Ctrl Pts',(2.70832326610889,-11.1502434939528,16.3869303818276));
#48607=CARTESIAN_POINT('Ctrl Pts',(2.72590857392964,-11.147020654347,16.3889609630524));
#48608=CARTESIAN_POINT('Ctrl Pts',(2.74353911819219,-11.1437580021669,16.3910168095262));
#48609=CARTESIAN_POINT('Ctrl Pts',(2.75886397947236,-11.1409220323114,16.3928037970154));
#48610=CARTESIAN_POINT('Ctrl Pts',(2.77564172384628,-11.1377895682063,16.3947777552928));
#48611=CARTESIAN_POINT('Ctrl Pts',(2.79017260044529,-11.1350548322832,16.3965012236886));
#48612=CARTESIAN_POINT('Ctrl Pts',(2.79235882544797,-11.1346433809843,16.3967605259869));
#48613=CARTESIAN_POINT('Ctrl Pts',(2.79449421169261,-11.13424101261,16.3970141065111));
#48614=CARTESIAN_POINT('Ctrl Pts',(2.79656618101408,-11.1338501710236,16.3972604239752));
#48615=CARTESIAN_POINT('Ctrl Pts',(2.81155319855809,-11.1310231264086,16.3990420932875));
#48616=CARTESIAN_POINT('Ctrl Pts',(2.82653415511714,-11.128174494239,16.4008376888312));
#48617=CARTESIAN_POINT('Ctrl Pts',(2.84150896902975,-11.125304341067,16.4026471655719));
#48618=CARTESIAN_POINT('Ctrl Pts',(2.9877609092892,-11.0972729095777,16.4203194709324));
#48619=CARTESIAN_POINT('Ctrl Pts',(3.13342693458816,-11.0671887043866,16.4393158344591));
#48620=CARTESIAN_POINT('Ctrl Pts',(3.27844000038263,-11.0351204092031,16.4595900055763));
#48621=CARTESIAN_POINT('Ctrl Pts',(3.40983090074459,-11.0060645296232,16.4779596716652));
#48622=CARTESIAN_POINT('Ctrl Pts',(3.54068575419653,-10.9753798121356,16.4973783531426));
#48623=CARTESIAN_POINT('Ctrl Pts',(3.67096096203933,-10.9431207808494,16.5178092758489));
#48624=CARTESIAN_POINT('Ctrl Pts',(3.78813583454779,-10.9141056831896,16.5361856868558));
#48625=CARTESIAN_POINT('Ctrl Pts',(3.90484177689973,-10.8838169747423,16.5553809953117));
#48626=CARTESIAN_POINT('Ctrl Pts',(4.02105135355173,-10.8522959606735,16.5753671327589));
#48627=CARTESIAN_POINT('Ctrl Pts',(4.12469412582962,-10.8241836021467,16.593191986371));
#48628=CARTESIAN_POINT('Ctrl Pts',(4.2279420807947,-10.7950910485532,16.6116458779085));
#48629=CARTESIAN_POINT('Ctrl Pts',(4.33077854876954,-10.7650482812465,16.6307081883437));
#48630=CARTESIAN_POINT('Ctrl Pts',(4.4224084153124,-10.7382794237283,16.6476931839933));
#48631=CARTESIAN_POINT('Ctrl Pts',(4.51371159158894,-10.7107561676242,16.6651612189951));
#48632=CARTESIAN_POINT('Ctrl Pts',(4.60467809233216,-10.6824999484507,16.6830973369985));
#48633=CARTESIAN_POINT('Ctrl Pts',(4.68609873252078,-10.6572088859648,16.6991512711214));
#48634=CARTESIAN_POINT('Ctrl Pts',(4.76724964968438,-10.6313306211052,16.7155802031916));
#48635=CARTESIAN_POINT('Ctrl Pts',(4.84812490671061,-10.6048805365343,16.7323732809376));
#48636=CARTESIAN_POINT('Ctrl Pts',(4.92104763596778,-10.5810313096271,16.7475150821126));
#48637=CARTESIAN_POINT('Ctrl Pts',(4.99374625116398,-10.5567171895405,16.7629529363442));
#48638=CARTESIAN_POINT('Ctrl Pts',(5.06621727472414,-10.531949354954,16.7786790259285));
#48639=CARTESIAN_POINT('Ctrl Pts',(5.13211670113978,-10.5094274418827,16.7929790900432));
#48640=CARTESIAN_POINT('Ctrl Pts',(5.19782793957924,-10.4865303686829,16.8075174857058));
#48641=CARTESIAN_POINT('Ctrl Pts',(5.26334901114175,-10.4632663744166,16.8222888789691));
#48642=CARTESIAN_POINT('Ctrl Pts',(5.32293003021169,-10.4421114626764,16.8357211175256));
#48643=CARTESIAN_POINT('Ctrl Pts',(5.38235379937692,-10.420653143382,16.8493460220469));
#48644=CARTESIAN_POINT('Ctrl Pts',(5.44161920194577,-10.398897403341,16.8631608536372));
#48645=CARTESIAN_POINT('Ctrl Pts',(5.49538550613805,-10.3791603276397,16.8756938392485));
#48646=CARTESIAN_POINT('Ctrl Pts',(5.54902146846579,-10.3591784639908,16.8883831411604));
#48647=CARTESIAN_POINT('Ctrl Pts',(5.60252622810342,-10.3389560486812,16.9012292544107));
#48648=CARTESIAN_POINT('Ctrl Pts',(5.64725725918507,-10.3220497118639,16.9119688576716));
#48649=CARTESIAN_POINT('Ctrl Pts',(5.6918965888703,-10.3049752448851,16.9228180609114));
#48650=CARTESIAN_POINT('Ctrl Pts',(5.73644276371282,-10.2877350949215,16.9337809951188));
#48651=CARTESIAN_POINT('Ctrl Pts',(-5.843530256039,-10.2251619023962,17.1593086092344));
#48652=CARTESIAN_POINT('Ctrl Pts',(-3.89568683736,-11.0033634786087,16.6619375925682));
#48653=CARTESIAN_POINT('Ctrl Pts',(0.0001633689883933,-11.7816837467847,
16.1645405511091));
#48654=CARTESIAN_POINT('Ctrl Pts',(3.896013575336,-11.0032981995481,16.6619793101207));
#48655=CARTESIAN_POINT('Ctrl Pts',(5.844020363005,-10.2249660868567,17.1594337605745));
#48656=CARTESIAN_POINT('Ctrl Pts',(-5.843530256039,-10.3258757279616,16.2770651088131));
#48657=CARTESIAN_POINT('Ctrl Pts',(-3.89568683736,-11.0553894883161,15.8346835239237));
#48658=CARTESIAN_POINT('Ctrl Pts',(0.0001633689883933,-11.7876690390135,
15.3921195066591));
#48659=CARTESIAN_POINT('Ctrl Pts',(3.896013575336,-11.0553280707653,15.8347206425293));
#48660=CARTESIAN_POINT('Ctrl Pts',(5.844020363005,-10.3256921635601,16.2771764234008));
#48661=CARTESIAN_POINT('Ctrl Pts',(-5.843530256039,-10.2973078611637,14.4766625890132));
#48662=CARTESIAN_POINT('Ctrl Pts',(-3.89568683736,-10.9728033087721,14.1582357115413));
#48663=CARTESIAN_POINT('Ctrl Pts',(0.0001633689883933,-11.6469739445733,
13.839942885095));
#48664=CARTESIAN_POINT('Ctrl Pts',(3.896013575336,-10.9727467649199,14.1582624073125));
#48665=CARTESIAN_POINT('Ctrl Pts',(5.844020363005,-10.2971378891111,14.4767427134021));
#48666=CARTESIAN_POINT('Ctrl Pts',(-5.843530256039,-9.55783041482319,11.8732201296673));
#48667=CARTESIAN_POINT('Ctrl Pts',(-3.89568683736,-10.276390078785,11.7328262507184));
#48668=CARTESIAN_POINT('Ctrl Pts',(0.0001633689883934,-10.9955719605932,
11.592156207881));
#48669=CARTESIAN_POINT('Ctrl Pts',(3.896013575336,-10.2763297597585,11.7328380489558));
#48670=CARTESIAN_POINT('Ctrl Pts',(5.844020363005,-9.55764960672994,11.8732554563753));
#48671=CARTESIAN_POINT('Ctrl Pts',(-5.843530256039,-8.22112111690873,9.63761418987316));
#48672=CARTESIAN_POINT('Ctrl Pts',(-3.89568683736,-9.09193883951927,9.6131438962805));
#48673=CARTESIAN_POINT('Ctrl Pts',(0.0001633689883931,-9.96185017516567,
9.58955563129661));
#48674=CARTESIAN_POINT('Ctrl Pts',(3.896013575336,-9.09186587855354,9.61314587466688));
#48675=CARTESIAN_POINT('Ctrl Pts',(5.844020363005,-8.22090199675714,9.63762034723964));
#48676=CARTESIAN_POINT('Ctrl Pts',(-5.843530256039,-7.02222755551629,8.43824701706476));
#48677=CARTESIAN_POINT('Ctrl Pts',(-3.89568683736,-8.04148396885872,8.43232683562214));
#48678=CARTESIAN_POINT('Ctrl Pts',(0.0001633689883938,-9.06239246807137,
8.42475648328517));
#48679=CARTESIAN_POINT('Ctrl Pts',(3.896013575336,-8.04139834349921,8.43232747055704));
#48680=CARTESIAN_POINT('Ctrl Pts',(5.844020363005,-7.02197108439241,8.43824850671153));
#48681=CARTESIAN_POINT('Ctrl Pts',(-5.843530256039,-6.40569322596623,7.94881077194426));
#48682=CARTESIAN_POINT('Ctrl Pts',(-3.89568683736,-7.50133620017675,7.9347606008931));
#48683=CARTESIAN_POINT('Ctrl Pts',(0.0001633689883938,-8.59759863808049,
7.92012362694403));
#48684=CARTESIAN_POINT('Ctrl Pts',(3.896013575336,-7.50124425475692,7.93476182852443));
#48685=CARTESIAN_POINT('Ctrl Pts',(5.844020363005,-6.4054175340111,7.94881430732273));
#48686=CARTESIAN_POINT('',(-5.73278765503808,-6.65588329694249,8.10254693662637));
#48687=CARTESIAN_POINT('Ctrl Pts',(-5.73644356953866,-10.287732124489,16.9337807348462));
#48688=CARTESIAN_POINT('Ctrl Pts',(-5.73766037023391,-10.363335737503,16.106357439364));
#48689=CARTESIAN_POINT('Ctrl Pts',(-5.73849618481051,-10.3386824467405,
15.2703428493243));
#48690=CARTESIAN_POINT('Ctrl Pts',(-5.73940756698809,-10.0903333051297,
13.6301040301155));
#48691=CARTESIAN_POINT('Ctrl Pts',(-5.73948313452165,-9.86673834734387,
12.8258710001043));
#48692=CARTESIAN_POINT('Ctrl Pts',(-5.73887402243792,-9.23545641682537,
11.2957057506713));
#48693=CARTESIAN_POINT('Ctrl Pts',(-5.73818934282062,-8.8274551097991,10.5699144763157));
#48694=CARTESIAN_POINT('Ctrl Pts',(-5.73605973643519,-7.85267850870576,
9.23785247231672));
#48695=CARTESIAN_POINT('Ctrl Pts',(-5.73461480966704,-7.28539109135887,
8.63201129368857));
#48696=CARTESIAN_POINT('Ctrl Pts',(-5.732787802167,-6.65588356458119,8.10254661754625));
#48697=CARTESIAN_POINT('Ctrl Pts',(5.73278688077132,-6.65588777852224,8.1025415711865));
#48698=CARTESIAN_POINT('Ctrl Pts',(5.37827627368246,-6.85241150406531,8.10465963825173));
#48699=CARTESIAN_POINT('Ctrl Pts',(5.01472560063427,-7.03192684229805,8.10373394496733));
#48700=CARTESIAN_POINT('Ctrl Pts',(4.64373673482061,-7.19313127670242,8.10099337416535));
#48701=CARTESIAN_POINT('Ctrl Pts',(4.36982161608589,-7.31215461098387,8.09896990703251));
#48702=CARTESIAN_POINT('Ctrl Pts',(4.09185162034693,-7.42119223737612,8.09595885654005));
#48703=CARTESIAN_POINT('Ctrl Pts',(3.81047150082134,-7.5197407633679,8.09246831279417));
#48704=CARTESIAN_POINT('Ctrl Pts',(3.56966521041932,-7.60407900662645,8.08948109076744));
#48705=CARTESIAN_POINT('Ctrl Pts',(3.32636134248185,-7.68073414882858,8.08614294160563));
#48706=CARTESIAN_POINT('Ctrl Pts',(3.08096402298937,-7.74943065949521,8.08277474483814));
#48707=CARTESIAN_POINT('Ctrl Pts',(3.03961664418193,-7.76100544219926,8.08220723208808));
#48708=CARTESIAN_POINT('Ctrl Pts',(2.99820983352411,-7.77235440392396,8.08163886854269));
#48709=CARTESIAN_POINT('Ctrl Pts',(2.95674552410237,-7.78347638387023,8.08107119111927));
#48710=CARTESIAN_POINT('Ctrl Pts',(2.75869139757556,-7.83660048153941,8.07835968192469));
#48711=CARTESIAN_POINT('Ctrl Pts',(2.55931825461576,-7.88459121383307,8.07570997194223));
#48712=CARTESIAN_POINT('Ctrl Pts',(2.3588932505288,-7.92725022184157,8.07321176886139));
#48713=CARTESIAN_POINT('Ctrl Pts',(2.16496913216616,-7.96852556348848,8.07079459625286));
#48714=CARTESIAN_POINT('Ctrl Pts',(1.97006028134188,-8.00480937407901,8.06851927227267));
#48715=CARTESIAN_POINT('Ctrl Pts',(1.77440869148724,-8.03597039260338,8.06646657500283));
#48716=CARTESIAN_POINT('Ctrl Pts',(1.58213144846987,-8.06659398598143,8.06444928001388));
#48717=CARTESIAN_POINT('Ctrl Pts',(1.38913686510899,-8.09226981697469,8.06264700825244));
#48718=CARTESIAN_POINT('Ctrl Pts',(1.19565462876281,-8.11292263500189,8.06113580896464));
#48719=CARTESIAN_POINT('Ctrl Pts',(0.997079151827903,-8.1341191193265,8.05958482875588));
#48720=CARTESIAN_POINT('Ctrl Pts',(0.797990009959274,-8.15002411796531,
8.05834046071093));
#48721=CARTESIAN_POINT('Ctrl Pts',(0.598635511115839,-8.16061444565142,
8.05748407636205));
#48722=CARTESIAN_POINT('Ctrl Pts',(0.41011089037405,-8.17062945671029,8.05667421485644));
#48723=CARTESIAN_POINT('Ctrl Pts',(0.221348960431186,-8.17589182255372,
8.05621132523823));
#48724=CARTESIAN_POINT('Ctrl Pts',(0.0325597200542654,-8.17643387335583,
8.05616342086763));
#48725=CARTESIAN_POINT('Ctrl Pts',(0.0217146407636161,-8.17646501169781,
8.05616066898041));
#48726=CARTESIAN_POINT('Ctrl Pts',(0.010869471349147,-8.17648058744749,
8.05615928631154));
#48727=CARTESIAN_POINT('Ctrl Pts',(2.42516200383473E-5,-8.17648061201097,
8.05615928567218));
#48728=CARTESIAN_POINT('Ctrl Pts',(1.61677462454062E-5,-8.17648061202928,
8.0561592856717));
#48729=CARTESIAN_POINT('Ctrl Pts',(8.08387248017682E-6,-8.17648061203894,
8.05615928567199));
#48730=CARTESIAN_POINT('Ctrl Pts',(-1.25747418398594E-12,-8.17648061203997,
8.05615928567305));
#48731=CARTESIAN_POINT('Ctrl Pts',(-0.189139035705872,-8.17648063611191,
8.0561593104538));
#48732=CARTESIAN_POINT('Ctrl Pts',(-0.378262933363979,-8.17174639869451,
8.05657974522599));
#48733=CARTESIAN_POINT('Ctrl Pts',(-0.567160529186507,-8.16224240278298,
8.05735224853584));
#48734=CARTESIAN_POINT('Ctrl Pts',(-0.75860062666825,-8.15261048610428,
8.05813514949495));
#48735=CARTESIAN_POINT('Ctrl Pts',(-0.949808289415187,-8.13807964420742,
8.05927965741794));
#48736=CARTESIAN_POINT('Ctrl Pts',(-1.14056371176547,-8.11866645037277,
8.06071380372489));
#48737=CARTESIAN_POINT('Ctrl Pts',(-1.33594378375974,-8.09878260559227,
8.06218271928834));
#48738=CARTESIAN_POINT('Ctrl Pts',(-1.53084942143149,-8.07377685544065,
8.06395548156749));
#48739=CARTESIAN_POINT('Ctrl Pts',(-1.72504444158472,-8.04372179853256,
8.06595395922777));
#48740=CARTESIAN_POINT('Ctrl Pts',(-1.93232436125451,-8.01164162584501,
8.06808709471475));
#48741=CARTESIAN_POINT('Ctrl Pts',(-2.13879467403457,-7.97380847538887,
8.07047738209557));
#48742=CARTESIAN_POINT('Ctrl Pts',(-2.34416816538383,-7.93037483013253,
8.07302899030251));
#48743=CARTESIAN_POINT('Ctrl Pts',(-2.5495416567331,-7.8869411848762,8.07558059850945));
#48744=CARTESIAN_POINT('Ctrl Pts',(-2.75381832665157,-7.83790747751988,
8.07829351057817));
#48745=CARTESIAN_POINT('Ctrl Pts',(-2.9567109605982,-7.78348624499325,8.08107129305309));
#48746=CARTESIAN_POINT('Ctrl Pts',(-3.20112609626292,-7.7179275666307,8.08441755588802));
#48747=CARTESIAN_POINT('Ctrl Pts',(-3.44354367002378,-7.64447761155163,
8.08778762182236));
#48748=CARTESIAN_POINT('Ctrl Pts',(-3.68356773262446,-7.56339748666701,
8.09086695035259));
#48749=CARTESIAN_POINT('Ctrl Pts',(-3.97268664594418,-7.46573312191761,
8.09457612896065));
#48750=CARTESIAN_POINT('Ctrl Pts',(-4.25833276625898,-7.35699881171472,
8.09786311779884));
#48751=CARTESIAN_POINT('Ctrl Pts',(-4.53981409580119,-7.23772737140737,
8.10018171708692));
#48752=CARTESIAN_POINT('Ctrl Pts',(-4.90286922679157,-7.08389085068814,
8.10317225066729));
#48753=CARTESIAN_POINT('Ctrl Pts',(-5.25899585877525,-6.91253101039286,
8.10454919088797));
#48754=CARTESIAN_POINT('Ctrl Pts',(-5.60670917229762,-6.72485657966638,
8.10316803578398));
#48755=CARTESIAN_POINT('Ctrl Pts',(-5.64886055313031,-6.70210583618183,
8.10300060591427));
#48756=CARTESIAN_POINT('Ctrl Pts',(-5.69088829700777,-6.6791153198583,8.10279270682702));
#48757=CARTESIAN_POINT('Ctrl Pts',(-5.73278975881162,-6.65588714129348,
8.10254235866335));
#48758=CARTESIAN_POINT('Ctrl Pts',(5.84532977015488,-6.60907067653791,8.11484374494995));
#48759=CARTESIAN_POINT('Ctrl Pts',(5.67447011930324,-6.70782274026614,8.11771294877927));
#48760=CARTESIAN_POINT('Ctrl Pts',(5.16429345659284,-6.98693741106745,8.12376642310323));
#48761=CARTESIAN_POINT('Ctrl Pts',(4.24590849141901,-7.40895819124323,8.12400293957608));
#48762=CARTESIAN_POINT('Ctrl Pts',(3.01583524949797,-7.83057380116843,8.11342583655146));
#48763=CARTESIAN_POINT('Ctrl Pts',(1.5827416161131,-8.13989354095393,8.09845002215385));
#48764=CARTESIAN_POINT('Ctrl Pts',(-0.000549049248834099,-8.25797507006647,
8.09084489616248));
#48765=CARTESIAN_POINT('Ctrl Pts',(-1.58374029028414,-8.13974006353747,
8.09845910700112));
#48766=CARTESIAN_POINT('Ctrl Pts',(-3.01660487844852,-7.83035051488068,
8.11343402782235));
#48767=CARTESIAN_POINT('Ctrl Pts',(-4.24645128469797,-7.40873441263074,
8.1240053767904));
#48768=CARTESIAN_POINT('Ctrl Pts',(-5.16457961062395,-6.98678753483177,
8.12376410532789));
#48769=CARTESIAN_POINT('Ctrl Pts',(-5.67458005472615,-6.70775903594086,
8.11771107859869));
#48770=CARTESIAN_POINT('Ctrl Pts',(-5.84532137971053,-6.60907553644657,
8.11484388868645));
#48771=CARTESIAN_POINT('Ctrl Pts',(5.72603251848978,-6.40553651593773,7.90654864603447));
#48772=CARTESIAN_POINT('Ctrl Pts',(5.55862522162997,-6.50183163678554,7.90984134163062));
#48773=CARTESIAN_POINT('Ctrl Pts',(5.0587624490829,-6.77403023907758,7.91713060303473));
#48774=CARTESIAN_POINT('Ctrl Pts',(4.15898620617447,-7.18569021983348,7.9194064566943));
#48775=CARTESIAN_POINT('Ctrl Pts',(2.95395178893228,-7.59702783009949,7.91108135352791));
#48776=CARTESIAN_POINT('Ctrl Pts',(1.55019345539187,-7.89883073461615,7.89790735180303));
#48777=CARTESIAN_POINT('Ctrl Pts',(-0.000537746227424225,-8.01404387038147,
7.89103083637919));
#48778=CARTESIAN_POINT('Ctrl Pts',(-1.55117163467799,-7.89868098502473,
7.89791550720898));
#48779=CARTESIAN_POINT('Ctrl Pts',(-2.95470571498482,-7.59680997565968,
7.9110882992896));
#48780=CARTESIAN_POINT('Ctrl Pts',(-4.15951798303049,-7.18547191412746,
7.91940776248282));
#48781=CARTESIAN_POINT('Ctrl Pts',(-5.05904281585884,-6.773884064197,7.91712760404102));
#48782=CARTESIAN_POINT('Ctrl Pts',(-5.55873293575348,-6.5017695177983,7.90983919864932));
#48783=CARTESIAN_POINT('Ctrl Pts',(-5.72602429756767,-6.40554125490832,
7.90654881060056));
#48784=CARTESIAN_POINT('Ctrl Pts',(5.72051931939661,-6.40299635313841,7.59202739925403));
#48785=CARTESIAN_POINT('Ctrl Pts',(5.55358754504462,-6.49829579986879,7.59531976312339));
#48786=CARTESIAN_POINT('Ctrl Pts',(5.05509604406011,-6.76774980134388,7.60262461997097));
#48787=CARTESIAN_POINT('Ctrl Pts',(4.15740464799149,-7.17560639151535,7.60498214643902));
#48788=CARTESIAN_POINT('Ctrl Pts',(2.95412552499078,-7.58366289837459,7.59678147557994));
#48789=CARTESIAN_POINT('Ctrl Pts',(1.5509282484579,-7.88347759639777,7.58370271852113));
#48790=CARTESIAN_POINT('Ctrl Pts',(-0.000538111079215552,-7.99805888798782,
7.57685722966631));
#48791=CARTESIAN_POINT('Ctrl Pts',(-1.55190650864731,-7.88332872496391,
7.58371083015612));
#48792=CARTESIAN_POINT('Ctrl Pts',(-2.95487868487001,-7.58344664067807,
7.59678835073835));
#48793=CARTESIAN_POINT('Ctrl Pts',(-4.15793535657866,-7.17538998909926,
7.60498339567978));
#48794=CARTESIAN_POINT('Ctrl Pts',(-5.05537566230955,-6.76760506823289,
7.60262160571017));
#48795=CARTESIAN_POINT('Ctrl Pts',(-5.55369495290555,-6.49823432383111,
7.59531762036264));
#48796=CARTESIAN_POINT('Ctrl Pts',(-5.72051112194647,-6.40300104308615,
7.592027563499));
#48797=CARTESIAN_POINT('Ctrl Pts',(5.83215265165326,-6.6027019454344,7.37631534334889));
#48798=CARTESIAN_POINT('Ctrl Pts',(5.66241585886446,-6.69911246418964,7.37918461663417));
#48799=CARTESIAN_POINT('Ctrl Pts',(5.1554779165898,-6.97177232001094,7.38527716439616));
#48800=CARTESIAN_POINT('Ctrl Pts',(4.24202288280943,-7.38484664402246,7.38570943211202));
#48801=CARTESIAN_POINT('Ctrl Pts',(3.01611906064791,-7.79874165528961,7.37542885317601));
#48802=CARTESIAN_POINT('Ctrl Pts',(1.5844008409398,-8.10338046623929,7.36068016455236));
#48803=CARTESIAN_POINT('Ctrl Pts',(-0.000549882842812274,-8.21997345439349,
7.35314930988947));
#48804=CARTESIAN_POINT('Ctrl Pts',(-1.58539966393749,-8.10322905712485,
7.3606891448144));
#48805=CARTESIAN_POINT('Ctrl Pts',(-3.01688686011958,-7.79852212707958,
7.375436876266));
#48806=CARTESIAN_POINT('Ctrl Pts',(-4.24256314704044,-7.38462734296759,
7.38571173436092));
#48807=CARTESIAN_POINT('Ctrl Pts',(-5.15576230240762,-6.97162583470661,
7.38527480944027));
#48808=CARTESIAN_POINT('Ctrl Pts',(-5.66252507110996,-6.69905027190079,
7.37918274642969));
#48809=CARTESIAN_POINT('Ctrl Pts',(-5.83214431663215,-6.60270669005865,
7.37631548637498));
#48810=CARTESIAN_POINT('',(-5.72001858724455,-6.64700966239077,7.39409314559782));
#48811=CARTESIAN_POINT('Origin',(-5.89877641407823,-6.95919970879477,7.74135818432323));
#48812=CARTESIAN_POINT('Ctrl Pts',(5.72001587221878,-6.64701148325172,7.39409251600456));
#48813=CARTESIAN_POINT('Ctrl Pts',(5.58565290454697,-6.72168733592391,7.39612364502573));
#48814=CARTESIAN_POINT('Ctrl Pts',(5.44860854991134,-6.79466770029646,7.39767007526861));
#48815=CARTESIAN_POINT('Ctrl Pts',(5.30887161640016,-6.86572132858295,7.39878665706021));
#48816=CARTESIAN_POINT('Ctrl Pts',(5.1302758002585,-6.95653397499499,7.40021374459784));
#48817=CARTESIAN_POINT('Ctrl Pts',(4.94728058316614,-7.04420061915497,7.40093782687921));
#48818=CARTESIAN_POINT('Ctrl Pts',(4.75989538421007,-7.12819823960006,7.40110494294509));
#48819=CARTESIAN_POINT('Ctrl Pts',(4.70375696841375,-7.15336294507689,7.40115500896548));
#48820=CARTESIAN_POINT('Ctrl Pts',(4.64722472964256,-7.17819808859506,7.40115523439491));
#48821=CARTESIAN_POINT('Ctrl Pts',(4.59029942585008,-7.20268894371145,7.40110993482223));
#48822=CARTESIAN_POINT('Ctrl Pts',(4.48483666528044,-7.24806196795919,7.40102601049213));
#48823=CARTESIAN_POINT('Ctrl Pts',(4.37802534628683,-7.29225649954224,7.4007825429084));
#48824=CARTESIAN_POINT('Ctrl Pts',(4.26987188704354,-7.33518654413751,7.40039822446667));
#48825=CARTESIAN_POINT('Ctrl Pts',(4.17517571350464,-7.37277490221194,7.40006172588302));
#48826=CARTESIAN_POINT('Ctrl Pts',(4.07945062248494,-7.40939381534365,7.39961727421961));
#48827=CARTESIAN_POINT('Ctrl Pts',(3.98270573857866,-7.4449835306767,7.39907881998807));
#48828=CARTESIAN_POINT('Ctrl Pts',(3.87908664057,-7.48310207557843,7.39850210585561));
#48829=CARTESIAN_POINT('Ctrl Pts',(3.77429690775606,-7.52004090555753,7.3978169305443));
#48830=CARTESIAN_POINT('Ctrl Pts',(3.66834908493288,-7.555728786703,7.39703672613765));
#48831=CARTESIAN_POINT('Ctrl Pts',(3.61537517352129,-7.57357272727574,7.39664662393433));
#48832=CARTESIAN_POINT('Ctrl Pts',(3.56211173626585,-7.59110392169548,7.39623275554249));
#48833=CARTESIAN_POINT('Ctrl Pts',(3.5085606927734,-7.60831352101272,7.39579651070001));
#48834=CARTESIAN_POINT('Ctrl Pts',(3.48178517102717,-7.61691832067135,7.39557838827878));
#48835=CARTESIAN_POINT('Ctrl Pts',(3.45493774755442,-7.6254427209945,7.39535467120603));
#48836=CARTESIAN_POINT('Ctrl Pts',(3.42801867261478,-7.63388561714074,7.39512552136858));
#48837=CARTESIAN_POINT('Ctrl Pts',(3.41455913514496,-7.63810706521386,7.39501094644986));
#48838=CARTESIAN_POINT('Ctrl Pts',(3.40108168479896,-7.64230813720522,7.39489501330451));
#48839=CARTESIAN_POINT('Ctrl Pts',(3.38758635409509,-7.64648869523428,7.39477774108775));
#48840=CARTESIAN_POINT('Ctrl Pts',(3.38083868874316,-7.64857897424881,7.39471910497938));
#48841=CARTESIAN_POINT('Ctrl Pts',(3.37408655330122,-7.65066412477043,7.39466013410096));
#48842=CARTESIAN_POINT('Ctrl Pts',(3.3673299519168,-7.65274412958196,7.39460083077426));
#48843=CARTESIAN_POINT('Ctrl Pts',(3.36057335053239,-7.65482413439349,7.39454152744755));
#48844=CARTESIAN_POINT('Ctrl Pts',(3.35536610976867,-7.65642365019241,7.39449566394423));
#48845=CARTESIAN_POINT('Ctrl Pts',(3.34704675410775,-7.65896868966984,7.39442192574389));
#48846=CARTESIAN_POINT('Ctrl Pts',(3.25218527717916,-7.68798850965474,7.39358112570173));
#48847=CARTESIAN_POINT('Ctrl Pts',(3.15684396878774,-7.71584499185392,7.39270673831623));
#48848=CARTESIAN_POINT('Ctrl Pts',(3.06103807353292,-7.7425135289854,7.39181551956672));
#48849=CARTESIAN_POINT('Ctrl Pts',(2.81798286979236,-7.81017039611988,7.38955453808784));
#48850=CARTESIAN_POINT('Ctrl Pts',(2.57193719390984,-7.87018487448976,7.3871846311959));
#48851=CARTESIAN_POINT('Ctrl Pts',(2.32323865480377,-7.9221824209829,7.38493236667366));
#48852=CARTESIAN_POINT('Ctrl Pts',(2.09715323564706,-7.96945204764125,7.38288489116218));
#48853=CARTESIAN_POINT('Ctrl Pts',(1.86887526640671,-8.01009597774375,7.38093460284897));
#48854=CARTESIAN_POINT('Ctrl Pts',(1.63866316117177,-8.04379642976548,7.37925911418169));
#48855=CARTESIAN_POINT('Ctrl Pts',(1.3874922641473,-8.08056501218121,7.3774310869757));
#48856=CARTESIAN_POINT('Ctrl Pts',(1.1340181123422,-8.10906858519484,7.3759304349394));
#48857=CARTESIAN_POINT('Ctrl Pts',(0.878690129281667,-8.12901172996105,
7.37484825163557));
#48858=CARTESIAN_POINT('Ctrl Pts',(0.631087833523658,-8.14835143714692,
7.37379881292052));
#48859=CARTESIAN_POINT('Ctrl Pts',(0.381741838955915,-8.15964088646107,
7.37314282965446));
#48860=CARTESIAN_POINT('Ctrl Pts',(0.131083074475465,-8.16256657218579,
7.37297043127167));
#48861=CARTESIAN_POINT('Ctrl Pts',(0.0873209945484005,-8.16307736259359,
7.37294033253635));
#48862=CARTESIAN_POINT('Ctrl Pts',(0.0435189611224462,-8.16333310546151,
7.37292499344789));
#48863=CARTESIAN_POINT('Ctrl Pts',(-0.000320651191468663,-8.16333198982214,
7.37292491924339));
#48864=CARTESIAN_POINT('Ctrl Pts',(-0.000413720047120908,-8.16333198745371,
7.37292491908586));
#48865=CARTESIAN_POINT('Ctrl Pts',(-0.000506788725943568,-8.16333198393689,
7.37292491898686));
#48866=CARTESIAN_POINT('Ctrl Pts',(-0.00059985722791523,-8.16333197927169,
7.37292491894639));
#48867=CARTESIAN_POINT('Ctrl Pts',(-0.245377838851759,-8.16331970940542,
7.37292481250585));
#48868=CARTESIAN_POINT('Ctrl Pts',(-0.488931755613559,-8.15536801383923,
7.37332890290789));
#48869=CARTESIAN_POINT('Ctrl Pts',(-0.730901381957773,-8.13972535157021,
7.37411291131156));
#48870=CARTESIAN_POINT('Ctrl Pts',(-0.980216234492042,-8.12360784089019,
7.37492071906206));
#48871=CARTESIAN_POINT('Ctrl Pts',(-1.22784963174372,-8.09932526051673,
7.37613203112047));
#48872=CARTESIAN_POINT('Ctrl Pts',(-1.47341230443435,-8.06709509687875,
7.37772761591521));
#48873=CARTESIAN_POINT('Ctrl Pts',(-1.5289648740937,-8.05980380789328,7.37808857808624));
#48874=CARTESIAN_POINT('Ctrl Pts',(-1.58441147063682,-8.05210556671063,
7.37846923010716));
#48875=CARTESIAN_POINT('Ctrl Pts',(-1.63974758292758,-8.04400252958216,
7.3788693880513));
#48876=CARTESIAN_POINT('Ctrl Pts',(-1.66249593119237,-8.04067141897518,
7.37903389061386));
#48877=CARTESIAN_POINT('Ctrl Pts',(-1.68522560774449,-8.03727189705941,
7.37920168975841));
#48878=CARTESIAN_POINT('Ctrl Pts',(-1.70793637302213,-8.03380422944271,
7.37937266330925));
#48879=CARTESIAN_POINT('Ctrl Pts',(-1.96557893968563,-7.99446522988985,
7.38131227493982));
#48880=CARTESIAN_POINT('Ctrl Pts',(-2.2207883398496,-7.94639486062531,7.38362138273935));
#48881=CARTESIAN_POINT('Ctrl Pts',(-2.47317150971626,-7.89003942090996,
7.3860437156412));
#48882=CARTESIAN_POINT('Ctrl Pts',(-2.49470738438798,-7.88523060704404,
7.38625041348803));
#48883=CARTESIAN_POINT('Ctrl Pts',(-2.51622268786283,-7.88036143821839,
7.38645794280466));
#48884=CARTESIAN_POINT('Ctrl Pts',(-2.53771717974228,-7.87543217538087,
7.38666614818949));
#48885=CARTESIAN_POINT('Ctrl Pts',(-2.67441352405635,-7.84408404145749,
7.3879902509007));
#48886=CARTESIAN_POINT('Ctrl Pts',(-2.81026874009531,-7.81030869440391,
7.38933832380954));
#48887=CARTESIAN_POINT('Ctrl Pts',(-2.94522550202804,-7.77418776918772,
7.39065223289004));
#48888=CARTESIAN_POINT('Ctrl Pts',(-2.98415816211496,-7.76376751544624,
7.39103127262754));
#48889=CARTESIAN_POINT('Ctrl Pts',(-3.02301611308487,-7.75315207789664,
7.39140741316152));
#48890=CARTESIAN_POINT('Ctrl Pts',(-3.06179791533473,-7.7423435060716,7.39177914203255));
#48891=CARTESIAN_POINT('Ctrl Pts',(-3.09023302610688,-7.7344185794487,7.3920516964527));
#48892=CARTESIAN_POINT('Ctrl Pts',(-3.11862720043851,-7.72638982465056,
7.39232187929955));
#48893=CARTESIAN_POINT('Ctrl Pts',(-3.1469800195739,-7.71825813772175,7.39258901229211));
#48894=CARTESIAN_POINT('Ctrl Pts',(-3.18049121270804,-7.70864701122754,
7.39290474616195));
#48895=CARTESIAN_POINT('Ctrl Pts',(-3.21394456796665,-7.69889206224753,
7.39321626893506));
#48896=CARTESIAN_POINT('Ctrl Pts',(-3.24733926263889,-7.68899472537593,
7.39352254275486));
#48897=CARTESIAN_POINT('Ctrl Pts',(-3.26403660997501,-7.68404605694013,
7.39367567966475));
#48898=CARTESIAN_POINT('Ctrl Pts',(-3.28071929216791,-7.6790617915099,7.39382750431879));
#48899=CARTESIAN_POINT('Ctrl Pts',(-3.29738720786073,-7.67404211112049,
7.3939778835142));
#48900=CARTESIAN_POINT('Ctrl Pts',(-3.30572116570713,-7.67153227092578,
7.39405307311191));
#48901=CARTESIAN_POINT('Ctrl Pts',(-3.31405143192873,-7.66901357699015,
7.39412790134407));
#48902=CARTESIAN_POINT('Ctrl Pts',(-3.32237799395243,-7.66648605224175,
7.39420235133963));
#48903=CARTESIAN_POINT('Ctrl Pts',(-3.33070455597614,-7.66395852749335,
7.39427680133519));
#48904=CARTESIAN_POINT('Ctrl Pts',(-3.34058221695287,-7.66094649443477,
7.39436464287305));
#48905=CARTESIAN_POINT('Ctrl Pts',(-3.34734655488609,-7.65887700853551,
7.39442454967878));
#48906=CARTESIAN_POINT('Ctrl Pts',(-3.55061731417835,-7.59668822165921,
7.39622477048512));
#48907=CARTESIAN_POINT('Ctrl Pts',(-3.74985865767998,-7.52978049086197,
7.39778867780606));
#48908=CARTESIAN_POINT('Ctrl Pts',(-3.94497680967061,-7.45869000841953,
7.39896700945016));
#48909=CARTESIAN_POINT('Ctrl Pts',(-4.05474130595829,-7.41869777337358,
7.39962988462632));
#48910=CARTESIAN_POINT('Ctrl Pts',(-4.16320143712219,-7.37738111165568,
7.4001711594348));
#48911=CARTESIAN_POINT('Ctrl Pts',(-4.27034412110881,-7.33483007898457,
7.40056737433741));
#48912=CARTESIAN_POINT('Ctrl Pts',(-4.46806378722257,-7.25630697633785,
7.40129854398276));
#48913=CARTESIAN_POINT('Ctrl Pts',(-4.66129573604226,-7.17358277320544,
7.40153435793695));
#48914=CARTESIAN_POINT('Ctrl Pts',(-4.85000961939606,-7.08719412760397,
7.40114665247284));
#48915=CARTESIAN_POINT('Ctrl Pts',(-5.00616780657878,-7.0157086912887,7.40082583144281));
#48916=CARTESIAN_POINT('Ctrl Pts',(-5.15923278578926,-6.94171325347014,
7.40007853980481));
#48917=CARTESIAN_POINT('Ctrl Pts',(-5.30919876766189,-6.8654904987653,7.39884386351234));
#48918=CARTESIAN_POINT('Ctrl Pts',(-5.44882245660878,-6.79452438991388,
7.39769433575639));
#48919=CARTESIAN_POINT('Ctrl Pts',(-5.58576002074305,-6.72162731991945,
7.39612251961714));
#48920=CARTESIAN_POINT('Ctrl Pts',(-5.72001849314537,-6.64700949805206,
7.39409296279186));
#48921=CARTESIAN_POINT('Ctrl Pts',(-5.71770960723051,-6.68335028393728,
8.11886589750961));
#48922=CARTESIAN_POINT('Ctrl Pts',(-5.721496759235,-6.6813783301849,8.11865841679221));
#48923=CARTESIAN_POINT('Ctrl Pts',(-5.76762296023213,-6.65682357416613,
8.11653387715794));
#48924=CARTESIAN_POINT('Ctrl Pts',(-5.85140117624736,-6.59964365038765,
8.12210181812362));
#48925=CARTESIAN_POINT('Ctrl Pts',(-5.94950294743152,-6.49819378604652,
8.15431025413625));
#48926=CARTESIAN_POINT('Ctrl Pts',(-6.01705132763319,-6.38857658526742,
8.20603404982171));
#48927=CARTESIAN_POINT('Ctrl Pts',(-6.04762129028345,-6.29253909066633,
8.26403289225712));
#48928=CARTESIAN_POINT('Ctrl Pts',(-6.05142104505506,-6.23757718496964,
8.30343898769059));
#48929=CARTESIAN_POINT('Ctrl Pts',(-6.05067380446042,-6.21682915403947,
8.31933149341578));
#48930=CARTESIAN_POINT('Ctrl Pts',(-5.60128072860216,-6.47591277950037,
7.91132944608927));
#48931=CARTESIAN_POINT('Ctrl Pts',(-5.60481509157088,-6.47408697639146,
7.91111770973153));
#48932=CARTESIAN_POINT('Ctrl Pts',(-5.6478672403021,-6.45135276446487,7.90890568143242));
#48933=CARTESIAN_POINT('Ctrl Pts',(-5.72616393016407,-6.39842545287255,
7.91348808972588));
#48934=CARTESIAN_POINT('Ctrl Pts',(-5.81784682618219,-6.30469904603656,
7.94236012175095));
#48935=CARTESIAN_POINT('Ctrl Pts',(-5.88081975256672,-6.2038613583221,7.98919173691161));
#48936=CARTESIAN_POINT('Ctrl Pts',(-5.90915113313628,-6.11618157328609,
8.04174195586025));
#48937=CARTESIAN_POINT('Ctrl Pts',(-5.91263441684734,-6.0665031749669,8.07730621375402));
#48938=CARTESIAN_POINT('Ctrl Pts',(-5.91194835104428,-6.04783961999084,
8.09161437792024));
#48939=CARTESIAN_POINT('Ctrl Pts',(-5.58641801495452,-6.47671513687815,
7.59599440984281));
#48940=CARTESIAN_POINT('Ctrl Pts',(-5.5914396953494,-6.47415139960797,7.59571095040917));
#48941=CARTESIAN_POINT('Ctrl Pts',(-5.65256568591855,-6.44225947547186,
7.59278698559726));
#48942=CARTESIAN_POINT('Ctrl Pts',(-5.76282180736241,-6.36873604510434,
7.59979555478798));
#48943=CARTESIAN_POINT('Ctrl Pts',(-5.89192971011888,-6.23901079269711,
7.64105456714741));
#48944=CARTESIAN_POINT('Ctrl Pts',(-5.98199882366734,-6.09762069092888,
7.70801622004692));
#48945=CARTESIAN_POINT('Ctrl Pts',(-6.02402385939053,-5.97078784562952,
7.78477094726962));
#48946=CARTESIAN_POINT('Ctrl Pts',(-6.02953497026119,-5.89570321681855,
7.83860015188576));
#48947=CARTESIAN_POINT('Ctrl Pts',(-6.02845916294772,-5.86690265917242,
7.86065144746598));
#48948=CARTESIAN_POINT('Ctrl Pts',(-5.68286000291914,-6.68523138736305,
7.37948114797694));
#48949=CARTESIAN_POINT('Ctrl Pts',(-5.69013455487577,-6.68152915634752,
7.37910549395911));
#48950=CARTESIAN_POINT('Ctrl Pts',(-5.77863954741206,-6.63550177846272,
7.37531163500955));
#48951=CARTESIAN_POINT('Ctrl Pts',(-5.93735490739454,-6.53002893406797,
7.38656833635098));
#48952=CARTESIAN_POINT('Ctrl Pts',(-6.1232092755155,-6.34417047782369,7.44782124655894));
#48953=CARTESIAN_POINT('Ctrl Pts',(-6.25429166682148,-6.13946766772676,
7.54674511464773));
#48954=CARTESIAN_POINT('Ctrl Pts',(-6.31696994181551,-5.95162571009039,
7.66149767844862));
#48955=CARTESIAN_POINT('Ctrl Pts',(-6.32552446128076,-5.8370923344154,7.74373065938116));
#48956=CARTESIAN_POINT('Ctrl Pts',(-6.32386337102072,-5.79257548224713,
7.77777893683687));
#48957=CARTESIAN_POINT('',(-5.99998177541742,-6.09546017895638,8.13557732174909));
#48958=CARTESIAN_POINT('',(-5.9999999892078,-6.44014740669715,7.42970580519182));
#48959=CARTESIAN_POINT('Ctrl Pts',(-5.99998177541743,-6.09546017895638,
8.13557732174909));
#48960=CARTESIAN_POINT('Ctrl Pts',(-5.99997919625023,-6.09857637890248,
8.11146641018613));
#48961=CARTESIAN_POINT('Ctrl Pts',(-5.9999803340948,-6.10217504456045,8.08748984324775));
#48962=CARTESIAN_POINT('Ctrl Pts',(-5.99999165905566,-6.10631456424762,
8.06375435735961));
#48963=CARTESIAN_POINT('Ctrl Pts',(-5.99999654214736,-6.10809944054681,
8.05352010087258));
#48964=CARTESIAN_POINT('Ctrl Pts',(-6.00000279747264,-6.10998446451239,
8.04333087802414));
#48965=CARTESIAN_POINT('Ctrl Pts',(-6.00000912002309,-6.11197215444399,
8.03319606361788));
#48966=CARTESIAN_POINT('Ctrl Pts',(-6.00002436664918,-6.11676540447511,
8.00875628621806));
#48967=CARTESIAN_POINT('Ctrl Pts',(-6.00004196881693,-6.12215899095557,
7.98463229462615));
#48968=CARTESIAN_POINT('Ctrl Pts',(-6.00006170986356,-6.12816391594866,
7.96094115182742));
#48969=CARTESIAN_POINT('Ctrl Pts',(-6.00007545974986,-6.13234642143875,
7.9444399740548));
#48970=CARTESIAN_POINT('Ctrl Pts',(-6.00008945445749,-6.13682448373006,
7.92814910102799));
#48971=CARTESIAN_POINT('Ctrl Pts',(-6.00009959581894,-6.14158753793689,
7.91210887700714));
#48972=CARTESIAN_POINT('Ctrl Pts',(-6.00011451576562,-6.14859493188932,
7.88851053780748));
#48973=CARTESIAN_POINT('Ctrl Pts',(-6.00011997332514,-6.15622144650364,
7.86545568059766));
#48974=CARTESIAN_POINT('Ctrl Pts',(-6.00010726677708,-6.16438990455441,
7.84306513481039));
#48975=CARTESIAN_POINT('Ctrl Pts',(-6.00010434192331,-6.16627015914626,
7.83791117230377));
#48976=CARTESIAN_POINT('Ctrl Pts',(-6.0001005134834,-6.16817892723834,7.83279234488374));
#48977=CARTESIAN_POINT('Ctrl Pts',(-6.00009580094069,-6.17011492270688,
7.82770999624424));
#48978=CARTESIAN_POINT('Ctrl Pts',(-6.00009028882588,-6.17237939646811,
7.82176533091493));
#48979=CARTESIAN_POINT('Ctrl Pts',(-6.00008356776384,-6.17468112514248,
7.81587057433163));
#48980=CARTESIAN_POINT('Ctrl Pts',(-6.00007594955505,-6.17701795841215,
7.81002763965109));
#48981=CARTESIAN_POINT('Ctrl Pts',(-6.00006018731391,-6.18185291772643,
7.79793847958003));
#48982=CARTESIAN_POINT('Ctrl Pts',(-6.00004624872792,-6.18690619132347,
7.78588595792757));
#48983=CARTESIAN_POINT('Ctrl Pts',(-6.00002902709531,-6.19209297392499,
7.77409400077235));
#48984=CARTESIAN_POINT('Ctrl Pts',(-6.00001165250664,-6.19732582357634,
7.76219731189432));
#48985=CARTESIAN_POINT('Ctrl Pts',(-5.99999048406169,-6.2026944521499,7.75056633780675));
#48986=CARTESIAN_POINT('Ctrl Pts',(-5.99997290021277,-6.2080602768582,7.7394209205877));
#48987=CARTESIAN_POINT('Ctrl Pts',(-5.99996100005097,-6.21169168784775,
7.73187807437623));
#48988=CARTESIAN_POINT('Ctrl Pts',(-5.99995104039366,-6.21532069069992,
7.7245573798538));
#48989=CARTESIAN_POINT('Ctrl Pts',(-5.99994980987496,-6.21889227642868,
7.71752287032711));
#48990=CARTESIAN_POINT('Ctrl Pts',(-5.99994574570744,-6.23068853981525,
7.69428923309306));
#48991=CARTESIAN_POINT('Ctrl Pts',(-5.99996685472504,-6.24333106014222,
7.67144245233745));
#48992=CARTESIAN_POINT('Ctrl Pts',(-5.99999370870832,-6.25680978298216,
7.6491604065561));
#48993=CARTESIAN_POINT('Ctrl Pts',(-6.0000205626916,-6.2702885058221,7.62687836077475));
#48994=CARTESIAN_POINT('Ctrl Pts',(-6.00005233393426,-6.28460341539502,
7.6051621505297));
#48995=CARTESIAN_POINT('Ctrl Pts',(-6.00007187511467,-6.29968647301357,
7.5841853475513));
#48996=CARTESIAN_POINT('Ctrl Pts',(-6.00009081506142,-6.31430546235059,
7.56385394878445));
#48997=CARTESIAN_POINT('Ctrl Pts',(-6.0000979707467,-6.32964551319117,7.54421778157841));
#48998=CARTESIAN_POINT('Ctrl Pts',(-6.00009088628216,-6.34559950855879,
7.52541402050796));
#48999=CARTESIAN_POINT('Ctrl Pts',(-6.00008371403553,-6.36175118650071,
7.50637726602054));
#49000=CARTESIAN_POINT('Ctrl Pts',(-6.00006153309211,-6.37853141538619,
7.48819446253251));
#49001=CARTESIAN_POINT('Ctrl Pts',(-6.00003861989632,-6.39578674332505,
7.4709791139653));
#49002=CARTESIAN_POINT('Ctrl Pts',(-6.00001938056299,-6.41027538161532,
7.4565240448229));
#49003=CARTESIAN_POINT('Ctrl Pts',(-5.99999990753438,-6.42509792872277,
7.44275065562263));
#49004=CARTESIAN_POINT('Ctrl Pts',(-5.99999991268315,-6.44014731027582,
7.42970569395491));
#49005=CARTESIAN_POINT('Ctrl Pts',(-5.7200186792232,-6.64700982302636,7.39409332428616));
#49006=CARTESIAN_POINT('Ctrl Pts',(-5.7727585915112,-6.61769118315081,7.39330242589221));
#49007=CARTESIAN_POINT('Ctrl Pts',(-5.82234911438972,-6.58559458350196,
7.39611192268061));
#49008=CARTESIAN_POINT('Ctrl Pts',(-5.86897225180668,-6.55106811709225,
7.40211988414016));
#49009=CARTESIAN_POINT('Ctrl Pts',(-5.91559538922365,-6.51654165068254,
7.40812784559972));
#49010=CARTESIAN_POINT('Ctrl Pts',(-5.95925138962019,-6.47958572443316,
7.41733473682809));
#49011=CARTESIAN_POINT('Ctrl Pts',(-6.00000003423404,-6.4401475070892,7.42970592100962));
#49012=CARTESIAN_POINT('Ctrl Pts',(-5.73278525690433,-6.65587891737084,
8.10255215275025));
#49013=CARTESIAN_POINT('Ctrl Pts',(-5.74761527810194,-6.64187384622179,
8.09761318170997));
#49014=CARTESIAN_POINT('Ctrl Pts',(-5.76160423035811,-6.62765828357803,
8.09343190819409));
#49015=CARTESIAN_POINT('Ctrl Pts',(-5.77475087102938,-6.61342753226589,
8.08988767501939));
#49016=CARTESIAN_POINT('Ctrl Pts',(-5.7887746893241,-6.59824726868458,8.08610696150641));
#49017=CARTESIAN_POINT('Ctrl Pts',(-5.80184019226813,-6.58304949672655,
8.08305131863796));
#49018=CARTESIAN_POINT('Ctrl Pts',(-5.81397380607243,-6.56802291292273,
8.08059407916663));
#49019=CARTESIAN_POINT('Ctrl Pts',(-5.81750441135948,-6.5636505192501,8.07987907844146));
#49020=CARTESIAN_POINT('Ctrl Pts',(-5.8209562778395,-6.55929233721068,8.07921485396509));
#49021=CARTESIAN_POINT('Ctrl Pts',(-5.8243304326853,-6.5549523578848,8.07859853892313));
#49022=CARTESIAN_POINT('Ctrl Pts',(-5.83655607327889,-6.53922722674923,
8.07636543269662));
#49023=CARTESIAN_POINT('Ctrl Pts',(-5.84776060403226,-6.52374510228417,
8.07475914495281));
#49024=CARTESIAN_POINT('Ctrl Pts',(-5.85802333829725,-6.50868496127945,
8.07363507561389));
#49025=CARTESIAN_POINT('Ctrl Pts',(-5.86887239880057,-6.49276441060259,
8.072446786416));
#49026=CARTESIAN_POINT('Ctrl Pts',(-5.87866929268569,-6.47731494656851,
8.07179769481914));
#49027=CARTESIAN_POINT('Ctrl Pts',(-5.88751987338268,-6.46249385037828,
8.07154513059879));
#49028=CARTESIAN_POINT('Ctrl Pts',(-5.89170343543667,-6.45548809812959,
8.07142574655783));
#49029=CARTESIAN_POINT('Ctrl Pts',(-5.89567570660684,-6.44862203152409,
8.07139532808666));
#49030=CARTESIAN_POINT('Ctrl Pts',(-5.89944849885801,-6.44190882017283,
8.07144059735559));
#49031=CARTESIAN_POINT('Ctrl Pts',(-5.90199189965474,-6.43738315696036,
8.07147111530808));
#49032=CARTESIAN_POINT('Ctrl Pts',(-5.90444465114991,-6.43292691848639,
8.07153605347808));
#49033=CARTESIAN_POINT('Ctrl Pts',(-5.90681044160722,-6.4285436545057,8.07163160007322));
#49034=CARTESIAN_POINT('Ctrl Pts',(-5.9099114189334,-6.42279825884871,8.07175683847893));
#49035=CARTESIAN_POINT('Ctrl Pts',(-5.91286301230243,-6.41717828879788,
8.07193462478606));
#49036=CARTESIAN_POINT('Ctrl Pts',(-5.91567435331598,-6.4116914615961,8.07215613452247));
#49037=CARTESIAN_POINT('Ctrl Pts',(-5.91815243471818,-6.40685504922909,
8.07235138623883));
#49038=CARTESIAN_POINT('Ctrl Pts',(-5.92052148273777,-6.40212216222683,
8.07258060357384));
#49039=CARTESIAN_POINT('Ctrl Pts',(-5.9227876888036,-6.39749723758926,8.07283826479711));
#49040=CARTESIAN_POINT('Ctrl Pts',(-5.92392079183651,-6.39518477527048,
8.07296709540874));
#49041=CARTESIAN_POINT('Ctrl Pts',(-5.92502817697261,-6.3928993003763,8.07310304094167));
#49042=CARTESIAN_POINT('Ctrl Pts',(-5.92611059719687,-6.39064132398295,
8.07324545116506));
#49043=CARTESIAN_POINT('Ctrl Pts',(-5.92687336413816,-6.38905015845549,
8.07334580572983));
#49044=CARTESIAN_POINT('Ctrl Pts',(-5.92731260918699,-6.38812757179801,
8.07340554956424));
#49045=CARTESIAN_POINT('Ctrl Pts',(-5.92808745871731,-6.38648961137362,
8.07351632282971));
#49046=CARTESIAN_POINT('Ctrl Pts',(-5.92841217545942,-6.38580319013711,
8.07356274466062));
#49047=CARTESIAN_POINT('Ctrl Pts',(-5.9287955171558,-6.38499101376511,8.0736183461214));
#49048=CARTESIAN_POINT('Ctrl Pts',(-5.92928369519092,-6.38395038033944,
8.07369144263413));
#49049=CARTESIAN_POINT('Ctrl Pts',(-5.93927522066233,-6.36265176665552,
8.07518750680789));
#49050=CARTESIAN_POINT('Ctrl Pts',(-5.94805545914819,-6.3416991033364,8.07736409307303));
#49051=CARTESIAN_POINT('Ctrl Pts',(-5.95569861714587,-6.32126287151163,
8.08008397448817));
#49052=CARTESIAN_POINT('Ctrl Pts',(-5.95898627403075,-6.31247235347184,
8.08125391456572));
#49053=CARTESIAN_POINT('Ctrl Pts',(-5.96206359504637,-6.30377677281201,
8.08252469091863));
#49054=CARTESIAN_POINT('Ctrl Pts',(-5.9649368000487,-6.29518712274744,8.0838866415702));
#49055=CARTESIAN_POINT('Ctrl Pts',(-5.97180219870552,-6.27466252670648,
8.08714096354386));
#49056=CARTESIAN_POINT('Ctrl Pts',(-5.9775031506717,-6.2547458399214,8.09091377323926));
#49057=CARTESIAN_POINT('Ctrl Pts',(-5.98217140046649,-6.2355691581327,8.09506266119555));
#49058=CARTESIAN_POINT('Ctrl Pts',(-5.98714021635121,-6.21515778229022,
8.0994786760378));
#49059=CARTESIAN_POINT('Ctrl Pts',(-5.99093857479877,-6.19558460226744,
8.1043210112003));
#49060=CARTESIAN_POINT('Ctrl Pts',(-5.99371838280598,-6.17695926812329,
8.10944787007493));
#49061=CARTESIAN_POINT('Ctrl Pts',(-5.99432005375399,-6.17292793846947,
8.11055754456733));
#49062=CARTESIAN_POINT('Ctrl Pts',(-5.99487399934209,-6.1689408443237,8.1116806455697));
#49063=CARTESIAN_POINT('Ctrl Pts',(-5.99538175392162,-6.16499882795019,
8.11281588855426));
#49064=CARTESIAN_POINT('Ctrl Pts',(-5.99773613140626,-6.14672032300294,
8.11807983028954));
#49065=CARTESIAN_POINT('Ctrl Pts',(-5.99909926553431,-6.1294140853808,8.12360223596205));
#49066=CARTESIAN_POINT('Ctrl Pts',(-5.9996680087375,-6.11314834194608,8.12924566890368));
#49067=CARTESIAN_POINT('Ctrl Pts',(-5.99987919730825,-6.10710846474153,
8.13134121664893));
#49068=CARTESIAN_POINT('Ctrl Pts',(-5.99998064351921,-6.10121167458743,
8.13345376339408));
#49069=CARTESIAN_POINT('Ctrl Pts',(-5.99998177541743,-6.09546017895638,
8.13557732174909));
#49070=CARTESIAN_POINT('Ctrl Pts',(-5.72202497003794,-10.282630745067,17.0373350432682));
#49071=CARTESIAN_POINT('Ctrl Pts',(-5.72274590418673,-10.3310953139824,
16.5600679618479));
#49072=CARTESIAN_POINT('Ctrl Pts',(-5.72404144894786,-10.3627265719337,
15.5563877915237));
#49073=CARTESIAN_POINT('Ctrl Pts',(-5.72530561181376,-10.1890958128617,
14.0392357399793));
#49074=CARTESIAN_POINT('Ctrl Pts',(-5.72546552594784,-9.77722827557498,
12.526135233631));
#49075=CARTESIAN_POINT('Ctrl Pts',(-5.72471376442816,-9.14170929304714,
11.0927040211933));
#49076=CARTESIAN_POINT('Ctrl Pts',(-5.72306595968661,-8.29718472548057,
9.77128759364862));
#49077=CARTESIAN_POINT('Ctrl Pts',(-5.72038925100475,-7.31941610585418,
8.65807787030266));
#49078=CARTESIAN_POINT('Ctrl Pts',(-5.71829764234389,-6.59327312663666,
8.03228833193905));
#49079=CARTESIAN_POINT('Ctrl Pts',(-5.71724205575826,-6.24681302335888,
7.7699843594215));
#49080=CARTESIAN_POINT('Ctrl Pts',(-5.90012992537085,-10.2258728720551,
17.031541509047));
#49081=CARTESIAN_POINT('Ctrl Pts',(-5.90074282924355,-10.2737314129026,
16.5568909290448));
#49082=CARTESIAN_POINT('Ctrl Pts',(-5.90184295197424,-10.3045732220607,
15.5587654379862));
#49083=CARTESIAN_POINT('Ctrl Pts',(-5.90291239263017,-10.1313394179603,
14.0503335166118));
#49084=CARTESIAN_POINT('Ctrl Pts',(-5.90304763810816,-9.72173758915438,
12.5458458210616));
#49085=CARTESIAN_POINT('Ctrl Pts',(-5.90241173218083,-9.09017458373661,
11.1204627334897));
#49086=CARTESIAN_POINT('Ctrl Pts',(-5.90101617902405,-8.25105475095447,
9.80605003590594));
#49087=CARTESIAN_POINT('Ctrl Pts',(-5.89873871610581,-7.27966994646323,
8.69819149816694));
#49088=CARTESIAN_POINT('Ctrl Pts',(-5.89695455612386,-6.55806882134033,
8.07501211881053));
#49089=CARTESIAN_POINT('Ctrl Pts',(-5.89604817364794,-6.21375837300073,
7.8137137118777));
#49090=CARTESIAN_POINT('Ctrl Pts',(-6.00738644022263,-10.07333564029,17.0159713723814));
#49091=CARTESIAN_POINT('Ctrl Pts',(-6.00770911568216,-10.1202651827221,
16.5484242038607));
#49092=CARTESIAN_POINT('Ctrl Pts',(-6.00828666207577,-10.1502618508912,
15.5651526753668));
#49093=CARTESIAN_POINT('Ctrl Pts',(-6.00884297265506,-9.97928411294258,
14.0795877254805));
#49094=CARTESIAN_POINT('Ctrl Pts',(-6.00891327897517,-9.57577907416303,
12.5976732429584));
#49095=CARTESIAN_POINT('Ctrl Pts',(-6.0085825645024,-8.95396889082556,11.1937656628233));
#49096=CARTESIAN_POINT('Ctrl Pts',(-6.00785461825364,-8.12782700841262,
9.89877135043688));
#49097=CARTESIAN_POINT('Ctrl Pts',(-6.00665324994361,-7.17162847329925,
8.80703886908177));
#49098=CARTESIAN_POINT('Ctrl Pts',(-6.00570635763836,-6.46111186998488,
8.19260787275657));
#49099=CARTESIAN_POINT('Ctrl Pts',(-6.00521778050847,-6.1221175179119,7.93494903754976));
#49100=CARTESIAN_POINT('Ctrl Pts',(-5.99965813360087,-9.88724153611006,
16.9969759522918));
#49101=CARTESIAN_POINT('Ctrl Pts',(-5.99962677163889,-9.93329878843649,
16.5381215791427));
#49102=CARTESIAN_POINT('Ctrl Pts',(-5.99956775772523,-9.96274069261619,
15.5729440399789));
#49103=CARTESIAN_POINT('Ctrl Pts',(-5.99950185524724,-9.79495907659826,
14.1150644943025));
#49104=CARTESIAN_POINT('Ctrl Pts',(-5.99949344308302,-9.39889493478627,
12.6604750418897));
#49105=CARTESIAN_POINT('Ctrl Pts',(-5.99953275683936,-8.78865516910236,
11.2827099739524));
#49106=CARTESIAN_POINT('Ctrl Pts',(-5.99961543411688,-7.97776892723705,
10.0116282351798));
#49107=CARTESIAN_POINT('Ctrl Pts',(-5.99972805551254,-7.03936234204484,
8.94022040002282));
#49108=CARTESIAN_POINT('Ctrl Pts',(-5.9998067257913,-6.34195020476634,8.33710919452135));
#49109=CARTESIAN_POINT('Ctrl Pts',(-5.99983414287826,-6.00926938820036,
8.08424026560283));
#49110=CARTESIAN_POINT('',(-5.99999988467789,-9.91329944128341,16.8993703244349));
#49111=CARTESIAN_POINT('Origin',(-5.5999816434089,-9.91328771269701,16.8993697092576));
#49112=CARTESIAN_POINT('Ctrl Pts',(-6.,-9.91329812074841,16.8993691889373));
#49113=CARTESIAN_POINT('Ctrl Pts',(-6.,-9.9568397826802,16.4254094106132));
#49114=CARTESIAN_POINT('Ctrl Pts',(-6.,-9.96638815209589,15.953283891413));
#49115=CARTESIAN_POINT('Ctrl Pts',(-6.,-9.94189523094625,15.4800411552409));
#49116=CARTESIAN_POINT('Ctrl Pts',(-6.,-9.91740229247353,15.0067980843589));
#49117=CARTESIAN_POINT('Ctrl Pts',(-6.,-9.85886801528275,14.5324377949245));
#49118=CARTESIAN_POINT('Ctrl Pts',(-6.,-9.76681036565181,14.0658326091363));
#49119=CARTESIAN_POINT('Ctrl Pts',(-6.,-9.67475271602093,13.5992274233484));
#49120=CARTESIAN_POINT('Ctrl Pts',(-6.,-9.54917169394994,13.1403773412066));
#49121=CARTESIAN_POINT('Ctrl Pts',(-6.,-9.39100128066893,12.6919788380545));
#49122=CARTESIAN_POINT('Ctrl Pts',(-6.,-9.2328308673878,12.2435803349021));
#49123=CARTESIAN_POINT('Ctrl Pts',(-6.,-9.0420710628966,11.8056334107393));
#49124=CARTESIAN_POINT('Ctrl Pts',(-6.,-8.82146085875875,11.3843739927917));
#49125=CARTESIAN_POINT('Ctrl Pts',(-6.,-8.60085065462106,10.9631145748444));
#49126=CARTESIAN_POINT('Ctrl Pts',(-6.,-8.35039005083675,10.5585426631122));
#49127=CARTESIAN_POINT('Ctrl Pts',(-6.,-8.07150643558797,10.1733977819344));
#49128=CARTESIAN_POINT('Ctrl Pts',(-6.,-7.792622820339,9.78825290075636));
#49129=CARTESIAN_POINT('Ctrl Pts',(-6.,-7.48531619362553,9.42253505013277));
#49130=CARTESIAN_POINT('Ctrl Pts',(-6.,-7.15537146437222,9.08219258646993));
#49131=CARTESIAN_POINT('Ctrl Pts',(-6.,-6.82542673511914,8.74185012280732));
#49132=CARTESIAN_POINT('Ctrl Pts',(-6.,-6.47284390332625,8.42688304610544));
#49133=CARTESIAN_POINT('Ctrl Pts',(-6.,-6.09546018099012,8.13557732069495));
#49134=CARTESIAN_POINT('Origin',(-5.599999999997,-9.91330329093349,16.899368849389));
#49135=CARTESIAN_POINT('Origin',(-5.6,-9.91330329095944,16.8993688494318));
#49136=CARTESIAN_POINT('Ctrl Pts',(-6.05065185023871,-4.09650686474605,
9.54349128053163));
#49137=CARTESIAN_POINT('Ctrl Pts',(-6.05140972708256,-4.0723989783453,9.55349643619757));
#49138=CARTESIAN_POINT('Ctrl Pts',(-6.04764687447984,-4.01080955139642,
9.58136929929187));
#49139=CARTESIAN_POINT('Ctrl Pts',(-6.01714389005373,-3.91255120432432,
9.63551943372867));
#49140=CARTESIAN_POINT('Ctrl Pts',(-5.94963119729813,-3.81288206008285,
9.7046038434688));
#49141=CARTESIAN_POINT('Ctrl Pts',(-5.85153569778131,-3.73419722399452,
9.77638417842136));
#49142=CARTESIAN_POINT('Ctrl Pts',(-5.76771443214422,-3.70073548179553,
9.82315751901543));
#49143=CARTESIAN_POINT('Ctrl Pts',(-5.72154537198058,-3.69027983102092,
9.84550922441198));
#49144=CARTESIAN_POINT('Ctrl Pts',(-5.71772607536419,-3.68946642963374,
9.84733621716733));
#49145=CARTESIAN_POINT('Ctrl Pts',(-5.91196388319657,-3.98378410118069,
9.28331121105742));
#49146=CARTESIAN_POINT('Ctrl Pts',(-5.91265976607569,-3.96208637840918,
9.29230536714295));
#49147=CARTESIAN_POINT('Ctrl Pts',(-5.9092102407762,-3.90646135451234,9.31752641532043));
#49148=CARTESIAN_POINT('Ctrl Pts',(-5.88093976386008,-3.81709709389408,
9.36716626955956));
#49149=CARTESIAN_POINT('Ctrl Pts',(-5.81799703832602,-3.72605533285352,
9.43109497458473));
#49150=CARTESIAN_POINT('Ctrl Pts',(-5.72631526514141,-3.65412316410241,
9.49785603133131));
#49151=CARTESIAN_POINT('Ctrl Pts',(-5.64797404963314,-3.62364364874167,
9.54143888864739));
#49152=CARTESIAN_POINT('Ctrl Pts',(-5.60487947444387,-3.61417509384371,
9.56225713834693));
#49153=CARTESIAN_POINT('Ctrl Pts',(-5.60131491490269,-3.61343908276037,
9.56395871527821));
#49154=CARTESIAN_POINT('Ctrl Pts',(-6.02845826007556,-3.8743345208937,9.01112785386752));
#49155=CARTESIAN_POINT('Ctrl Pts',(-6.02954938100152,-3.84087507001535,
9.02502218021019));
#49156=CARTESIAN_POINT('Ctrl Pts',(-6.02409034814899,-3.75673115811109,
9.06310624745352));
#49157=CARTESIAN_POINT('Ctrl Pts',(-5.98215261412372,-3.62681858681912,
9.13454712209158));
#49158=CARTESIAN_POINT('Ctrl Pts',(-5.89212705130421,-3.49804224901997,
9.22353624826158));
#49159=CARTESIAN_POINT('Ctrl Pts',(-5.76302541892318,-3.39736161362055,
9.31528648438854));
#49160=CARTESIAN_POINT('Ctrl Pts',(-5.65271278399101,-3.35446635079726,
9.37550371289834));
#49161=CARTESIAN_POINT('Ctrl Pts',(-5.59153007899971,-3.34102908670047,
9.40461648632458));
#49162=CARTESIAN_POINT('Ctrl Pts',(-5.58646575731296,-3.33998355022766,
9.40699867986969));
#49163=CARTESIAN_POINT('Ctrl Pts',(-6.32381572581365,-3.83986183316476,
8.90525672846377));
#49164=CARTESIAN_POINT('Ctrl Pts',(-6.32550038395361,-3.78817424015326,
8.92675213935762));
#49165=CARTESIAN_POINT('Ctrl Pts',(-6.31702550013207,-3.65971176909999,
8.98478709160199));
#49166=CARTESIAN_POINT('Ctrl Pts',(-6.25447459339337,-3.46637296327811,
9.09005775360737));
#49167=CARTESIAN_POINT('Ctrl Pts',(-6.12345620551607,-3.27822119685277,
9.21790555729585));
#49168=CARTESIAN_POINT('Ctrl Pts',(-5.937616052749,-3.13212498574318,9.34828223376809));
#49169=CARTESIAN_POINT('Ctrl Pts',(-5.77882600926223,-3.06954994799304,
9.43406098886272));
#49170=CARTESIAN_POINT('Ctrl Pts',(-5.69024266127033,-3.04978819593502,
9.47586226246463));
#49171=CARTESIAN_POINT('Ctrl Pts',(-5.68290661947263,-3.0482489982039,9.47928521174236));
#49172=CARTESIAN_POINT('',(-5.73278765687023,-3.68906981625968,9.8154374870846));
#49173=CARTESIAN_POINT('',(-5.72001858491459,-3.0799676634134,9.45352580072754));
#49174=CARTESIAN_POINT('Origin',(-5.89876013871265,-3.22462655825293,9.8975005542016));
#49175=CARTESIAN_POINT('',(-5.99999998735835,-3.21424020897419,9.29218418198714));
#49176=CARTESIAN_POINT('Ctrl Pts',(-6.00000003704887,-3.21424025835317,
9.29218432473884));
#49177=CARTESIAN_POINT('Ctrl Pts',(-5.95925151906109,-3.18380747703174,
9.32015314616885));
#49178=CARTESIAN_POINT('Ctrl Pts',(-5.91559554599687,-3.15735621311459,
9.34755442745742));
#49179=CARTESIAN_POINT('Ctrl Pts',(-5.86897240659433,-3.13488993689926,
9.37445124425472));
#49180=CARTESIAN_POINT('Ctrl Pts',(-5.82234926719179,-3.11242366068393,
9.40134806105201));
#49181=CARTESIAN_POINT('Ctrl Pts',(-5.77275871290704,-3.09394217276707,
9.42773982822785));
#49182=CARTESIAN_POINT('Ctrl Pts',(-5.72001867761081,-3.07996773842414,
9.4535260309681));
#49183=CARTESIAN_POINT('',(-5.9999819026388,-3.99788652873932,9.3466120296767));
#49184=CARTESIAN_POINT('Ctrl Pts',(-5.9999819026388,-3.99788652873932,9.3466120296767));
#49185=CARTESIAN_POINT('Ctrl Pts',(-5.99997892502811,-3.97149634512734,
9.33560737629572));
#49186=CARTESIAN_POINT('Ctrl Pts',(-5.99997956294922,-3.94521403643915,
9.32545947544754));
#49187=CARTESIAN_POINT('Ctrl Pts',(-5.99997436131157,-3.91905572044391,
9.31619701323493));
#49188=CARTESIAN_POINT('Ctrl Pts',(-5.99997319891254,-3.91321017653617,
9.31412715026793));
#49189=CARTESIAN_POINT('Ctrl Pts',(-5.99997162450337,-3.90737086585166,
9.31210133530766));
#49190=CARTESIAN_POINT('Ctrl Pts',(-5.99996939181339,-3.9015380218435,9.31011961125842));
#49191=CARTESIAN_POINT('Ctrl Pts',(-5.99995605169999,-3.86668732551883,
9.29827899578118));
#49192=CARTESIAN_POINT('Ctrl Pts',(-5.9999237641423,-3.83206867179135,9.28801549899031));
#49193=CARTESIAN_POINT('Ctrl Pts',(-5.99990968741117,-3.79764807109586,
9.27929778340875));
#49194=CARTESIAN_POINT('Ctrl Pts',(-5.99990773622705,-3.79287701104904,
9.27808941563857));
#49195=CARTESIAN_POINT('Ctrl Pts',(-5.99990608047017,-3.78810971834973,
9.27691070715592));
#49196=CARTESIAN_POINT('Ctrl Pts',(-5.99990478331505,-3.78334605668427,
9.27576155474841));
#49197=CARTESIAN_POINT('Ctrl Pts',(-5.9998966985705,-3.75365570796689,9.26859926277548));
#49198=CARTESIAN_POINT('Ctrl Pts',(-5.99989594461753,-3.7241164923183,9.26260358244453));
#49199=CARTESIAN_POINT('Ctrl Pts',(-5.99989840958442,-3.6947401127648,9.25777487994042));
#49200=CARTESIAN_POINT('Ctrl Pts',(-5.99990034204125,-3.67170995132592,
9.25398932842249));
#49201=CARTESIAN_POINT('Ctrl Pts',(-5.99990481363489,-3.64877936325589,
9.25092042635753));
#49202=CARTESIAN_POINT('Ctrl Pts',(-5.99991482494673,-3.6259412251828,9.24857354713652));
#49203=CARTESIAN_POINT('Ctrl Pts',(-5.99991833498322,-3.61793401302479,
9.24775071474223));
#49204=CARTESIAN_POINT('Ctrl Pts',(-5.99992684845666,-3.60967244995355,
9.2469869642076));
#49205=CARTESIAN_POINT('Ctrl Pts',(-5.99993256981174,-3.60152318467775,
9.24633123599943));
#49206=CARTESIAN_POINT('Ctrl Pts',(-5.99993836287564,-3.5932717802666,9.24566728919611));
#49207=CARTESIAN_POINT('Ctrl Pts',(-5.99994102036157,-3.58513584158189,
9.24511412208589));
#49208=CARTESIAN_POINT('Ctrl Pts',(-5.99994630413676,-3.57751190194319,
9.24467223767596));
#49209=CARTESIAN_POINT('Ctrl Pts',(-5.9999470916684,-3.57637557546306,9.24460637606373));
#49210=CARTESIAN_POINT('Ctrl Pts',(-5.99994796568151,-3.57525064535877,
9.24454289917138));
#49211=CARTESIAN_POINT('Ctrl Pts',(-5.99994897476035,-3.57413844577657,
9.24448172000767));
#49212=CARTESIAN_POINT('Ctrl Pts',(-5.99997574698198,-3.54463029204011,
9.24285855434815));
#49213=CARTESIAN_POINT('Ctrl Pts',(-5.99996192315438,-3.51552751704015,
9.24253165400506));
#49214=CARTESIAN_POINT('Ctrl Pts',(-5.99993728662295,-3.48683842875823,
9.24342037855321));
#49215=CARTESIAN_POINT('Ctrl Pts',(-5.99991766072212,-3.46398418878542,
9.24412835239656));
#49216=CARTESIAN_POINT('Ctrl Pts',(-5.99989194171101,-3.4413915343842,9.24560839507766));
#49217=CARTESIAN_POINT('Ctrl Pts',(-5.99987472933798,-3.41905659359933,
9.24784231031407));
#49218=CARTESIAN_POINT('Ctrl Pts',(-5.99985423749428,-3.39246618014718,
9.25050185306036));
#49219=CARTESIAN_POINT('Ctrl Pts',(-5.99984743226518,-3.36623979468742,
9.25422906380482));
#49220=CARTESIAN_POINT('Ctrl Pts',(-5.99986332455246,-3.34036723982923,
9.25903426734148));
#49221=CARTESIAN_POINT('Ctrl Pts',(-5.99987871369806,-3.3153137968055,9.26368734059547));
#49222=CARTESIAN_POINT('Ctrl Pts',(-5.99991598087344,-3.29059138763699,
9.26935207733197));
#49223=CARTESIAN_POINT('Ctrl Pts',(-5.9999511570379,-3.26620847344255,9.27606922917231));
#49224=CARTESIAN_POINT('Ctrl Pts',(-5.99997640640063,-3.24870647871583,
9.28089078393606));
#49225=CARTESIAN_POINT('Ctrl Pts',(-5.99999991134788,-3.23137977939288,
9.28625531048571));
#49226=CARTESIAN_POINT('Ctrl Pts',(-5.99999991596861,-3.21424016050503,
9.29218404186559));
#49227=CARTESIAN_POINT('Ctrl Pts',(-5.9999819026388,-3.99788652873932,9.3466120296767));
#49228=CARTESIAN_POINT('Ctrl Pts',(-5.99997890799539,-3.98519840970855,
9.35715883213799));
#49229=CARTESIAN_POINT('Ctrl Pts',(-5.99925065772263,-3.97204910714977,
9.36865876554123));
#49230=CARTESIAN_POINT('Ctrl Pts',(-5.99760763522023,-3.95857513389356,
9.38112775869376));
#49231=CARTESIAN_POINT('Ctrl Pts',(-5.99700537153811,-3.95363613595889,
9.38569837274031));
#49232=CARTESIAN_POINT('Ctrl Pts',(-5.99628002057492,-3.94865393845055,
9.39039903246601));
#49233=CARTESIAN_POINT('Ctrl Pts',(-5.99542154791787,-3.94363681618573,
9.39522993978368));
#49234=CARTESIAN_POINT('Ctrl Pts',(-5.99297223882613,-3.92932246024583,
9.40901300569433));
#49235=CARTESIAN_POINT('Ctrl Pts',(-5.98943905602187,-3.914720076621,9.42385864009363));
#49236=CARTESIAN_POINT('Ctrl Pts',(-5.9846468393107,-3.9000247023485,9.43974507481651));
#49237=CARTESIAN_POINT('Ctrl Pts',(-5.98035089087139,-3.88685113905285,
9.453986355745));
#49238=CARTESIAN_POINT('Ctrl Pts',(-5.97504355429744,-3.87360276162521,
9.46906389698083));
#49239=CARTESIAN_POINT('Ctrl Pts',(-5.96859394862519,-3.86046121996682,
9.48493891553766));
#49240=CARTESIAN_POINT('Ctrl Pts',(-5.96744221923484,-3.85811448738632,
9.48777377496526));
#49241=CARTESIAN_POINT('Ctrl Pts',(-5.96625404234337,-3.85577127801689,
9.49063400267137));
#49242=CARTESIAN_POINT('Ctrl Pts',(-5.96502863926366,-3.85343278478609,
9.4935192944734));
#49243=CARTESIAN_POINT('Ctrl Pts',(-5.96428753790516,-3.85201850687305,
9.49526426615625));
#49244=CARTESIAN_POINT('Ctrl Pts',(-5.96353282016883,-3.85060595508656,
9.49701840481362));
#49245=CARTESIAN_POINT('Ctrl Pts',(-5.96276437690544,-3.84919536030071,
9.49878163548696));
#49246=CARTESIAN_POINT('Ctrl Pts',(-5.95818717714525,-3.84079321218763,
9.50928424433221));
#49247=CARTESIAN_POINT('Ctrl Pts',(-5.9531229036142,-3.83245988915338,9.52010985266385));
#49248=CARTESIAN_POINT('Ctrl Pts',(-5.94754929030463,-3.82424849588493,
9.53123959893818));
#49249=CARTESIAN_POINT('Ctrl Pts',(-5.94476248364985,-3.8201427992507,9.53680447207534));
#49250=CARTESIAN_POINT('Ctrl Pts',(-5.9418483004759,-3.81606760916532,9.54244537605093));
#49251=CARTESIAN_POINT('Ctrl Pts',(-5.93880412211886,-3.81203044433949,
9.54815934825822));
#49252=CARTESIAN_POINT('Ctrl Pts',(-5.93728203294034,-3.81001186192658,
9.55101633436187));
#49253=CARTESIAN_POINT('Ctrl Pts',(-5.93572744171875,-3.80800278761671,
9.55389158725416));
#49254=CARTESIAN_POINT('Ctrl Pts',(-5.93414001676768,-3.80600420060038,
9.55678471395299));
#49255=CARTESIAN_POINT('Ctrl Pts',(-5.9330828181687,-3.80467317490864,9.55871148818607));
#49256=CARTESIAN_POINT('Ctrl Pts',(-5.93173984860894,-3.80301368285739,
9.56113444361949));
#49257=CARTESIAN_POINT('Ctrl Pts',(-5.93065095545942,-3.80169303734624,
9.56307800903407));
#49258=CARTESIAN_POINT('Ctrl Pts',(-5.93010483305342,-3.8010306820873,9.56405278293258));
#49259=CARTESIAN_POINT('Ctrl Pts',(-5.92962351987447,-3.80045288203708,
9.56490693977137));
#49260=CARTESIAN_POINT('Ctrl Pts',(-5.9292789011774,-3.8000409048946,9.56551731005603));
#49261=CARTESIAN_POINT('Ctrl Pts',(-5.92342174375046,-3.79303891980119,
9.57589119538594));
#49262=CARTESIAN_POINT('Ctrl Pts',(-5.91678402183533,-3.78574286570555,
9.58714431119368));
#49263=CARTESIAN_POINT('Ctrl Pts',(-5.90922580100395,-3.77831400530464,
9.59925023020935));
#49264=CARTESIAN_POINT('Ctrl Pts',(-5.90846944344672,-3.7775705929552,9.60046167977386));
#49265=CARTESIAN_POINT('Ctrl Pts',(-5.90770386059727,-3.77682588945337,
9.6016816510152));
#49266=CARTESIAN_POINT('Ctrl Pts',(-5.90692890757045,-3.77608008326768,
9.60291010453114));
#49267=CARTESIAN_POINT('Ctrl Pts',(-5.89944452236005,-3.76887719406945,
9.61477433243671));
#49268=CARTESIAN_POINT('Ctrl Pts',(-5.89108567512895,-3.76156832512594,
9.62743169755309));
#49269=CARTESIAN_POINT('Ctrl Pts',(-5.88173640074049,-3.75432835168381,
9.64083690558411));
#49270=CARTESIAN_POINT('Ctrl Pts',(-5.87446311616708,-3.74869600151837,
9.65126551092012));
#49271=CARTESIAN_POINT('Ctrl Pts',(-5.86659043159745,-3.74310588829126,
9.66214639069774));
#49272=CARTESIAN_POINT('Ctrl Pts',(-5.85806724378538,-3.73765871579024,
9.67344653471384));
#49273=CARTESIAN_POINT('Ctrl Pts',(-5.8478284059915,-3.73111507074768,9.68702130793009));
#49274=CARTESIAN_POINT('Ctrl Pts',(-5.83665027253931,-3.72477596569576,
9.70120218750934));
#49275=CARTESIAN_POINT('Ctrl Pts',(-5.82445357514376,-3.71885526366353,
9.71590692351583));
#49276=CARTESIAN_POINT('Ctrl Pts',(-5.81280378431398,-3.71320004914077,
9.72995229113683));
#49277=CARTESIAN_POINT('Ctrl Pts',(-5.80022371135754,-3.70792744423552,
9.74447553567856));
#49278=CARTESIAN_POINT('Ctrl Pts',(-5.78667898044615,-3.7032345474092,9.75938338006826));
#49279=CARTESIAN_POINT('Ctrl Pts',(-5.77401425347524,-3.69884654905051,
9.77332265875571));
#49280=CARTESIAN_POINT('Ctrl Pts',(-5.76050602541545,-3.69496516378039,
9.78759826545324));
#49281=CARTESIAN_POINT('Ctrl Pts',(-5.7461478796606,-3.69178345774301,9.80210884284901));
#49282=CARTESIAN_POINT('Ctrl Pts',(-5.74177234227017,-3.69081385665596,
9.80653083264045));
#49283=CARTESIAN_POINT('Ctrl Pts',(-5.73731804252361,-3.68990948299376,
9.81097445275041));
#49284=CARTESIAN_POINT('Ctrl Pts',(-5.73278526695723,-3.68907650035723,
9.81543630638497));
#49285=CARTESIAN_POINT('Ctrl Pts',(-5.71725994859976,-3.6056013506233,9.29487895543824));
#49286=CARTESIAN_POINT('Ctrl Pts',(-5.71831552981187,-3.65953318106983,
9.72607761564714));
#49287=CARTESIAN_POINT('Ctrl Pts',(-5.72040712143486,-3.83841163152394,
10.6678343458936));
#49288=CARTESIAN_POINT('Ctrl Pts',(-5.72308379499235,-4.31359623826603,
12.0712142427945));
#49289=CARTESIAN_POINT('Ctrl Pts',(-5.72473157500471,-5.03571382654535,
13.4633014200608));
#49290=CARTESIAN_POINT('Ctrl Pts',(-5.72548332476085,-5.95934168456203,
14.7303918598931));
#49291=CARTESIAN_POINT('Ctrl Pts',(-5.72532341316257,-7.06379075900272,
15.8436292363302));
#49292=CARTESIAN_POINT('Ctrl Pts',(-5.72405927318753,-8.29086345814456,
16.7525709110518));
#49293=CARTESIAN_POINT('Ctrl Pts',(-5.72276375585025,-9.17588690984407,
17.2270157661404));
#49294=CARTESIAN_POINT('Ctrl Pts',(-5.72204284054482,-9.61344026743877,
17.4236765036483));
#49295=CARTESIAN_POINT('Ctrl Pts',(-5.89606004581221,-3.66000666368765,
9.28811662465129));
#49296=CARTESIAN_POINT('Ctrl Pts',(-5.89696640239014,-3.71414242649981,
9.71695052206151));
#49297=CARTESIAN_POINT('Ctrl Pts',(-5.89875049980449,-3.89303118636646,
10.6534681301436));
#49298=CARTESIAN_POINT('Ctrl Pts',(-5.90102787762071,-4.36677305776408,
12.0486428922503));
#49299=CARTESIAN_POINT('Ctrl Pts',(-5.90242337426096,-5.08552707877001,
13.4325466081192));
#49300=CARTESIAN_POINT('Ctrl Pts',(-5.90305925435447,-6.00416238723668,
14.6921861279471));
#49301=CARTESIAN_POINT('Ctrl Pts',(-5.90292401435139,-7.10228463864252,
15.7991541637147));
#49302=CARTESIAN_POINT('Ctrl Pts',(-5.90185462016992,-8.322003131726,16.7033913584665));
#49303=CARTESIAN_POINT('Ctrl Pts',(-5.9007545479202,-9.20182078389947,17.1757422132168));
#49304=CARTESIAN_POINT('Ctrl Pts',(-5.90014167552026,-9.63680489054994,
17.3716193894984));
#49305=CARTESIAN_POINT('Ctrl Pts',(-6.00522116866736,-3.81082060828096,
9.26937107071129));
#49306=CARTESIAN_POINT('Ctrl Pts',(-6.00570971511597,-3.86446243505639,
9.69178123092468));
#49307=CARTESIAN_POINT('Ctrl Pts',(-6.00665653329783,-4.0413170753428,10.6143250570191));
#49308=CARTESIAN_POINT('Ctrl Pts',(-6.00785781208216,-4.50868641018821,
11.9882849936967));
#49309=CARTESIAN_POINT('Ctrl Pts',(-6.00858569914826,-5.21711252467402,
13.3512402332268));
#49310=CARTESIAN_POINT('Ctrl Pts',(-6.00891638705178,-6.12202585435753,
14.5916957615917));
#49311=CARTESIAN_POINT('Ctrl Pts',(-6.00884608631042,-7.20364747990103,
15.6820971652467));
#49312=CARTESIAN_POINT('Ctrl Pts',(-6.00828982250237,-8.40469064056497,
16.5729470365179));
#49313=CARTESIAN_POINT('Ctrl Pts',(-6.00771232487956,-9.27122184737554,
17.0386027958654));
#49314=CARTESIAN_POINT('Ctrl Pts',(-6.00738967876521,-9.69958976605554,
17.2317327933039));
#49315=CARTESIAN_POINT('Ctrl Pts',(-5.99983391384278,-3.99652936940203,
9.2462882081223));
#49316=CARTESIAN_POINT('Ctrl Pts',(-5.99980647643591,-4.04917980289419,
9.66083589408773));
#49317=CARTESIAN_POINT('Ctrl Pts',(-5.99972775387988,-4.22278351469519,
10.5663714352303));
#49318=CARTESIAN_POINT('Ctrl Pts',(-5.99961507899353,-4.68144737106702,
11.9147614578706));
#49319=CARTESIAN_POINT('Ctrl Pts',(-5.99953236569529,-5.37679277436971,
13.2525493754026));
#49320=CARTESIAN_POINT('Ctrl Pts',(-5.99949303625143,-6.26485171777721,
14.4699140490644));
#49321=CARTESIAN_POINT('Ctrl Pts',(-5.99950145165108,-7.3265302039202,15.5402095165816));
#49322=CARTESIAN_POINT('Ctrl Pts',(-5.99956738117704,-8.50519588233293,
16.4144492818083));
#49323=CARTESIAN_POINT('Ctrl Pts',(-5.99962642146639,-9.35578039726249,
16.871538751569));
#49324=CARTESIAN_POINT('Ctrl Pts',(-5.99965779862438,-9.77618429775514,
17.061077895889));
#49325=CARTESIAN_POINT('',(-5.99999997114735,-9.6786333714602,17.0348538902214));
#49326=CARTESIAN_POINT('Ctrl Pts',(-6.,-3.99788652685643,9.34661203088348));
#49327=CARTESIAN_POINT('Ctrl Pts',(-6.,-4.06147282781482,9.81908884364364));
#49328=CARTESIAN_POINT('Ctrl Pts',(-6.,-4.1579509296493,10.2819181094307));
#49329=CARTESIAN_POINT('Ctrl Pts',(-6.,-4.2877238070187,10.7378298887288));
#49330=CARTESIAN_POINT('Ctrl Pts',(-6.,-4.4174966843882,11.1937416680273));
#49331=CARTESIAN_POINT('Ctrl Pts',(-6.,-4.58056433729266,11.6427359608369));
#49332=CARTESIAN_POINT('Ctrl Pts',(-6.,-4.77466778468932,12.0768286890182));
#49333=CARTESIAN_POINT('Ctrl Pts',(-6.,-4.96877123208584,12.5109214171993));
#49334=CARTESIAN_POINT('Ctrl Pts',(-6.,-5.19391047397451,12.930112580752));
#49335=CARTESIAN_POINT('Ctrl Pts',(-6.,-5.4484267220564,13.3317963060837));
#49336=CARTESIAN_POINT('Ctrl Pts',(-6.,-5.70294297013846,13.7334800314157));
#49337=CARTESIAN_POINT('Ctrl Pts',(-6.,-5.98683622441378,14.1176563185267));
#49338=CARTESIAN_POINT('Ctrl Pts',(-6.,-6.29607551364862,14.4788351606867));
#49339=CARTESIAN_POINT('Ctrl Pts',(-6.,-6.60531480288324,14.8400140028466));
#49340=CARTESIAN_POINT('Ctrl Pts',(-6.,-6.93990012707735,15.1781954000556));
#49341=CARTESIAN_POINT('Ctrl Pts',(-6.,-7.29796324417597,15.4912222498826));
#49342=CARTESIAN_POINT('Ctrl Pts',(-6.,-7.65602636127484,15.8042490997097));
#49343=CARTESIAN_POINT('Ctrl Pts',(-6.,-8.03756727127826,16.0921214021547));
#49344=CARTESIAN_POINT('Ctrl Pts',(-6.,-8.43516131244481,16.3499544329203));
#49345=CARTESIAN_POINT('Ctrl Pts',(-6.,-8.83275507233027,16.6077872812798));
#49346=CARTESIAN_POINT('Ctrl Pts',(-6.,-9.24640194066504,16.835580900463));
#49347=CARTESIAN_POINT('Ctrl Pts',(-6.,-9.67863396568507,17.0348526013128));
#49348=CARTESIAN_POINT('',(-5.73644356943,-9.52121843706026,17.376327826582));
#49349=CARTESIAN_POINT('Origin',(-5.5999816381906,-9.67863859075266,17.0348433699664));
#49350=CARTESIAN_POINT('Ctrl Pts',(-5.732787802673,-3.68906940981089,9.81543755867358));
#49351=CARTESIAN_POINT('Ctrl Pts',(-5.73461480969872,-3.83284536601077,
10.625338537734));
#49352=CARTESIAN_POINT('Ctrl Pts',(-5.73605973938219,-4.07387518713724,
11.4195438346354));
#49353=CARTESIAN_POINT('Ctrl Pts',(-5.73818934988832,-4.74008577639406,
12.9297554589891));
#49354=CARTESIAN_POINT('Ctrl Pts',(-5.73887403071099,-5.1646384849479,13.6459905214075));
#49355=CARTESIAN_POINT('Ctrl Pts',(-5.73948314349551,-6.17415916067771,
14.9577795955828));
#49356=CARTESIAN_POINT('Ctrl Pts',(-5.73940757545737,-6.75884790405006,
15.5535353523723));
#49357=CARTESIAN_POINT('Ctrl Pts',(-5.7384961905607,-8.05516230656083,16.588732228699));
#49358=CARTESIAN_POINT('Ctrl Pts',(-5.7376603737696,-8.76684603821501,17.0280903673069));
#49359=CARTESIAN_POINT('Ctrl Pts',(-5.73644356975375,-9.52121823634833,
17.3763277339283));
#49360=CARTESIAN_POINT('Origin',(-5.599999999997,-9.67863108576248,17.0348569102134));
#49361=CARTESIAN_POINT('',(-5.593361696257,-9.87744142979155,17.381887715825));
#49362=CARTESIAN_POINT('Origin',(-5.599999999997,-9.67863108576248,17.0348569102134));
#49363=CARTESIAN_POINT('Origin',(-5.6,-9.67863108578652,17.0348569102573));
#49364=CARTESIAN_POINT('Ctrl Pts',(-5.59335880963398,-9.87743876208659,
17.3818891889333));
#49365=CARTESIAN_POINT('Ctrl Pts',(-5.59335897597999,-9.88085962292803,
17.3799294167645));
#49366=CARTESIAN_POINT('Ctrl Pts',(-5.5933624992167,-9.95658496857357,17.3365326542547));
#49367=CARTESIAN_POINT('Ctrl Pts',(-5.5933624992167,-10.0355852075694,17.2909218450052));
#49368=CARTESIAN_POINT('Ctrl Pts',(-5.59335897597999,-10.111030579166,17.2470401532232));
#49369=CARTESIAN_POINT('Ctrl Pts',(-5.59335880963397,-10.1144382220706,
17.2450574869161));
#49370=CARTESIAN_POINT('Ctrl Pts',(-5.83074004398886,-9.87939819740596,
17.385309456316));
#49371=CARTESIAN_POINT('Ctrl Pts',(-5.83074021197022,-9.88281933951952,
17.3833494092227));
#49372=CARTESIAN_POINT('Ctrl Pts',(-5.83074376984249,-9.95855095781758,
17.3399466417508));
#49373=CARTESIAN_POINT('Ctrl Pts',(-5.83074376984249,-10.0375588128472,
17.2943314353822));
#49374=CARTESIAN_POINT('Ctrl Pts',(-5.83074021197022,-10.1130125212199,
17.2504473138048));
#49375=CARTESIAN_POINT('Ctrl Pts',(-5.83074004398886,-10.1164205428521,
17.2484645413711));
#49376=CARTESIAN_POINT('Ctrl Pts',(-6.00000347487355,-9.79664251977179,
17.2408563364913));
#49377=CARTESIAN_POINT('Ctrl Pts',(-6.00000357360975,-9.80004967468002,
17.2389042213875));
#49378=CARTESIAN_POINT('Ctrl Pts',(-6.00000566485702,-9.87547170311362,
17.1956771557035));
#49379=CARTESIAN_POINT('Ctrl Pts',(-6.00000566485702,-9.95415740029349,
17.1502479472561));
#49380=CARTESIAN_POINT('Ctrl Pts',(-6.00000357360975,-10.0293041515222,
17.1065440874721));
#49381=CARTESIAN_POINT('Ctrl Pts',(-6.00000347487355,-10.0326983102474,
17.1045694623189));
#49382=CARTESIAN_POINT('Ctrl Pts',(-5.9999999999769,-9.67862555751017,17.0348533300724));
#49383=CARTESIAN_POINT('Ctrl Pts',(-5.99999999996752,-9.68201281532632,
17.0329126138071));
#49384=CARTESIAN_POINT('Ctrl Pts',(-5.99999999976693,-9.75699439866858,
16.9899379593132));
#49385=CARTESIAN_POINT('Ctrl Pts',(-5.99999999976693,-9.83522068189101,
16.9447739936378));
#49386=CARTESIAN_POINT('Ctrl Pts',(-5.99999999996752,-9.90992861607117,
16.9013253648968));
#49387=CARTESIAN_POINT('Ctrl Pts',(-5.9999999999769,-9.91330295456663,16.8993622717116));
#49388=CARTESIAN_POINT('Origin',(-5.47626352655027,8.61291825284854,-14.9180130853614));
#49389=CARTESIAN_POINT('Ctrl Pts',(-6.00000000001697,-9.67863488304264,
17.0348530242413));
#49390=CARTESIAN_POINT('Ctrl Pts',(-6.00000000001004,-9.68201982098913,
17.0329138284059));
#49391=CARTESIAN_POINT('Ctrl Pts',(-6.00000000000346,-9.68540450273407,
17.0309741411426));
#49392=CARTESIAN_POINT('Ctrl Pts',(-5.9999999999973,-9.68878892524755,17.0290339619835));
#49393=CARTESIAN_POINT('Ctrl Pts',(-5.99999999993208,-9.72458345042307,
17.0085141269222));
#49394=CARTESIAN_POINT('Ctrl Pts',(-5.99999999990817,-9.7603489793636,16.9879392663706));
#49395=CARTESIAN_POINT('Ctrl Pts',(-5.99999999990817,-9.79608195797147,
16.9673088199809));
#49396=CARTESIAN_POINT('Ctrl Pts',(-5.99999999990817,-9.831814800472,16.9466784521728));
#49397=CARTESIAN_POINT('Ctrl Pts',(-5.99999999993208,-9.86751509309911,
16.9259924988281));
#49398=CARTESIAN_POINT('Ctrl Pts',(-5.9999999999973,-9.90318155030038,16.9052543226624));
#49399=CARTESIAN_POINT('Ctrl Pts',(-6.00000000000346,-9.90655401250716,
16.9032934125848));
#49400=CARTESIAN_POINT('Ctrl Pts',(-6.00000000001004,-9.90992617222899,
16.9013320356057));
#49401=CARTESIAN_POINT('Ctrl Pts',(-6.00000000001698,-9.91329802836123,
16.8993701945871));
#49402=CARTESIAN_POINT('Ctrl Pts',(-5.67781977236543,-9.69011180339119,
17.4901976785338));
#49403=CARTESIAN_POINT('Ctrl Pts',(-3.78521318157696,-8.87555307108949,
17.9135245439353));
#49404=CARTESIAN_POINT('Ctrl Pts',(-2.07656941121626E-10,-8.05543132883925,
18.3265320501275));
#49405=CARTESIAN_POINT('Ctrl Pts',(3.7852131811623,-8.87555307099925,17.9135245439808));
#49406=CARTESIAN_POINT('Ctrl Pts',(5.67781977174296,-9.69011180312139,17.4901976786702));
#49407=CARTESIAN_POINT('Ctrl Pts',(-5.67781977236543,-9.88673787499947,
17.3789566884608));
#49408=CARTESIAN_POINT('Ctrl Pts',(-3.78521318157695,-9.58451115251288,
17.5169843132773));
#49409=CARTESIAN_POINT('Ctrl Pts',(-2.07656941988987E-10,-9.35257726240188,
17.7858656006621));
#49410=CARTESIAN_POINT('Ctrl Pts',(3.7852131811623,-9.58451115249001,17.5169843133112));
#49411=CARTESIAN_POINT('Ctrl Pts',(5.67781977174296,-9.8867378749017,17.3789566885092));
#49412=CARTESIAN_POINT('Ctrl Pts',(-5.67781977236543,-10.0824830841441,
17.2660356209527));
#49413=CARTESIAN_POINT('Ctrl Pts',(-3.78521318157695,-10.2888890425898,
17.110829551969));
#49414=CARTESIAN_POINT('Ctrl Pts',(-2.07657304546194E-10,-10.5762499707986,
17.0878203717078));
#49415=CARTESIAN_POINT('Ctrl Pts',(3.7852131811623,-10.288889042623,17.1108295519695));
#49416=CARTESIAN_POINT('Ctrl Pts',(5.67781977174296,-10.0824830842147,17.2660356209062));
#49417=CARTESIAN_POINT('Ctrl Pts',(-5.67781977236543,-10.2772191551084,
17.1515085360387));
#49418=CARTESIAN_POINT('Ctrl Pts',(-3.78521318157695,-10.9872896356005,
16.6958668793638));
#49419=CARTESIAN_POINT('Ctrl Pts',(-2.07657334903855E-10,-11.70142277916,
16.2468455207269));
#49420=CARTESIAN_POINT('Ctrl Pts',(3.7852131811623,-10.9872896356761,16.6958668793104));
#49421=CARTESIAN_POINT('Ctrl Pts',(5.67781977174296,-10.2772191553433,17.1515085358907));
#49422=CARTESIAN_POINT('Ctrl Pts',(-5.59336169625718,-9.87744142978604,
17.3818877158154));
#49423=CARTESIAN_POINT('Ctrl Pts',(-5.58014016745599,-9.87200777751962,
17.3847476856453));
#49424=CARTESIAN_POINT('Ctrl Pts',(-5.56083360318078,-9.86407899010458,
17.3889225081183));
#49425=CARTESIAN_POINT('Ctrl Pts',(-5.53540587426982,-9.8537223397616,17.3943811899286));
#49426=CARTESIAN_POINT('Ctrl Pts',(-5.51006695575766,-9.84340186167177,
17.3998208064221));
#49427=CARTESIAN_POINT('Ctrl Pts',(-5.47864940081797,-9.83067044535519,
17.4065354728229));
#49428=CARTESIAN_POINT('Ctrl Pts',(-5.44109677171059,-9.81563689153736,
17.414473213808));
#49429=CARTESIAN_POINT('Ctrl Pts',(-5.41364441246037,-9.80464680828554,
17.420275995726));
#49430=CARTESIAN_POINT('Ctrl Pts',(-5.38291292798052,-9.79242729789503,
17.4267319893631));
#49431=CARTESIAN_POINT('Ctrl Pts',(-5.34887409163183,-9.77903528808476,
17.4338128228857));
#49432=CARTESIAN_POINT('Ctrl Pts',(-5.3032827335042,-9.76109813215338,17.4432968373704));
#49433=CARTESIAN_POINT('Ctrl Pts',(-5.25175863170486,-9.74105586033139,
17.4539027245749));
#49434=CARTESIAN_POINT('Ctrl Pts',(-5.19421946047611,-9.71908218930116,
17.4655424394124));
#49435=CARTESIAN_POINT('Ctrl Pts',(-5.15775787470716,-9.70515785091014,
17.4729183270348));
#49436=CARTESIAN_POINT('Ctrl Pts',(-5.11888059666409,-9.69045878605213,
17.4807088833052));
#49437=CARTESIAN_POINT('Ctrl Pts',(-5.07756380861576,-9.67503820006752,
17.4888863196405));
#49438=CARTESIAN_POINT('Ctrl Pts',(-5.01427499272364,-9.65141703604609,
17.5014124691102));
#49439=CARTESIAN_POINT('Ctrl Pts',(-4.94526265229308,-9.62610071293147,
17.5148476008571));
#49440=CARTESIAN_POINT('Ctrl Pts',(-4.87043052304886,-9.59931643249468,
17.5290729115528));
#49441=CARTESIAN_POINT('Ctrl Pts',(-4.84061083524584,-9.58864322449272,
17.5347415237937));
#49442=CARTESIAN_POINT('Ctrl Pts',(-4.80986688853492,-9.57773739840919,
17.5405353296213));
#49443=CARTESIAN_POINT('Ctrl Pts',(-4.77819214858275,-9.56661529838823,
17.5464456503157));
#49444=CARTESIAN_POINT('Ctrl Pts',(-4.70105849582066,-9.53953099707122,
17.560838337512));
#49445=CARTESIAN_POINT('Ctrl Pts',(-4.61840565271533,-9.51116108590143,
17.5759237012421));
#49446=CARTESIAN_POINT('Ctrl Pts',(-4.53013308906807,-9.48177309561077,
17.5915603571314));
#49447=CARTESIAN_POINT('Ctrl Pts',(-4.50292731933294,-9.47271566186475,
17.5963796038143));
#49448=CARTESIAN_POINT('Ctrl Pts',(-4.47518769076899,-9.46356184078189,
17.6012510356091));
#49449=CARTESIAN_POINT('Ctrl Pts',(-4.44691113574349,-9.45432033449753,
17.606170015553));
#49450=CARTESIAN_POINT('Ctrl Pts',(-4.35780736095133,-9.42519892653396,
17.6216704780645));
#49451=CARTESIAN_POINT('Ctrl Pts',(-4.26337227850525,-9.39520347024718,
17.6376449404718));
#49452=CARTESIAN_POINT('Ctrl Pts',(-4.16350775218228,-9.3646357796818,17.6539333069341));
#49453=CARTESIAN_POINT('Ctrl Pts',(-4.13544084860851,-9.35604473684446,
17.6585111488136));
#49454=CARTESIAN_POINT('Ctrl Pts',(-4.10694505979946,-9.34740876721134,
17.6631136333997));
#49455=CARTESIAN_POINT('Ctrl Pts',(-4.07801817026704,-9.33873522591717,
17.6677368410205));
#49456=CARTESIAN_POINT('Ctrl Pts',(-3.98951353504935,-9.31219768176034,
17.6818819949114));
#49457=CARTESIAN_POINT('Ctrl Pts',(-3.89697326305071,-9.2853063905167,17.6962222527625));
#49458=CARTESIAN_POINT('Ctrl Pts',(-3.80033518871561,-9.25828974819128,
17.710636274634));
#49459=CARTESIAN_POINT('Ctrl Pts',(-3.7559843940544,-9.24589080952809,17.7172514035949));
#49460=CARTESIAN_POINT('Ctrl Pts',(-3.71077051392982,-9.23346584687373,
17.7238818616415));
#49461=CARTESIAN_POINT('Ctrl Pts',(-3.66468761883613,-9.22103894118868,
17.7305148186855));
#49462=CARTESIAN_POINT('Ctrl Pts',(-3.62894139461506,-9.21139946528144,
17.735659963522));
#49463=CARTESIAN_POINT('Ctrl Pts',(-3.59267228232048,-9.2017588456811,17.7408065977769));
#49464=CARTESIAN_POINT('Ctrl Pts',(-3.5558776755651,-9.19212881406848,17.7459484822605));
#49465=CARTESIAN_POINT('Ctrl Pts',(-3.51376315393471,-9.18110643306174,
17.7518338014526));
#49466=CARTESIAN_POINT('Ctrl Pts',(-3.4709601292138,-9.17009772630246,17.7577130026888));
#49467=CARTESIAN_POINT('Ctrl Pts',(-3.42746486524502,-9.15912127550914,
17.7635761932811));
#49468=CARTESIAN_POINT('Ctrl Pts',(-3.40571723326063,-9.15363305011248,
17.7665077885773));
#49469=CARTESIAN_POINT('Ctrl Pts',(-3.38379654146372,-9.14815288863244,
17.7694353810684));
#49470=CARTESIAN_POINT('Ctrl Pts',(-3.36170232017993,-9.14268316429187,
17.7723577061799));
#49471=CARTESIAN_POINT('Ctrl Pts',(-3.35065520953803,-9.13994830212158,
17.7738188687356));
#49472=CARTESIAN_POINT('Ctrl Pts',(-3.33956471652441,-9.13721604922948,
17.7752787144339));
#49473=CARTESIAN_POINT('Ctrl Pts',(-3.3284307836757,-9.13448670717797,17.776737082515));
#49474=CARTESIAN_POINT('Ctrl Pts',(-3.32286381725134,-9.13312203615221,
17.7774662665555));
#49475=CARTESIAN_POINT('Ctrl Pts',(-3.31728599086821,-9.13175809283616,
17.7781950811909));
#49476=CARTESIAN_POINT('Ctrl Pts',(-3.31169729739565,-9.13039491526983,
17.7789235061383));
#49477=CARTESIAN_POINT('Ctrl Pts',(-3.30610860392309,-9.1290317377035,17.7796519310857));
#49478=CARTESIAN_POINT('Ctrl Pts',(-3.30168365407788,-9.12795439452993,
17.7802276294396));
#49479=CARTESIAN_POINT('Ctrl Pts',(-3.29489860859576,-9.12630771796404,
17.7811075915741));
#49480=CARTESIAN_POINT('Ctrl Pts',(-3.26344298383387,-9.11867368805258,
17.7851871159899));
#49481=CARTESIAN_POINT('Ctrl Pts',(-3.23208742976809,-9.11117310786538,
17.7891959499156));
#49482=CARTESIAN_POINT('Ctrl Pts',(-3.20083332668445,-9.10380424140559,
17.7931349824984));
#49483=CARTESIAN_POINT('Ctrl Pts',(-3.02530585865806,-9.06241964404725,
17.8152571471911));
#49484=CARTESIAN_POINT('Ctrl Pts',(-2.8529813703057,-9.02519047366263,17.835177050746));
#49485=CARTESIAN_POINT('Ctrl Pts',(-2.68409749795662,-8.99178992522898,
17.8530636449176));
#49486=CARTESIAN_POINT('Ctrl Pts',(-2.50184996588225,-8.95574641534673,
17.872365592461));
#49487=CARTESIAN_POINT('Ctrl Pts',(-2.32360980605014,-8.92416076071654,
17.8893000331733));
#49488=CARTESIAN_POINT('Ctrl Pts',(-2.14964334505202,-8.89659253190684,
17.9040958435864));
#49489=CARTESIAN_POINT('Ctrl Pts',(-2.1368280328082,-8.89456170678009,17.9051857831601));
#49490=CARTESIAN_POINT('Ctrl Pts',(-2.12403588914884,-8.89255268013611,
17.9062641193081));
#49491=CARTESIAN_POINT('Ctrl Pts',(-2.11126700969829,-8.89056527486909,
17.9073309444277));
#49492=CARTESIAN_POINT('Ctrl Pts',(-1.93627437198519,-8.86332864136276,
17.9219513770491));
#49493=CARTESIAN_POINT('Ctrl Pts',(-1.76565553955631,-8.8401523257222,17.9344099411939));
#49494=CARTESIAN_POINT('Ctrl Pts',(-1.59964365071508,-8.82055945059309,
17.944954301049));
#49495=CARTESIAN_POINT('Ctrl Pts',(-1.55749255292429,-8.81558473943635,
17.9476315571569));
#49496=CARTESIAN_POINT('Ctrl Pts',(-1.51563819099902,-8.81084107829389,
17.9501854021757));
#49497=CARTESIAN_POINT('Ctrl Pts',(-1.47408386155455,-8.80632074147676,
17.9526198695952));
#49498=CARTESIAN_POINT('Ctrl Pts',(-1.30958959117416,-8.78842682966187,
17.9622567942498));
#49499=CARTESIAN_POINT('Ctrl Pts',(-1.14980067354256,-8.77403078416562,
17.9700237199791));
#49500=CARTESIAN_POINT('Ctrl Pts',(-0.99489992585915,-8.76263900451734,
17.9761777098795));
#49501=CARTESIAN_POINT('Ctrl Pts',(-0.923085664592712,-8.75735760818978,
17.9790307899657));
#49502=CARTESIAN_POINT('Ctrl Pts',(-0.852321370951163,-8.752722228548,17.9815370749662));
#49503=CARTESIAN_POINT('Ctrl Pts',(-0.782621885807213,-8.74868521421749,
17.9837215486527));
#49504=CARTESIAN_POINT('Ctrl Pts',(-0.633275179992519,-8.74003500983875,
17.9884022711622));
#49505=CARTESIAN_POINT('Ctrl Pts',(-0.488819950878624,-8.73412973518557,
17.9916063726453));
#49506=CARTESIAN_POINT('Ctrl Pts',(-0.349378098451702,-8.73049565100499,
17.993578507991));
#49507=CARTESIAN_POINT('Ctrl Pts',(-0.26231014410065,-8.72822651681009,
17.9948099158305));
#49508=CARTESIAN_POINT('Ctrl Pts',(-0.177195960558656,-8.72684351736445,
17.9955607558549));
#49509=CARTESIAN_POINT('Ctrl Pts',(-0.0940577120238034,-8.72623777582956,
17.9958879713096));
#49510=CARTESIAN_POINT('Ctrl Pts',(0.0407719420152373,-8.72525541304196,
17.9964186337583));
#49511=CARTESIAN_POINT('Ctrl Pts',(0.170403009420359,-8.72631553881596,
17.9958365055659));
#49512=CARTESIAN_POINT('Ctrl Pts',(0.294765062228333,-8.72898214507651,
17.9943853356517));
#49513=CARTESIAN_POINT('Ctrl Pts',(0.343253157233777,-8.73002184050436,
17.9938195323131));
#49514=CARTESIAN_POINT('Ctrl Pts',(0.390940632154933,-8.73130611756855,
17.9931213835911));
#49515=CARTESIAN_POINT('Ctrl Pts',(0.437824623194182,-8.73281054765871,
17.9923044400091));
#49516=CARTESIAN_POINT('Ctrl Pts',(0.474197692479818,-8.7339776995733,17.9916706470053));
#49517=CARTESIAN_POINT('Ctrl Pts',(0.510087174592007,-8.73527737333325,
17.9909653435499));
#49518=CARTESIAN_POINT('Ctrl Pts',(0.545492010715984,-8.73669849287197,
17.9901946506401));
#49519=CARTESIAN_POINT('Ctrl Pts',(0.575387451174148,-8.73789847002779,
17.9895438863231));
#49520=CARTESIAN_POINT('Ctrl Pts',(0.604937348457799,-8.73918504043949,
17.9888464976008));
#49521=CARTESIAN_POINT('Ctrl Pts',(0.634141294414872,-8.74055156720631,
17.988106142045));
#49522=CARTESIAN_POINT('Ctrl Pts',(0.666036220849481,-8.74204401178083,
17.9872975668605));
#49523=CARTESIAN_POINT('Ctrl Pts',(0.697518424605556,-8.74363181504274,
17.986437747903));
#49524=CARTESIAN_POINT('Ctrl Pts',(0.728587589446316,-8.74530656799649,
17.9855313071974));
#49525=CARTESIAN_POINT('Ctrl Pts',(0.744122171866696,-8.74614394447337,
17.9850780868446));
#49526=CARTESIAN_POINT('Ctrl Pts',(0.75955349455732,-8.74700305820267,17.9846132107042));
#49527=CARTESIAN_POINT('Ctrl Pts',(0.774881512307569,-8.74788288241698,
17.9841372421394));
#49528=CARTESIAN_POINT('Ctrl Pts',(0.782545521182692,-8.74832279452414,
17.983899257857));
#49529=CARTESIAN_POINT('Ctrl Pts',(0.79018370382266,-8.74876788424227,17.9836585004475));
#49530=CARTESIAN_POINT('Ctrl Pts',(0.797796055871818,-8.74921802409098,
17.9834150397507));
#49531=CARTESIAN_POINT('Ctrl Pts',(0.805408407920975,-8.74966816393968,
17.9831715790539));
#49532=CARTESIAN_POINT('Ctrl Pts',(0.814759539845752,-8.75023074091324,
17.9828673475052));
#49533=CARTESIAN_POINT('Ctrl Pts',(0.820555616113578,-8.75058346697539,
17.9826766173275));
#49534=CARTESIAN_POINT('Ctrl Pts',(0.913356226197327,-8.75623094161981,
17.9796228485315));
#49535=CARTESIAN_POINT('Ctrl Pts',(1.01104127809055,-8.76312889262544,17.9758958258308));
#49536=CARTESIAN_POINT('Ctrl Pts',(1.11355367159285,-8.77158547768657,17.9713324330503));
#49537=CARTESIAN_POINT('Ctrl Pts',(1.22617244491014,-8.78087577131352,17.9663191494896));
#49538=CARTESIAN_POINT('Ctrl Pts',(1.34461811515858,-8.79204710949622,17.9602965148535));
#49539=CARTESIAN_POINT('Ctrl Pts',(1.46878588139576,-8.80553711524201,17.9530327656252));
#49540=CARTESIAN_POINT('Ctrl Pts',(1.51530094558083,-8.81059066901154,17.9503116587565));
#49541=CARTESIAN_POINT('Ctrl Pts',(1.56261868623562,-8.81596996869409,17.9474162054766));
#49542=CARTESIAN_POINT('Ctrl Pts',(1.61073229320877,-8.82169925971597,17.944333619927));
#49543=CARTESIAN_POINT('Ctrl Pts',(1.74015317028542,-8.83711048983832,17.9360417675677));
#49544=CARTESIAN_POINT('Ctrl Pts',(1.87533562169987,-8.85505222115745,17.9263967929664));
#49545=CARTESIAN_POINT('Ctrl Pts',(2.01612326058408,-8.87600820007434,17.9151439566848));
#49546=CARTESIAN_POINT('Ctrl Pts',(2.02944741125243,-8.87799147518787,17.9140789875778));
#49547=CARTESIAN_POINT('Ctrl Pts',(2.04282173407464,-8.88000176774852,17.9129996081194));
#49548=CARTESIAN_POINT('Ctrl Pts',(2.05624607591149,-8.8820394998444,17.9119055968046));
#49549=CARTESIAN_POINT('Ctrl Pts',(2.18614502510105,-8.90175735724116,17.9013195344174));
#49550=CARTESIAN_POINT('Ctrl Pts',(2.32073011534617,-8.92404342112689,17.8893639098098));
#49551=CARTESIAN_POINT('Ctrl Pts',(2.45984826428021,-8.94928033766466,17.8758377542891));
#49552=CARTESIAN_POINT('Ctrl Pts',(2.57756099628316,-8.97063417550504,17.8643928009739));
#49553=CARTESIAN_POINT('Ctrl Pts',(2.69851861493594,-8.99410110387364,17.8518232189882));
#49554=CARTESIAN_POINT('Ctrl Pts',(2.82261224042596,-9.01991399804188,17.8380070639727));
#49555=CARTESIAN_POINT('Ctrl Pts',(2.92930800732048,-9.04210793852974,17.8261279263531));
#49556=CARTESIAN_POINT('Ctrl Pts',(3.03832180266503,-9.06603631713803,17.8133271708017));
#49557=CARTESIAN_POINT('Ctrl Pts',(3.14957564004199,-9.09184572100983,17.7995283192272));
#49558=CARTESIAN_POINT('Ctrl Pts',(3.2464634479155,-9.11432239797324,17.787511291215));
#49559=CARTESIAN_POINT('Ctrl Pts',(3.34504998146593,-9.13822573668744,17.7747372610822));
#49560=CARTESIAN_POINT('Ctrl Pts',(3.44527888894342,-9.16365079871295,17.7611569125572));
#49561=CARTESIAN_POINT('Ctrl Pts',(3.44869579451264,-9.16451756498047,17.7606939446403));
#49562=CARTESIAN_POINT('Ctrl Pts',(3.45211460825154,-9.16538609969273,17.7602300396971));
#49563=CARTESIAN_POINT('Ctrl Pts',(3.455535327867,-9.16625640655736,17.7597651958156));
#49564=CARTESIAN_POINT('Ctrl Pts',(3.53359307397269,-9.186116026728,17.7491578763752));
#49565=CARTESIAN_POINT('Ctrl Pts',(3.61264341668592,-9.20689847768366,17.738061605207));
#49566=CARTESIAN_POINT('Ctrl Pts',(3.69265792828245,-9.22864750213413,17.7264538847221));
#49567=CARTESIAN_POINT('Ctrl Pts',(3.69938882440102,-9.23047705056648,17.7254774323362));
#49568=CARTESIAN_POINT('Ctrl Pts',(3.70612654329246,-9.23231343855504,17.7244973609549));
#49569=CARTESIAN_POINT('Ctrl Pts',(3.71287106704227,-9.2341566918957,17.7235136573507));
#49570=CARTESIAN_POINT('Ctrl Pts',(3.74621479932002,-9.24326941033083,17.7186504007541));
#49571=CARTESIAN_POINT('Ctrl Pts',(3.77972485700455,-9.25254992951069,17.7136983661869));
#49572=CARTESIAN_POINT('Ctrl Pts',(3.81339908956568,-9.26200133171344,17.7086559866148));
#49573=CARTESIAN_POINT('Ctrl Pts',(3.83364189329859,-9.26768291270993,17.7056248291909));
#49574=CARTESIAN_POINT('Ctrl Pts',(3.85394402439297,-9.27342624546287,17.7025610239924));
#49575=CARTESIAN_POINT('Ctrl Pts',(3.87430501375982,-9.27923199511567,17.6994642337049));
#49576=CARTESIAN_POINT('Ctrl Pts',(3.88448550844324,-9.28213486994208,17.6979158385612));
#49577=CARTESIAN_POINT('Ctrl Pts',(3.89468071769478,-9.2850533489971,17.696359197152));
#49578=CARTESIAN_POINT('Ctrl Pts',(3.90489058173839,-9.28798751523955,17.6947942674634));
#49579=CARTESIAN_POINT('Ctrl Pts',(3.9099955137602,-9.28945459836077,17.6940118026191));
#49580=CARTESIAN_POINT('Ctrl Pts',(3.91510410948001,-9.29092560327908,17.6932272657054));
#49581=CARTESIAN_POINT('Ctrl Pts',(3.92021636137619,-9.29240054033904,17.6924406514873));
#49582=CARTESIAN_POINT('Ctrl Pts',(3.92532861327237,-9.29387547739899,17.6916540372692));
#49583=CARTESIAN_POINT('Ctrl Pts',(3.93220897303425,-9.29586539662442,17.6905928060135));
#49584=CARTESIAN_POINT('Ctrl Pts',(3.93556407805506,-9.29683715828189,17.6900745716907));
#49585=CARTESIAN_POINT('Ctrl Pts',(3.94194458963118,-9.29868518881035,17.6890890287421));
#49586=CARTESIAN_POINT('Ctrl Pts',(3.94830740862757,-9.30053254622933,17.6881038759401));
#49587=CARTESIAN_POINT('Ctrl Pts',(3.95465255312891,-9.30237916219918,17.6871191496326));
#49588=CARTESIAN_POINT('Ctrl Pts',(4.02986442886426,-9.32426793885767,17.6754467420683));
#49589=CARTESIAN_POINT('Ctrl Pts',(4.10259295180635,-9.34605169598413,17.6638347266839));
#49590=CARTESIAN_POINT('Ctrl Pts',(4.17286884397023,-9.36762209671566,17.6523407877799));
#49591=CARTESIAN_POINT('Ctrl Pts',(4.24079488558807,-9.38847123704941,17.6412311775238));
#49592=CARTESIAN_POINT('Ctrl Pts',(4.30642960316497,-9.40912113845815,17.6302318353715));
#49593=CARTESIAN_POINT('Ctrl Pts',(4.36980087516246,-9.42948272269656,17.6193901793195));
#49594=CARTESIAN_POINT('Ctrl Pts',(4.43124954177303,-9.44922656185413,17.6088774455956));
#49595=CARTESIAN_POINT('Ctrl Pts',(4.49057003742806,-9.46869938263085,17.5985129410387));
#49596=CARTESIAN_POINT('Ctrl Pts',(4.54778744955938,-9.48782728920201,17.5883359882086));
#49597=CARTESIAN_POINT('Ctrl Pts',(4.60354013708818,-9.50646553512084,17.5784195580521));
#49598=CARTESIAN_POINT('Ctrl Pts',(4.65729604831056,-9.52477635419472,17.5686811746484));
#49599=CARTESIAN_POINT('Ctrl Pts',(4.70907777628743,-9.54269760101514,17.5591538849115));
#49600=CARTESIAN_POINT('Ctrl Pts',(4.75989452685353,-9.56028487677992,17.549804140802));
#49601=CARTESIAN_POINT('Ctrl Pts',(4.80880999465553,-9.57749700556393,17.5406576780202));
#49602=CARTESIAN_POINT('Ctrl Pts',(4.85584473182189,-9.59428067508138,17.5317428072007));
#49603=CARTESIAN_POINT('Ctrl Pts',(4.90206086815699,-9.61077223866507,17.5229830923596));
#49604=CARTESIAN_POINT('Ctrl Pts',(4.94646117235429,-9.62685016187419,17.5144469635652));
#49605=CARTESIAN_POINT('Ctrl Pts',(4.98906423000779,-9.64246863080901,17.5061586889104));
#49606=CARTESIAN_POINT('Ctrl Pts',(4.98944484203018,-9.64260816485599,17.5060846421834));
#49607=CARTESIAN_POINT('Ctrl Pts',(4.98982531060002,-9.64274766226093,17.5060106152213));
#49608=CARTESIAN_POINT('Ctrl Pts',(4.99020563573023,-9.64288712299273,17.5059366080404));
#49609=CARTESIAN_POINT('Ctrl Pts',(5.03327003572535,-9.65867832967558,17.4975567388471));
#49610=CARTESIAN_POINT('Ctrl Pts',(5.07449545385076,-9.67399898203165,17.4894307118898));
#49611=CARTESIAN_POINT('Ctrl Pts',(5.11390005292712,-9.68880632332554,17.4815810747738));
#49612=CARTESIAN_POINT('Ctrl Pts',(5.15370342836636,-9.70376351559733,17.4736519989676));
#49613=CARTESIAN_POINT('Ctrl Pts',(5.19164894890748,-9.71819696689999,17.4660049342146));
#49614=CARTESIAN_POINT('Ctrl Pts',(5.22775413193609,-9.73206714983678,17.4586605744959));
#49615=CARTESIAN_POINT('Ctrl Pts',(5.26453872222235,-9.74619833416345,17.4511780126999));
#49616=CARTESIAN_POINT('Ctrl Pts',(5.2994130686145,-9.75974485716931,17.4440096577332));
#49617=CARTESIAN_POINT('Ctrl Pts',(5.33239434212503,-9.77266950709506,17.4371747702162));
#49618=CARTESIAN_POINT('Ctrl Pts',(5.36640803709531,-9.78599874072917,17.4301259284215));
#49619=CARTESIAN_POINT('Ctrl Pts',(5.39840829740277,-9.7986665527749,17.4234317651715));
#49620=CARTESIAN_POINT('Ctrl Pts',(5.42841238787458,-9.81063699877864,17.4171105675975));
#49621=CARTESIAN_POINT('Ctrl Pts',(5.45995951237177,-9.82322305436067,17.4104642869171));
#49622=CARTESIAN_POINT('Ctrl Pts',(5.48929989813585,-9.83503814518865,17.4042303351122));
#49623=CARTESIAN_POINT('Ctrl Pts',(5.51645165227666,-9.84604608684465,17.3984266695236));
#49624=CARTESIAN_POINT('Ctrl Pts',(5.54440170931256,-9.85737767873876,17.3924523673338));
#49625=CARTESIAN_POINT('Ctrl Pts',(5.57003257818161,-9.86785394712241,17.3869340238601));
#49626=CARTESIAN_POINT('Ctrl Pts',(5.59336165995587,-9.87744149987479,17.3818876747373));
#49627=CARTESIAN_POINT('Ctrl Pts',(-5.8463733386606,-9.55547465583272,17.3476041037463));
#49628=CARTESIAN_POINT('Ctrl Pts',(-5.81071187586262,-9.54063151443765,
17.3552733125109));
#49629=CARTESIAN_POINT('Ctrl Pts',(-5.69191576204028,-9.4916725193938,17.380602960615));
#49630=CARTESIAN_POINT('Ctrl Pts',(-5.48048670779979,-9.40738955295889,
17.4243735747273));
#49631=CARTESIAN_POINT('Ctrl Pts',(-5.20213851496678,-9.30184043404152,
17.4793711370373));
#49632=CARTESIAN_POINT('Ctrl Pts',(-4.89413177237216,-9.19155749159157,
17.5369648709957));
#49633=CARTESIAN_POINT('Ctrl Pts',(-4.55275559255447,-9.07723151098239,
17.5967689263156));
#49634=CARTESIAN_POINT('Ctrl Pts',(-4.17237668547323,-8.95957536536919,
17.6583990236104));
#49635=CARTESIAN_POINT('Ctrl Pts',(-3.74657700614932,-8.84000925011093,
17.7211108191622));
#49636=CARTESIAN_POINT('Ctrl Pts',(-3.27005258562448,-8.72141473082344,
17.783401453449));
#49637=CARTESIAN_POINT('Ctrl Pts',(-2.73873739986321,-8.60813796297983,
17.8430033606407));
#49638=CARTESIAN_POINT('Ctrl Pts',(-2.14785706271427,-8.50557223079316,
17.8970963536719));
#49639=CARTESIAN_POINT('Ctrl Pts',(-1.4967968550619,-8.42118487526943,17.9417530293261));
#49640=CARTESIAN_POINT('Ctrl Pts',(-0.805603071092674,-8.36491582767002,
17.9716807938175));
#49641=CARTESIAN_POINT('Ctrl Pts',(-0.113474661740786,-8.34312739996358,
17.9833785830982));
#49642=CARTESIAN_POINT('Ctrl Pts',(0.536087305492918,-8.35364335445179,
17.9777186569795));
#49643=CARTESIAN_POINT('Ctrl Pts',(1.11980900607103,-8.38850996828337,17.9591202910325));
#49644=CARTESIAN_POINT('Ctrl Pts',(1.636919179711,-8.43934018271074,17.9321437718199));
#49645=CARTESIAN_POINT('Ctrl Pts',(2.09765854466679,-8.50038395982727,17.8998516626081));
#49646=CARTESIAN_POINT('Ctrl Pts',(2.51230476687163,-8.56810866040446,17.8641104411872));
#49647=CARTESIAN_POINT('Ctrl Pts',(2.88629849960366,-8.63961055570718,17.8264433928252));
#49648=CARTESIAN_POINT('Ctrl Pts',(3.22331998694596,-8.71249671744812,17.7881005995987));
#49649=CARTESIAN_POINT('Ctrl Pts',(3.52773839095892,-8.7852276671472,17.7498824286448));
#49650=CARTESIAN_POINT('Ctrl Pts',(3.80298126733865,-8.85663091467915,17.7123972644307));
#49651=CARTESIAN_POINT('Ctrl Pts',(4.05169100707615,-8.92576431324658,17.6761335665833));
#49652=CARTESIAN_POINT('Ctrl Pts',(4.27621239277721,-8.99193794361065,17.6414484058552));
#49653=CARTESIAN_POINT('Ctrl Pts',(4.47890149179128,-9.05474661932589,17.6085504399071));
#49654=CARTESIAN_POINT('Ctrl Pts',(4.66211487979546,-9.11402962441174,17.5775210304017));
#49655=CARTESIAN_POINT('Ctrl Pts',(4.82817101282,-9.16982306444236,17.548339195531));
#49656=CARTESIAN_POINT('Ctrl Pts',(4.97931089694066,-9.22231312182208,17.5209060859325));
#49657=CARTESIAN_POINT('Ctrl Pts',(5.11759928752743,-9.2717709266513,17.495079082544));
#49658=CARTESIAN_POINT('Ctrl Pts',(5.24463817723889,-9.31841704262003,17.4707425653601));
#49659=CARTESIAN_POINT('Ctrl Pts',(5.36152006758449,-9.36236512845068,17.4478370666325));
#49660=CARTESIAN_POINT('Ctrl Pts',(5.46894627430349,-9.40363534662726,17.42635189288));
#49661=CARTESIAN_POINT('Ctrl Pts',(5.5675550051916,-9.44226364631247,17.4062679240946));
#49662=CARTESIAN_POINT('Ctrl Pts',(5.65799001946662,-9.47832302411334,17.387546454043));
#49663=CARTESIAN_POINT('Ctrl Pts',(5.74089747013883,-9.5119186332035,17.3701316688078));
#49664=CARTESIAN_POINT('Ctrl Pts',(5.80283354338081,-9.5373887531129,17.356951424237));
#49665=CARTESIAN_POINT('Ctrl Pts',(5.8372084201771,-9.55166080740083,17.3495754016711));
#49666=CARTESIAN_POINT('Ctrl Pts',(5.84634761756587,-9.55546494241973,17.3476100580218));
#49667=CARTESIAN_POINT('Ctrl Pts',(-5.81214108390672,-9.67762768152041,
17.422552109006));
#49668=CARTESIAN_POINT('Ctrl Pts',(-5.77669442398367,-9.66284839961546,
17.4302152968869));
#49669=CARTESIAN_POINT('Ctrl Pts',(-5.6586054670479,-9.61409646251181,17.4555271005114));
#49670=CARTESIAN_POINT('Ctrl Pts',(-5.4483945072021,-9.53015286520016,17.4992766414301));
#49671=CARTESIAN_POINT('Ctrl Pts',(-5.17161296303814,-9.42501288020989,
17.5542583452189));
#49672=CARTESIAN_POINT('Ctrl Pts',(-4.86532906973079,-9.3151511687536,17.6118418521599));
#49673=CARTESIAN_POINT('Ctrl Pts',(-4.5258683630326,-9.20126101315959,17.6716394125171));
#49674=CARTESIAN_POINT('Ctrl Pts',(-4.14764202883284,-9.08405588457841,
17.73326560891));
#49675=CARTESIAN_POINT('Ctrl Pts',(-3.72427988122061,-8.96495263246336,
17.7959753909885));
#49676=CARTESIAN_POINT('Ctrl Pts',(-3.25051918720775,-8.84682286565692,
17.8582653016694));
#49677=CARTESIAN_POINT('Ctrl Pts',(-2.72232654864596,-8.7339958797264,17.9178671153977));
#49678=CARTESIAN_POINT('Ctrl Pts',(-2.1349611118646,-8.63184254874727,17.9719599109248));
#49679=CARTESIAN_POINT('Ctrl Pts',(-1.48780923344429,-8.54779798948218,
18.0166156513017));
#49680=CARTESIAN_POINT('Ctrl Pts',(-0.800784407919693,-8.49175868625974,
18.0465417244253));
#49681=CARTESIAN_POINT('Ctrl Pts',(-0.112803388434847,-8.47005849434548,
18.0582381566499));
#49682=CARTESIAN_POINT('Ctrl Pts',(0.532891166728138,-8.48053201472142,
18.0525789661958));
#49683=CARTESIAN_POINT('Ctrl Pts',(1.11309345819553,-8.51525647368222,18.0339820169203));
#49684=CARTESIAN_POINT('Ctrl Pts',(1.62709043164589,-8.56587948303477,18.0070066017781));
#49685=CARTESIAN_POINT('Ctrl Pts',(2.08506564285918,-8.62667559462568,17.974715114357));
#49686=CARTESIAN_POINT('Ctrl Pts',(2.49723975402976,-8.69412739933001,17.9389741366442));
#49687=CARTESIAN_POINT('Ctrl Pts',(2.86902032483964,-8.76534345922683,17.9013071615013));
#49688=CARTESIAN_POINT('Ctrl Pts',(3.20406354354222,-8.83794065763298,17.8629644838458));
#49689=CARTESIAN_POINT('Ctrl Pts',(3.50670973291176,-8.91038560785036,17.8247466485053));
#49690=CARTESIAN_POINT('Ctrl Pts',(3.78036309777869,-8.98151023781651,17.7872621736466));
#49691=CARTESIAN_POINT('Ctrl Pts',(4.02764738382,-9.05037575367207,17.750999611039));
#49692=CARTESIAN_POINT('Ctrl Pts',(4.25089072086612,-9.11629450106337,17.7163160896842));
#49693=CARTESIAN_POINT('Ctrl Pts',(4.45243283978244,-9.17886240441804,17.6834203038348));
#49694=CARTESIAN_POINT('Ctrl Pts',(4.63461440918886,-9.23791890672294,17.6523936427792));
#49695=CARTESIAN_POINT('Ctrl Pts',(4.79973861820133,-9.29349953159147,17.6232151550724));
#49696=CARTESIAN_POINT('Ctrl Pts',(4.9500320169126,-9.34578932814734,17.5957860347958));
#49697=CARTESIAN_POINT('Ctrl Pts',(5.08754619050864,-9.39505798668279,17.5699637272056));
#49698=CARTESIAN_POINT('Ctrl Pts',(5.21387275743999,-9.44152482985382,17.5456326932636));
#49699=CARTESIAN_POINT('Ctrl Pts',(5.33009684078889,-9.4853026874993,17.5227335504965));
#49700=CARTESIAN_POINT('Ctrl Pts',(5.43691472795915,-9.52641127632892,17.501255677646));
#49701=CARTESIAN_POINT('Ctrl Pts',(5.53496016576123,-9.56488609405541,17.4811800103912));
#49702=CARTESIAN_POINT('Ctrl Pts',(5.62487271584546,-9.60079963775867,17.4624678661905));
#49703=CARTESIAN_POINT('Ctrl Pts',(5.70729474319025,-9.63425659180306,17.4450633926373));
#49704=CARTESIAN_POINT('Ctrl Pts',(5.76886296772336,-9.65961934027998,17.4318922291228));
#49705=CARTESIAN_POINT('Ctrl Pts',(5.80303184039065,-9.67383042396305,17.4245217359534));
#49706=CARTESIAN_POINT('Ctrl Pts',(5.81211616128011,-9.67761826069822,17.4225578918343));
#49707=CARTESIAN_POINT('Ctrl Pts',(-5.75637793437334,-9.81403840381243,
17.4252871466828));
#49708=CARTESIAN_POINT('Ctrl Pts',(-5.72124343449299,-9.79938715618852,
17.4329279577232));
#49709=CARTESIAN_POINT('Ctrl Pts',(-5.6041894339736,-9.75105556027103,17.4581672492143));
#49710=CARTESIAN_POINT('Ctrl Pts',(-5.39579946274376,-9.66782737176423,
17.501797818414));
#49711=CARTESIAN_POINT('Ctrl Pts',(-5.12141106912661,-9.56358205149893,
17.5566355014982));
#49712=CARTESIAN_POINT('Ctrl Pts',(-4.81780022720726,-9.45466429365216,
17.6140695093037));
#49713=CARTESIAN_POINT('Ctrl Pts',(-4.48134885127786,-9.34176852335966,
17.6737106747822));
#49714=CARTESIAN_POINT('Ctrl Pts',(-4.10654179458656,-9.22560739565263,
17.7351728067037));
#49715=CARTESIAN_POINT('Ctrl Pts',(-3.68709221215214,-9.10758918936382,
17.7977114360113));
#49716=CARTESIAN_POINT('Ctrl Pts',(-3.21781356780073,-8.99056166571874,
17.859826087837));
#49717=CARTESIAN_POINT('Ctrl Pts',(-2.69473704827974,-8.87881314592504,
17.9192542591247));
#49718=CARTESIAN_POINT('Ctrl Pts',(-2.11318875262544,-8.77765876537053,
17.97318332707));
#49719=CARTESIAN_POINT('Ctrl Pts',(-1.47256892305503,-8.69445237153633,
18.017698294401));
#49720=CARTESIAN_POINT('Ctrl Pts',(-0.792573669743242,-8.6389796067912,
18.0475260652017));
#49721=CARTESIAN_POINT('Ctrl Pts',(-0.111652214361621,-8.61749917698253,
18.0591824466625));
#49722=CARTESIAN_POINT('Ctrl Pts',(0.527433781118694,-8.62786675128895,
18.0535427952304));
#49723=CARTESIAN_POINT('Ctrl Pts',(1.10168186396621,-8.66223950646855,18.0350078632655));
#49724=CARTESIAN_POINT('Ctrl Pts',(1.6104437947622,-8.71235326743348,18.0081196177625));
#49725=CARTESIAN_POINT('Ctrl Pts',(2.06380279066605,-8.77254445237208,17.9759294726917));
#49726=CARTESIAN_POINT('Ctrl Pts',(2.471875939082,-8.8393339587489,17.9402975746886));
#49727=CARTESIAN_POINT('Ctrl Pts',(2.84000970754068,-8.90986088796221,17.9027425846969));
#49728=CARTESIAN_POINT('Ctrl Pts',(3.17181456380946,-8.98176608815248,17.8645111850715));
#49729=CARTESIAN_POINT('Ctrl Pts',(3.47157828024225,-9.05353078406801,17.8264018584624));
#49730=CARTESIAN_POINT('Ctrl Pts',(3.74266244641465,-9.12399725049448,17.7890217327069));
#49731=CARTESIAN_POINT('Ctrl Pts',(3.98765665383845,-9.19223432334608,17.7528583757986));
#49732=CARTESIAN_POINT('Ctrl Pts',(4.20885881341848,-9.25755929255515,17.7182683265255));
#49733=CARTESIAN_POINT('Ctrl Pts',(4.40857962993792,-9.31957027594431,17.6854600901218));
#49734=CARTESIAN_POINT('Ctrl Pts',(4.58913208163627,-9.3781067089517,17.6545151837928));
#49735=CARTESIAN_POINT('Ctrl Pts',(4.75279328253527,-9.43320245485805,17.6254130205343));
#49736=CARTESIAN_POINT('Ctrl Pts',(4.90176552988434,-9.48503972981198,17.5980553273719));
#49737=CARTESIAN_POINT('Ctrl Pts',(5.03807866068162,-9.53388480985318,17.5723001660497));
#49738=CARTESIAN_POINT('Ctrl Pts',(5.16330731160006,-9.57995417027385,17.548032522943));
#49739=CARTESIAN_POINT('Ctrl Pts',(5.27852455024402,-9.62335879843351,17.5251933812032));
#49740=CARTESIAN_POINT('Ctrl Pts',(5.38441837965784,-9.66411743944915,17.5037723401632));
#49741=CARTESIAN_POINT('Ctrl Pts',(5.4816151955655,-9.70226458024048,17.4837505483551));
#49742=CARTESIAN_POINT('Ctrl Pts',(5.5707476032503,-9.73787152713718,17.4650895405272));
#49743=CARTESIAN_POINT('Ctrl Pts',(5.65245152948686,-9.7710416913486,17.4477336532073));
#49744=CARTESIAN_POINT('Ctrl Pts',(5.71348061603488,-9.79618593614716,17.4346000847585));
#49745=CARTESIAN_POINT('Ctrl Pts',(5.74734932939181,-9.81027420187925,17.4272509118054));
#49746=CARTESIAN_POINT('Ctrl Pts',(5.7563538024379,-9.81402928407118,17.4252927635236));
#49747=CARTESIAN_POINT('Ctrl Pts',(-5.69417905513898,-9.9277103189944,17.3549354620686));
#49748=CARTESIAN_POINT('Ctrl Pts',(-5.65936952811319,-9.91321664820986,
17.362543583712));
#49749=CARTESIAN_POINT('Ctrl Pts',(-5.54339798862242,-9.86540498256572,
17.3876752760031));
#49750=CARTESIAN_POINT('Ctrl Pts',(-5.33693877355696,-9.78307476204316,
17.431121086189));
#49751=CARTESIAN_POINT('Ctrl Pts',(-5.06512202552609,-9.67996770527826,
17.48572544092));
#49752=CARTESIAN_POINT('Ctrl Pts',(-4.76441068914013,-9.5722613821277,17.5429109986631));
#49753=CARTESIAN_POINT('Ctrl Pts',(-4.43124774750502,-9.46064969374635,
17.6022880427151));
#49754=CARTESIAN_POINT('Ctrl Pts',(-4.06020097215969,-9.34584328386552,
17.6634701828468));
#49755=CARTESIAN_POINT('Ctrl Pts',(-3.64507978641427,-9.22923895256998,
17.7257146637894));
#49756=CARTESIAN_POINT('Ctrl Pts',(-3.180788195249,-9.1136531696858,17.7875267698037));
#49757=CARTESIAN_POINT('Ctrl Pts',(-2.66343645887594,-9.00332024433173,
17.8466545610653));
#49758=CARTESIAN_POINT('Ctrl Pts',(-2.0884329388477,-8.90348131169733,17.9003005100313));
#49759=CARTESIAN_POINT('Ctrl Pts',(-1.45520082765633,-8.82138187250908,
17.9445728184062));
#49760=CARTESIAN_POINT('Ctrl Pts',(-0.783193111485207,-8.76665929244331,
17.974232179735));
#49761=CARTESIAN_POINT('Ctrl Pts',(-0.110332699532594,-8.74547074609478,
17.9858206162357));
#49762=CARTESIAN_POINT('Ctrl Pts',(0.521192190350527,-8.75569750097974,
17.9802140384361));
#49763=CARTESIAN_POINT('Ctrl Pts',(1.08866283073277,-8.7896040759372,17.961785002976));
#49764=CARTESIAN_POINT('Ctrl Pts',(1.59148482702499,-8.83904420757627,17.9350464911301));
#49765=CARTESIAN_POINT('Ctrl Pts',(2.03962503535982,-8.89843673409496,17.9030310875698));
#49766=CARTESIAN_POINT('Ctrl Pts',(2.44307842316623,-8.9643535814534,17.8675876986891));
#49767=CARTESIAN_POINT('Ctrl Pts',(2.80711889697381,-9.03397438360193,17.8302264162518));
#49768=CARTESIAN_POINT('Ctrl Pts',(3.13530190870835,-9.1049716283224,17.7921874581311));
#49769=CARTESIAN_POINT('Ctrl Pts',(3.43185318841762,-9.17584572137997,17.7542655605531));
#49770=CARTESIAN_POINT('Ctrl Pts',(3.70008397692616,-9.24545241579932,17.7170653115438));
#49771=CARTESIAN_POINT('Ctrl Pts',(3.94254344408661,-9.31287039114815,17.6810724844686));
#49772=CARTESIAN_POINT('Ctrl Pts',(4.16149389258016,-9.37742322400891,17.6466425384257));
#49773=CARTESIAN_POINT('Ctrl Pts',(4.35921216621147,-9.4387117148047,17.613983614923));
#49774=CARTESIAN_POINT('Ctrl Pts',(4.53797926335854,-9.49657512665328,17.583177424839));
#49775=CARTESIAN_POINT('Ctrl Pts',(4.70004247198356,-9.55104503278127,17.5542039813712));
#49776=CARTESIAN_POINT('Ctrl Pts',(4.84757660412767,-9.60229988245748,17.5269658902415));
#49777=CARTESIAN_POINT('Ctrl Pts',(4.98258705753238,-9.65060148608525,17.5013222155595));
#49778=CARTESIAN_POINT('Ctrl Pts',(5.10662947642265,-9.69616263511548,17.4771587717524));
#49779=CARTESIAN_POINT('Ctrl Pts',(5.22076345927117,-9.73909195903942,17.4544170892153));
#49780=CARTESIAN_POINT('Ctrl Pts',(5.32566771121937,-9.77940696831178,17.4330870766611));
#49781=CARTESIAN_POINT('Ctrl Pts',(5.4219603766622,-9.81714085302345,17.413150195144));
#49782=CARTESIAN_POINT('Ctrl Pts',(5.51026622868089,-9.8523633594578,17.3945683316977));
#49783=CARTESIAN_POINT('Ctrl Pts',(5.59121384820522,-9.88517616538835,17.3772861883258));
#49784=CARTESIAN_POINT('Ctrl Pts',(5.65167852005776,-9.91004987479868,17.3642085773892));
#49785=CARTESIAN_POINT('Ctrl Pts',(5.68523421205636,-9.9239866959767,17.3568907578296));
#49786=CARTESIAN_POINT('Ctrl Pts',(5.69415549150679,-9.92770142712335,17.3549409634383));
#49787=CARTESIAN_POINT('',(5.7364427498306,-9.52121898129658,17.3763264188218));
#49788=CARTESIAN_POINT('Origin',(5.599999999773,-9.67863108544441,17.0348569101661));
#49789=CARTESIAN_POINT('Ctrl Pts',(-5.73644387793042,-9.52121721533639,
17.3763301032685));
#49790=CARTESIAN_POINT('Ctrl Pts',(-5.66411038162322,-9.49169730087515,
17.3916242108731));
#49791=CARTESIAN_POINT('Ctrl Pts',(-5.58548128683522,-9.46019526466375,
17.407976703292));
#49792=CARTESIAN_POINT('Ctrl Pts',(-5.50055659194694,-9.42702544965956,
17.4252224559801));
#49793=CARTESIAN_POINT('Ctrl Pts',(-5.41741954382298,-9.39455385220615,
17.4421051892423));
#49794=CARTESIAN_POINT('Ctrl Pts',(-5.3282491481451,-9.3604841148662,17.4598438858076));
#49795=CARTESIAN_POINT('Ctrl Pts',(-5.23304540339397,-9.32515773279535,
17.4782590776983));
#49796=CARTESIAN_POINT('Ctrl Pts',(-5.13477099393748,-9.28869194728111,
17.4972682260551));
#49797=CARTESIAN_POINT('Ctrl Pts',(-5.03006776433377,-9.25088687600408,
17.5169983552411));
#49798=CARTESIAN_POINT('Ctrl Pts',(-4.9189357129117,-9.21216968518984,17.537224895896));
#49799=CARTESIAN_POINT('Ctrl Pts',(-4.80780366148964,-9.17345249437559,
17.557451436551));
#49800=CARTESIAN_POINT('Ctrl Pts',(-4.69024278824921,-9.13382318061147,
17.5781743903966));
#49801=CARTESIAN_POINT('Ctrl Pts',(-4.56625309151927,-9.09376132461316,
17.5991415631926));
#49802=CARTESIAN_POINT('Ctrl Pts',(-4.44622752890923,-9.05498030544612,
17.6194383844411));
#49803=CARTESIAN_POINT('Ctrl Pts',(-4.32017765149417,-9.01579421513404,
17.6399639238612));
#49804=CARTESIAN_POINT('Ctrl Pts',(-4.18810345927408,-8.97668492680345,
17.6604647283727));
#49805=CARTESIAN_POINT('Ctrl Pts',(-4.05161756545643,-8.93626926281454,
17.6816503255034));
#49806=CARTESIAN_POINT('Ctrl Pts',(-3.90869817218809,-8.89593533402846,
17.7028096566685));
#49807=CARTESIAN_POINT('Ctrl Pts',(-3.75934527946908,-8.856266693735,17.7236357378929));
#49808=CARTESIAN_POINT('Ctrl Pts',(-3.60999238675007,-8.81659805344155,
17.7444618191173));
#49809=CARTESIAN_POINT('Ctrl Pts',(-3.45420599458039,-8.77759469628942,
17.7649546527636));
#49810=CARTESIAN_POINT('Ctrl Pts',(-3.29198610296003,-8.73989286152806,
17.7847794985823));
#49811=CARTESIAN_POINT('Ctrl Pts',(-3.21175007622309,-8.72124505334789,
17.7945851200957));
#49812=CARTESIAN_POINT('Ctrl Pts',(-3.12994014689571,-8.70291646379771,
17.8042268961841));
#49813=CARTESIAN_POINT('Ctrl Pts',(-3.04655631966383,-8.68498886666937,
17.8136618172413));
#49814=CARTESIAN_POINT('Ctrl Pts',(-3.00486440604789,-8.67602506810521,
17.8183792777699));
#49815=CARTESIAN_POINT('Ctrl Pts',(-2.96277900922897,-8.66716153817332,
17.8230449853729));
#49816=CARTESIAN_POINT('Ctrl Pts',(-2.92030014046422,-8.65840882966546,
17.8276534235764));
#49817=CARTESIAN_POINT('Ctrl Pts',(-2.89906070608185,-8.65403247541154,
17.8299576426782));
#49818=CARTESIAN_POINT('Ctrl Pts',(-2.87772290314608,-8.64968382778711,
17.8322475419892));
#49819=CARTESIAN_POINT('Ctrl Pts',(-2.85628673150918,-8.64536421936501,
17.834522419904));
#49820=CARTESIAN_POINT('Ctrl Pts',(-2.84556864569073,-8.64320441515397,
17.8356598588614));
#49821=CARTESIAN_POINT('Ctrl Pts',(-2.83482596766454,-8.64105187082454,
17.836793542316));
#49822=CARTESIAN_POINT('Ctrl Pts',(-2.82405869742173,-8.63890675413443,
17.8379233819689));
#49823=CARTESIAN_POINT('Ctrl Pts',(-2.81867506230032,-8.63783419578937,
17.8384883017953));
#49824=CARTESIAN_POINT('Ctrl Pts',(-2.81328527912276,-8.63676349435921,
17.8390522606617));
#49825=CARTESIAN_POINT('Ctrl Pts',(-2.80788934788906,-8.63569467088992,
17.8396152474944));
#49826=CARTESIAN_POINT('Ctrl Pts',(-2.80249341665537,-8.63462584742063,
17.8401782343271));
#49827=CARTESIAN_POINT('Ctrl Pts',(-2.79531838615154,-8.63320975323161,
17.8409241692332));
#49828=CARTESIAN_POINT('Ctrl Pts',(-2.79168311001559,-8.63249385544467,
17.8413012807856));
#49829=CARTESIAN_POINT('Ctrl Pts',(-2.04607521596783,-8.48566070678899,
17.9186481837106));
#49830=CARTESIAN_POINT('Ctrl Pts',(-1.30047967324348,-8.39780990969505,
17.9651212818614));
#49831=CARTESIAN_POINT('Ctrl Pts',(-0.55486679613319,-8.36896299940472,
17.9806923161373));
#49832=CARTESIAN_POINT('Ctrl Pts',(-0.369912415081077,-8.36180732572766,
17.9845548178393));
#49833=CARTESIAN_POINT('Ctrl Pts',(-0.184956967406051,-8.35828253263868,
17.986515779255));
#49834=CARTESIAN_POINT('Ctrl Pts',(-7.72943142945967E-13,-8.35838942589688,
17.9865746356273));
#49835=CARTESIAN_POINT('Ctrl Pts',(6.96532233517991E-5,-8.35838946615197,
17.9865746577921));
#49836=CARTESIAN_POINT('Ctrl Pts',(0.000139306447692276,-8.35838950692212,
17.9865746796872));
#49837=CARTESIAN_POINT('Ctrl Pts',(0.000208959672248314,-8.35838954820731,
17.9865747013125));
#49838=CARTESIAN_POINT('Ctrl Pts',(0.465533924648662,-8.35866535788534,
17.9867191711212));
#49839=CARTESIAN_POINT('Ctrl Pts',(0.930858888603267,-8.38166467718553,
17.9746778420633));
#49840=CARTESIAN_POINT('Ctrl Pts',(1.39618385153606,-8.42737858503983,17.9504582799483));
#49841=CARTESIAN_POINT('Ctrl Pts',(1.62884633300245,-8.45023553896698,17.9383484988907));
#49842=CARTESIAN_POINT('Ctrl Pts',(1.86150881432015,-8.47877078912326,17.9231942078017));
#49843=CARTESIAN_POINT('Ctrl Pts',(2.09417129412707,-8.51298109397737,17.9049966542053));
#49844=CARTESIAN_POINT('Ctrl Pts',(2.21050253403054,-8.53008624640443,17.8958978774071));
#49845=CARTESIAN_POINT('Ctrl Pts',(2.32683377547297,-8.54861015630717,17.8860382965441));
#49846=CARTESIAN_POINT('Ctrl Pts',(2.44316501613488,-8.5685522661496,17.8754180780318));
#49847=CARTESIAN_POINT('Ctrl Pts',(2.50133063646584,-8.57852332107081,17.8701079687756));
#49848=CARTESIAN_POINT('Ctrl Pts',(2.55949625670459,-8.58884892557739,17.864607700846));
#49849=CARTESIAN_POINT('Ctrl Pts',(2.61766187686913,-8.59952900439952,17.8589172978087));
#49850=CARTESIAN_POINT('Ctrl Pts',(2.64674468695139,-8.60486904381058,17.8560720962901));
#49851=CARTESIAN_POINT('Ctrl Pts',(2.67582749702413,-8.61029770177647,17.8531793610399));
#49852=CARTESIAN_POINT('Ctrl Pts',(2.70491030708909,-8.61581496835059,17.8502390950788));
#49853=CARTESIAN_POINT('Ctrl Pts',(2.73217544152499,-8.62098740576383,17.8474825957402));
#49854=CARTESIAN_POINT('Ctrl Pts',(2.75944057595433,-8.62623772183578,17.8446843213643));
#49855=CARTESIAN_POINT('Ctrl Pts',(2.78670571038341,-8.63156590812219,17.8418442744992));
#49856=CARTESIAN_POINT('Ctrl Pts',(2.78852338601201,-8.63192112054128,17.8416549380415));
#49857=CARTESIAN_POINT('Ctrl Pts',(2.79172337447383,-8.63254733872129,17.8413211462471));
#49858=CARTESIAN_POINT('Ctrl Pts',(2.79215873726898,-8.63263258364449,17.8412757081596));
#49859=CARTESIAN_POINT('Ctrl Pts',(2.80635256732739,-8.63541176451781,17.8397943218317));
#49860=CARTESIAN_POINT('Ctrl Pts',(2.82657169823296,-8.63939985249501,17.8376810545087));
#49861=CARTESIAN_POINT('Ctrl Pts',(2.85281612998569,-8.6446742432296,17.8348952271828));
#49862=CARTESIAN_POINT('Ctrl Pts',(2.87906085573414,-8.64994869304904,17.8321093686494));
#49863=CARTESIAN_POINT('Ctrl Pts',(2.91133101732391,-8.65650947442629,17.8286509348427));
#49864=CARTESIAN_POINT('Ctrl Pts',(2.94962661475501,-8.66448013438173,17.8244550000515));
#49865=CARTESIAN_POINT('Ctrl Pts',(2.98792266551261,-8.67245088869036,17.8202590155906));
#49866=CARTESIAN_POINT('Ctrl Pts',(3.03224429476531,-8.68183155489256,17.8153255123835));
#49867=CARTESIAN_POINT('Ctrl Pts',(3.08259150251312,-8.69279183462203,17.8095653204095));
#49868=CARTESIAN_POINT('Ctrl Pts',(3.13293969676294,-8.70375232910697,17.8038050155705));
#49869=CARTESIAN_POINT('Ctrl Pts',(3.18931370564027,-8.71629249885724,17.797217989197));
#49870=CARTESIAN_POINT('Ctrl Pts',(3.2517135291451,-8.73062820904404,17.7896908282125));
#49871=CARTESIAN_POINT('Ctrl Pts',(3.31411405755573,-8.74496408117561,17.7821635821966));
#49872=CARTESIAN_POINT('Ctrl Pts',(3.38254053673707,-8.76109553416888,17.7736961798243));
#49873=CARTESIAN_POINT('Ctrl Pts',(3.45699296668911,-8.77928459686504,17.7641509726701));
#49874=CARTESIAN_POINT('Ctrl Pts',(3.53144681502674,-8.79747400607916,17.7546055836711));
#49875=CARTESIAN_POINT('Ctrl Pts',(3.61192684373679,-8.81772110315139,17.7439823482514));
#49876=CARTESIAN_POINT('Ctrl Pts',(3.69843305281927,-8.84033409273623,17.732119385857));
#49877=CARTESIAN_POINT('Ctrl Pts',(3.77372916539131,-8.86001672855428,17.7217937114186));
#49878=CARTESIAN_POINT('Ctrl Pts',(3.85359082346075,-8.88149251454903,17.7105284259308));
#49879=CARTESIAN_POINT('Ctrl Pts',(3.93801802702761,-8.90499316277047,17.6982018453617));
#49880=CARTESIAN_POINT('Ctrl Pts',(3.98561695038899,-8.91824251258163,17.6912522848051));
#49881=CARTESIAN_POINT('Ctrl Pts',(4.03466705650711,-8.93213595430368,17.6839651349225));
#49882=CARTESIAN_POINT('Ctrl Pts',(4.08516835096818,-8.94671873895556,17.676316648598));
#49883=CARTESIAN_POINT('Ctrl Pts',(4.11041899819872,-8.95401013128149,17.6724924054358));
#49884=CARTESIAN_POINT('Ctrl Pts',(4.13603243296646,-8.9614738754163,17.6685777961487));
#49885=CARTESIAN_POINT('Ctrl Pts',(4.16200866737389,-8.96911590964012,17.6645697329619));
#49886=CARTESIAN_POINT('Ctrl Pts',(4.17499678457761,-8.97293692675204,17.6625657013686));
#49887=CARTESIAN_POINT('Ctrl Pts',(4.18807560110365,-8.97680251739733,17.660538304294));
#49888=CARTESIAN_POINT('Ctrl Pts',(4.20124511680291,-8.98071343504126,17.6584871457692));
#49889=CARTESIAN_POINT('Ctrl Pts',(4.20782987465255,-8.98266889386323,17.6574615665068));
#49890=CARTESIAN_POINT('Ctrl Pts',(4.21443730725747,-8.98463568449712,17.6564300467572));
#49891=CARTESIAN_POINT('Ctrl Pts',(4.22106741461914,-8.9866139021614,17.6553925365324));
#49892=CARTESIAN_POINT('Ctrl Pts',(4.22769752198081,-8.98859211982568,17.6543550263075));
#49893=CARTESIAN_POINT('Ctrl Pts',(4.23593900697649,-8.99105802557391,17.6530617434669));
#49894=CARTESIAN_POINT('Ctrl Pts',(4.24102576089831,-8.99258293191174,17.6522619840224));
#49895=CARTESIAN_POINT('Ctrl Pts',(4.37039703482885,-9.03136583326327,17.6319217238558));
#49896=CARTESIAN_POINT('Ctrl Pts',(4.49374245266343,-9.07012830039618,17.61160848498));
#49897=CARTESIAN_POINT('Ctrl Pts',(4.61106201570063,-9.10839870848643,17.5915703319006));
#49898=CARTESIAN_POINT('Ctrl Pts',(4.72934461225931,-9.14698326440435,17.5713676929279));
#49899=CARTESIAN_POINT('Ctrl Pts',(4.84150201989796,-9.18506758915995,17.5514447066701));
#49900=CARTESIAN_POINT('Ctrl Pts',(4.9475342399474,-9.22221578420815,17.5320306005081));
#49901=CARTESIAN_POINT('Ctrl Pts',(5.05275997752547,-9.25908142959233,17.5127641582951));
#49902=CARTESIAN_POINT('Ctrl Pts',(5.15195334967944,-9.29502519376288,17.4939988518562));
#49903=CARTESIAN_POINT('Ctrl Pts',(5.24511435771002,-9.32966737365834,17.4759343044898));
#49904=CARTESIAN_POINT('Ctrl Pts',(5.33934638774133,-9.36470781606304,17.4576620787386));
#49905=CARTESIAN_POINT('Ctrl Pts',(5.42740655466849,-9.3984164865661,17.4401068637726));
#49906=CARTESIAN_POINT('Ctrl Pts',(5.50929485983757,-9.43044842471371,17.4234499554535));
#49907=CARTESIAN_POINT('Ctrl Pts',(5.59118316500664,-9.46248036286132,17.4067930471343));
#49908=CARTESIAN_POINT('Ctrl Pts',(5.66689960841764,-9.4928355706219,17.3910344443383));
#49909=CARTESIAN_POINT('Ctrl Pts',(5.73644419141664,-9.52121731728258,17.3763300250081));
#49910=CARTESIAN_POINT('Origin',(5.6,-9.67863108576213,17.0348569102136));
#49911=CARTESIAN_POINT('Origin',(5.59997427801229,-9.67865015413163,17.0348418886071));
#49912=CARTESIAN_POINT('Ctrl Pts',(5.7176130128486,-3.68945532772947,9.84748761497653));
#49913=CARTESIAN_POINT('Ctrl Pts',(5.72101169066759,-3.69017805224285,9.84586230390886));
#49914=CARTESIAN_POINT('Ctrl Pts',(5.76688773959286,-3.70048425892532,9.8236880828416));
#49915=CARTESIAN_POINT('Ctrl Pts',(5.85062090523121,-3.73363357303796,9.7770831424454));
#49916=CARTESIAN_POINT('Ctrl Pts',(5.94915275497326,-3.81230845463928,9.70513932835593));
#49917=CARTESIAN_POINT('Ctrl Pts',(6.01699168753275,-3.91212539537255,9.63586548676976));
#49918=CARTESIAN_POINT('Ctrl Pts',(6.04750393498136,-4.01010954209592,9.58182952763555));
#49919=CARTESIAN_POINT('Ctrl Pts',(6.05138588436001,-4.07133194826796,9.55406663714884));
#49920=CARTESIAN_POINT('Ctrl Pts',(6.05073510899355,-4.09501988092087,9.54419767224957));
#49921=CARTESIAN_POINT('Ctrl Pts',(5.60116392361712,-3.61346410389966,9.56401900963965));
#49922=CARTESIAN_POINT('Ctrl Pts',(5.6043354827448,-3.6141179583603,9.56250546762696));
#49923=CARTESIAN_POINT('Ctrl Pts',(5.64715015969186,-3.62344889768341,9.54185530555744));
#49924=CARTESIAN_POINT('Ctrl Pts',(5.72539812923533,-3.65363741952875,9.49843452207815));
#49925=CARTESIAN_POINT('Ctrl Pts',(5.81747684225603,-3.72555031859565,9.43152778111091));
#49926=CARTESIAN_POINT('Ctrl Pts',(5.88071656821272,-3.81671595959616,9.36742946903526));
#49927=CARTESIAN_POINT('Ctrl Pts',(5.90899203942426,-3.90581940681478,9.31789944012116));
#49928=CARTESIAN_POINT('Ctrl Pts',(5.91255165229384,-3.96110742538711,9.29277836968071));
#49929=CARTESIAN_POINT('Ctrl Pts',(5.91195414402012,-3.98242656800513,9.28390550969072));
#49930=CARTESIAN_POINT('Ctrl Pts',(5.58625429018143,-3.33992185286638,9.4070408693956));
#49931=CARTESIAN_POINT('Ctrl Pts',(5.59076091566283,-3.34085079789971,9.4049216144276));
#49932=CARTESIAN_POINT('Ctrl Pts',(5.65155980037929,-3.35409562789098,9.37603625759484));
#49933=CARTESIAN_POINT('Ctrl Pts',(5.76176077930928,-3.39659253349918,9.31602842442839));
#49934=CARTESIAN_POINT('Ctrl Pts',(5.89142705504701,-3.49725390257798,9.22407233768376));
#49935=CARTESIAN_POINT('Ctrl Pts',(5.98187551871793,-3.62620437369158,9.13484987539963));
#49936=CARTESIAN_POINT('Ctrl Pts',(6.02382013630363,-3.75573644179709,9.0635694766303));
#49937=CARTESIAN_POINT('Ctrl Pts',(6.02944021185559,-3.83935013265183,9.02565148550328));
#49938=CARTESIAN_POINT('Ctrl Pts',(6.02850383718158,-3.87220383486143,9.0119569801733));
#49939=CARTESIAN_POINT('Ctrl Pts',(5.68265567725631,-3.04810711614505,9.47943574065643));
#49940=CARTESIAN_POINT('Ctrl Pts',(5.68918455596363,-3.04947481887442,9.47639027304701));
#49941=CARTESIAN_POINT('Ctrl Pts',(5.77722643655303,-3.06895754584997,9.43490778788664));
#49942=CARTESIAN_POINT('Ctrl Pts',(5.93587673121703,-3.13096513514427,9.3494127976663));
#49943=CARTESIAN_POINT('Ctrl Pts',(6.12253650192003,-3.27704376992711,9.21873820754285));
#49944=CARTESIAN_POINT('Ctrl Pts',(6.25416912891128,-3.46545114247581,9.09055820339493));
#49945=CARTESIAN_POINT('Ctrl Pts',(6.31673010125175,-3.65822436169862,8.98552625787696));
#49946=CARTESIAN_POINT('Ctrl Pts',(6.32544301813554,-3.78585922915993,8.92775966642298));
#49947=CARTESIAN_POINT('Ctrl Pts',(6.32399773550576,-3.83659112696463,8.90658585651305));
#49948=CARTESIAN_POINT('',(5.99998069488466,-3.99788653537587,9.34660672384924));
#49949=CARTESIAN_POINT('',(5.99999998706781,-3.21424121943635,9.2921838327228));
#49950=CARTESIAN_POINT('Ctrl Pts',(5.99998069488466,-3.99788653537587,9.34660672384924));
#49951=CARTESIAN_POINT('Ctrl Pts',(5.99997825547866,-3.97544692625939,9.33725008234246));
#49952=CARTESIAN_POINT('Ctrl Pts',(5.99997953090646,-3.95288229363252,9.32837835501087));
#49953=CARTESIAN_POINT('Ctrl Pts',(5.99999093101457,-3.93025585224078,9.32009551206795));
#49954=CARTESIAN_POINT('Ctrl Pts',(5.99999583058559,-3.92053139566385,9.31653568818149));
#49955=CARTESIAN_POINT('Ctrl Pts',(6.00000208202755,-3.91079590771391,9.313084395188));
#49956=CARTESIAN_POINT('Ctrl Pts',(6.0000083910374,-3.90105617909432,9.3097484395143));
#49957=CARTESIAN_POINT('Ctrl Pts',(6.00002365440229,-3.87749288859613,9.30167777392408));
#49958=CARTESIAN_POINT('Ctrl Pts',(6.00004122708332,-3.85390258847053,9.29428474465244));
#49959=CARTESIAN_POINT('Ctrl Pts',(6.00006097205355,-3.83038110088263,9.28763749735748));
#49960=CARTESIAN_POINT('Ctrl Pts',(6.00007474334107,-3.81397585110789,9.28300132152971));
#49961=CARTESIAN_POINT('Ctrl Pts',(6.00008877497374,-3.79760486147016,9.2787272046869));
#49962=CARTESIAN_POINT('Ctrl Pts',(6.00009896189812,-3.78130850697401,9.27482624452034));
#49963=CARTESIAN_POINT('Ctrl Pts',(6.00011392971824,-3.75736399796689,9.26909449783633));
#49964=CARTESIAN_POINT('Ctrl Pts',(6.00011947181448,-3.73358031968664,9.26417081834576));
#49965=CARTESIAN_POINT('Ctrl Pts',(6.0001068790683,-3.71010072455357,9.26004886835312));
#49966=CARTESIAN_POINT('Ctrl Pts',(6.00010389446192,-3.70453582642796,9.25907192511121));
#49967=CARTESIAN_POINT('Ctrl Pts',(6.00009995311129,-3.698988058318,9.258139800092));
#49968=CARTESIAN_POINT('Ctrl Pts',(6.00009507698778,-3.69345939306189,9.25725200972086));
#49969=CARTESIAN_POINT('Ctrl Pts',(6.00008968453197,-3.68734529793109,9.25627021130589));
#49970=CARTESIAN_POINT('Ctrl Pts',(6.00008315014167,-3.68125456446157,9.2553426362406));
#49971=CARTESIAN_POINT('Ctrl Pts',(6.00007576287927,-3.67518971333856,9.25446844767461));
#49972=CARTESIAN_POINT('Ctrl Pts',(6.00006006901019,-3.66230524080158,9.25261127783775));
#49973=CARTESIAN_POINT('Ctrl Pts',(6.00004619203746,-3.64934307924697,9.25096136123653));
#49974=CARTESIAN_POINT('Ctrl Pts',(6.00002901871136,-3.63653958486174,9.24955726473395));
#49975=CARTESIAN_POINT('Ctrl Pts',(6.00001169308667,-3.62362254495518,9.24814071625034));
#49976=CARTESIAN_POINT('Ctrl Pts',(5.9999905602067,-3.61086748883357,9.2469745209682));
#49977=CARTESIAN_POINT('Ctrl Pts',(5.99997298498214,-3.5985341229454,9.24604863264794));
#49978=CARTESIAN_POINT('Ctrl Pts',(5.99996108050175,-3.59018018631326,9.24542148735557));
#49979=CARTESIAN_POINT('Ctrl Pts',(5.99995110675469,-3.58202007426576,9.24490350011415));
#49980=CARTESIAN_POINT('Ctrl Pts',(5.99994986561638,-3.57413696972424,9.24447901888708));
#49981=CARTESIAN_POINT('Ctrl Pts',(5.99994572912138,-3.54786397313808,9.24306429785034));
#49982=CARTESIAN_POINT('Ctrl Pts',(5.99996726956826,-3.52150110691479,9.24259411083022));
#49983=CARTESIAN_POINT('Ctrl Pts',(5.99999448700643,-3.49521226937049,9.24315082110635));
#49984=CARTESIAN_POINT('Ctrl Pts',(6.0000217044446,-3.46892343182619,9.24370753138247));
#49985=CARTESIAN_POINT('Ctrl Pts',(6.00005373135004,-3.44270963425123,9.24529169775039));
#49986=CARTESIAN_POINT('Ctrl Pts',(6.00007304312752,-3.41676089682398,9.24793117163163));
#49987=CARTESIAN_POINT('Ctrl Pts',(6.00009158147329,-3.39185139963973,9.25046493526453));
#49988=CARTESIAN_POINT('Ctrl Pts',(6.00009812241609,-3.36718699899513,9.25397091649523));
#49989=CARTESIAN_POINT('Ctrl Pts',(6.00009050007888,-3.34294012363997,9.25842391697067));
#49990=CARTESIAN_POINT('Ctrl Pts',(6.00008278309713,-3.31839218126482,9.26293220917188));
#49991=CARTESIAN_POINT('Ctrl Pts',(6.00006013980506,-3.29427323053127,9.26841096327143));
#49992=CARTESIAN_POINT('Ctrl Pts',(6.00003725529026,-3.27075809151588,9.27478305130894));
#49993=CARTESIAN_POINT('Ctrl Pts',(6.00001849832783,-3.25148424705605,9.28000584134386));
#49994=CARTESIAN_POINT('Ctrl Pts',(5.99999989152894,-3.23261615806335,9.2858276417319));
#49995=CARTESIAN_POINT('Ctrl Pts',(5.99999989737976,-3.21424117270406,9.29218369762246));
#49996=CARTESIAN_POINT('',(5.72001574683959,-3.07996623050488,9.45352741085221));
#49997=CARTESIAN_POINT('Ctrl Pts',(5.72001583932757,-3.07996630534764,9.45352764057597));
#49998=CARTESIAN_POINT('Ctrl Pts',(5.77275232442229,-3.09393993078643,9.42774314696833));
#49999=CARTESIAN_POINT('Ctrl Pts',(5.82234187961538,-3.11241974313512,9.40135240094038));
#50000=CARTESIAN_POINT('Ctrl Pts',(5.86896567632587,-3.13488603146277,9.37445534842813));
#50001=CARTESIAN_POINT('Ctrl Pts',(5.91558947303636,-3.15735231979043,9.34755829591588));
#50002=CARTESIAN_POINT('Ctrl Pts',(5.95924775859859,-3.18380528255528,9.3201555191835));
#50003=CARTESIAN_POINT('Ctrl Pts',(6.00000001914382,-3.21424127110487,9.29218398209336));
#50004=CARTESIAN_POINT('',(5.732784907806,-3.68906816095735,9.81544004097578));
#50005=CARTESIAN_POINT('Origin',(5.89877293621907,-3.22461215454891,9.89752349969974));
#50006=CARTESIAN_POINT('Ctrl Pts',(5.7327825100706,-3.68907486546999,9.81543885690915));
#50007=CARTESIAN_POINT('Ctrl Pts',(5.74764948384582,-3.69180670821221,9.80080167796743));
#50008=CARTESIAN_POINT('Ctrl Pts',(5.76167658134928,-3.69530452754189,9.78635735023664));
#50009=CARTESIAN_POINT('Ctrl Pts',(5.77486160049988,-3.69936666582116,9.77221490407054));
#50010=CARTESIAN_POINT('Ctrl Pts',(5.78891900853863,-3.70369757612544,9.75713672070559));
#50011=CARTESIAN_POINT('Ctrl Pts',(5.80201936622981,-3.70867022853965,9.74240158470817));
#50012=CARTESIAN_POINT('Ctrl Pts',(5.81418801307471,-3.71408129430063,9.72810973814384));
#50013=CARTESIAN_POINT('Ctrl Pts',(5.81740490064576,-3.71551175657096,9.72433156427077));
#50014=CARTESIAN_POINT('Ctrl Pts',(5.8205568113287,-3.7169730546453,9.72058421196347));
#50015=CARTESIAN_POINT('Ctrl Pts',(5.82364449135978,-3.71846183295476,9.71686920835376));
#50016=CARTESIAN_POINT('Ctrl Pts',(5.83601524515966,-3.72442660577562,9.70198508999997));
#50017=CARTESIAN_POINT('Ctrl Pts',(5.84735402368391,-3.73082847913117,9.68762273979523));
#50018=CARTESIAN_POINT('Ctrl Pts',(5.85773994244867,-3.73744892184006,9.6738670485));
#50019=CARTESIAN_POINT('Ctrl Pts',(5.86865590927978,-3.7444072405651,9.6594093319206));
#50020=CARTESIAN_POINT('Ctrl Pts',(5.87851959247198,-3.75160756637909,9.6456214755469));
#50021=CARTESIAN_POINT('Ctrl Pts',(5.88743536558818,-3.75884759269843,9.63256909564335));
#50022=CARTESIAN_POINT('Ctrl Pts',(5.89158024689428,-3.76221343089952,9.62650113442928));
#50023=CARTESIAN_POINT('Ctrl Pts',(5.8955204092406,-3.76558850460084,9.62059170537446));
#50024=CARTESIAN_POINT('Ctrl Pts',(5.89926696894881,-3.76895557030682,9.61484542094946));
#50025=CARTESIAN_POINT('Ctrl Pts',(5.90175393687619,-3.77119062995416,9.61103103490477));
#50026=CARTESIAN_POINT('Ctrl Pts',(5.90415560487913,-3.77342219894787,9.60728851115445));
#50027=CARTESIAN_POINT('Ctrl Pts',(5.90647529181436,-3.77564564485586,9.60361893755839));
#50028=CARTESIAN_POINT('Ctrl Pts',(5.90966133214877,-3.77869950020014,9.59857885680029));
#50029=CARTESIAN_POINT('Ctrl Pts',(5.91269274269099,-3.78173796382313,9.59367641974815));
#50030=CARTESIAN_POINT('Ctrl Pts',(5.91557902779535,-3.78474891647479,9.58891407316326));
#50031=CARTESIAN_POINT('Ctrl Pts',(5.91807289117107,-3.78735049749416,9.5847992191897));
#50032=CARTESIAN_POINT('Ctrl Pts',(5.92045834780138,-3.78993149928615,9.58078901354365));
#50033=CARTESIAN_POINT('Ctrl Pts',(5.92274147618617,-3.79248497313327,9.57688456026381));
#50034=CARTESIAN_POINT('Ctrl Pts',(5.92388304037856,-3.79376171005683,9.57493233362389));
#50035=CARTESIAN_POINT('Ctrl Pts',(5.92499901532196,-3.79503156983948,9.57300654433216));
#50036=CARTESIAN_POINT('Ctrl Pts',(5.92609014106788,-3.79629373914138,9.57110731271001));
#50037=CARTESIAN_POINT('Ctrl Pts',(5.92686106600724,-3.79718551334446,9.56976542793769));
#50038=CARTESIAN_POINT('Ctrl Pts',(5.92731171353663,-3.79771183702838,9.56897640141495));
#50039=CARTESIAN_POINT('Ctrl Pts',(5.92809603246344,-3.7986380362319,9.56759650003687));
#50040=CARTESIAN_POINT('Ctrl Pts',(5.92842179641288,-3.79902272962663,9.56702336313122));
#50041=CARTESIAN_POINT('Ctrl Pts',(5.92880480754124,-3.79947665663788,9.56634829711098));
#50042=CARTESIAN_POINT('Ctrl Pts',(5.92928969071536,-3.80005638685381,9.56548940150969));
#50043=CARTESIAN_POINT('Ctrl Pts',(5.93928521267292,-3.81200711315668,9.54778387923122));
#50044=CARTESIAN_POINT('Ctrl Pts',(5.94806892639471,-3.82437504732193,9.53071818637277));
#50045=CARTESIAN_POINT('Ctrl Pts',(5.95571469163255,-3.83695616247855,9.51437147298147));
#50046=CARTESIAN_POINT('Ctrl Pts',(5.95896087035118,-3.84229775315098,9.50743111430189));
#50047=CARTESIAN_POINT('Ctrl Pts',(5.96200197167069,-3.84767833832296,9.50061999222101));
#50048=CARTESIAN_POINT('Ctrl Pts',(5.96484395211758,-3.85308457920931,9.49394263078481));
#50049=CARTESIAN_POINT('Ctrl Pts',(5.97172175150301,-3.86616807536293,9.47778293044895));
#50050=CARTESIAN_POINT('Ctrl Pts',(5.97743430190242,-3.87939847007179,9.46240829174299));
#50051=CARTESIAN_POINT('Ctrl Pts',(5.98211309003572,-3.89258616441926,9.44786214539775));
#50052=CARTESIAN_POINT('Ctrl Pts',(5.98709331622123,-3.90662349606251,9.43237884141757));
#50053=CARTESIAN_POINT('Ctrl Pts',(5.99090179182026,-3.92061275286255,9.41783420575638));
#50054=CARTESIAN_POINT('Ctrl Pts',(5.99369013037234,-3.9343760335644,9.40425257196093));
#50055=CARTESIAN_POINT('Ctrl Pts',(5.99430533024733,-3.93741266932761,9.40125601352407));
#50056=CARTESIAN_POINT('Ctrl Pts',(5.99487086199565,-3.94043847980818,9.39830623162827));
#50057=CARTESIAN_POINT('Ctrl Pts',(5.99538834779487,-3.94345183865437,9.39540332080571));
#50058=CARTESIAN_POINT('Ctrl Pts',(5.99774241059584,-3.95715972392664,9.38219786784031));
#50059=CARTESIAN_POINT('Ctrl Pts',(5.99910410221826,-3.97060616074746,9.36996372163261));
#50060=CARTESIAN_POINT('Ctrl Pts',(5.99967027283376,-3.98363782450936,9.35869135705663));
#50061=CARTESIAN_POINT('Ctrl Pts',(5.99987914390199,-3.98844545220349,9.35453276816853));
#50062=CARTESIAN_POINT('Ctrl Pts',(5.99997953584385,-3.99319708251765,9.35050490868574));
#50063=CARTESIAN_POINT('Ctrl Pts',(5.99998069488466,-3.99788653537587,9.34660672384923));
#50064=CARTESIAN_POINT('Ctrl Pts',(5.99970218902464,-4.00041486383445,9.24574070855039));
#50065=CARTESIAN_POINT('Ctrl Pts',(5.99970218902464,-4.05365231287788,9.67397466963937));
#50066=CARTESIAN_POINT('Ctrl Pts',(5.99970218902464,-4.23216229704141,10.6067282950652));
#50067=CARTESIAN_POINT('Ctrl Pts',(5.99970218902464,-4.7103395450234,11.9928022384675));
#50068=CARTESIAN_POINT('Ctrl Pts',(5.99970218902464,-5.43783918301558,13.3613505076908));
#50069=CARTESIAN_POINT('Ctrl Pts',(5.99970218902464,-6.36842741850186,14.5997819466434));
#50070=CARTESIAN_POINT('Ctrl Pts',(5.99970218902464,-7.48063208193852,15.6796604855679));
#50071=CARTESIAN_POINT('Ctrl Pts',(5.99970218902464,-8.63550391275622,16.4940252554982));
#50072=CARTESIAN_POINT('Ctrl Pts',(5.99970218902464,-9.43064084707896,16.9071646182876));
#50073=CARTESIAN_POINT('Ctrl Pts',(5.99970218902464,-9.77579624509523,17.06208514011));
#50074=CARTESIAN_POINT('Ctrl Pts',(6.00690499952675,-3.81528531867719,9.26875000770376));
#50075=CARTESIAN_POINT('Ctrl Pts',(6.00690499952675,-3.86952777852313,9.7050827268058));
#50076=CARTESIAN_POINT('Ctrl Pts',(6.00690499952675,-4.05137912813777,10.6553011459376));
#50077=CARTESIAN_POINT('Ctrl Pts',(6.00690499952675,-4.53860924447568,12.067600402351));
#50078=CARTESIAN_POINT('Ctrl Pts',(6.00690499952675,-5.27974784182031,13.4618117081885));
#50079=CARTESIAN_POINT('Ctrl Pts',(6.00690499952675,-6.22793540867418,14.7236676441621));
#50080=CARTESIAN_POINT('Ctrl Pts',(6.00690499952675,-7.36100880388284,15.8238001511061));
#50081=CARTESIAN_POINT('Ctrl Pts',(6.00690499952675,-8.5377034970597,16.6535599584588));
#50082=CARTESIAN_POINT('Ctrl Pts',(6.00690499952675,-9.3477361651398,17.0744403871867));
#50083=CARTESIAN_POINT('Ctrl Pts',(6.00690499952675,-9.69940847689799,17.2322837299283));
#50084=CARTESIAN_POINT('Ctrl Pts',(5.89977162083546,-3.66341997502774,9.2876249804719));
#50085=CARTESIAN_POINT('Ctrl Pts',(5.89977162083546,-3.71848686465799,9.73060126728731));
#50086=CARTESIAN_POINT('Ctrl Pts',(5.89977162083546,-3.90307920092505,10.6951463942138));
#50087=CARTESIAN_POINT('Ctrl Pts',(5.89977162083546,-4.39773556012829,12.1289587817135));
#50088=CARTESIAN_POINT('Ctrl Pts',(5.89977162083546,-5.1500624594129,13.5442219724419));
#50089=CARTESIAN_POINT('Ctrl Pts',(5.89977162083546,-6.11268709790595,14.8252934760138));
#50090=CARTESIAN_POINT('Ctrl Pts',(5.89977162083546,-7.26287951709116,15.9420407043495));
#50091=CARTESIAN_POINT('Ctrl Pts',(5.89977162083546,-8.45747592600413,16.7844293584207));
#50092=CARTESIAN_POINT('Ctrl Pts',(5.89977162083546,-9.27972785235618,17.2116599331396));
#50093=CARTESIAN_POINT('Ctrl Pts',(5.89977162083546,-9.63674611439996,17.3719009223656));
#50094=CARTESIAN_POINT('Ctrl Pts',(5.72171418897201,-3.60697683468152,9.29464016057385));
#50095=CARTESIAN_POINT('Ctrl Pts',(5.72171418897201,-3.66235013659085,9.74008563368347));
#50096=CARTESIAN_POINT('Ctrl Pts',(5.72171418897201,-3.84796120360022,10.709955506594));
#50097=CARTESIAN_POINT('Ctrl Pts',(5.72171418897201,-4.34537764260743,12.1517635871689));
#50098=CARTESIAN_POINT('Ctrl Pts',(5.72171418897201,-5.10186285004451,13.5748510415821));
#50099=CARTESIAN_POINT('Ctrl Pts',(5.72171418897201,-6.0698532529814,14.8630643126808));
#50100=CARTESIAN_POINT('Ctrl Pts',(5.72171418897201,-7.22640822631808,15.9859866631895));
#50101=CARTESIAN_POINT('Ctrl Pts',(5.72171418897201,-8.42765808906915,16.8330690265054));
#50102=CARTESIAN_POINT('Ctrl Pts',(5.72171418897201,-9.25445149468778,17.2626597327244));
#50103=CARTESIAN_POINT('Ctrl Pts',(5.72171418897201,-9.61345666312839,17.4237918449321));
#50104=CARTESIAN_POINT('Ctrl Pts',(5.73278343891033,-3.68907227129128,9.81543931495127));
#50105=CARTESIAN_POINT('Ctrl Pts',(5.73338951195738,-3.73677169448297,10.0841578313552));
#50106=CARTESIAN_POINT('Ctrl Pts',(5.73395354731066,-3.79517193860139,10.3512383428457));
#50107=CARTESIAN_POINT('Ctrl Pts',(5.73447555432297,-3.86412900186718,10.6157493871671));
#50108=CARTESIAN_POINT('Ctrl Pts',(5.73532470053474,-3.97630111386147,11.0460281879475));
#50109=CARTESIAN_POINT('Ctrl Pts',(5.7360626339114,-4.11640867475991,11.4695101586091));
#50110=CARTESIAN_POINT('Ctrl Pts',(5.73668941370095,-4.28354705454678,11.8826222728609));
#50111=CARTESIAN_POINT('Ctrl Pts',(5.73681689631878,-4.31754182998523,11.9666463825406));
#50112=CARTESIAN_POINT('Ctrl Pts',(5.73693978068686,-4.3526547996942,12.0502413363141));
#50113=CARTESIAN_POINT('Ctrl Pts',(5.73705806732598,-4.38887829682059,12.1333768104643));
#50114=CARTESIAN_POINT('Ctrl Pts',(5.73707478352026,-4.39399737891054,12.1451254639772));
#50115=CARTESIAN_POINT('Ctrl Pts',(5.73709140789253,-4.39913863949845,12.1568649410002));
#50116=CARTESIAN_POINT('Ctrl Pts',(5.73710794044422,-4.40430204004992,12.1685951618524));
#50117=CARTESIAN_POINT('Ctrl Pts',(5.73767502814514,-4.58141329317504,12.5709567632529));
#50118=CARTESIAN_POINT('Ctrl Pts',(5.73813408876969,-4.78457571005312,12.9624318070339));
#50119=CARTESIAN_POINT('Ctrl Pts',(5.73848518363096,-5.01222351458537,13.3397802002642));
#50120=CARTESIAN_POINT('Ctrl Pts',(5.73855071722427,-5.05471510385475,13.4102141452326));
#50121=CARTESIAN_POINT('Ctrl Pts',(5.73861248923238,-5.09805970732631,13.4801557828557));
#50122=CARTESIAN_POINT('Ctrl Pts',(5.73867049997421,-5.14224706204589,13.5495838576326));
#50123=CARTESIAN_POINT('Ctrl Pts',(5.73897977963041,-5.3778284292935,13.9197341163462));
#50124=CARTESIAN_POINT('Ctrl Pts',(5.73918215131397,-5.6373663945189,14.2752903707391));
#50125=CARTESIAN_POINT('Ctrl Pts',(5.73927764639914,-5.91884406793555,14.6132515745047));
#50126=CARTESIAN_POINT('Ctrl Pts',(5.73929840900891,-5.98004314514966,14.6867313413138));
#50127=CARTESIAN_POINT('Ctrl Pts',(5.73931411925514,-6.04227924864683,14.7593791926461));
#50128=CARTESIAN_POINT('Ctrl Pts',(5.73932477725726,-6.10553147686454,14.8311640048254));
#50129=CARTESIAN_POINT('Ctrl Pts',(5.739373586197,-6.39519872996674,15.1599067217915));
#50130=CARTESIAN_POINT('Ctrl Pts',(5.73931644036589,-6.70617912931026,15.4705526572465));
#50131=CARTESIAN_POINT('Ctrl Pts',(5.73915333068962,-7.03611036566116,15.7604173878931));
#50132=CARTESIAN_POINT('Ctrl Pts',(5.7391174737338,-7.10864027337172,15.8241393391545));
#50133=CARTESIAN_POINT('Ctrl Pts',(5.73907649576432,-7.18208588698078,15.8868568479539));
#50134=CARTESIAN_POINT('Ctrl Pts',(5.7390303964735,-7.2564218957479,15.9485411327689));
#50135=CARTESIAN_POINT('Ctrl Pts',(5.73900084502645,-7.3040741825488,15.988083170065));
#50136=CARTESIAN_POINT('Ctrl Pts',(5.73896918906768,-7.3520923590695,16.02720062128));
#50137=CARTESIAN_POINT('Ctrl Pts',(5.73893542850084,-7.40046852267685,16.065887648773));
#50138=CARTESIAN_POINT('Ctrl Pts',(5.73869640199973,-7.74297417965619,16.3397937376393));
#50139=CARTESIAN_POINT('Ctrl Pts',(5.73835187101066,-8.10342818285287,16.5921266953169));
#50140=CARTESIAN_POINT('Ctrl Pts',(5.73790180004051,-8.47900260085346,16.8207961663496));
#50141=CARTESIAN_POINT('Ctrl Pts',(5.73786596894725,-8.50890286745421,16.8390010222174));
#50142=CARTESIAN_POINT('Ctrl Pts',(5.73782946892097,-8.53889894702324,16.8570558798847));
#50143=CARTESIAN_POINT('Ctrl Pts',(5.73779229993823,-8.56898940139243,16.8749596757298));
#50144=CARTESIAN_POINT('Ctrl Pts',(5.73741169656715,-8.87710997742077,17.058291167545));
#50145=CARTESIAN_POINT('Ctrl Pts',(5.73696095093767,-9.19512783840813,17.2257844016345));
#50146=CARTESIAN_POINT('Ctrl Pts',(5.73644003523888,-9.52122270930497,17.3763183336115));
#50147=CARTESIAN_POINT('Ctrl Pts',(5.99999999930593,-3.99788653301806,9.34660672531438));
#50148=CARTESIAN_POINT('Ctrl Pts',(5.99999999931563,-4.01825012982366,9.49792584373936));
#50149=CARTESIAN_POINT('Ctrl Pts',(5.9999999983592,-4.04202369729047,9.6482576246397));
#50150=CARTESIAN_POINT('Ctrl Pts',(5.99999999609539,-4.06917084355555,9.79770305083865));
#50151=CARTESIAN_POINT('Ctrl Pts',(5.99999999382037,-4.09645246638317,9.94788877242653));
#50152=CARTESIAN_POINT('Ctrl Pts',(5.99999999024014,-4.12714128052617,10.0971797858705));
#50153=CARTESIAN_POINT('Ctrl Pts',(5.9999999903916,-4.16125231177404,10.2456707880721));
#50154=CARTESIAN_POINT('Ctrl Pts',(5.99999999048551,-4.1824037372745,10.3377464672779));
#50155=CARTESIAN_POINT('Ctrl Pts',(5.99999999231395,-4.20487200130163,10.429514367737));
#50156=CARTESIAN_POINT('Ctrl Pts',(5.9999999950529,-4.22867039396756,10.520994409904));
#50157=CARTESIAN_POINT('Ctrl Pts',(5.99999999721691,-4.24747319330309,10.5932715968644));
#50158=CARTESIAN_POINT('Ctrl Pts',(5.99999999999964,-4.26710645549874,10.6653690537662));
#50159=CARTESIAN_POINT('Ctrl Pts',(5.99999999999964,-4.28757894249402,10.7372995926901));
#50160=CARTESIAN_POINT('Ctrl Pts',(5.99999999999964,-4.33786650262272,10.913986054968));
#50161=CARTESIAN_POINT('Ctrl Pts',(5.99999998462024,-4.39314035947195,11.0896695374196));
#50162=CARTESIAN_POINT('Ctrl Pts',(5.99999998025194,-4.45330084831765,11.2638532253973));
#50163=CARTESIAN_POINT('Ctrl Pts',(5.99999997588668,-4.51341958947054,11.4379160405689));
#50164=CARTESIAN_POINT('Ctrl Pts',(5.99999998175302,-4.57841806285475,11.6104807002592));
#50165=CARTESIAN_POINT('Ctrl Pts',(5.99999999007194,-4.64814658232175,11.7810647426391));
#50166=CARTESIAN_POINT('Ctrl Pts',(5.99999999337619,-4.6758425268787,11.8488201778063));
#50167=CARTESIAN_POINT('Ctrl Pts',(5.99999999675164,-4.7042841621304,11.9162633242021));
#50168=CARTESIAN_POINT('Ctrl Pts',(5.99999999861006,-4.73345997583683,11.983364769614));
#50169=CARTESIAN_POINT('Ctrl Pts',(5.99999999947164,-4.74698602854524,12.0144733342829));
#50170=CARTESIAN_POINT('Ctrl Pts',(5.99999999999964,-4.76066986105812,12.0455084646858));
#50171=CARTESIAN_POINT('Ctrl Pts',(5.99999999999964,-4.77450986189331,12.0764672982565));
#50172=CARTESIAN_POINT('Ctrl Pts',(5.99999999999964,-4.86135084173874,12.2707227375566));
#50173=CARTESIAN_POINT('Ctrl Pts',(5.99999998564321,-4.95440528223575,12.4619539561128));
#50174=CARTESIAN_POINT('Ctrl Pts',(5.99999998504707,-5.05350675322791,12.6499606228551));
#50175=CARTESIAN_POINT('Ctrl Pts',(5.99999998445021,-5.15272817727757,12.8381948540754));
#50176=CARTESIAN_POINT('Ctrl Pts',(5.99999999412994,-5.25801152344585,13.023197247302));
#50177=CARTESIAN_POINT('Ctrl Pts',(5.99999999838049,-5.36923749341353,13.2047460650019));
#50178=CARTESIAN_POINT('Ctrl Pts',(5.99999999937176,-5.39517633608685,13.2470847941782));
#50179=CARTESIAN_POINT('Ctrl Pts',(5.99999999999964,-5.42143857101673,13.2892355886078));
#50180=CARTESIAN_POINT('Ctrl Pts',(5.99999999999964,-5.44802303613172,13.3311954268116));
#50181=CARTESIAN_POINT('Ctrl Pts',(5.99999999999964,-5.45163185422273,13.3368914384691));
#50182=CARTESIAN_POINT('Ctrl Pts',(5.99999999998809,-5.45524657348537,13.3425839531359));
#50183=CARTESIAN_POINT('Ctrl Pts',(5.99999999996604,-5.4588671850516,13.34827295269));
#50184=CARTESIAN_POINT('Ctrl Pts',(5.99999999925237,-5.57604776336622,13.5323966140054));
#50185=CARTESIAN_POINT('Ctrl Pts',(5.99999999047919,-5.69940422499466,13.7128361170636));
#50186=CARTESIAN_POINT('Ctrl Pts',(5.99999999007259,-5.82856611522884,13.8890432899602));
#50187=CARTESIAN_POINT('Ctrl Pts',(5.99999998966574,-5.95780780329363,14.0653593258513));
#50188=CARTESIAN_POINT('Ctrl Pts',(5.99999999693161,-6.0928617689166,14.2374373446999));
#50189=CARTESIAN_POINT('Ctrl Pts',(5.99999999941399,-6.23331420401645,14.4047579275877));
#50190=CARTESIAN_POINT('Ctrl Pts',(5.9999999997784,-6.25393267611085,14.4293206542263));
#50191=CARTESIAN_POINT('Ctrl Pts',(5.99999999999964,-6.27466741733337,14.4537809157782));
#50192=CARTESIAN_POINT('Ctrl Pts',(5.99999999999964,-6.2955170479287,14.4781371321465));
#50193=CARTESIAN_POINT('Ctrl Pts',(5.99999999999964,-6.32570224107129,14.5133990084633));
#50194=CARTESIAN_POINT('Ctrl Pts',(5.99999999953037,-6.35612917108748,14.5484417054598));
#50195=CARTESIAN_POINT('Ctrl Pts',(5.99999999872727,-6.38679633278149,14.5832632927422));
#50196=CARTESIAN_POINT('Ctrl Pts',(5.99999999501559,-6.52853212226999,14.7441997763321));
#50197=CARTESIAN_POINT('Ctrl Pts',(5.99999998445152,-6.6753964956604,14.9004162347669));
#50198=CARTESIAN_POINT('Ctrl Pts',(5.999999984192,-6.82720752829195,15.0517246168236));
#50199=CARTESIAN_POINT('Ctrl Pts',(5.99999998393248,-6.9790185609235,15.2030329988804));
#50200=CARTESIAN_POINT('Ctrl Pts',(5.99999999999964,-7.13577669839019,15.3494336839672));
#50201=CARTESIAN_POINT('Ctrl Pts',(5.99999999999964,-7.29733250616056,15.4906976787841));
#50202=CARTESIAN_POINT('Ctrl Pts',(5.99999999999964,-7.36277743002716,15.5479225567596));
#50203=CARTESIAN_POINT('Ctrl Pts',(5.99999999597136,-7.42900259215504,15.6043159764659));
#50204=CARTESIAN_POINT('Ctrl Pts',(5.99999999157427,-7.4959686438229,15.6598380057875));
#50205=CARTESIAN_POINT('Ctrl Pts',(5.99999998233622,-7.63666088216823,15.7764869404068));
#50206=CARTESIAN_POINT('Ctrl Pts',(5.99999997355915,-7.78062539150357,15.8892868534789));
#50207=CARTESIAN_POINT('Ctrl Pts',(5.9999999766057,-7.92744931055709,15.9979550108572));
#50208=CARTESIAN_POINT('Ctrl Pts',(5.99999997965606,-8.07445659054523,16.1067588783776));
#50209=CARTESIAN_POINT('Ctrl Pts',(5.99999999487359,-8.22433003955843,16.2114204204104));
#50210=CARTESIAN_POINT('Ctrl Pts',(5.99999999914227,-8.3766267401238,16.3116995118965));
#50211=CARTESIAN_POINT('Ctrl Pts',(5.99999999968358,-8.39593950507439,16.3244159168884));
#50212=CARTESIAN_POINT('Ctrl Pts',(5.99999999999964,-8.41529120489321,16.3370619088378));
#50213=CARTESIAN_POINT('Ctrl Pts',(5.99999999999964,-8.43468090863971,16.3496370511817));
#50214=CARTESIAN_POINT('Ctrl Pts',(5.99999999999964,-8.54220010411144,16.4193683480303));
#50215=CARTESIAN_POINT('Ctrl Pts',(5.99999999306097,-8.65090020066499,16.4868824523981));
#50216=CARTESIAN_POINT('Ctrl Pts',(5.99999999145041,-8.76082946575123,16.5522391036968));
#50217=CARTESIAN_POINT('Ctrl Pts',(5.99999998952811,-8.89203617744543,16.6302459137806));
#50218=CARTESIAN_POINT('Ctrl Pts',(5.99999999274889,-9.02499344698057,16.7051805038707));
#50219=CARTESIAN_POINT('Ctrl Pts',(5.99999999547939,-9.15977660596245,16.77710082022));
#50220=CARTESIAN_POINT('Ctrl Pts',(5.99999999819764,-9.29395486698284,16.8486983629151));
#50221=CARTESIAN_POINT('Ctrl Pts',(5.99999999961508,-9.42994306423093,16.9173088546184));
#50222=CARTESIAN_POINT('Ctrl Pts',(5.99999999985075,-9.56784005909749,16.9829441671397));
#50223=CARTESIAN_POINT('Ctrl Pts',(5.99999999991363,-9.60463569607508,17.000457914519));
#50224=CARTESIAN_POINT('Ctrl Pts',(5.99999999993318,-9.6415673578591,17.0177595662489));
#50225=CARTESIAN_POINT('Ctrl Pts',(5.99999999993287,-9.67863716454406,17.0348487658757));
#50226=CARTESIAN_POINT('Ctrl Pts',(-5.843530343888,-3.68102569951235,9.52189994868111));
#50227=CARTESIAN_POINT('Ctrl Pts',(-3.895686895925,-3.12103648012649,10.4637294176103));
#50228=CARTESIAN_POINT('Ctrl Pts',(0.0001666015752724,-2.56022887445691,
11.4058027387879));
#50229=CARTESIAN_POINT('Ctrl Pts',(3.896020099076,-3.1210844467252,10.4636488408523));
#50230=CARTESIAN_POINT('Ctrl Pts',(5.844030148614,-3.68116939546044,9.52165827066205));
#50231=CARTESIAN_POINT('Ctrl Pts',(-5.843530343888,-3.79662279658476,10.3005519341134));
#50232=CARTESIAN_POINT('Ctrl Pts',(-3.895686895925,-3.28186758282363,11.18029373168));
#50233=CARTESIAN_POINT('Ctrl Pts',(0.0001666015752724,-2.76485680927171,
12.0606419220534));
#50234=CARTESIAN_POINT('Ctrl Pts',(3.896020099076,-3.28191180342724,11.1802184343602));
#50235=CARTESIAN_POINT('Ctrl Pts',(5.844030148614,-3.79675488524719,10.3003261880898));
#50236=CARTESIAN_POINT('Ctrl Pts',(-5.843530343888,-4.23585843751791,11.9385072545362));
#50237=CARTESIAN_POINT('Ctrl Pts',(-3.895686895925,-3.77925766167596,12.680422361665));
#50238=CARTESIAN_POINT('Ctrl Pts',(0.0001666015752724,-3.32387356034649,
13.4219941444237));
#50239=CARTESIAN_POINT('Ctrl Pts',(3.896020099076,-3.77929661126955,12.680358934072));
#50240=CARTESIAN_POINT('Ctrl Pts',(5.844030148614,-4.23597560350961,11.9383168755067));
#50241=CARTESIAN_POINT('Ctrl Pts',(-5.843530343888,-5.50359507107154,14.2139339843199));
#50242=CARTESIAN_POINT('Ctrl Pts',(-3.895686895925,-5.0227305589228,14.7660279845532));
#50243=CARTESIAN_POINT('Ctrl Pts',(0.0001666015752723,-4.54131537343371,
15.3185232177626));
#50244=CARTESIAN_POINT('Ctrl Pts',(3.896020099076,-5.02277173499103,14.7659807289254));
#50245=CARTESIAN_POINT('Ctrl Pts',(5.844030148614,-5.50371846323605,14.2137923143161));
#50246=CARTESIAN_POINT('Ctrl Pts',(-5.843530343888,-7.3885036558207,16.1560614685031));
#50247=CARTESIAN_POINT('Ctrl Pts',(-3.895686895925,-6.77499014877311,16.5818442606898));
#50248=CARTESIAN_POINT('Ctrl Pts',(0.0001666015752726,-6.16225463083715,
17.0065471100577));
#50249=CARTESIAN_POINT('Ctrl Pts',(3.896020099076,-6.77504255683397,16.5818079353));
#50250=CARTESIAN_POINT('Ctrl Pts',(5.844030148614,-7.38866108637799,16.1559522105549));
#50251=CARTESIAN_POINT('Ctrl Pts',(-5.843530343888,-8.93341404016312,17.0810032252174));
#50252=CARTESIAN_POINT('Ctrl Pts',(-3.895686895925,-8.18554344792886,17.4915898940687));
#50253=CARTESIAN_POINT('Ctrl Pts',(0.0001666015752719,-7.43613134758468,
17.9044809341154));
#50254=CARTESIAN_POINT('Ctrl Pts',(3.896020099076,-8.1856075461192,17.4915545789671));
#50255=CARTESIAN_POINT('Ctrl Pts',(5.844030148614,-8.93360594737697,17.0808978667065));
#50256=CARTESIAN_POINT('Ctrl Pts',(-5.843530343888,-9.7478162324362,17.4349042421601));
#50257=CARTESIAN_POINT('Ctrl Pts',(-3.895686895925,-8.92797948591053,17.8601610805119));
#50258=CARTESIAN_POINT('Ctrl Pts',(0.0001666015752719,-8.10806017489658,
18.2855080497002));
#50259=CARTESIAN_POINT('Ctrl Pts',(3.896020099076,-8.92804961467074,17.8601247000316));
#50260=CARTESIAN_POINT('Ctrl Pts',(5.844030148614,-9.74802660653542,17.4347951191954));
#50261=CARTESIAN_POINT('Ctrl Pts',(-5.73278975507593,-3.68906394503202,
9.81543852465543));
#50262=CARTESIAN_POINT('Ctrl Pts',(-5.37827938811351,-3.5926364172673,9.98669208751431));
#50263=CARTESIAN_POINT('Ctrl Pts',(-5.01472906935724,-3.5020771266496,10.1416940408098));
#50264=CARTESIAN_POINT('Ctrl Pts',(-4.64374065706591,-3.41910155232867,
10.2799308470485));
#50265=CARTESIAN_POINT('Ctrl Pts',(-4.36982475309857,-3.35783729529447,
10.3819967296689));
#50266=CARTESIAN_POINT('Ctrl Pts',(-4.09185399305988,-3.300710650761,10.4749208688385));
#50267=CARTESIAN_POINT('Ctrl Pts',(-3.8104731320656,-3.24841333385155,10.5585213690633));
#50268=CARTESIAN_POINT('Ctrl Pts',(-3.56966629229311,-3.20365708579314,
10.6300670036577));
#50269=CARTESIAN_POINT('Ctrl Pts',(-3.32636189347357,-3.16243849649299,
10.6947833712621));
#50270=CARTESIAN_POINT('Ctrl Pts',(-3.08096406234829,-3.12517322062064,
10.7525923015923));
#50271=CARTESIAN_POINT('Ctrl Pts',(-3.03961649590347,-3.11889432050505,
10.7623326427231));
#50272=CARTESIAN_POINT('Ctrl Pts',(-2.99820949786317,-3.11272759517701,
10.771876989757));
#50273=CARTESIAN_POINT('Ctrl Pts',(-2.95674500133169,-3.10667495605758,
10.7812251058998));
#50274=CARTESIAN_POINT('Ctrl Pts',(-2.75869126751695,-3.07776473460763,
10.8258760593922));
#50275=CARTESIAN_POINT('Ctrl Pts',(-2.55931851145658,-3.05147470370263,
10.866112310125));
#50276=CARTESIAN_POINT('Ctrl Pts',(-2.3588938886275,-3.02798173187965,10.9018069262272));
#50277=CARTESIAN_POINT('Ctrl Pts',(-2.16496946930528,-3.00525068788607,
10.9363438888161));
#50278=CARTESIAN_POINT('Ctrl Pts',(-1.97006030543694,-2.9851382609123,10.9666289729053));
#50279=CARTESIAN_POINT('Ctrl Pts',(-1.77440839311645,-2.96778003865636,
10.9925888897745));
#50280=CARTESIAN_POINT('Ctrl Pts',(-1.58213143387715,-2.95072124197205,
11.0181010037043));
#50281=CARTESIAN_POINT('Ctrl Pts',(-1.38913712967679,-2.93632253343784,
11.0394357553739));
#50282=CARTESIAN_POINT('Ctrl Pts',(-1.19565516824816,-2.92468739892694,
11.0565659989504));
#50283=CARTESIAN_POINT('Ctrl Pts',(-0.997079050885878,-2.91274592480137,
11.0741472619982));
#50284=CARTESIAN_POINT('Ctrl Pts',(-0.797989259347558,-2.90371574544053,
11.0872992420739));
#50285=CARTESIAN_POINT('Ctrl Pts',(-0.598634105458042,-2.89767892437813,
11.0960425446415));
#50286=CARTESIAN_POINT('Ctrl Pts',(-0.410109704659265,-2.89197007737159,
11.104310832897));
#50287=CARTESIAN_POINT('Ctrl Pts',(-0.221347991964562,-2.88893803264954,
11.1086367045487));
#50288=CARTESIAN_POINT('Ctrl Pts',(-0.0325589666053618,-2.88862552635304,
11.1090821638272));
#50289=CARTESIAN_POINT('Ctrl Pts',(-0.021713010796759,-2.88860757282277,
11.1091077555248));
#50290=CARTESIAN_POINT('Ctrl Pts',(-0.0108669648422019,-2.88859858781384,
11.1091205521597));
#50291=CARTESIAN_POINT('Ctrl Pts',(-2.08685607461212E-5,-2.88859857671928,
11.1091205700193));
#50292=CARTESIAN_POINT('Ctrl Pts',(-1.39123740674034E-5,-2.88859857671216,
11.1091205700308));
#50293=CARTESIAN_POINT('Ctrl Pts',(-6.95618740951635E-6,-2.88859857670874,
11.1091205700369));
#50294=CARTESIAN_POINT('Ctrl Pts',(-7.71824779259152E-13,-2.888598576709,
11.1091205700379));
#50295=CARTESIAN_POINT('Ctrl Pts',(0.189138135939297,-2.88859858396895,
11.1091205956408));
#50296=CARTESIAN_POINT('Ctrl Pts',(0.378261102849913,-2.8913297812093,11.1052308718856));
#50297=CARTESIAN_POINT('Ctrl Pts',(0.567157735032297,-2.89675072938151,
11.097386492419));
#50298=CARTESIAN_POINT('Ctrl Pts',(0.758596842520583,-2.90224464141074,
11.0894365306513));
#50299=CARTESIAN_POINT('Ctrl Pts',(0.9498034815225,-2.91050114709193,11.0774248224279));
#50300=CARTESIAN_POINT('Ctrl Pts',(1.14055784443443,-2.92144963097601,11.0613297422791));
#50301=CARTESIAN_POINT('Ctrl Pts',(1.33593682192776,-2.93266354794085,11.0448444558922));
#50302=CARTESIAN_POINT('Ctrl Pts',(1.53084132769911,-2.9467015227625,11.0240754452359));
#50303=CARTESIAN_POINT('Ctrl Pts',(1.72503517650004,-2.96345959006647,10.9990465232928));
#50304=CARTESIAN_POINT('Ctrl Pts',(1.93231732485309,-2.98134711953489,10.9723306991647));
#50305=CARTESIAN_POINT('Ctrl Pts',(2.13878979419026,-3.00233390089858,10.9407611301654));
#50306=CARTESIAN_POINT('Ctrl Pts',(2.3441653530124,-3.02626068936978,10.9044219674174));
#50307=CARTESIAN_POINT('Ctrl Pts',(2.54954091183454,-3.05018747784097,10.8680828046695));
#50308=CARTESIAN_POINT('Ctrl Pts',(2.75381956014164,-3.07705404236012,10.8269744144489));
#50309=CARTESIAN_POINT('Ctrl Pts',(2.95671406643458,-3.10667058743364,10.7812326584043));
#50310=CARTESIAN_POINT('Ctrl Pts',(3.20113148620673,-3.14234823914386,10.7261297273662));
#50311=CARTESIAN_POINT('Ctrl Pts',(3.4435512564494,-3.18199220866165,10.6642045337227));
#50312=CARTESIAN_POINT('Ctrl Pts',(3.6835774224282,-3.22519952773969,10.5955259435043));
#50313=CARTESIAN_POINT('Ctrl Pts',(3.97270114029476,-3.27724493987194,10.5127990905348));
#50314=CARTESIAN_POINT('Ctrl Pts',(4.25835187551307,-3.33445985228253,10.4202739795983));
#50315=CARTESIAN_POINT('Ctrl Pts',(4.53983760443492,-3.3961047918017,10.318138965713));
#50316=CARTESIAN_POINT('Ctrl Pts',(4.90288791141567,-3.47561224783496,10.1864088482163));
#50317=CARTESIAN_POINT('Ctrl Pts',(5.25900976155327,-3.56248371088252,10.0386967436174));
#50318=CARTESIAN_POINT('Ctrl Pts',(5.6067184086683,-3.6551237001607,9.87547719539454));
#50319=CARTESIAN_POINT('Ctrl Pts',(5.6488656544825,-3.6663529877632,9.85569265889333));
#50320=CARTESIAN_POINT('Ctrl Pts',(5.69088928597589,-3.67766709728277,9.83568028366369));
#50321=CARTESIAN_POINT('Ctrl Pts',(5.73278665883251,-3.68906325960823,9.81544090739529));
#50322=CARTESIAN_POINT('Ctrl Pts',(-5.8453425191731,-3.7231328100584,9.78106691208113));
#50323=CARTESIAN_POINT('Ctrl Pts',(-5.67506455328666,-3.67640115211964,
9.86772733904583));
#50324=CARTESIAN_POINT('Ctrl Pts',(-5.16554261231927,-3.54223933518448,
10.1122105914422));
#50325=CARTESIAN_POINT('Ctrl Pts',(-4.2479673722814,-3.3315423036423,10.4776605637613));
#50326=CARTESIAN_POINT('Ctrl Pts',(-3.01809829204943,-3.11148833491602,
10.8376786076768));
#50327=CARTESIAN_POINT('Ctrl Pts',(-1.5847636096142,-2.94366648313399,11.0983867442987));
#50328=CARTESIAN_POINT('Ctrl Pts',(-0.000577220786009364,-2.87785633358549,
11.197120468893));
#50329=CARTESIAN_POINT('Ctrl Pts',(1.58371386520435,-2.94357748223322,11.0985217867746));
#50330=CARTESIAN_POINT('Ctrl Pts',(3.01728962515512,-3.11136351464933,10.8378775916792));
#50331=CARTESIAN_POINT('Ctrl Pts',(4.24739718405343,-3.33142250739312,10.4778629558088));
#50332=CARTESIAN_POINT('Ctrl Pts',(5.16523409169761,-3.54216090499289,10.1123513050415));
#50333=CARTESIAN_POINT('Ctrl Pts',(5.67493343697088,-3.67636527157484,9.86779379746524));
#50334=CARTESIAN_POINT('Ctrl Pts',(5.84532822576121,-3.72312888450214,9.78107419617581));
#50335=CARTESIAN_POINT('Ctrl Pts',(-5.72604640297174,-3.64453078977728,
9.50066684202224));
#50336=CARTESIAN_POINT('Ctrl Pts',(-5.55920897504384,-3.59938887890874,
9.58541783912223));
#50337=CARTESIAN_POINT('Ctrl Pts',(-5.05998748611983,-3.46975016126909,
9.82453542560563));
#50338=CARTESIAN_POINT('Ctrl Pts',(-4.16100412910273,-3.26599618147832,
10.1820357658773));
#50339=CARTESIAN_POINT('Ctrl Pts',(-2.95616914600619,-3.05303432798076,
10.5342751778561));
#50340=CARTESIAN_POINT('Ctrl Pts',(-1.55217413832987,-2.89053739077631,
10.789367770727));
#50341=CARTESIAN_POINT('Ctrl Pts',(-0.000565337860044441,-2.82679815128164,
10.8859758425079));
#50342=CARTESIAN_POINT('Ctrl Pts',(1.55114593661906,-2.8904511972708,10.789499906014));
#50343=CARTESIAN_POINT('Ctrl Pts',(2.95537697819746,-3.05291349664009,10.534469871294));
#50344=CARTESIAN_POINT('Ctrl Pts',(4.16044551304384,-3.26588029055499,10.1822337713712));
#50345=CARTESIAN_POINT('Ctrl Pts',(5.05968520530428,-3.46967435460816,9.82467306139067));
#50346=CARTESIAN_POINT('Ctrl Pts',(5.55908050810257,-3.59935421833968,9.58548283353558));
#50347=CARTESIAN_POINT('Ctrl Pts',(5.7260323983644,-3.6445269978645,9.50067396559784));
#50348=CARTESIAN_POINT('Ctrl Pts',(-5.72051779202094,-3.37344235740397,
9.34118936873082));
#50349=CARTESIAN_POINT('Ctrl Pts',(-5.55415467081518,-3.32879645284527,
9.42508071207038));
#50350=CARTESIAN_POINT('Ctrl Pts',(-5.05630407037826,-3.20054253028145,
9.66183113507364));
#50351=CARTESIAN_POINT('Ctrl Pts',(-4.15940711858513,-2.99876113157881,
10.0160784557331));
#50352=CARTESIAN_POINT('Ctrl Pts',(-2.95633243052256,-2.78754959294785,
10.3655357023154));
#50353=CARTESIAN_POINT('Ctrl Pts',(-1.5529049313792,-2.62613144283214,10.6189509912225));
#50354=CARTESIAN_POINT('Ctrl Pts',(-0.000565719984574329,-2.56273619156729,
10.7150256790838));
#50355=CARTESIAN_POINT('Ctrl Pts',(1.55187664827042,-2.62604575142131,10.6190823491583));
#50356=CARTESIAN_POINT('Ctrl Pts',(2.95554107092965,-2.78742966586911,10.3657289784477));
#50357=CARTESIAN_POINT('Ctrl Pts',(4.15884962684187,-2.99864629259101,10.0162747578376));
#50358=CARTESIAN_POINT('Ctrl Pts',(5.05600259450201,-3.20046751258044,9.66196743919455));
#50359=CARTESIAN_POINT('Ctrl Pts',(5.55402656806235,-3.32876217187809,9.4251450482282));
#50360=CARTESIAN_POINT('Ctrl Pts',(5.72050382722823,-3.37343860686065,9.34119641994125));
#50361=CARTESIAN_POINT('Ctrl Pts',(-5.8321369521679,-3.08677373258812,9.40625311678606));
#50362=CARTESIAN_POINT('Ctrl Pts',(-5.6629787715248,-3.04120920698067,9.49089236294299));
#50363=CARTESIAN_POINT('Ctrl Pts',(-5.15669403421204,-2.91030605895675,
9.72980983428538));
#50364=CARTESIAN_POINT('Ctrl Pts',(-4.24405124974489,-2.70425182829767,
10.0876100470662));
#50365=CARTESIAN_POINT('Ctrl Pts',(-3.01836174675186,-2.48831932058566,
10.4410836918675));
#50366=CARTESIAN_POINT('Ctrl Pts',(-1.58641566211653,-2.32303952972319,
10.6978445692024));
#50367=CARTESIAN_POINT('Ctrl Pts',(-0.000578094601629952,-2.25804067749337,
10.7953224050997));
#50368=CARTESIAN_POINT('Ctrl Pts',(1.58536576833291,-2.32295171259286,10.6979777817111));
#50369=CARTESIAN_POINT('Ctrl Pts',(3.0175550085335,-2.48819663021148,10.4412793413565));
#50370=CARTESIAN_POINT('Ctrl Pts',(4.24348372250814,-2.70413450834432,10.0878084330091));
#50371=CARTESIAN_POINT('Ctrl Pts',(5.15638741473864,-2.91022948542556,9.72994741671057));
#50372=CARTESIAN_POINT('Ctrl Pts',(5.66284851503276,-3.04117421967098,9.49095727370096));
#50373=CARTESIAN_POINT('Ctrl Pts',(5.83212275275338,-3.08676990438137,9.40626023074137));
#50374=CARTESIAN_POINT('Ctrl Pts',(-5.72001848982158,-3.07996758646315,
9.45352556453397));
#50375=CARTESIAN_POINT('Ctrl Pts',(-5.58622578267763,-3.04453966207226,
9.51893357204611));
#50376=CARTESIAN_POINT('Ctrl Pts',(-5.44977387166592,-3.00953603645086,
9.5826456141395));
#50377=CARTESIAN_POINT('Ctrl Pts',(-5.31065166372667,-2.97511769228166,
9.64449101662499));
#50378=CARTESIAN_POINT('Ctrl Pts',(-5.13208489793212,-2.93094090344732,
9.72387110744355));
#50379=CARTESIAN_POINT('Ctrl Pts',(-4.94911791823773,-2.88772691608189,
9.80017676710201));
#50380=CARTESIAN_POINT('Ctrl Pts',(-4.76175997779212,-2.8458635140101,9.87302804119503));
#50381=CARTESIAN_POINT('Ctrl Pts',(-4.7051486885805,-2.83321424408094,9.89504047652233));
#50382=CARTESIAN_POINT('Ctrl Pts',(-4.64813670743062,-2.82068854073505,
9.91673738375662));
#50383=CARTESIAN_POINT('Ctrl Pts',(-4.59072480806432,-2.80829778838811,
9.9381078908515));
#50384=CARTESIAN_POINT('Ctrl Pts',(-4.4857722613471,-2.78564671728773,9.97717451587178));
#50385=CARTESIAN_POINT('Ctrl Pts',(-4.37948383410515,-2.76344222716346,
10.0151514952229));
#50386=CARTESIAN_POINT('Ctrl Pts',(-4.27186582327879,-2.74174263669791,
10.0519746286223));
#50387=CARTESIAN_POINT('Ctrl Pts',(-4.17673451642801,-2.7225608066003,10.0845252470152));
#50388=CARTESIAN_POINT('Ctrl Pts',(-4.08056426553211,-2.70377355566689,
10.1161742105508));
#50389=CARTESIAN_POINT('Ctrl Pts',(-3.98336429796612,-2.68542343476573,
10.1468761006882));
#50390=CARTESIAN_POINT('Ctrl Pts',(-3.87978521472512,-2.6658690177438,10.1795929185415));
#50391=CARTESIAN_POINT('Ctrl Pts',(-3.7750360592736,-2.6468099807019,10.2112347704345));
#50392=CARTESIAN_POINT('Ctrl Pts',(-3.66912935139674,-2.62829352068104,
10.2417467237293));
#50393=CARTESIAN_POINT('Ctrl Pts',(-3.6161759974583,-2.61903529067062,10.2570027003767));
#50394=CARTESIAN_POINT('Ctrl Pts',(-3.56293325208084,-2.60991270167467,
10.2719761901948));
#50395=CARTESIAN_POINT('Ctrl Pts',(-3.509403031323,-2.60093137580247,10.2866602299529));
#50396=CARTESIAN_POINT('Ctrl Pts',(-3.48263792094408,-2.59644071286637,
10.294002249832));
#50397=CARTESIAN_POINT('Ctrl Pts',(-3.45580094155328,-2.59198536552492,
10.3012719064436));
#50398=CARTESIAN_POINT('Ctrl Pts',(-3.42889234295528,-2.58756602568168,
10.3084683245832));
#50399=CARTESIAN_POINT('Ctrl Pts',(-3.41543804365629,-2.58535635576006,
10.312066533653));
#50400=CARTESIAN_POINT('Ctrl Pts',(-3.40196583954607,-2.58315568770107,
10.3156464330547));
#50401=CARTESIAN_POINT('Ctrl Pts',(-3.38847576308459,-2.58096410694689,
10.3192079130426));
#50402=CARTESIAN_POINT('Ctrl Pts',(-3.38173072485385,-2.5798683165698,10.3209886530365));
#50403=CARTESIAN_POINT('Ctrl Pts',(-3.37498121853475,-2.57877479801818,
10.3227647881738));
#50404=CARTESIAN_POINT('Ctrl Pts',(-3.36822724826745,-2.5776835619006,10.3245363047155));
#50405=CARTESIAN_POINT('Ctrl Pts',(-3.36147327800015,-2.57659232578302,
10.3263078212572));
#50406=CARTESIAN_POINT('Ctrl Pts',(-3.35627145380202,-2.57575348794432,
10.3276690999076));
#50407=CARTESIAN_POINT('Ctrl Pts',(-3.3479519497851,-2.57441671143473,10.3298369848019));
#50408=CARTESIAN_POINT('Ctrl Pts',(-3.25356415140478,-2.5592504958275,10.3544324272589));
#50409=CARTESIAN_POINT('Ctrl Pts',(-3.15870247896028,-2.54463161966691,
10.3780134172734));
#50410=CARTESIAN_POINT('Ctrl Pts',(-3.06338153310827,-2.53058637637817,
10.4005674015095));
#50411=CARTESIAN_POINT('Ctrl Pts',(-2.82247525276361,-2.49508958931858,
10.4575684771985));
#50412=CARTESIAN_POINT('Ctrl Pts',(-2.57863516797202,-2.46325459397254,
10.5080123788613));
#50413=CARTESIAN_POINT('Ctrl Pts',(-2.33218278235404,-2.43545349318644,
10.5516955911938));
#50414=CARTESIAN_POINT('Ctrl Pts',(-2.10395730382933,-2.40970848157087,
10.5921481192271));
#50415=CARTESIAN_POINT('Ctrl Pts',(-1.87349141229418,-2.38742283707054,
10.6268027113683));
#50416=CARTESIAN_POINT('Ctrl Pts',(-1.64104497974962,-2.36891812822664,
10.6554678629544));
#50417=CARTESIAN_POINT('Ctrl Pts',(-1.3922221275377,-2.3491097173877,10.6861525445761));
#50418=CARTESIAN_POINT('Ctrl Pts',(-1.14112895901219,-2.33363391051612,
10.7099744151135));
#50419=CARTESIAN_POINT('Ctrl Pts',(-0.888194890405294,-2.32271175966412,
10.7267278495743));
#50420=CARTESIAN_POINT('Ctrl Pts',(-0.642857048742712,-2.31211762763951,
10.7429781375394));
#50421=CARTESIAN_POINT('Ctrl Pts',(-0.39578685941527,-2.30580769801516,
10.7525781133018));
#50422=CARTESIAN_POINT('Ctrl Pts',(-0.147396649499607,-2.30401191327079,
10.7553051728695));
#50423=CARTESIAN_POINT('Ctrl Pts',(-0.098524625314327,-2.30365858358244,
10.7558417355673));
#50424=CARTESIAN_POINT('Ctrl Pts',(-0.0496015747295809,-2.3034800992254,
10.756112120393));
#50425=CARTESIAN_POINT('Ctrl Pts',(-0.000630754449614001,-2.30347834825338,
10.7561144689972));
#50426=CARTESIAN_POINT('Ctrl Pts',(-0.000533215627239487,-2.30347834476584,
10.7561144736751));
#50427=CARTESIAN_POINT('Ctrl Pts',(-0.000435676615370138,-2.30347834197944,
10.7561144772896));
#50428=CARTESIAN_POINT('Ctrl Pts',(-0.000338137414028911,-2.30347833989419,
10.7561144798408));
#50429=CARTESIAN_POINT('Ctrl Pts',(0.244409904318021,-2.30347310752446,
10.7561208812728));
#50430=CARTESIAN_POINT('Ctrl Pts',(0.487933354864567,-2.30778625269226,
10.7494552516389));
#50431=CARTESIAN_POINT('Ctrl Pts',(0.729872147671101,-2.31627266092412,
10.7363207591529));
#50432=CARTESIAN_POINT('Ctrl Pts',(0.979162356039925,-2.32501693236518,
10.7227871693939));
#50433=CARTESIAN_POINT('Ctrl Pts',(1.22677062301498,-2.33819212181328,10.7023856402231));
#50434=CARTESIAN_POINT('Ctrl Pts',(1.47230782490225,-2.35567297733128,10.6752950678761));
#50435=CARTESIAN_POINT('Ctrl Pts',(1.528321383462,-2.35966082486195,10.6691149886501));
#50436=CARTESIAN_POINT('Ctrl Pts',(1.58422716278209,-2.36387287435707,10.6625866267576));
#50437=CARTESIAN_POINT('Ctrl Pts',(1.64002053878389,-2.36830785902908,10.6557118041948));
#50438=CARTESIAN_POINT('Ctrl Pts',(1.66262960639652,-2.37010504133809,10.6529259299695));
#50439=CARTESIAN_POINT('Ctrl Pts',(1.6852202161838,-2.3719388327086,10.6500831621575));
#50440=CARTESIAN_POINT('Ctrl Pts',(1.70779213306391,-2.37380899889092,10.6471836667687));
#50441=CARTESIAN_POINT('Ctrl Pts',(1.96542943282148,-2.39515519504559,10.6140886413609));
#50442=CARTESIAN_POINT('Ctrl Pts',(2.2206321287962,-2.42118695686794,10.5736172429053));
#50443=CARTESIAN_POINT('Ctrl Pts',(2.4730072388591,-2.45145930067294,10.5260280642484));
#50444=CARTESIAN_POINT('Ctrl Pts',(2.49462591754807,-2.45405245684322,10.5219515324454));
#50445=CARTESIAN_POINT('Ctrl Pts',(2.51622385526068,-2.45667675055344,10.51782274966));
#50446=CARTESIAN_POINT('Ctrl Pts',(2.53780080883655,-2.45933191372699,10.5136418660488));
#50447=CARTESIAN_POINT('Ctrl Pts',(2.67453329246864,-2.47615760016557,10.4871477366566));
#50448=CARTESIAN_POINT('Ctrl Pts',(2.81042370077703,-2.4942183611075,10.4585625221685));
#50449=CARTESIAN_POINT('Ctrl Pts',(2.94541467454037,-2.51342296590514,10.4279279256618));
#50450=CARTESIAN_POINT('Ctrl Pts',(2.98455461983106,-2.51899124325105,10.4190455804365));
#50451=CARTESIAN_POINT('Ctrl Pts',(3.02361901368985,-2.52465562262786,10.4099909370238));
#50452=CARTESIAN_POINT('Ctrl Pts',(3.062606395271,-2.53041373041998,10.4007650315162));
#50453=CARTESIAN_POINT('Ctrl Pts',(3.0908514097118,-2.53458528108956,10.3940811809029));
#50454=CARTESIAN_POINT('Ctrl Pts',(3.11905600485032,-2.53880602549,10.3873074429548));
#50455=CARTESIAN_POINT('Ctrl Pts',(3.14721977094275,-2.54307494828719,10.3804442461762));
#50456=CARTESIAN_POINT('Ctrl Pts',(3.18073927009834,-2.54815566631426,10.3722759167749));
#50457=CARTESIAN_POINT('Ctrl Pts',(3.21420086917299,-2.55330468622933,10.3639808691688));
#50458=CARTESIAN_POINT('Ctrl Pts',(3.24760374504299,-2.55852039067303,10.3555598279387));
#50459=CARTESIAN_POINT('Ctrl Pts',(3.26430518297799,-2.56112824289488,10.3513493073237));
#50460=CARTESIAN_POINT('Ctrl Pts',(3.28099194011519,-2.56375276624447,10.3471072882752));
#50461=CARTESIAN_POINT('Ctrl Pts',(3.29766391504872,-2.56639375418664,10.3428338619783));
#50462=CARTESIAN_POINT('Ctrl Pts',(3.30599990251548,-2.56771424815772,10.3406971488299));
#50463=CARTESIAN_POINT('Ctrl Pts',(3.31433219443153,-2.56903885827675,10.3385525838679));
#50464=CARTESIAN_POINT('Ctrl Pts',(3.32266077821784,-2.57036755844855,10.3364001785307));
#50465=CARTESIAN_POINT('Ctrl Pts',(3.33098936200414,-2.57169625862036,10.3342477731935));
#50466=CARTESIAN_POINT('Ctrl Pts',(3.34087181527658,-2.57327928504732,10.3316817010557));
#50467=CARTESIAN_POINT('Ctrl Pts',(3.34763539263782,-2.57436590294479,10.3299194528409));
#50468=CARTESIAN_POINT('Ctrl Pts',(3.55089958588706,-2.60702177401758,10.2769590233857));
#50469=CARTESIAN_POINT('Ctrl Pts',(3.75013357593846,-2.64183173682445,10.2197943054953));
#50470=CARTESIAN_POINT('Ctrl Pts',(3.94524370460647,-2.67839851809335,10.158815086571));
#50471=CARTESIAN_POINT('Ctrl Pts',(4.0552261841343,-2.69901100653647,10.1244414446553));
#50472=CARTESIAN_POINT('Ctrl Pts',(4.16389879090913,-2.72018245532118,10.0888553228505));
#50473=CARTESIAN_POINT('Ctrl Pts',(4.27124838423353,-2.74184714293357,10.0521233937558));
#50474=CARTESIAN_POINT('Ctrl Pts',(4.46895191147968,-2.78174655032778,9.98447495914437));
#50475=CARTESIAN_POINT('Ctrl Pts',(4.66216685332365,-2.82331649695166,9.91294166868344));
#50476=CARTESIAN_POINT('Ctrl Pts',(4.85086295645824,-2.86617782292787,9.83792425129904));
#50477=CARTESIAN_POINT('Ctrl Pts',(5.00709279590326,-2.90166460810482,9.77581401754829));
#50478=CARTESIAN_POINT('Ctrl Pts',(5.16022547334113,-2.93803744985436,9.7113149597602));
#50479=CARTESIAN_POINT('Ctrl Pts',(5.3102552388505,-2.97510203019643,9.64464181156364));
#50480=CARTESIAN_POINT('Ctrl Pts',(5.44951286408245,-3.00950537290067,9.58275579679139));
#50481=CARTESIAN_POINT('Ctrl Pts',(5.58609733333168,-3.04450498702027,9.5189965480568));
#50482=CARTESIAN_POINT('Ctrl Pts',(5.72001565386956,-3.07996615527252,9.45352717993155));
#50483=CARTESIAN_POINT('Ctrl Pts',(6.00000005199879,6.44013554119082,7.42971628364908));
#50484=CARTESIAN_POINT('Ctrl Pts',(6.00000005199403,9.01014101712317,5.2020156589276));
#50485=CARTESIAN_POINT('Ctrl Pts',(6.00000005199597,9.65438823628283,1.86247620859738));
#50486=CARTESIAN_POINT('Ctrl Pts',(-1.77480316135306E-8,8.02987800172561,
9.26373598251951));
#50487=CARTESIAN_POINT('Ctrl Pts',(-1.77539708778783E-8,11.2342873349703,
6.48612918736558));
#50488=CARTESIAN_POINT('Ctrl Pts',(-1.77515442403932E-8,12.0375664802193,
2.32222701533043));
#50489=CARTESIAN_POINT('Ctrl Pts',(-6.00000008250361,6.44013553309638,7.42971627433652));
#50490=CARTESIAN_POINT('Ctrl Pts',(-6.00000008250837,9.01014100581212,5.20201565240322));
#50491=CARTESIAN_POINT('Ctrl Pts',(-6.00000008250642,9.65438822416544,1.86247620625276));
#50492=CARTESIAN_POINT('',(5.7200157459055,6.64701177631153,7.39409270204038));
#50493=CARTESIAN_POINT('',(5.99999953411714,6.4401355833762,7.4297163323166));
#50494=CARTESIAN_POINT('Ctrl Pts',(5.72001583931743,6.64701193944996,7.39409288350795));
#50495=CARTESIAN_POINT('Ctrl Pts',(5.77253148998233,6.61781801791691,7.39330532480335));
#50496=CARTESIAN_POINT('Ctrl Pts',(5.82202450461072,6.5858191061159,7.39608179412492));
#50497=CARTESIAN_POINT('Ctrl Pts',(5.86865900539029,6.55130191359264,7.40207789646962));
#50498=CARTESIAN_POINT('Ctrl Pts',(5.91529350616986,6.51678472106939,7.40807399881431));
#50499=CARTESIAN_POINT('Ctrl Pts',(5.95906967163339,6.47974956148326,7.41729007990723));
#50500=CARTESIAN_POINT('Ctrl Pts',(5.99999937684364,6.44013572009114,7.42971649001226));
#50501=CARTESIAN_POINT('Origin',(6.,0.,0.));
#50502=CARTESIAN_POINT('Origin',(-6.,0.,0.));
#50503=CARTESIAN_POINT('Ctrl Pts',(-5.72001846589485,6.6470094591946,7.39409290851757));
#50504=CARTESIAN_POINT('Ctrl Pts',(-5.5231394901781,6.75643001701867,7.39707039774803));
#50505=CARTESIAN_POINT('Ctrl Pts',(-5.32171545225581,6.86151613067316,7.39900784396097));
#50506=CARTESIAN_POINT('Ctrl Pts',(-5.11578943779626,6.96176314152386,7.40010341334367));
#50507=CARTESIAN_POINT('Ctrl Pts',(-4.91516479974086,7.05942938500864,7.40117077829727));
#50508=CARTESIAN_POINT('Ctrl Pts',(-4.71026659833169,7.1525025851152,7.40143882576999));
#50509=CARTESIAN_POINT('Ctrl Pts',(-4.50119423812476,7.24046082476656,7.40113344297331));
#50510=CARTESIAN_POINT('Ctrl Pts',(-4.46405236415797,7.25608667721419,7.40107919147237));
#50511=CARTESIAN_POINT('Ctrl Pts',(-4.42677882349615,7.27155100068417,7.40100689257849));
#50512=CARTESIAN_POINT('Ctrl Pts',(-4.38937426489685,7.28685073592356,7.40091787860229));
#50513=CARTESIAN_POINT('Ctrl Pts',(-4.17290200939842,7.3753952427918,7.40040272598668));
#50514=CARTESIAN_POINT('Ctrl Pts',(-3.95203428931582,7.45845302868536,7.39930682641914));
#50515=CARTESIAN_POINT('Ctrl Pts',(-3.7269248624741,7.5355061201909,7.39778910172017));
#50516=CARTESIAN_POINT('Ctrl Pts',(-3.71074103037603,7.54104571181556,7.3976799876682));
#50517=CARTESIAN_POINT('Ctrl Pts',(-3.69453527868055,7.54655424740712,7.39756870270795));
#50518=CARTESIAN_POINT('Ctrl Pts',(-3.67830766648862,7.55203152508966,7.39745531031399));
#50519=CARTESIAN_POINT('Ctrl Pts',(-3.60089666987613,7.57815992396402,7.39691439165503));
#50520=CARTESIAN_POINT('Ctrl Pts',(-3.52298895693033,7.60357773171555,7.39632456351004));
#50521=CARTESIAN_POINT('Ctrl Pts',(-3.44459143400836,7.62826428789934,7.39569108136119));
#50522=CARTESIAN_POINT('Ctrl Pts',(-3.40047427644871,7.64215631724125,7.39533459775393));
#50523=CARTESIAN_POINT('Ctrl Pts',(-3.35620200852254,7.6558167669054,7.39496429626105));
#50524=CARTESIAN_POINT('Ctrl Pts',(-3.31177650809438,7.66924224160979,7.39458087586784));
#50525=CARTESIAN_POINT('Ctrl Pts',(-3.25009102911909,7.68788371620499,7.39404849085527));
#50526=CARTESIAN_POINT('Ctrl Pts',(-3.18810964288943,7.70607203893023,7.39349109916318));
#50527=CARTESIAN_POINT('Ctrl Pts',(-3.12583671604774,7.72379802072698,7.39291073386073));
#50528=CARTESIAN_POINT('Ctrl Pts',(-3.09470025262689,7.73266101162535,7.3926205512095));
#50529=CARTESIAN_POINT('Ctrl Pts',(-3.06349090352057,7.74140841611209,7.39232462394246));
#50530=CARTESIAN_POINT('Ctrl Pts',(-3.03220922812262,7.75003908895116,7.39202318308018));
#50531=CARTESIAN_POINT('Ctrl Pts',(-3.00884507995295,7.75648530119685,7.39179803820284));
#50532=CARTESIAN_POINT('Ctrl Pts',(-2.98452267292826,7.76311520667045,7.39156074387149));
#50533=CARTESIAN_POINT('Ctrl Pts',(-2.96129868966198,7.76936973295334,7.39133170399724));
#50534=CARTESIAN_POINT('Ctrl Pts',(-2.95342866082446,7.77148923595362,7.39125408809498));
#50535=CARTESIAN_POINT('Ctrl Pts',(-2.94568489488984,7.77356606825519,7.39117742788552));
#50536=CARTESIAN_POINT('Ctrl Pts',(-2.9381477896787,7.77557976789438,7.39110253765057));
#50537=CARTESIAN_POINT('Ctrl Pts',(-2.68063742192718,7.84437919686656,7.38854386142102));
#50538=CARTESIAN_POINT('Ctrl Pts',(-2.42065148233588,7.90438548668657,7.38592323930718));
#50539=CARTESIAN_POINT('Ctrl Pts',(-2.15860855950913,7.95529807856872,7.38352069964086));
#50540=CARTESIAN_POINT('Ctrl Pts',(-2.01267631483025,7.98365140609092,7.38218272034092));
#50541=CARTESIAN_POINT('Ctrl Pts',(-1.86610582915604,8.00918356196372,7.38091238473016));
#50542=CARTESIAN_POINT('Ctrl Pts',(-1.71896772590052,8.03183579119116,7.37975842699033));
#50543=CARTESIAN_POINT('Ctrl Pts',(-1.45705453073431,8.07215789405457,7.3777043244021));
#50544=CARTESIAN_POINT('Ctrl Pts',(-1.19334276940858,8.10335765529222,7.37601877690129));
#50545=CARTESIAN_POINT('Ctrl Pts',(-0.928342879505017,8.1252642313035,7.37479855228938));
#50546=CARTESIAN_POINT('Ctrl Pts',(-0.668537591582842,8.14674138848295,
7.3736022468617));
#50547=CARTESIAN_POINT('Ctrl Pts',(-0.407493628490775,8.15928616787887,
7.37285308614969));
#50548=CARTESIAN_POINT('Ctrl Pts',(-0.145694535144678,8.16268769725533,
7.372646938407));
#50549=CARTESIAN_POINT('Ctrl Pts',(-0.0970991151635496,8.16331909267582,
7.37260867304861));
#50550=CARTESIAN_POINT('Ctrl Pts',(-0.0484776976229812,8.16363531386543,
7.37258913331296));
#50551=CARTESIAN_POINT('Ctrl Pts',(0.000166591020086083,8.16363481584133,
7.37258895560197));
#50552=CARTESIAN_POINT('Ctrl Pts',(0.00190546548824369,8.1636347980386,
7.37258894924938));
#50553=CARTESIAN_POINT('Ctrl Pts',(0.00364430926348846,8.16363437718273,
7.37258896579267));
#50554=CARTESIAN_POINT('Ctrl Pts',(0.00538312221381099,8.16363355325788,
7.3725890052864));
#50555=CARTESIAN_POINT('Ctrl Pts',(0.259912769618426,8.16351294609251,7.37259478642919));
#50556=CARTESIAN_POINT('Ctrl Pts',(0.513782238937853,8.15476007749901,7.37309182573407));
#50557=CARTESIAN_POINT('Ctrl Pts',(0.766576370396224,8.13753903915246,7.37403648893198));
#50558=CARTESIAN_POINT('Ctrl Pts',(1.00754521736796,8.12112357202875,7.37493696237361));
#50559=CARTESIAN_POINT('Ctrl Pts',(1.24753735727697,8.09701304609678,7.37624432959361));
#50560=CARTESIAN_POINT('Ctrl Pts',(1.48618589673797,8.06530630036304,7.37792465400272));
#50561=CARTESIAN_POINT('Ctrl Pts',(1.56754515871502,8.0544969426422,7.37849750458088));
#50562=CARTESIAN_POINT('Ctrl Pts',(1.6487503410598,8.04280946435164,7.3791078552369));
#50563=CARTESIAN_POINT('Ctrl Pts',(1.72978561822472,8.03024812918833,7.37975303236793));
#50564=CARTESIAN_POINT('Ctrl Pts',(1.89313269532141,8.00492758417209,7.3810535498987));
#50565=CARTESIAN_POINT('Ctrl Pts',(2.05578951477151,7.97605676126106,7.3824955366271));
#50566=CARTESIAN_POINT('Ctrl Pts',(2.21765372151952,7.94371404951127,7.38401368809007));
#50567=CARTESIAN_POINT('Ctrl Pts',(2.33873564296813,7.9195202035573,7.38514933567936));
#50568=CARTESIAN_POINT('Ctrl Pts',(2.45937279180157,7.89338226720244,7.38632911534868));
#50569=CARTESIAN_POINT('Ctrl Pts',(2.57952171143478,7.86533439980899,7.38752196222305));
#50570=CARTESIAN_POINT('Ctrl Pts',(2.63959617125139,7.85131046611226,7.38811838566023));
#50571=CARTESIAN_POINT('Ctrl Pts',(2.69954857141069,7.83680903390877,7.38871806148018));
#50572=CARTESIAN_POINT('Ctrl Pts',(2.7593736446158,7.82183476231597,7.38931646224121));
#50573=CARTESIAN_POINT('Ctrl Pts',(2.78928618121835,7.81434762651956,7.38961566262172));
#50574=CARTESIAN_POINT('Ctrl Pts',(2.81916688587343,7.80674227990913,7.38991454333619));
#50575=CARTESIAN_POINT('Ctrl Pts',(2.84901510459825,7.79901931313223,7.39021251677589));
#50576=CARTESIAN_POINT('Ctrl Pts',(2.87148424617008,7.79320561833642,7.39043682521665));
#50577=CARTESIAN_POINT('Ctrl Pts',(2.89300660022682,7.7875698938843,7.39065136963934));
#50578=CARTESIAN_POINT('Ctrl Pts',(2.91567876299272,7.78156096265451,7.39087679799907));
#50579=CARTESIAN_POINT('Ctrl Pts',(2.92312451421291,7.77958757319457,7.39095083078994));
#50580=CARTESIAN_POINT('Ctrl Pts',(2.93069416777718,7.77757354050241,7.39102603214866));
#50581=CARTESIAN_POINT('Ctrl Pts',(2.93846165110485,7.77549814727366,7.39110311474753));
#50582=CARTESIAN_POINT('Ctrl Pts',(3.1129971918326,7.72886401056257,7.39283516263321));
#50583=CARTESIAN_POINT('Ctrl Pts',(3.2853220231655,7.67854873869928,7.39445121691232));
#50584=CARTESIAN_POINT('Ctrl Pts',(3.45533244333518,7.62478460087811,7.39587259330837));
#50585=CARTESIAN_POINT('Ctrl Pts',(3.67851266022001,7.5542060332375,7.39773849712785));
#50586=CARTESIAN_POINT('Ctrl Pts',(3.89770434676101,7.47768574414708,7.39926806331439));
#50587=CARTESIAN_POINT('Ctrl Pts',(4.11277404326721,7.39575790599373,7.4002663862923));
#50588=CARTESIAN_POINT('Ctrl Pts',(4.33342340127712,7.31170457265415,7.40129060926625));
#50589=CARTESIAN_POINT('Ctrl Pts',(4.54973416432406,7.22195941871552,7.40175575729507));
#50590=CARTESIAN_POINT('Ctrl Pts',(4.76157917497623,7.12705170436546,7.4014738087237));
#50591=CARTESIAN_POINT('Ctrl Pts',(4.88434076837461,7.07205384435666,7.40131042297403));
#50592=CARTESIAN_POINT('Ctrl Pts',(5.00560304486508,7.01532149034196,7.4008965645055));
#50593=CARTESIAN_POINT('Ctrl Pts',(5.12534365331553,6.95695073152344,7.4001987774091));
#50594=CARTESIAN_POINT('Ctrl Pts',(5.32794536978775,6.85818711171679,7.39901811810486));
#50595=CARTESIAN_POINT('Ctrl Pts',(5.52619035504277,6.75473480708681,7.3970239419566));
#50596=CARTESIAN_POINT('Ctrl Pts',(5.72001565335726,6.64701161468287,7.39409252225231));
#50597=CARTESIAN_POINT('Ctrl Pts',(6.00000005305837,9.65438841513202,-1.86247527920914));
#50598=CARTESIAN_POINT('Ctrl Pts',(6.00000005303346,9.01014286082918,-5.20200782794672));
#50599=CARTESIAN_POINT('Ctrl Pts',(6.00000005304398,6.44014582844665,-7.42970736600423));
#50600=CARTESIAN_POINT('Ctrl Pts',(-1.7587155508212E-8,12.0375667041905,
-2.32222585665684));
#50601=CARTESIAN_POINT('Ctrl Pts',(-1.7618217734301E-8,11.2342896346967,
-6.48611942381034));
#50602=CARTESIAN_POINT('Ctrl Pts',(-1.76051041844286E-8,8.02989082900566,
-9.26372486430082));
#50603=CARTESIAN_POINT('Ctrl Pts',(-6.00000008328868,9.65438840314804,-1.86247527680773));
#50604=CARTESIAN_POINT('Ctrl Pts',(-6.0000000833136,9.01014284963475,-5.20200782145258));
#50605=CARTESIAN_POINT('Ctrl Pts',(-6.00000008330308,6.44014582040185,-7.42970735677997));
#50606=CARTESIAN_POINT('Origin',(6.,0.,0.));
#50607=CARTESIAN_POINT('Origin',(-6.,0.,0.));
#50608=CARTESIAN_POINT('Ctrl Pts',(6.00000005573429,3.21424330149493,-9.2921832640953));
#50609=CARTESIAN_POINT('Ctrl Pts',(6.00000005573452,4.88217919558463E-7,
-10.4040165263461));
#50610=CARTESIAN_POINT('Ctrl Pts',(6.00000005573716,-3.2142424294058,-9.29218356575536));
#50611=CARTESIAN_POINT('Ctrl Pts',(-1.69778360931036E-8,4.00767676717802,
-11.5859514948856));
#50612=CARTESIAN_POINT('Ctrl Pts',(-1.69775501936307E-8,6.08730473134062E-7,
-12.9722399354743));
#50613=CARTESIAN_POINT('Ctrl Pts',(-1.69742616027712E-8,-4.00767567982168,
-11.5859518710102));
#50614=CARTESIAN_POINT('Ctrl Pts',(-6.00000008491477,3.21424329763521,-9.29218325293956));
#50615=CARTESIAN_POINT('Ctrl Pts',(-6.00000008491454,4.8821256750661E-7,
-10.4040165138571));
#50616=CARTESIAN_POINT('Ctrl Pts',(-6.00000008491191,-3.21424242555678,
-9.29218355459962));
#50617=CARTESIAN_POINT('Origin',(6.,0.,0.));
#50618=CARTESIAN_POINT('Origin',(-6.,0.,0.));
#50619=CARTESIAN_POINT('Ctrl Pts',(6.00000005306065,-6.44014511329475,-7.42970798589525));
#50620=CARTESIAN_POINT('Ctrl Pts',(6.00000005305654,-9.01014216102169,-5.20200886777526));
#50621=CARTESIAN_POINT('Ctrl Pts',(6.00000005306017,-9.65438814672,-1.86247667057917));
#50622=CARTESIAN_POINT('Ctrl Pts',(-1.75871222825539E-8,-8.02988993733495,
-9.26372563720854));
#50623=CARTESIAN_POINT('Ctrl Pts',(-1.75922418001345E-8,-11.2342887621353,
-6.48612072033671));
#50624=CARTESIAN_POINT('Ctrl Pts',(-1.75877127682732E-8,-12.0375663695084,
-2.32222759153221));
#50625=CARTESIAN_POINT('Ctrl Pts',(-6.0000000832888,-6.44014510527518,-7.42970797666555));
#50626=CARTESIAN_POINT('Ctrl Pts',(-6.00000008329291,-9.01014214981644,
-5.20200886130693));
#50627=CARTESIAN_POINT('Ctrl Pts',(-6.00000008328928,-9.65438813471616,
-1.86247666825039));
#50628=CARTESIAN_POINT('Origin',(6.,0.,0.));
#50629=CARTESIAN_POINT('Origin',(-6.,0.,0.));
#50630=CARTESIAN_POINT('Ctrl Pts',(6.000000013908,-9.65439079723555,1.86246301485801));
#50631=CARTESIAN_POINT('Ctrl Pts',(6.00000001391134,-9.01014839527905,5.20200203764751));
#50632=CARTESIAN_POINT('Ctrl Pts',(6.00000001391262,-6.44014751247661,7.42970592721792));
#50633=CARTESIAN_POINT('Ctrl Pts',(-1.18290251301301E-8,-12.0375696345227,
2.32221055724884));
#50634=CARTESIAN_POINT('Ctrl Pts',(-1.18248668144419E-8,-11.2342964981915,
6.48611218277015));
#50635=CARTESIAN_POINT('Ctrl Pts',(-1.18232696314301E-8,-8.02989290222649,
9.26372303973634));
#50636=CARTESIAN_POINT('Ctrl Pts',(-6.00000003423866,-9.65439078915668,
1.86246301331147));
#50637=CARTESIAN_POINT('Ctrl Pts',(-6.00000003423532,-9.01014838773964,
5.20200203330458));
#50638=CARTESIAN_POINT('Ctrl Pts',(-6.00000003423404,-6.4401475070892,7.42970592100962));
#50639=CARTESIAN_POINT('Origin',(6.,0.,0.));
#50640=CARTESIAN_POINT('Origin',(-6.,0.,0.));
#50641=CARTESIAN_POINT('Ctrl Pts',(6.00000005197452,-3.21424126676338,9.29218396954236));
#50642=CARTESIAN_POINT('Ctrl Pts',(6.00000005200753,6.38646761553304E-7,
10.4040161294932));
#50643=CARTESIAN_POINT('Ctrl Pts',(6.00000005199697,3.21424240755215,9.29218357491516));
#50644=CARTESIAN_POINT('Ctrl Pts',(-1.77795276204544E-8,-4.00767422901088,
11.5859523713311));
#50645=CARTESIAN_POINT('Ctrl Pts',(-1.77383742545913E-8,7.96323979804973E-7,
12.9722394371238));
#50646=CARTESIAN_POINT('Ctrl Pts',(-1.7751541202668E-8,4.007675651458,11.5859518792905));
#50647=CARTESIAN_POINT('Ctrl Pts',(-6.00000008253,-3.2142412626098,9.29218395789083));
#50648=CARTESIAN_POINT('Ctrl Pts',(-6.00000008249699,6.38688659984361E-7,
10.4040161164194));
#50649=CARTESIAN_POINT('Ctrl Pts',(-6.00000008250755,3.21424240348237,9.29218356326364));
#50650=CARTESIAN_POINT('Origin',(6.,0.,0.));
#50651=CARTESIAN_POINT('Origin',(-6.,0.,0.));
#50652=CARTESIAN_POINT('Origin',(-7.4,0.,0.));
#50653=CARTESIAN_POINT('',(-7.4,-6.00000000007803,-10.3923048453649));
#50654=CARTESIAN_POINT('Origin',(-7.4,-6.75000000009103,-11.6913429510374));
#50655=CARTESIAN_POINT('Origin',(-6.,-6.75000000009103,-11.6913429510374));
#50656=CARTESIAN_POINT('',(-6.,-6.00000000007803,-10.3923048453649));
#50657=CARTESIAN_POINT('Origin',(-6.,-6.75000000009103,-11.6913429510374));
#50658=CARTESIAN_POINT('',(-6.,-6.00000000008095,-10.3923048453666));
#50659=CARTESIAN_POINT('Origin',(-7.4,-7.10542735750424E-15,1.23069611929084E-14));
#50660=CARTESIAN_POINT('',(-7.4,11.9999999999972,-9.50004519495451E-11));
#50661=CARTESIAN_POINT('Origin',(-7.4,13.5,-1.05000452776949E-10));
#50662=CARTESIAN_POINT('Origin',(-6.,13.5,-1.05000452776949E-10));
#50663=CARTESIAN_POINT('',(-6.,11.9999999999972,-9.50004519495451E-11));
#50664=CARTESIAN_POINT('Origin',(-6.,13.5,-1.05000452776949E-10));
#50665=CARTESIAN_POINT('',(-6.,12.,-9.33005511289567E-11));
#50666=CARTESIAN_POINT('Origin',(-6.,0.,0.));
#50667=CARTESIAN_POINT('Ctrl Pts',(-6.00000000001697,9.91329802718485,16.8993701947934));
#50668=CARTESIAN_POINT('Ctrl Pts',(-6.00000000001004,9.90992616536129,16.9013320391245));
#50669=CARTESIAN_POINT('Ctrl Pts',(-6.00000000000346,9.90655400604938,16.9032934158647));
#50670=CARTESIAN_POINT('Ctrl Pts',(-5.9999999999973,9.90318155035889,16.9052543221561));
#50671=CARTESIAN_POINT('Ctrl Pts',(-5.99999999993207,9.86751358933603,16.9259933727437));
#50672=CARTESIAN_POINT('Ctrl Pts',(-5.99999999990816,9.83181247294486,16.9466797991169));
#50673=CARTESIAN_POINT('Ctrl Pts',(-5.99999999990816,9.79607949297214,16.9673102431511));
#50674=CARTESIAN_POINT('Ctrl Pts',(-5.99999999990816,9.76034664910791,16.9879406086031));
#50675=CARTESIAN_POINT('Ctrl Pts',(-5.99999999993207,9.72458194169295,17.0085149922637));
#50676=CARTESIAN_POINT('Ctrl Pts',(-5.9999999999973,9.68878892570787,17.0290339621741));
#50677=CARTESIAN_POINT('Ctrl Pts',(-6.00000000000346,9.68540449666687,17.030974145077));
#50678=CARTESIAN_POINT('Ctrl Pts',(-6.00000000001005,9.68201981451976,17.0329138325694));
#50679=CARTESIAN_POINT('Ctrl Pts',(-6.00000000001698,9.67863488229756,17.0348530251257));
#50680=CARTESIAN_POINT('Ctrl Pts',(-5.59335880963394,10.1144382223412,17.2450574867612));
#50681=CARTESIAN_POINT('Ctrl Pts',(-5.59335897597996,10.1110305794363,17.2470401530682));
#50682=CARTESIAN_POINT('Ctrl Pts',(-5.59336249921667,10.0355852078339,17.290921844848));
#50683=CARTESIAN_POINT('Ctrl Pts',(-5.59336249921667,9.95658496883867,17.3365326540989));
#50684=CARTESIAN_POINT('Ctrl Pts',(-5.59335897597996,9.8808596232004,17.3799294166115));
#50685=CARTESIAN_POINT('Ctrl Pts',(-5.59335880963394,9.87743876235887,17.3818891887806));
#50686=CARTESIAN_POINT('Ctrl Pts',(-5.83074004399705,10.1164205431219,17.2484645412161));
#50687=CARTESIAN_POINT('Ctrl Pts',(-5.83074021197843,10.1130125214895,17.2504473136498));
#50688=CARTESIAN_POINT('Ctrl Pts',(-5.83074376985068,10.0375588131129,17.2943314352281));
#50689=CARTESIAN_POINT('Ctrl Pts',(-5.83074376985068,9.95855095808478,17.3399466416001));
#50690=CARTESIAN_POINT('Ctrl Pts',(-5.83074021197843,9.88281933979067,17.3833494090707));
#50691=CARTESIAN_POINT('Ctrl Pts',(-5.83074004399706,9.87939819767688,17.3853094561641));
#50692=CARTESIAN_POINT('Ctrl Pts',(-6.00000347488293,10.032698310508,17.1045694621537));
#50693=CARTESIAN_POINT('Ctrl Pts',(-6.00000357361913,10.0293041517828,17.1065440873071));
#50694=CARTESIAN_POINT('Ctrl Pts',(-6.0000056648664,9.9541574005552,17.150247947096));
#50695=CARTESIAN_POINT('Ctrl Pts',(-6.0000056648664,9.87547170337378,17.1956771555442));
#50696=CARTESIAN_POINT('Ctrl Pts',(-6.00000357361913,9.80004967494153,17.2389042212267));
#50697=CARTESIAN_POINT('Ctrl Pts',(-6.00000347488293,9.79664252003297,17.2408563363307));
#50698=CARTESIAN_POINT('Ctrl Pts',(-5.9999999999769,9.91330295482226,16.8993622715434));
#50699=CARTESIAN_POINT('Ctrl Pts',(-5.99999999996752,9.90992861632677,16.9013253647289));
#50700=CARTESIAN_POINT('Ctrl Pts',(-5.99999999976692,9.83522068214671,16.9447739934753));
#50701=CARTESIAN_POINT('Ctrl Pts',(-5.99999999976692,9.75699439892178,16.9899379591503));
#50702=CARTESIAN_POINT('Ctrl Pts',(-5.99999999996752,9.68201281558242,17.0329126136427));
#50703=CARTESIAN_POINT('Ctrl Pts',(-5.9999999999769,9.67862555776604,17.0348533299082));
#50704=CARTESIAN_POINT('Origin',(-5.47627002207303,-8.61187340852115,-14.9162298767998));
#50705=CARTESIAN_POINT('Ctrl Pts',(-5.67764080609729,10.3018641582453,17.1369991243702));
#50706=CARTESIAN_POINT('Ctrl Pts',(-3.78509387073152,11.0754256155854,16.6434327621663));
#50707=CARTESIAN_POINT('Ctrl Pts',(-2.06625885672274E-10,11.8428793690334,
16.139965968215));
#50708=CARTESIAN_POINT('Ctrl Pts',(3.78509387031849,11.0754256156717,16.6434327621122));
#50709=CARTESIAN_POINT('Ctrl Pts',(5.67764080547772,10.3018641584994,17.1369991242081));
#50710=CARTESIAN_POINT('Ctrl Pts',(-5.67764080609729,10.1072228441386,17.2516559727875));
#50711=CARTESIAN_POINT('Ctrl Pts',(-3.78509387073152,10.3777222791838,17.0590267241778));
#50712=CARTESIAN_POINT('Ctrl Pts',(-2.06625885672274E-10,10.7263798579245,
16.9926767289465));
#50713=CARTESIAN_POINT('Ctrl Pts',(3.78509387031849,10.3777222792149,17.0590267241666));
#50714=CARTESIAN_POINT('Ctrl Pts',(5.67764080547772,10.1072228442253,17.2516559727239));
#50715=CARTESIAN_POINT('Ctrl Pts',(-5.67764080609729,9.91156711681775,17.3647101833925));
#50716=CARTESIAN_POINT('Ctrl Pts',(-3.78509387073152,9.67398347124902,17.4658476572635));
#50717=CARTESIAN_POINT('Ctrl Pts',(-2.06625885672274E-10,9.51038903349187,
17.703153565319));
#50718=CARTESIAN_POINT('Ctrl Pts',(3.78509387031849,9.67398347122895,17.4658476572803));
#50719=CARTESIAN_POINT('Ctrl Pts',(5.67764080547772,9.9115671167385,17.3647101834302));
#50720=CARTESIAN_POINT('Ctrl Pts',(-5.67764080609729,9.71502525886082,17.476087692197));
#50721=CARTESIAN_POINT('Ctrl Pts',(-3.78509387073152,8.96560581046126,17.8630892232464));
#50722=CARTESIAN_POINT('Ctrl Pts',(-2.06625885672274E-10,8.21991077201455,
18.2569604826357));
#50723=CARTESIAN_POINT('Ctrl Pts',(3.78509387031849,8.9656058103827,17.8630892232866));
#50724=CARTESIAN_POINT('Ctrl Pts',(5.67764080547772,9.71502525861462,17.4760876923232));
#50725=CARTESIAN_POINT('Ctrl Pts',(-5.59336169625725,10.1144356127312,17.2450590604929));
#50726=CARTESIAN_POINT('Ctrl Pts',(-5.58009644052922,10.1196464220428,17.2417725309575));
#50727=CARTESIAN_POINT('Ctrl Pts',(-5.56074614028905,10.1272433830581,17.2369826570738));
#50728=CARTESIAN_POINT('Ctrl Pts',(-5.5352745867697,10.1371658803818,17.230732297382));
#50729=CARTESIAN_POINT('Ctrl Pts',(-5.50989210967062,10.1470536777985,17.2245037957864));
#50730=CARTESIAN_POINT('Ctrl Pts',(-5.47843096196783,10.1592509013913,17.2168250726809));
#50731=CARTESIAN_POINT('Ctrl Pts',(-5.44083463512139,10.173657996845,17.20776445536));
#50732=CARTESIAN_POINT('Ctrl Pts',(-5.41345000605419,10.1841519200026,17.2011648307354));
#50733=CARTESIAN_POINT('Ctrl Pts',(-5.38280993445691,10.1958174830056,17.1938325924219));
#50734=CARTESIAN_POINT('Ctrl Pts',(-5.34888648441894,10.2086021906203,17.1858024957018));
#50735=CARTESIAN_POINT('Ctrl Pts',(-5.30328426186975,10.2257882693128,17.1750078902796));
#50736=CARTESIAN_POINT('Ctrl Pts',(-5.25174934345171,10.2449983658296,17.1629512115716));
#50737=CARTESIAN_POINT('Ctrl Pts',(-5.19419938890525,10.2660693387113,17.1497389007395));
#50738=CARTESIAN_POINT('Ctrl Pts',(-5.15774847940527,10.2794152419642,17.1413705058342));
#50739=CARTESIAN_POINT('Ctrl Pts',(-5.11888420999868,10.2935068469148,17.1325389958659));
#50740=CARTESIAN_POINT('Ctrl Pts',(-5.07758279459578,10.3082935510227,17.1232765115135));
#50741=CARTESIAN_POINT('Ctrl Pts',(-5.01428717611989,10.330954604466,17.1090814852658));
#50742=CARTESIAN_POINT('Ctrl Pts',(-4.94526809232021,10.3552503413877,17.0938729633411));
#50743=CARTESIAN_POINT('Ctrl Pts',(-4.87042927208283,10.3809642545926,17.077788318177));
#50744=CARTESIAN_POINT('Ctrl Pts',(-4.84061551893453,10.3912079791507,17.0713806324482));
#50745=CARTESIAN_POINT('Ctrl Pts',(-4.80987804824268,10.4016762852682,17.064834182456));
#50746=CARTESIAN_POINT('Ctrl Pts',(-4.77821033099659,10.412353497345,17.0581587754218));
#50747=CARTESIAN_POINT('Ctrl Pts',(-4.70107154407374,10.4383619140844,17.0418982790671));
#50748=CARTESIAN_POINT('Ctrl Pts',(-4.61841362703178,10.4656129205248,17.0248708085413));
#50749=CARTESIAN_POINT('Ctrl Pts',(-4.53013604596957,10.4938502952785,17.0072373680404));
#50750=CARTESIAN_POINT('Ctrl Pts',(-4.5029336634511,10.5025515290473,17.0018036940787));
#50751=CARTESIAN_POINT('Ctrl Pts',(-4.47519762107238,10.5113461063362,16.9963126659037));
#50752=CARTESIAN_POINT('Ctrl Pts',(-4.44692485278666,10.5202256645349,16.9907694986755));
#50753=CARTESIAN_POINT('Ctrl Pts',(-4.35781685157385,10.5482115934237,16.9732989578675));
#50754=CARTESIAN_POINT('Ctrl Pts',(-4.26337760064318,10.5770449555143,16.9553085241858));
#50755=CARTESIAN_POINT('Ctrl Pts',(-4.16350896194574,10.6064361864374,16.9369795343976));
#50756=CARTESIAN_POINT('Ctrl Pts',(-4.13544397238834,10.6146956821079,16.9318287391759));
#50757=CARTESIAN_POINT('Ctrl Pts',(-4.10695019584106,10.6229989651231,16.9266513682192));
#50758=CARTESIAN_POINT('Ctrl Pts',(-4.07802541751535,10.6313389654857,16.9214518301025));
#50759=CARTESIAN_POINT('Ctrl Pts',(-3.98974865386987,10.6567921680142,16.9055831381382));
#50760=CARTESIAN_POINT('Ctrl Pts',(-3.89745734345782,10.6825893275272,16.8895067819342));
#50761=CARTESIAN_POINT('Ctrl Pts',(-3.80108980519495,10.7085129050089,16.8733587990892));
#50762=CARTESIAN_POINT('Ctrl Pts',(-3.75649682711523,10.7205087445128,16.865886504393));
#50763=CARTESIAN_POINT('Ctrl Pts',(-3.71103102545146,10.7325312845965,16.8583990963389));
#50764=CARTESIAN_POINT('Ctrl Pts',(-3.66468636943619,10.744556982028,16.8509112588752));
#50765=CARTESIAN_POINT('Ctrl Pts',(-3.62924738986443,10.7537528307461,16.8451854354097));
#50766=CARTESIAN_POINT('Ctrl Pts',(-3.59329450802114,10.7629504997334,16.8394593763233));
#50767=CARTESIAN_POINT('Ctrl Pts',(-3.55682518416501,10.7721390106437,16.8337399403038));
#50768=CARTESIAN_POINT('Ctrl Pts',(-3.51474448759309,10.7827413168748,16.8271404800932));
#50769=CARTESIAN_POINT('Ctrl Pts',(-3.47197612996742,10.793331619192,16.8205497196155));
#50770=CARTESIAN_POINT('Ctrl Pts',(-3.42851638099064,10.8038920970697,16.8139787813401));
#50771=CARTESIAN_POINT('Ctrl Pts',(-3.40678650650224,10.8091723360085,16.8106933122025));
#50772=CARTESIAN_POINT('Ctrl Pts',(-3.38488378417552,10.8144451187503,16.807412798479));
#50773=CARTESIAN_POINT('Ctrl Pts',(-3.36280774501983,10.8197081683452,16.8041386601616));
#50774=CARTESIAN_POINT('Ctrl Pts',(-3.35176972544199,10.8223396931427,16.8025015910029));
#50775=CARTESIAN_POINT('Ctrl Pts',(-3.34068837665689,10.824968784646,16.8008661156837));
#50776=CARTESIAN_POINT('Ctrl Pts',(-3.329563641285,10.8275951534672,16.7992324146027));
#50777=CARTESIAN_POINT('Ctrl Pts',(-3.32400127359906,10.8289083378778,16.7984155640621));
#50778=CARTESIAN_POINT('Ctrl Pts',(-3.31842805926641,10.8302208416174,16.7975991570803));
#50779=CARTESIAN_POINT('Ctrl Pts',(-3.31284399116671,10.8315326281783,16.7967832164111));
#50780=CARTESIAN_POINT('Ctrl Pts',(-3.30725992306701,10.8328444147391,16.7959672757419));
#50781=CARTESIAN_POINT('Ctrl Pts',(-3.30284643875128,10.8338793307461,16.7953235622363));
#50782=CARTESIAN_POINT('Ctrl Pts',(-3.29605921846272,10.8354657997138,16.7943368161553));
#50783=CARTESIAN_POINT('Ctrl Pts',(-3.26420947511142,10.8429104718047,16.7897064066363));
#50784=CARTESIAN_POINT('Ctrl Pts',(-3.23246236016097,10.8502239577099,16.7851582556376));
#50785=CARTESIAN_POINT('Ctrl Pts',(-3.20081930670522,10.8574079585424,16.7806912635389));
#50786=CARTESIAN_POINT('Ctrl Pts',(-3.02528053486219,10.8972609608712,16.7559107755265));
#50787=CARTESIAN_POINT('Ctrl Pts',(-2.85294730102254,10.9331280561869,16.7336284739108));
#50788=CARTESIAN_POINT('Ctrl Pts',(-2.68405734170938,10.965319242956,16.7136456366304));
#50789=CARTESIAN_POINT('Ctrl Pts',(-2.50183512068232,11.000051618844,16.6920853437245));
#50790=CARTESIAN_POINT('Ctrl Pts',(-2.32362196374915,11.0305054291441,16.673201482853));
#50791=CARTESIAN_POINT('Ctrl Pts',(-2.14968414968948,11.0570992276331,16.6567269918556));
#50792=CARTESIAN_POINT('Ctrl Pts',(-2.13682519185225,11.0590652666761,16.6555090578125));
#50793=CARTESIAN_POINT('Ctrl Pts',(-2.12398957734927,11.0610102121526,16.6543042908842));
#50794=CARTESIAN_POINT('Ctrl Pts',(-2.11117740281031,11.0629342344934,16.6531125827101));
#50795=CARTESIAN_POINT('Ctrl Pts',(-1.93621865371079,11.0892080368811,16.6368390164403));
#50796=CARTESIAN_POINT('Ctrl Pts',(-1.76563532274712,11.1115805033522,16.6230001913334));
#50797=CARTESIAN_POINT('Ctrl Pts',(-1.59966047058675,11.1305046374962,16.611306904573));
#50798=CARTESIAN_POINT('Ctrl Pts',(-1.55744727000663,11.1353177056208,16.608332893432));
#50799=CARTESIAN_POINT('Ctrl Pts',(-1.51553191253223,11.1399076896846,16.6054976961029));
#50800=CARTESIAN_POINT('Ctrl Pts',(-1.4739177101694,11.144281984227,16.6027966142496));
#50801=CARTESIAN_POINT('Ctrl Pts',(-1.30946665141412,11.1615683270611,16.592122475486));
#50802=CARTESIAN_POINT('Ctrl Pts',(-1.14972249376552,11.1754876800011,16.5835416973234));
#50803=CARTESIAN_POINT('Ctrl Pts',(-0.994867947072776,11.1865094923556,
16.5767553295172));
#50804=CARTESIAN_POINT('Ctrl Pts',(-0.92299758165632,11.1916248841758,16.5736056723421));
#50805=CARTESIAN_POINT('Ctrl Pts',(-0.852179763570651,11.1961158964594,
16.5708427266013));
#50806=CARTESIAN_POINT('Ctrl Pts',(-0.782429370895834,11.2000281392655,
16.5684376238844));
#50807=CARTESIAN_POINT('Ctrl Pts',(-0.63313574563942,11.2084018973047,16.5632897460024));
#50808=CARTESIAN_POINT('Ctrl Pts',(-0.488734980008948,11.2141260764705,
16.5597796943306));
#50809=CARTESIAN_POINT('Ctrl Pts',(-0.349348861740403,11.217649377585,16.5576195692001));
#50810=CARTESIAN_POINT('Ctrl Pts',(-0.262235556568476,11.219851364476,16.5562695377763));
#50811=CARTESIAN_POINT('Ctrl Pts',(-0.177080119921806,11.2211931540916,
16.5554472184677));
#50812=CARTESIAN_POINT('Ctrl Pts',(-0.0939047510573158,11.2217787688429,
16.5550866247168));
#50813=CARTESIAN_POINT('Ctrl Pts',(0.0408608595924439,11.2227276162076,
16.5545023695735));
#50814=CARTESIAN_POINT('Ctrl Pts',(0.170426606793054,11.2216933965749,16.5551294163659));
#50815=CARTESIAN_POINT('Ctrl Pts',(0.294722175599717,11.2191050882499,16.5567121120903));
#50816=CARTESIAN_POINT('Ctrl Pts',(0.343048653829801,11.2180987464541,16.5573274687857));
#50817=CARTESIAN_POINT('Ctrl Pts',(0.39057881329367,11.2168570902673,16.5580874888303));
#50818=CARTESIAN_POINT('Ctrl Pts',(0.437309818782762,11.2154038620237,16.5589779158886));
#50819=CARTESIAN_POINT('Ctrl Pts',(0.473889189930983,11.2142663265752,16.5596749105606));
#50820=CARTESIAN_POINT('Ctrl Pts',(0.509978917654201,11.2129991403243,16.5604518167948));
#50821=CARTESIAN_POINT('Ctrl Pts',(0.54557792579095,11.2116133394693,16.5613019839969));
#50822=CARTESIAN_POINT('Ctrl Pts',(0.57526124286935,11.2104578250789,16.562010874046));
#50823=CARTESIAN_POINT('Ctrl Pts',(0.604603386602295,11.2092198383741,16.5627707017228));
#50824=CARTESIAN_POINT('Ctrl Pts',(0.63360395775032,11.2079057382371,16.5635776247857));
#50825=CARTESIAN_POINT('Ctrl Pts',(0.66549434102706,11.2064606923165,16.5644649550944));
#50826=CARTESIAN_POINT('Ctrl Pts',(0.696971607506147,11.2049236195612,16.565409227215));
#50827=CARTESIAN_POINT('Ctrl Pts',(0.72803544167861,11.2033027340259,16.566405465553));
#50828=CARTESIAN_POINT('Ctrl Pts',(0.743567358764841,11.2024922912583,16.5669035847219));
#50829=CARTESIAN_POINT('Ctrl Pts',(0.758995917773488,11.2016608950771,16.5674146951219));
#50830=CARTESIAN_POINT('Ctrl Pts',(0.774321073540383,11.2008095475201,16.5679381887524));
#50831=CARTESIAN_POINT('Ctrl Pts',(0.78198365142383,11.2003838737417,16.5681999355677));
#50832=CARTESIAN_POINT('Ctrl Pts',(0.789620378496776,11.1999532121061,16.5684647781712));
#50833=CARTESIAN_POINT('Ctrl Pts',(0.797231250412047,11.1995176869327,16.568732641022));
#50834=CARTESIAN_POINT('Ctrl Pts',(0.804842122327319,11.1990821617592,16.5690005038728));
#50835=CARTESIAN_POINT('Ctrl Pts',(0.814188517455632,11.1985380526612,16.5693351922555));
#50836=CARTESIAN_POINT('Ctrl Pts',(0.819986296560143,11.1981966446342,16.5695452149902));
#50837=CARTESIAN_POINT('Ctrl Pts',(0.912968818906988,11.1927212757168,16.572913477781));
#50838=CARTESIAN_POINT('Ctrl Pts',(1.01085354095602,11.1860331615183,16.5770308029976));
#50839=CARTESIAN_POINT('Ctrl Pts',(1.11358303372777,11.1778352860948,16.582083555389));
#50840=CARTESIAN_POINT('Ctrl Pts',(1.22623354122959,11.1688457077178,16.587624273111));
#50841=CARTESIAN_POINT('Ctrl Pts',(1.34471056847521,11.1580407498769,16.594289802264));
#50842=CARTESIAN_POINT('Ctrl Pts',(1.46890926180699,11.1450008094671,16.6023433050796));
#50843=CARTESIAN_POINT('Ctrl Pts',(1.5153838009226,11.1401213280138,16.6053568861534));
#50844=CARTESIAN_POINT('Ctrl Pts',(1.56265915901644,11.1349285741414,16.6085650327152));
#50845=CARTESIAN_POINT('Ctrl Pts',(1.61072854597778,11.1293994266995,16.6119823022452));
#50846=CARTESIAN_POINT('Ctrl Pts',(1.74017461065096,11.1145099841127,16.6211846682527));
#50847=CARTESIAN_POINT('Ctrl Pts',(1.87538177215511,11.0971828232636,16.6319023435538));
#50848=CARTESIAN_POINT('Ctrl Pts',(2.01619359516505,11.0769554205139,16.6444269216333));
#50849=CARTESIAN_POINT('Ctrl Pts',(2.02948594729991,11.0750459944843,16.6456092165473));
#50850=CARTESIAN_POINT('Ctrl Pts',(2.04282821055348,11.073110706827,16.6468076250757));
#50851=CARTESIAN_POINT('Ctrl Pts',(2.05622023291824,11.0711491577268,16.6480224000727));
#50852=CARTESIAN_POINT('Ctrl Pts',(2.18611588770076,11.0521231512119,16.6598050860141));
#50853=CARTESIAN_POINT('Ctrl Pts',(2.32069562423643,11.0306273685102,16.6731268726598));
#50854=CARTESIAN_POINT('Ctrl Pts',(2.45980641009447,11.0062966218195,16.6882185446969));
#50855=CARTESIAN_POINT('Ctrl Pts',(2.57751721923923,10.9857087726287,16.7009886035811));
#50856=CARTESIAN_POINT('Ctrl Pts',(2.69847171418945,10.9630906897146,16.7150261711485));
#50857=CARTESIAN_POINT('Ctrl Pts',(2.8225610436928,10.9382204193277,16.7304718941296));
#50858=CARTESIAN_POINT('Ctrl Pts',(2.92925609545944,10.9168363503106,16.7437525059247));
#50859=CARTESIAN_POINT('Ctrl Pts',(3.0382684385968,10.8937870905112,16.7580742686304));
#50860=CARTESIAN_POINT('Ctrl Pts',(3.14952010302847,10.8689331626843,16.773525861029));
#50861=CARTESIAN_POINT('Ctrl Pts',(3.24640822738952,10.8472880892155,16.7869825208781));
#50862=CARTESIAN_POINT('Ctrl Pts',(3.3449946083139,10.8242742071437,16.8012961393943));
#50863=CARTESIAN_POINT('Ctrl Pts',(3.44522290323984,10.7998013031438,16.8165243674134));
#50864=CARTESIAN_POINT('Ctrl Pts',(3.44872500220626,10.7989461900056,16.8170564602885));
#50865=CARTESIAN_POINT('Ctrl Pts',(3.45222910514424,10.7980892956838,16.8175896697499));
#50866=CARTESIAN_POINT('Ctrl Pts',(3.45573520958506,10.7972306164005,16.8181239982249));
#50867=CARTESIAN_POINT('Ctrl Pts',(3.53381527626721,10.7781080440915,16.8300233593707));
#50868=CARTESIAN_POINT('Ctrl Pts',(3.61288815689678,10.7581001783265,16.8424777122093));
#50869=CARTESIAN_POINT('Ctrl Pts',(3.69292540360855,10.7371656451114,16.8555137028688));
#50870=CARTESIAN_POINT('Ctrl Pts',(3.69954958158591,10.7354330258674,16.8565926095752));
#50871=CARTESIAN_POINT('Ctrl Pts',(3.70618036529556,10.7336940593849,16.8576755002928));
#50872=CARTESIAN_POINT('Ctrl Pts',(3.71281773766541,10.7319487224599,16.8587623900056));
#50873=CARTESIAN_POINT('Ctrl Pts',(3.74627869988891,10.7231499614955,16.8642417233314));
#50874=CARTESIAN_POINT('Ctrl Pts',(3.77990711605412,10.7141892955713,16.8698226908658));
#50875=CARTESIAN_POINT('Ctrl Pts',(3.81370081314067,10.7050637966849,16.875507197817));
#50876=CARTESIAN_POINT('Ctrl Pts',(3.83394934879054,10.6995959726392,16.8789132454405));
#50877=CARTESIAN_POINT('Ctrl Pts',(3.85425722354602,10.6940689701107,16.8823564659578));
#50878=CARTESIAN_POINT('Ctrl Pts',(3.8746239679551,10.6884821641204,16.8858372669345));
#50879=CARTESIAN_POINT('Ctrl Pts',(3.88480734015964,10.6856887611252,16.8875776674229));
#50880=CARTESIAN_POINT('Ctrl Pts',(3.89500542977759,10.6828804072687,16.8893274630326));
#50881=CARTESIAN_POINT('Ctrl Pts',(3.90521817699174,10.6800570246534,16.8910867046236));
#50882=CARTESIAN_POINT('Ctrl Pts',(3.91032455059882,10.6786453333457,16.8919663254192));
#50883=CARTESIAN_POINT('Ctrl Pts',(3.91543458860496,10.6772298848486,16.8928483077104));
#50884=CARTESIAN_POINT('Ctrl Pts',(3.92054828348311,10.675810669452,16.8937326578414));
#50885=CARTESIAN_POINT('Ctrl Pts',(3.92566197836127,10.6743914540554,16.8946170079723));
#50886=CARTESIAN_POINT('Ctrl Pts',(3.93254611569438,10.6724762287361,16.895810469717));
#50887=CARTESIAN_POINT('Ctrl Pts',(3.93590033118955,10.6715417128619,16.8963928180947));
#50888=CARTESIAN_POINT('Ctrl Pts',(3.94215184180214,10.6697999834134,16.8974781857667));
#50889=CARTESIAN_POINT('Ctrl Pts',(3.94838636554841,10.6680589024911,16.8985631804318));
#50890=CARTESIAN_POINT('Ctrl Pts',(3.95460391944251,10.6663185318536,16.8996477635096));
#50891=CARTESIAN_POINT('Ctrl Pts',(4.02981766553141,10.6452652691942,16.9127679644141));
#50892=CARTESIAN_POINT('Ctrl Pts',(4.10254807846764,10.6243167745196,16.9258274386836));
#50893=CARTESIAN_POINT('Ctrl Pts',(4.17282587990966,10.6035771746011,16.9387612046173));
#50894=CARTESIAN_POINT('Ctrl Pts',(4.24075388489511,10.5835310203709,16.9512625193824));
#50895=CARTESIAN_POINT('Ctrl Pts',(4.30639057590207,10.5636799432642,16.9636464456261));
#50896=CARTESIAN_POINT('Ctrl Pts',(4.36976383142682,10.5441095500937,16.9758595468081));
#50897=CARTESIAN_POINT('Ctrl Pts',(4.43121450937757,10.5251328710808,16.9877021346836));
#50898=CARTESIAN_POINT('Ctrl Pts',(4.4905370197739,10.5064200395023,16.9993841484537));
#50899=CARTESIAN_POINT('Ctrl Pts',(4.54775645034366,10.4880420601335,17.010861252205));
#50900=CARTESIAN_POINT('Ctrl Pts',(4.60351117571902,10.4701345209906,17.022044564611));
#50901=CARTESIAN_POINT('Ctrl Pts',(4.65726912320849,10.4525448611279,17.0330333575748));
#50902=CARTESIAN_POINT('Ctrl Pts',(4.70905288634901,10.4353327752034,17.0437903335549));
#50903=CARTESIAN_POINT('Ctrl Pts',(4.75987167753236,10.4184414303612,17.0543468571241));
#50904=CARTESIAN_POINT('Ctrl Pts',(4.80878918164385,10.401913682668,17.0646801492342));
#50905=CARTESIAN_POINT('Ctrl Pts',(4.85582595139816,10.3858007083745,17.0747581939838));
#50906=CARTESIAN_POINT('Ctrl Pts',(4.90207917597453,10.3699561462908,17.0846683572354));
#50907=CARTESIAN_POINT('Ctrl Pts',(4.94651380654213,10.3545126244029,17.0943317286087));
#50908=CARTESIAN_POINT('Ctrl Pts',(4.98914847135176,10.339514167028,17.103720703033));
#50909=CARTESIAN_POINT('Ctrl Pts',(4.98949673383339,10.339391651699,17.1037973971397));
#50910=CARTESIAN_POINT('Ctrl Pts',(4.9898448762078,10.3392691660419,17.1038740729512));
#50911=CARTESIAN_POINT('Ctrl Pts',(4.99019289848491,10.3391467100793,17.103950730453));
#50912=CARTESIAN_POINT('Ctrl Pts',(5.03325928084211,10.3239932683266,17.1134367935652));
#50913=CARTESIAN_POINT('Ctrl Pts',(5.07448668094134,10.3092949186304,17.122642277991));
#50914=CARTESIAN_POINT('Ctrl Pts',(5.11389326224849,10.2950925682147,17.1315414279138));
#50915=CARTESIAN_POINT('Ctrl Pts',(5.15369851217184,10.2807465354191,17.1405306087824));
#50916=CARTESIAN_POINT('Ctrl Pts',(5.19164591938828,10.2669065813742,17.1492072354232));
#50917=CARTESIAN_POINT('Ctrl Pts',(5.22775300182795,10.2536103929835,17.1575474221413));
#50918=CARTESIAN_POINT('Ctrl Pts',(5.2645392540316,10.2400641049303,17.1660444867422));
#50919=CARTESIAN_POINT('Ctrl Pts',(5.2994153039346,10.2270822307516,17.1741923411339));
#50920=CARTESIAN_POINT('Ctrl Pts',(5.33239832281596,10.2147000575187,17.1819683887808));
#50921=CARTESIAN_POINT('Ctrl Pts',(5.36641335057651,10.2019304572657,17.1899877419372));
#50922=CARTESIAN_POINT('Ctrl Pts',(5.39841504349945,10.1897986823172,17.1976116558626));
#50923=CARTESIAN_POINT('Ctrl Pts',(5.42842066614186,10.1783385418951,17.2048181455367));
#50924=CARTESIAN_POINT('Ctrl Pts',(5.45996866099105,10.1662893184773,17.2123950687631));
#50925=CARTESIAN_POINT('Ctrl Pts',(5.4893101307546,10.1549825787082,17.2195105357911));
#50926=CARTESIAN_POINT('Ctrl Pts',(5.51646318129051,10.1444519643233,17.2261421901412));
#50927=CARTESIAN_POINT('Ctrl Pts',(5.54440810081889,10.1336142438549,17.2329672445457));
#50928=CARTESIAN_POINT('Ctrl Pts',(5.57003513091122,10.1235985826726,17.2392798431885));
#50929=CARTESIAN_POINT('Ctrl Pts',(5.5933616601283,10.1144355424442,17.2450591004647));
#50930=CARTESIAN_POINT('Ctrl Pts',(-5.8463733010073,10.2457285249441,16.949086006428));
#50931=CARTESIAN_POINT('Ctrl Pts',(-5.81071183845632,10.2597918252233,16.9400660732668));
#50932=CARTESIAN_POINT('Ctrl Pts',(-5.69191996054832,10.3062057866106,16.9103322240196));
#50933=CARTESIAN_POINT('Ctrl Pts',(-5.48049741245665,10.38625136138,16.8592278496599));
#50934=CARTESIAN_POINT('Ctrl Pts',(-5.20215554396402,10.4866532305168,16.7953196613188));
#50935=CARTESIAN_POINT('Ctrl Pts',(-4.8941493129655,10.5916725641874,16.7286085483737));
#50936=CARTESIAN_POINT('Ctrl Pts',(-4.55276913235771,10.7006290440657,16.6595003165788));
#50937=CARTESIAN_POINT('Ctrl Pts',(-4.17238356880022,10.8128325911058,16.5884207304473));
#50938=CARTESIAN_POINT('Ctrl Pts',(-3.74657439469726,10.9269282942293,16.5162276658936));
#50939=CARTESIAN_POINT('Ctrl Pts',(-3.27003381845878,11.040174418721,16.4446648480292));
#50940=CARTESIAN_POINT('Ctrl Pts',(-2.7386885358987,11.1484347150953,16.3763620028265));
#50941=CARTESIAN_POINT('Ctrl Pts',(-2.14775624702771,11.2465694809231,16.3145802149633));
#50942=CARTESIAN_POINT('Ctrl Pts',(-1.49664356863671,11.3274377514689,16.2638265111147));
#50943=CARTESIAN_POINT('Ctrl Pts',(-0.805427675793565,11.3814836225517,
16.2300643076986));
#50944=CARTESIAN_POINT('Ctrl Pts',(-0.113326822037204,11.4024992910628,
16.2170495538243));
#50945=CARTESIAN_POINT('Ctrl Pts',(0.53617904501584,11.3923351802427,16.2233294580765));
#50946=CARTESIAN_POINT('Ctrl Pts',(1.11984701048415,11.3587959812637,16.2442251910393));
#50947=CARTESIAN_POINT('Ctrl Pts',(1.63691896299704,11.3100216749588,16.2747552179192));
#50948=CARTESIAN_POINT('Ctrl Pts',(2.09763398174282,11.251537564875,16.3114723839704));
#50949=CARTESIAN_POINT('Ctrl Pts',(2.51226399840957,11.1867259151241,16.352250871855));
#50950=CARTESIAN_POINT('Ctrl Pts',(2.88624760864777,11.1183574017561,16.3953378720742));
#50951=CARTESIAN_POINT('Ctrl Pts',(3.22326429257175,11.0487107246453,16.4392863234276));
#50952=CARTESIAN_POINT('Ctrl Pts',(3.5276819915208,10.9792486772936,16.4831632372597));
#50953=CARTESIAN_POINT('Ctrl Pts',(3.80292724584096,10.9110843998516,16.5262573892699));
#50954=CARTESIAN_POINT('Ctrl Pts',(4.05164145117326,10.8451121085737,16.567997008493));
#50955=CARTESIAN_POINT('Ctrl Pts',(4.27616841465673,10.7819862052094,16.6079630105325));
#50956=CARTESIAN_POINT('Ctrl Pts',(4.47886355109388,10.7220901690397,16.6459087067021));
#50957=CARTESIAN_POINT('Ctrl Pts',(4.66208312275494,10.665574932594,16.6817355221251));
#50958=CARTESIAN_POINT('Ctrl Pts',(4.82814550061594,10.6124043230814,16.7154642022297));
#50959=CARTESIAN_POINT('Ctrl Pts',(4.97929162609239,10.5623996874633,16.7472065332161));
#50960=CARTESIAN_POINT('Ctrl Pts',(5.11758619996814,10.5153019885475,16.7771259862501));
#50961=CARTESIAN_POINT('Ctrl Pts',(5.24463111730424,10.4709008672825,16.8053557320035));
#50962=CARTESIAN_POINT('Ctrl Pts',(5.36151871454931,10.4290880708158,16.8319644193218));
#50963=CARTESIAN_POINT('Ctrl Pts',(5.46895006319928,10.3898443662126,16.8569640935366));
#50964=CARTESIAN_POINT('Ctrl Pts',(5.56756311190895,10.3531353396374,16.8803762516901));
#50965=CARTESIAN_POINT('Ctrl Pts',(5.65800137336307,10.3188910900565,16.9022446821647));
#50966=CARTESIAN_POINT('Ctrl Pts',(5.74091079056104,10.2870108104913,16.9226324749478));
#50967=CARTESIAN_POINT('Ctrl Pts',(5.80284291074193,10.2628628056022,16.9380991790113));
#50968=CARTESIAN_POINT('Ctrl Pts',(5.83721317799972,10.2493407521394,16.9467699786851));
#50969=CARTESIAN_POINT('Ctrl Pts',(5.8463475785683,10.2457385387449,16.9490805710439));
#50970=CARTESIAN_POINT('Ctrl Pts',(-5.81214048410627,10.2495588935256,17.0923498933693));
#50971=CARTESIAN_POINT('Ctrl Pts',(-5.77669382793542,10.2635850491913,17.0833822545817));
#50972=CARTESIAN_POINT('Ctrl Pts',(-5.65860909322797,10.3098800300599,17.0538187973008));
#50973=CARTESIAN_POINT('Ctrl Pts',(-5.44840462333573,10.3897376720867,17.0029977853316));
#50974=CARTESIAN_POINT('Ctrl Pts',(-5.17162939485601,10.4899212401681,16.9394359874193));
#50975=CARTESIAN_POINT('Ctrl Pts',(-4.86534603850363,10.5947210968573,16.8730845645311));
#50976=CARTESIAN_POINT('Ctrl Pts',(-4.52588138421029,10.7034540320265,16.8043505326476));
#50977=CARTESIAN_POINT('Ctrl Pts',(-4.14764846583199,10.8154286837038,16.7336596024664));
#50978=CARTESIAN_POINT('Ctrl Pts',(-3.72427691755522,10.9292912020793,16.6618663983565));
#50979=CARTESIAN_POINT('Ctrl Pts',(-3.25050020753745,11.0423043121599,16.590705725778));
#50980=CARTESIAN_POINT('Ctrl Pts',(-2.72227770251836,11.15033962184,16.522792381771));
#50981=CARTESIAN_POINT('Ctrl Pts',(-2.13486068559317,11.2482679994735,16.4613676733713));
#50982=CARTESIAN_POINT('Ctrl Pts',(-1.48765672131871,11.3289640567501,16.4109103803494));
#50983=CARTESIAN_POINT('Ctrl Pts',(-0.800609992132193,11.3828936033401,
16.3773462735944));
#50984=CARTESIAN_POINT('Ctrl Pts',(-0.112656412763598,11.4038639976422,
16.3644072235699));
#50985=CARTESIAN_POINT('Ctrl Pts',(0.532982300217447,11.3937217510365,16.3706507298466));
#50986=CARTESIAN_POINT('Ctrl Pts',(1.11313112312745,11.3602548559676,16.3914240619341));
#50987=CARTESIAN_POINT('Ctrl Pts',(1.62709005444509,11.3115851034049,16.4217752045558));
#50988=CARTESIAN_POINT('Ctrl Pts',(2.08504101968106,11.2532253592082,16.458278206289));
#50989=CARTESIAN_POINT('Ctrl Pts',(2.49719897986104,11.1885503635626,16.4988204899594));
#50990=CARTESIAN_POINT('Ctrl Pts',(2.86896944948211,11.1203248275706,16.5416599927212));
#50991=CARTESIAN_POINT('Ctrl Pts',(3.20400785780452,11.0508227302716,16.585358255767));
#50992=CARTESIAN_POINT('Ctrl Pts',(3.50665331436974,10.9815039732325,16.6289876548034));
#50993=CARTESIAN_POINT('Ctrl Pts',(3.78030901480038,10.913479603221,16.6718408587469));
#50994=CARTESIAN_POINT('Ctrl Pts',(4.02759771527588,10.8476422395178,16.713349047024));
#50995=CARTESIAN_POINT('Ctrl Pts',(4.25084657567494,10.7846452014045,16.7530951266326));
#50996=CARTESIAN_POINT('Ctrl Pts',(4.45239467779643,10.7248714440366,16.7908333899151));
#50997=CARTESIAN_POINT('Ctrl Pts',(4.63458237830649,10.6684718441651,16.8264654138834));
#50998=CARTESIAN_POINT('Ctrl Pts',(4.79971278139797,10.6154105462015,16.8600114553183));
#50999=CARTESIAN_POINT('Ctrl Pts',(4.95001237250278,10.5655095013055,16.8915823408029));
#51000=CARTESIAN_POINT('Ctrl Pts',(5.08753268216066,10.5185104478698,16.9213403268495));
#51001=CARTESIAN_POINT('Ctrl Pts',(5.21386523142879,10.4742037174266,16.9494175499695));
#51002=CARTESIAN_POINT('Ctrl Pts',(5.33009497893724,10.432481545317,16.9758819840215));
#51003=CARTESIAN_POINT('Ctrl Pts',(5.43691796894504,10.3933249838663,17.0007453247105));
#51004=CARTESIAN_POINT('Ctrl Pts',(5.53496769036703,10.3566998929772,17.0240287063314));
#51005=CARTESIAN_POINT('Ctrl Pts',(5.62488345963333,10.3225366416241,17.0457754968935));
#51006=CARTESIAN_POINT('Ctrl Pts',(5.7073074330221,10.2907346235822,17.0660483615429));
#51007=CARTESIAN_POINT('Ctrl Pts',(5.76887172101577,10.2666481665187,17.0814266234462));
#51008=CARTESIAN_POINT('Ctrl Pts',(5.8030360081916,10.25316138296,17.0900473914712));
#51009=CARTESIAN_POINT('Ctrl Pts',(5.81211556016687,10.2495686125498,17.0923446256674));
#51010=CARTESIAN_POINT('Ctrl Pts',(-5.75637626233754,10.1837201417723,17.2118536969054));
#51011=CARTESIAN_POINT('Ctrl Pts',(-5.72124177183205,10.1976628995511,17.2029857527102));
#51012=CARTESIAN_POINT('Ctrl Pts',(-5.60419197535415,10.2436849161472,17.1737500606415));
#51013=CARTESIAN_POINT('Ctrl Pts',(-5.39580847211975,10.3230818240993,17.1234891203679));
#51014=CARTESIAN_POINT('Ctrl Pts',(-5.12142638366231,10.422693332199,17.0606301153465));
#51015=CARTESIAN_POINT('Ctrl Pts',(-4.81781612208664,10.5268917270792,16.9950214475401));
#51016=CARTESIAN_POINT('Ctrl Pts',(-4.4813608879283,10.6349920036448,16.9270704092175));
#51017=CARTESIAN_POINT('Ctrl Pts',(-4.10654736969582,10.746302542252,16.8572016117894));
#51018=CARTESIAN_POINT('Ctrl Pts',(-3.6870885478391,10.8594742827435,16.7862625466688));
#51019=CARTESIAN_POINT('Ctrl Pts',(-3.21779412721873,10.9717844531648,16.7159688619445));
#51020=CARTESIAN_POINT('Ctrl Pts',(-2.69468813604672,11.0791301006442,16.6489027355764));
#51021=CARTESIAN_POINT('Ctrl Pts',(-2.11308889884579,11.1764171542247,16.5882613465945));
#51022=CARTESIAN_POINT('Ctrl Pts',(-1.47241765961012,11.2565721948536,16.5384595621686));
#51023=CARTESIAN_POINT('Ctrl Pts',(-0.792400884630377,11.3101333762541,
16.5053368948279));
#51024=CARTESIAN_POINT('Ctrl Pts',(-0.111506716586297,11.3309592637304,
16.4925680681425));
#51025=CARTESIAN_POINT('Ctrl Pts',(0.527523869479962,11.3208869439873,16.4987295537772));
#51026=CARTESIAN_POINT('Ctrl Pts',(1.1017189194122,11.2876496094038,16.5192293101599));
#51027=CARTESIAN_POINT('Ctrl Pts',(1.61044309404501,11.2393099586255,16.5491830326528));
#51028=CARTESIAN_POINT('Ctrl Pts',(2.06377799636403,11.1813404285803,16.5852128420941));
#51029=CARTESIAN_POINT('Ctrl Pts',(2.471835069819,11.1170910356783,16.6252361147083));
#51030=CARTESIAN_POINT('Ctrl Pts',(2.8399587584862,11.049307038833,16.6675348168625));
#51031=CARTESIAN_POINT('Ctrl Pts',(3.17175878031802,10.9802473078334,16.7106894353203));
#51032=CARTESIAN_POINT('Ctrl Pts',(3.47152170733553,10.9113626526124,16.7537839684948));
#51033=CARTESIAN_POINT('Ctrl Pts',(3.74260813031438,10.8437577418764,16.7961193514205));
#51034=CARTESIAN_POINT('Ctrl Pts',(3.98760666094978,10.7783205269083,16.8371328805859));
#51035=CARTESIAN_POINT('Ctrl Pts',(4.2088142490919,10.715701342194,16.8764114516135));
#51036=CARTESIAN_POINT('Ctrl Pts',(4.40854095591408,10.6562818812914,16.9137111633865));
#51037=CARTESIAN_POINT('Ctrl Pts',(4.58909944985825,10.6002131348132,16.948933651213));
#51038=CARTESIAN_POINT('Ctrl Pts',(4.75276676007855,10.5474603926735,16.9820979165458));
#51039=CARTESIAN_POINT('Ctrl Pts',(4.9017451190426,10.4978474838834,17.0133125992741));
#51040=CARTESIAN_POINT('Ctrl Pts',(5.03806430892174,10.4511183877206,17.0427373075265));
#51041=CARTESIAN_POINT('Ctrl Pts',(5.16329886926211,10.4070653142114,17.0705019749049));
#51042=CARTESIAN_POINT('Ctrl Pts',(5.27852170413661,10.3655817362365,17.0966731628961));
#51043=CARTESIAN_POINT('Ctrl Pts',(5.38442057509479,10.3266493824282,17.1212618367615));
#51044=CARTESIAN_POINT('Ctrl Pts',(5.48162162178821,10.2902348018342,17.1442883625899));
#51045=CARTESIAN_POINT('Ctrl Pts',(5.57075720609127,10.2562691463666,17.1657951865642));
#51046=CARTESIAN_POINT('Ctrl Pts',(5.65246304775603,10.22465260939,17.1858439664136));
#51047=CARTESIAN_POINT('Ctrl Pts',(5.71348822191349,10.2007079571406,17.2010518028893));
#51048=CARTESIAN_POINT('Ctrl Pts',(5.74735238451962,10.1873010376137,17.2095768782592));
#51049=CARTESIAN_POINT('Ctrl Pts',(5.75635212911942,10.1837295664958,17.2118486069642));
#51050=CARTESIAN_POINT('Ctrl Pts',(-5.69417655262727,10.0659550938109,17.2751196141304));
#51051=CARTESIAN_POINT('Ctrl Pts',(-5.65936703870486,10.0797907515111,17.2663717926203));
#51052=CARTESIAN_POINT('Ctrl Pts',(-5.54339967722055,10.1254596259212,17.2375325657588));
#51053=CARTESIAN_POINT('Ctrl Pts',(-5.33694689371025,10.2042475512871,17.1879568994398));
#51054=CARTESIAN_POINT('Ctrl Pts',(-5.06513642187847,10.3030878613366,17.1259669913686));
#51055=CARTESIAN_POINT('Ctrl Pts',(-4.76442569371336,10.4064653591534,17.0612832475125));
#51056=CARTESIAN_POINT('Ctrl Pts',(-4.43125897055681,10.5136948306663,16.9943122258059));
#51057=CARTESIAN_POINT('Ctrl Pts',(-4.06020584535738,10.6240854956199,16.9254766893615));
#51058=CARTESIAN_POINT('Ctrl Pts',(-3.64507557266572,10.7362955187036,16.8556150441424));
#51059=CARTESIAN_POINT('Ctrl Pts',(-3.18076844304463,10.8476227562837,16.7864187240801));
#51060=CARTESIAN_POINT('Ctrl Pts',(-2.66338764499731,10.954000403985,16.7204284189311));
#51061=CARTESIAN_POINT('Ctrl Pts',(-2.0883338678018,11.0503844700961,16.660784761969));
#51062=CARTESIAN_POINT('Ctrl Pts',(-1.45505107693594,11.1297758587313,16.6118203238809));
#51063=CARTESIAN_POINT('Ctrl Pts',(-0.783022235707487,11.1828161548434,
16.5792630691678));
#51064=CARTESIAN_POINT('Ctrl Pts',(-0.110188903191932,11.2034373433835,
16.5667129564925));
#51065=CARTESIAN_POINT('Ctrl Pts',(0.521281123172272,11.1934641215224,16.5727689772592));
#51066=CARTESIAN_POINT('Ctrl Pts',(1.08869926730035,11.160551584388,16.5929179599979));
#51067=CARTESIAN_POINT('Ctrl Pts',(1.59148386671455,11.1126783998152,16.6223631937593));
#51068=CARTESIAN_POINT('Ctrl Pts',(2.03960018326053,11.0552595066297,16.6577887420727));
#51069=CARTESIAN_POINT('Ctrl Pts',(2.44303760716516,10.9916096766539,16.6971505484544));
#51070=CARTESIAN_POINT('Ctrl Pts',(2.80706804716866,10.9244464844029,16.7387613933694));
#51071=CARTESIAN_POINT('Ctrl Pts',(3.13524621666746,10.8560073839613,16.7812259290856));
#51072=CARTESIAN_POINT('Ctrl Pts',(3.4317966606496,10.7877303502555,16.8236428919148));
#51073=CARTESIAN_POINT('Ctrl Pts',(3.7000296333615,10.7207111125095,16.8653236203182));
#51074=CARTESIAN_POINT('Ctrl Pts',(3.94249333601839,10.6558311443833,16.9057130400457));
#51075=CARTESIAN_POINT('Ctrl Pts',(4.1614491203754,10.5937366998712,16.9444029536336));
#51076=CARTESIAN_POINT('Ctrl Pts',(4.35917319283043,10.5348078145404,16.9811516032074));
#51077=CARTESIAN_POINT('Ctrl Pts',(4.53794624447247,10.4791957319084,17.0158605727866));
#51078=CARTESIAN_POINT('Ctrl Pts',(4.70001547858034,10.4268674063087,17.0485471811394));
#51079=CARTESIAN_POINT('Ctrl Pts',(4.84755564240603,10.3776493108809,17.0793172456371));
#51080=CARTESIAN_POINT('Ctrl Pts',(4.98257207879255,10.3312885255543,17.108327008496));
#51081=CARTESIAN_POINT('Ctrl Pts',(5.10662033523898,10.2875798190821,17.1357036274334));
#51082=CARTESIAN_POINT('Ctrl Pts',(5.22075984776427,10.2464183166914,17.1615118961645));
#51083=CARTESIAN_POINT('Ctrl Pts',(5.32566908184452,10.2077866315443,17.1857618662613));
#51084=CARTESIAN_POINT('Ctrl Pts',(5.42196592776539,10.171652230936,17.2084729378999));
#51085=CARTESIAN_POINT('Ctrl Pts',(5.51027491708016,10.1379473510794,17.2296863832694));
#51086=CARTESIAN_POINT('Ctrl Pts',(5.59122442533868,10.1065733678469,17.249462542477));
#51087=CARTESIAN_POINT('Ctrl Pts',(5.65168521434887,10.082812435781,17.2644640766896));
#51088=CARTESIAN_POINT('Ctrl Pts',(5.68523639401818,10.0695083794281,17.2728736875046));
#51089=CARTESIAN_POINT('Ctrl Pts',(5.69415298772929,10.0659643045932,17.2751146638057));
#51090=CARTESIAN_POINT('Ctrl Pts',(-5.73644387793316,10.2877346863031,16.9337810350644));
#51091=CARTESIAN_POINT('Ctrl Pts',(-5.66411037901632,10.3157397302585,16.9158630923735));
#51092=CARTESIAN_POINT('Ctrl Pts',(-5.58548128436389,10.345652422121,16.8967577750015));
#51093=CARTESIAN_POINT('Ctrl Pts',(-5.50055659235639,10.3771725884928,16.8766547495792));
#51094=CARTESIAN_POINT('Ctrl Pts',(-5.41741952890743,10.4080292688012,16.8569748842709));
#51095=CARTESIAN_POINT('Ctrl Pts',(-5.32824911790177,10.4404263047604,16.8363389710469));
#51096=CARTESIAN_POINT('Ctrl Pts',(-5.23304535782008,10.4740375249085,16.8149530194337));
#51097=CARTESIAN_POINT('Ctrl Pts',(-5.13477096437687,10.5087328170914,16.7928773007731));
#51098=CARTESIAN_POINT('Ctrl Pts',(-5.03006775494901,10.544722138694,16.7700022177755));
#51099=CARTESIAN_POINT('Ctrl Pts',(-4.91893572786536,10.5815974241754,16.7465854223469));
#51100=CARTESIAN_POINT('Ctrl Pts',(-4.80780370078171,10.6184727096568,16.7231686269183));
#51101=CARTESIAN_POINT('Ctrl Pts',(-4.69024285604226,10.6562339622146,16.699210116964));
#51102=CARTESIAN_POINT('Ctrl Pts',(-4.56625319197586,10.6944229852801,16.6749991241893));
#51103=CARTESIAN_POINT('Ctrl Pts',(-4.44622762213337,10.7313910607216,16.6515621851015));
#51104=CARTESIAN_POINT('Ctrl Pts',(-4.32017773748643,10.7687597473468,16.6278888032932));
#51105=CARTESIAN_POINT('Ctrl Pts',(-4.18810353803503,10.8060686117601,16.6042695666098));
#51106=CARTESIAN_POINT('Ctrl Pts',(-4.05161768088946,10.8446236994286,16.579861379566));
#51107=CARTESIAN_POINT('Ctrl Pts',(-3.90869832845551,10.8831151723678,16.5555108443855));
#51108=CARTESIAN_POINT('Ctrl Pts',(-3.75934548073319,10.9209853985322,16.5315698407257));
#51109=CARTESIAN_POINT('Ctrl Pts',(-3.60999263301087,10.9588556246966,16.5076288370659));
#51110=CARTESIAN_POINT('Ctrl Pts',(-3.45420629000018,10.9961046088078,16.4840973614737));
#51111=CARTESIAN_POINT('Ctrl Pts',(-3.29198645170111,11.0321243382672,16.4613590428076));
#51112=CARTESIAN_POINT('Ctrl Pts',(-3.21175044287551,11.0499401575966,16.4501123792904));
#51113=CARTESIAN_POINT('Ctrl Pts',(-3.12994053214575,11.0674544734859,16.4390602443938));
#51114=CARTESIAN_POINT('Ctrl Pts',(-3.04655672419778,11.0845891516794,16.428251951463));
#51115=CARTESIAN_POINT('Ctrl Pts',(-3.00486482022379,11.0931564907761,16.4228478049976));
#51116=CARTESIAN_POINT('Ctrl Pts',(-2.9627794332184,11.1016288762653,16.4175046172165));
#51117=CARTESIAN_POINT('Ctrl Pts',(-2.92030057443875,11.1099962543511,16.4122287688642));
#51118=CARTESIAN_POINT('Ctrl Pts',(-2.89906114504893,11.1141799433939,16.4095908446881));
#51119=CARTESIAN_POINT('Ctrl Pts',(-2.87772334714861,11.1183373778354,16.4069697552516));
#51120=CARTESIAN_POINT('Ctrl Pts',(-2.85628718059005,11.1224672837817,16.4043663037934));
#51121=CARTESIAN_POINT('Ctrl Pts',(-2.84556909731076,11.1245322367549,16.4030645780643));
#51122=CARTESIAN_POINT('Ctrl Pts',(-2.83482642183447,11.1265903074306,16.4017672618231));
#51123=CARTESIAN_POINT('Ctrl Pts',(-2.82405915415227,11.128641335461,16.4004744562027));
#51124=CARTESIAN_POINT('Ctrl Pts',(-2.81867552031118,11.1296668494762,16.3998280533925));
#51125=CARTESIAN_POINT('Ctrl Pts',(-2.81328573841659,11.1306906028192,16.399182778237));
#51126=CARTESIAN_POINT('Ctrl Pts',(-2.80788980846857,11.131712575377,16.3985386434259));
#51127=CARTESIAN_POINT('Ctrl Pts',(-2.80249387852054,11.1327345479348,16.3978945086147));
#51128=CARTESIAN_POINT('Ctrl Pts',(-2.79531885000099,11.1340885934571,16.3970411026223));
#51129=CARTESIAN_POINT('Ctrl Pts',(-2.79168357446015,11.1347731305368,16.3966096727281));
#51130=CARTESIAN_POINT('Ctrl Pts',(-2.04577399270848,11.2752309200605,16.3080860688738));
#51131=CARTESIAN_POINT('Ctrl Pts',(-1.29987672192816,11.3594145287903,16.2552346233375));
#51132=CARTESIAN_POINT('Ctrl Pts',(-0.553962161422298,11.3872886566001,
16.2380598751199));
#51133=CARTESIAN_POINT('Ctrl Pts',(-0.369309316851761,11.3941889602844,
16.2338082271684));
#51134=CARTESIAN_POINT('Ctrl Pts',(-0.184655412730056,11.3976383199709,
16.2317430976133));
#51135=CARTESIAN_POINT('Ctrl Pts',(1.07492380563405E-12,11.3976358484824,
16.2318648996165));
#51136=CARTESIAN_POINT('Ctrl Pts',(6.93460617175366E-5,11.3976358475542,
16.2318649453584));
#51137=CARTESIAN_POINT('Ctrl Pts',(0.000138692122572115,11.3976358461392,
16.2318649914088));
#51138=CARTESIAN_POINT('Ctrl Pts',(0.000208038183639729,11.3976358442374,
16.2318650377675));
#51139=CARTESIAN_POINT('Ctrl Pts',(0.465532887795667,11.397623082842,16.2321761135824));
#51140=CARTESIAN_POINT('Ctrl Pts',(0.93085773638585,11.3756953661397,16.2460734179067));
#51141=CARTESIAN_POINT('Ctrl Pts',(1.39618258395421,11.3318637068722,16.2735530077344));
#51142=CARTESIAN_POINT('Ctrl Pts',(1.62884500773839,11.3099478772385,16.2872928026482));
#51143=CARTESIAN_POINT('Ctrl Pts',(1.86150743137387,11.2825562791905,16.304427889156));
#51144=CARTESIAN_POINT('Ctrl Pts',(2.09416985349857,11.2496916138933,16.3249560837549));
#51145=CARTESIAN_POINT('Ctrl Pts',(2.21050106456092,11.2332592812448,16.3352201810544));
#51146=CARTESIAN_POINT('Ctrl Pts',(2.32683227716226,11.2154586948964,16.3463325557894));
#51147=CARTESIAN_POINT('Ctrl Pts',(2.44316348898306,11.1962902777384,16.3582928083244));
#51148=CARTESIAN_POINT('Ctrl Pts',(2.50132909489346,11.1867060691593,16.3642729345919));
#51149=CARTESIAN_POINT('Ctrl Pts',(2.55949470071167,11.1767799037176,16.3704650303328));
#51150=CARTESIAN_POINT('Ctrl Pts',(2.61766030645565,11.1665118394568,16.3768690421441));
#51151=CARTESIAN_POINT('Ctrl Pts',(2.64674310932764,11.1613778073265,16.3800710480498));
#51152=CARTESIAN_POINT('Ctrl Pts',(2.6758259121901,11.1561583005427,16.3833260329749));
#51153=CARTESIAN_POINT('Ctrl Pts',(2.70490871504478,11.1508533266947,16.3866339898157));
#51154=CARTESIAN_POINT('Ctrl Pts',(2.73217384272104,11.1458799137123,16.3897351993539));
#51155=CARTESIAN_POINT('Ctrl Pts',(2.75943897039075,11.1408313831947,16.3928829662399));
#51156=CARTESIAN_POINT('Ctrl Pts',(2.78670409806019,11.135707741571,16.3960772844348));
#51157=CARTESIAN_POINT('Ctrl Pts',(2.78852177323815,11.1353661654627,16.3962902389811));
#51158=CARTESIAN_POINT('Ctrl Pts',(2.7917217802675,11.1347639810534,16.3966656658502));
#51159=CARTESIAN_POINT('Ctrl Pts',(2.79215712359383,11.1346820117671,16.396716768754));
#51160=CARTESIAN_POINT('Ctrl Pts',(2.80635022328155,11.1320096422105,16.398382829915));
#51161=CARTESIAN_POINT('Ctrl Pts',(2.82656862381981,11.1281855968624,16.4007798930427));
#51162=CARTESIAN_POINT('Ctrl Pts',(2.85281232520862,11.1231359515119,16.4039546435487));
#51163=CARTESIAN_POINT('Ctrl Pts',(2.87905632057885,11.1180862495954,16.4071294296181));
#51164=CARTESIAN_POINT('Ctrl Pts',(2.91132575179097,11.1118109200526,16.4110819203721));
#51165=CARTESIAN_POINT('Ctrl Pts',(2.94962061884499,11.1041919647284,16.4158866461266));
#51166=CARTESIAN_POINT('Ctrl Pts',(2.98791593921205,11.0965729192152,16.4206914287567));
#51167=CARTESIAN_POINT('Ctrl Pts',(3.03223683807327,11.0876102158814,16.4263484663581));
#51168=CARTESIAN_POINT('Ctrl Pts',(3.08258331542866,11.0771417830772,16.4329601381591));
#51169=CARTESIAN_POINT('Ctrl Pts',(3.13293077927501,11.0666731451541,16.4395719395095));
#51170=CARTESIAN_POINT('Ctrl Pts',(3.18930405774871,11.0546987185142,16.4471384121424));
#51171=CARTESIAN_POINT('Ctrl Pts',(3.25170315084976,11.0410123546368,16.455789792554));
#51172=CARTESIAN_POINT('Ctrl Pts',(3.31410294885478,11.0273258361485,16.4644412706976));
#51173=CARTESIAN_POINT('Ctrl Pts',(3.38252869763159,11.0119273413779,16.4741776807566));
#51174=CARTESIAN_POINT('Ctrl Pts',(3.45698039718018,10.9945666515411,16.4851571204632));
#51175=CARTESIAN_POINT('Ctrl Pts',(3.53143351514183,10.9772056309579,16.4961367693441));
#51176=CARTESIAN_POINT('Ctrl Pts',(3.61191281348369,10.957882340169,16.5083594947387));
#51177=CARTESIAN_POINT('Ctrl Pts',(3.69841829220576,10.9363024868442,16.5220112677421));
#51178=CARTESIAN_POINT('Ctrl Pts',(3.77371777394213,10.9175181069955,16.533894577876));
#51179=CARTESIAN_POINT('Ctrl Pts',(3.85358328686691,10.8970232575265,16.5468611021372));
#51180=CARTESIAN_POINT('Ctrl Pts',(3.9380148309801,10.8745966667332,16.5610506886561));
#51181=CARTESIAN_POINT('Ctrl Pts',(3.98561399049141,10.8619534433541,16.5690502153639));
#51182=CARTESIAN_POINT('Ctrl Pts',(4.03466435231841,10.8486958059363,16.5774387518806));
#51183=CARTESIAN_POINT('Ctrl Pts',(4.08516592204748,10.8347805625576,16.5862436136911));
#51184=CARTESIAN_POINT('Ctrl Pts',(4.11041670691202,10.8278229408682,16.5906460445963));
#51185=CARTESIAN_POINT('Ctrl Pts',(4.13603028420328,10.820700881924,16.5951525547403));
#51186=CARTESIAN_POINT('Ctrl Pts',(4.16200666602408,10.8134087423863,16.5997667430059));
#51187=CARTESIAN_POINT('Ctrl Pts',(4.17499485693448,10.8097626726174,16.6020738371387));
#51188=CARTESIAN_POINT('Ctrl Pts',(4.18807374838966,10.8060740804569,16.6044078506744));
#51189=CARTESIAN_POINT('Ctrl Pts',(4.20124334024048,10.8023422462392,16.6067692381573));
#51190=CARTESIAN_POINT('Ctrl Pts',(4.2078281361659,10.8004763291304,16.6079499318988));
#51191=CARTESIAN_POINT('Ctrl Pts',(4.21443560715221,10.7985996013682,16.6091374691186));
#51192=CARTESIAN_POINT('Ctrl Pts',(4.22106575320089,10.7967119720507,16.6103319072856));
#51193=CARTESIAN_POINT('Ctrl Pts',(4.22769589924957,10.7948243427332,16.6115263454525));
#51194=CARTESIAN_POINT('Ctrl Pts',(4.23593743780306,10.7924713596529,16.6130152502058));
#51195=CARTESIAN_POINT('Ctrl Pts',(4.2410242164579,10.7910162879412,16.6139359822734));
#51196=CARTESIAN_POINT('Ctrl Pts',(4.3703949964166,10.7540098099686,16.6373527325978));
#51197=CARTESIAN_POINT('Ctrl Pts',(4.49373992023327,10.7170369625673,16.6607652887357));
#51198=CARTESIAN_POINT('Ctrl Pts',(4.61105898920646,10.6805483865231,16.6838892449829));
#51199=CARTESIAN_POINT('Ctrl Pts',(4.72934236899263,10.6437598905363,16.707203269914));
#51200=CARTESIAN_POINT('Ctrl Pts',(4.84150042710314,10.6074637179565,16.7302238946238));
#51201=CARTESIAN_POINT('Ctrl Pts',(4.94753316486883,10.5720763462447,16.7526882263514));
#51202=CARTESIAN_POINT('Ctrl Pts',(5.0527582749985,10.5369585122244,16.7749814522913));
#51203=CARTESIAN_POINT('Ctrl Pts',(5.15195101980991,10.5027356280522,16.7967268648974));
#51204=CARTESIAN_POINT('Ctrl Pts',(5.2451114006037,10.4697704218163,16.8176954447603));
#51205=CARTESIAN_POINT('Ctrl Pts',(5.33934432336991,10.4364256919352,16.8389054328465));
#51206=CARTESIAN_POINT('Ctrl Pts',(5.42740518308715,10.4043678502821,16.8593205447843));
#51207=CARTESIAN_POINT('Ctrl Pts',(5.50929398110152,10.3739263971821,16.8787326755966));
#51208=CARTESIAN_POINT('Ctrl Pts',(5.59118277911589,10.3434849440822,16.8981448064088));
#51209=CARTESIAN_POINT('Ctrl Pts',(5.66689951542738,10.3146598775781,16.9165539572384));
#51210=CARTESIAN_POINT('Ctrl Pts',(5.73644419138209,10.2877345675704,16.9337810842153));
#51211=CARTESIAN_POINT('Ctrl Pts',(-5.843530343931,6.40544352337877,7.94861259136425));
#51212=CARTESIAN_POINT('Ctrl Pts',(-3.895686895954,7.5011174617541,7.93455912692836));
#51213=CARTESIAN_POINT('Ctrl Pts',(0.0001666015277053,8.59741135523303,
7.91991927812663));
#51214=CARTESIAN_POINT('Ctrl Pts',(3.896020099009,7.50102369434968,7.93456037909693));
#51215=CARTESIAN_POINT('Ctrl Pts',(5.844030148514,6.40516236820509,7.94861619754387));
#51216=CARTESIAN_POINT('Ctrl Pts',(-5.843530343931,7.02207626292374,8.43809571307178));
#51217=CARTESIAN_POINT('Ctrl Pts',(-3.895686895954,8.04135143326013,8.43217787140772));
#51218=CARTESIAN_POINT('Ctrl Pts',(0.0001666015277053,9.06227985942128,
8.42460953303723));
#51219=CARTESIAN_POINT('Ctrl Pts',(3.896020099009,8.04126411194929,8.43217851873466));
#51220=CARTESIAN_POINT('Ctrl Pts',(5.844030148514,7.02181471204778,8.4380972315977));
#51221=CARTESIAN_POINT('Ctrl Pts',(-5.843530343931,8.22106606565346,9.63752218475374));
#51222=CARTESIAN_POINT('Ctrl Pts',(-3.895686895954,9.0918900806387,9.61305666122109));
#51223=CARTESIAN_POINT('Ctrl Pts',(0.0001666015277053,9.96180836750487,
9.58947319442851));
#51224=CARTESIAN_POINT('Ctrl Pts',(3.896020099009,9.09181567541838,9.61305867834303));
#51225=CARTESIAN_POINT('Ctrl Pts',(5.844030148514,8.22084260802873,9.63752846273313));
#51226=CARTESIAN_POINT('Ctrl Pts',(-5.843530343931,9.557830382581,11.8732201358499));
#51227=CARTESIAN_POINT('Ctrl Pts',(-3.895686895954,10.2763900681474,11.7328262526707));
#51228=CARTESIAN_POINT('Ctrl Pts',(0.0001666015277054,10.9955725683271,
11.5921560888775));
#51229=CARTESIAN_POINT('Ctrl Pts',(3.896020099009,10.2763285555535,11.7328382843686));
#51230=CARTESIAN_POINT('Ctrl Pts',(5.844030148514,9.55764599673119,11.8732561615899));
#51231=CARTESIAN_POINT('Ctrl Pts',(-5.843530343931,10.2973084060429,14.4766646280625));
#51232=CARTESIAN_POINT('Ctrl Pts',(-3.895686895954,10.972803840489,14.1582376025316));
#51233=CARTESIAN_POINT('Ctrl Pts',(0.0001666015277051,11.6469750209433,
13.8399443642564));
#51234=CARTESIAN_POINT('Ctrl Pts',(3.896020099009,10.9727461777759,14.1582648265603));
#51235=CARTESIAN_POINT('Ctrl Pts',(5.844030148514,10.2971350706646,14.4767463379645));
#51236=CARTESIAN_POINT('Ctrl Pts',(-5.843530343931,10.3258757620666,16.2770693368357));
#51237=CARTESIAN_POINT('Ctrl Pts',(-3.895686895954,11.0553896705852,15.8346874489017));
#51238=CARTESIAN_POINT('Ctrl Pts',(0.0001666015277058,11.7876699867244,
15.3921227606342));
#51239=CARTESIAN_POINT('Ctrl Pts',(3.896020099009,11.0553270377124,15.8347253020195));
#51240=CARTESIAN_POINT('Ctrl Pts',(5.844030148514,10.3256885653351,16.2771828541457));
#51241=CARTESIAN_POINT('Ctrl Pts',(-5.843530343931,10.2251611575698,17.159314850801));
#51242=CARTESIAN_POINT('Ctrl Pts',(-3.895686895954,11.0033631004084,16.661943431523));
#51243=CARTESIAN_POINT('Ctrl Pts',(0.0001666015277058,11.7816843623499,
16.1645455758364));
#51244=CARTESIAN_POINT('Ctrl Pts',(3.896020099009,11.0032965296051,16.6619859745965));
#51245=CARTESIAN_POINT('Ctrl Pts',(5.844030148514,10.2249614672313,17.1594424786931));
#51246=CARTESIAN_POINT('',(5.73278665926685,6.65588954520332,8.10254295276797));
#51247=CARTESIAN_POINT('Ctrl Pts',(5.73278665926685,6.65588954520332,8.10254295276797));
#51248=CARTESIAN_POINT('Ctrl Pts',(5.73375888620758,6.99202136443375,8.38525883796284));
#51249=CARTESIAN_POINT('Ctrl Pts',(5.73463611962229,7.31053409065034,8.68980953075562));
#51250=CARTESIAN_POINT('Ctrl Pts',(5.73539800543143,7.60866057961232,9.01380228009759));
#51251=CARTESIAN_POINT('Ctrl Pts',(5.7358525360122,7.78651873701786,9.20709189220604));
#51252=CARTESIAN_POINT('Ctrl Pts',(5.73626601263528,7.95712059774996,9.4073003281479));
#51253=CARTESIAN_POINT('Ctrl Pts',(5.73663411343628,8.1198745794402,9.61391171627937));
#51254=CARTESIAN_POINT('Ctrl Pts',(5.73680084043203,8.19359211099577,9.70749395227842));
#51255=CARTESIAN_POINT('Ctrl Pts',(5.73695825843206,8.26569958462528,9.80238969913112));
#51256=CARTESIAN_POINT('Ctrl Pts',(5.73710596584106,8.33615716844976,9.89853823864722));
#51257=CARTESIAN_POINT('Ctrl Pts',(5.73762707028046,8.5847280422313,10.2377455344846));
#51258=CARTESIAN_POINT('Ctrl Pts',(5.73808755028673,8.81277732605215,10.5925991843482));
#51259=CARTESIAN_POINT('Ctrl Pts',(5.7384511752828,9.01856735398873,10.9604768333983));
#51260=CARTESIAN_POINT('Ctrl Pts',(5.73875620561864,9.19119630418346,11.2690745482264));
#51261=CARTESIAN_POINT('Ctrl Pts',(5.73899308048749,9.34816097570251,11.5868367228597));
#51262=CARTESIAN_POINT('Ctrl Pts',(5.73914041321966,9.48841420861512,11.9121967999306));
#51263=CARTESIAN_POINT('Ctrl Pts',(5.73916137871713,9.50837229094943,11.9584956486033));
#51264=CARTESIAN_POINT('Ctrl Pts',(5.73918053104131,9.52799194545917,12.0049483191629));
#51265=CARTESIAN_POINT('Ctrl Pts',(5.73919780856664,9.54727141212101,12.0515497100057));
#51266=CARTESIAN_POINT('Ctrl Pts',(5.73934667546454,9.71338746988924,12.4530773803036));
#51267=CARTESIAN_POINT('Ctrl Pts',(5.73938505124021,9.85421925005767,12.8656005110965));
#51268=CARTESIAN_POINT('Ctrl Pts',(5.73932699215388,9.96862920325058,13.2858435141329));
#51269=CARTESIAN_POINT('Ctrl Pts',(5.73927451059684,10.0720482004273,13.665715271193));
#51270=CARTESIAN_POINT('Ctrl Pts',(5.73914323250993,10.1538778096344,14.0518946860673));
#51271=CARTESIAN_POINT('Ctrl Pts',(5.73894353985269,10.2132541970825,14.4419342915027));
#51272=CARTESIAN_POINT('Ctrl Pts',(5.73893603912074,10.215484456184,14.4565847176629));
#51273=CARTESIAN_POINT('Ctrl Pts',(5.7389283964977,10.2176830628771,14.4712406634984));
#51274=CARTESIAN_POINT('Ctrl Pts',(5.73892061255889,10.2198499690232,14.4859019942209));
#51275=CARTESIAN_POINT('Ctrl Pts',(5.73870205362586,10.2806927771524,14.897565662103));
#51276=CARTESIAN_POINT('Ctrl Pts',(5.73837208348003,10.3165409130782,15.3134787414899));
#51277=CARTESIAN_POINT('Ctrl Pts',(5.73794343795648,10.3271730562598,15.7305176790661));
#51278=CARTESIAN_POINT('Ctrl Pts',(5.73753129228904,10.3373959362556,16.1315035329577));
#51279=CARTESIAN_POINT('Ctrl Pts',(5.73702792165988,10.3243069727082,16.5335294805983));
#51280=CARTESIAN_POINT('Ctrl Pts',(5.73644464706835,10.2877344027066,16.9337810712876));
#51281=CARTESIAN_POINT('Ctrl Pts',(-5.7327897547535,6.65588713928974,8.10254235490551));
#51282=CARTESIAN_POINT('Ctrl Pts',(-5.37903306893985,6.85199393532157,8.1046567014769));
#51283=CARTESIAN_POINT('Ctrl Pts',(-5.01625135988035,7.03117595252705,8.1037396655483));
#51284=CARTESIAN_POINT('Ctrl Pts',(-4.6460573053147,7.19212481080525,8.10101244173934));
#51285=CARTESIAN_POINT('Ctrl Pts',(-4.37169929920774,7.31140713664976,8.098991243189));
#51286=CARTESIAN_POINT('Ctrl Pts',(-4.09327000298005,7.42067123776832,8.0959775624238));
#51287=CARTESIAN_POINT('Ctrl Pts',(-3.81142588255404,7.5194084477233,8.09248201619626));
#51288=CARTESIAN_POINT('Ctrl Pts',(-3.57233107521407,7.60316947901887,8.08951666446013));
#51289=CARTESIAN_POINT('Ctrl Pts',(-3.33077878398178,7.67935406186102,8.08620479042068));
#51290=CARTESIAN_POINT('Ctrl Pts',(-3.08716977929676,7.74769216833986,8.08286047253372));
#51291=CARTESIAN_POINT('Ctrl Pts',(-3.04361334355598,7.75991078212773,8.0822625202235));
#51292=CARTESIAN_POINT('Ctrl Pts',(-2.99999115841705,7.77187869233266,8.08166353316822));
#51293=CARTESIAN_POINT('Ctrl Pts',(-2.95630551460348,7.783594544369,8.08106530891504));
#51294=CARTESIAN_POINT('Ctrl Pts',(-2.75784036736928,7.83682000006536,8.07834755877739));
#51295=CARTESIAN_POINT('Ctrl Pts',(-2.55806426654974,7.88488745634565,8.07569240201061));
#51296=CARTESIAN_POINT('Ctrl Pts',(-2.35724376584312,7.92759984415222,8.07318988699391));
#51297=CARTESIAN_POINT('Ctrl Pts',(-2.16325032346373,7.96886018915527,8.07077244703639));
#51298=CARTESIAN_POINT('Ctrl Pts',(-1.96828228463633,8.00512331767119,8.06849745748605));
#51299=CARTESIAN_POINT('Ctrl Pts',(-1.77257993163001,8.03625973710509,8.06644561273015));
#51300=CARTESIAN_POINT('Ctrl Pts',(-1.57996180764706,8.06690545294229,8.0644261046276));
#51301=CARTESIAN_POINT('Ctrl Pts',(-1.38663233238503,8.09258461604006,8.06262277294384));
#51302=CARTESIAN_POINT('Ctrl Pts',(-1.19282060581187,8.11322305871492,8.06111193464765));
#51303=CARTESIAN_POINT('Ctrl Pts',(-0.994702314851606,8.13432009480826,
8.05956752499583));
#51304=CARTESIAN_POINT('Ctrl Pts',(-0.796080102885767,8.15014941282128,
8.05832876462942));
#51305=CARTESIAN_POINT('Ctrl Pts',(-0.59719868379037,8.16068915179076,8.05747633859425));
#51306=CARTESIAN_POINT('Ctrl Pts',(-0.408374169346901,8.17069592417969,
8.05666701747757));
#51307=CARTESIAN_POINT('Ctrl Pts',(-0.219315999797635,8.17593478931577,
8.0562059446956));
#51308=CARTESIAN_POINT('Ctrl Pts',(-0.0302336110270316,8.1764388741411,
8.05616136972021));
#51309=CARTESIAN_POINT('Ctrl Pts',(-0.0201629718368322,8.17646572199525,
8.05615899563082));
#51310=CARTESIAN_POINT('Ctrl Pts',(-0.0100922639442051,8.17647915107978,
8.05615780282402));
#51311=CARTESIAN_POINT('Ctrl Pts',(-2.15189915158098E-5,8.17647917058928,
8.05615780154597));
#51312=CARTESIAN_POINT('Ctrl Pts',(-1.43459939669992E-5,8.17647917060317,
8.05615780154506));
#51313=CARTESIAN_POINT('Ctrl Pts',(-7.17299643689954E-6,8.17647917061026,
8.05615780154476));
#51314=CARTESIAN_POINT('Ctrl Pts',(1.07469816165171E-12,8.17647917061055,
8.05615780154506));
#51315=CARTESIAN_POINT('Ctrl Pts',(0.18943579711537,8.17647917827287,8.05615780943295));
#51316=CARTESIAN_POINT('Ctrl Pts',(0.378858612885447,8.17173001867108,8.05657949522161));
#51317=CARTESIAN_POINT('Ctrl Pts',(0.568057836295289,8.16219561556172,8.05735427144708));
#51318=CARTESIAN_POINT('Ctrl Pts',(0.769443680254818,8.15204708650211,8.05817895223188));
#51319=CARTESIAN_POINT('Ctrl Pts',(0.970576200329105,8.13647662698269,8.05940367890533));
#51320=CARTESIAN_POINT('Ctrl Pts',(1.17120141047458,8.11550423737469,8.06094475234051));
#51321=CARTESIAN_POINT('Ctrl Pts',(1.36703229033906,8.09503302387756,8.06244899882344));
#51322=CARTESIAN_POINT('Ctrl Pts',(1.56237981688653,8.0694154937033,8.06425464009947));
#51323=CARTESIAN_POINT('Ctrl Pts',(1.75700778088661,8.03872640369093,8.06628301653371));
#51324=CARTESIAN_POINT('Ctrl Pts',(1.95878306564105,8.00691031853628,8.06838588101525));
#51325=CARTESIAN_POINT('Ctrl Pts',(2.15978496848557,7.96964334863419,8.07072813122281));
#51326=CARTESIAN_POINT('Ctrl Pts',(2.35975028992456,7.92706670092953,8.07322138619571));
#51327=CARTESIAN_POINT('Ctrl Pts',(2.55971561136355,7.88449005322488,8.0757146411686));
#51328=CARTESIAN_POINT('Ctrl Pts',(2.75864435139702,7.83660410476304,8.07835888608861));
#51329=CARTESIAN_POINT('Ctrl Pts',(2.95627331052934,7.783603529238,8.08106520728543));
#51330=CARTESIAN_POINT('Ctrl Pts',(3.19882930073948,7.71855432220565,8.08438675702491));
#51331=CARTESIAN_POINT('Ctrl Pts',(3.4394292441421,7.64573016185184,8.08773178925052));
#51332=CARTESIAN_POINT('Ctrl Pts',(3.67768100681231,7.56538588953542,8.09079284969756));
#51333=CARTESIAN_POINT('Ctrl Pts',(3.96257907131849,7.46931135300075,8.09445322218305));
#51334=CARTESIAN_POINT('Ctrl Pts',(4.24411946379384,7.36248453264372,8.09770721708057));
#51335=CARTESIAN_POINT('Ctrl Pts',(4.52163169077914,7.24541657642252,8.10003238704001));
#51336=CARTESIAN_POINT('Ctrl Pts',(4.88861255955403,7.09060645959825,8.10310718090057));
#51337=CARTESIAN_POINT('Ctrl Pts',(5.24854925703452,6.91789304800925,8.10455499757065));
#51338=CARTESIAN_POINT('Ctrl Pts',(5.5998912593694,6.72853477684402,8.10319558761065));
#51339=CARTESIAN_POINT('Ctrl Pts',(5.64432825807231,6.70458514032395,8.10302365229341));
#51340=CARTESIAN_POINT('Ctrl Pts',(5.68862777036575,6.68036922783882,8.10280688011413));
#51341=CARTESIAN_POINT('Ctrl Pts',(5.73278665919283,6.65588954516668,8.10254295270319));
#51342=CARTESIAN_POINT('Ctrl Pts',(-5.84424404754221,6.60982561991869,8.11494609712149));
#51343=CARTESIAN_POINT('Ctrl Pts',(-5.61083003141265,6.74470098061893,8.11886064004874));
#51344=CARTESIAN_POINT('Ctrl Pts',(-4.83877334320068,7.15840509626737,8.12664832309506));
#51345=CARTESIAN_POINT('Ctrl Pts',(-3.4739964644456,7.71340775361018,8.11883512382398));
#51346=CARTESIAN_POINT('Ctrl Pts',(-1.74184413166379,8.12609642238157,8.0994612827205));
#51347=CARTESIAN_POINT('Ctrl Pts',(0.00546389148000443,8.26248517348045,
8.09063507506571));
#51348=CARTESIAN_POINT('Ctrl Pts',(1.75277317531105,8.12437426464466,8.09956481566326));
#51349=CARTESIAN_POINT('Ctrl Pts',(3.48454184722242,7.71000021151431,8.11895024293463));
#51350=CARTESIAN_POINT('Ctrl Pts',(4.84546451123536,7.15511681611458,8.12662863672576));
#51351=CARTESIAN_POINT('Ctrl Pts',(5.61402512777244,6.74285772429285,8.11880770412169));
#51352=CARTESIAN_POINT('Ctrl Pts',(5.84435329640009,6.60976254643618,8.1149443088601));
#51353=CARTESIAN_POINT('Ctrl Pts',(-5.72536415493237,6.40694478209925,7.90745488128355));
#51354=CARTESIAN_POINT('Ctrl Pts',(-5.49665064991634,6.53847614205489,7.91194597692562));
#51355=CARTESIAN_POINT('Ctrl Pts',(-4.74015267330978,6.94198191326917,7.92158137971138));
#51356=CARTESIAN_POINT('Ctrl Pts',(-3.40298511486256,7.48347479664365,7.91659886786272));
#51357=CARTESIAN_POINT('Ctrl Pts',(-1.70614179652305,7.88616883277403,7.89960762793621));
#51358=CARTESIAN_POINT('Ctrl Pts',(0.0053517777339369,8.01925550389425,
7.89162120971071));
#51359=CARTESIAN_POINT('Ctrl Pts',(1.71684729000813,7.88448836413846,7.89970073156132));
#51360=CARTESIAN_POINT('Ctrl Pts',(3.41331638270933,7.48014986638464,7.91669525727088));
#51361=CARTESIAN_POINT('Ctrl Pts',(4.74670889513164,6.93877415913986,7.92154621389461));
#51362=CARTESIAN_POINT('Ctrl Pts',(5.4997813999677,6.53667859342793,7.91188514788741));
#51363=CARTESIAN_POINT('Ctrl Pts',(5.72547120249297,6.40688327557001,7.90745282059258));
#51364=CARTESIAN_POINT('Ctrl Pts',(-5.7194149784166,6.40360983160495,7.59392594682071));
#51365=CARTESIAN_POINT('Ctrl Pts',(-5.49136603844791,6.5337759497367,7.59841892092599));
#51366=CARTESIAN_POINT('Ctrl Pts',(-4.73696752025829,6.93323604774542,7.60809613134932));
#51367=CARTESIAN_POINT('Ctrl Pts',(-3.40255792642537,7.47005167289838,7.60327372800129));
#51368=CARTESIAN_POINT('Ctrl Pts',(-1.70680590972389,7.87002583666974,7.58642156961049));
#51369=CARTESIAN_POINT('Ctrl Pts',(0.00535495091468471,8.00237757076679,
7.5784734111445));
#51370=CARTESIAN_POINT('Ctrl Pts',(1.71751142262118,7.86835521722273,7.58651415030087));
#51371=CARTESIAN_POINT('Ctrl Pts',(3.41287492734901,7.46675197777174,7.60336893780237));
#51372=CARTESIAN_POINT('Ctrl Pts',(4.74350648116296,6.93005899438803,7.60806032165927));
#51373=CARTESIAN_POINT('Ctrl Pts',(5.49448772027338,6.53199702945591,7.5983580829355));
#51374=CARTESIAN_POINT('Ctrl Pts',(5.71952172603672,6.40354895607179,7.59392388778129));
#51375=CARTESIAN_POINT('Ctrl Pts',(-5.83025895397455,6.60198838021539,7.3778062669314));
#51376=CARTESIAN_POINT('Ctrl Pts',(-5.59840732478868,6.73365395594057,7.38172521605155));
#51377=CARTESIAN_POINT('Ctrl Pts',(-4.83128643333009,7.13784639841503,7.38961116079864));
#51378=CARTESIAN_POINT('Ctrl Pts',(-3.47299336195986,7.68185251078179,7.38217434496566));
#51379=CARTESIAN_POINT('Ctrl Pts',(-1.74340617768423,8.08814661704716,7.36312745843566));
#51380=CARTESIAN_POINT('Ctrl Pts',(0.0054713540043873,8.22280750341084,
7.35439118899612));
#51381=CARTESIAN_POINT('Ctrl Pts',(1.75433527096293,8.08644761515946,7.36322976207848));
#51382=CARTESIAN_POINT('Ctrl Pts',(3.48350520534007,7.67850429798651,7.38228669101555));
#51383=CARTESIAN_POINT('Ctrl Pts',(4.83793702132043,7.13463029795999,7.38958996088061));
#51384=CARTESIAN_POINT('Ctrl Pts',(5.60158110182676,6.73185449623961,7.38167225921689));
#51385=CARTESIAN_POINT('Ctrl Pts',(5.83036749767586,6.60192679025215,7.37780448255811));
#51386=CARTESIAN_POINT('Origin',(5.89878270283593,6.95921850207614,7.74135566505664));
#51387=CARTESIAN_POINT('Ctrl Pts',(5.71061633139555,6.68825430759423,8.1203063081284));
#51388=CARTESIAN_POINT('Ctrl Pts',(5.71571542223483,6.68567794625997,8.11996801621166));
#51389=CARTESIAN_POINT('Ctrl Pts',(5.76276700635191,6.66117775605966,8.11739155262433));
#51390=CARTESIAN_POINT('Ctrl Pts',(5.84736859742446,6.60432471294745,8.12235110026491));
#51391=CARTESIAN_POINT('Ctrl Pts',(5.94575166176578,6.50451738948382,8.15321624698963));
#51392=CARTESIAN_POINT('Ctrl Pts',(6.01456588634735,6.3959192625854,8.20362766067628));
#51393=CARTESIAN_POINT('Ctrl Pts',(6.04741736776337,6.29826329603432,8.26181413939222));
#51394=CARTESIAN_POINT('Ctrl Pts',(6.05207362756165,6.24151474090948,8.30216609769673));
#51395=CARTESIAN_POINT('Ctrl Pts',(6.05138819518176,6.21914710908527,8.31924280036705));
#51396=CARTESIAN_POINT('Ctrl Pts',(5.59392208653217,6.47899731163308,7.91253200724143));
#51397=CARTESIAN_POINT('Ctrl Pts',(5.59866955743605,6.47661703590363,7.91219372773975));
#51398=CARTESIAN_POINT('Ctrl Pts',(5.6424838618781,6.45398236827702,7.90956757196331));
#51399=CARTESIAN_POINT('Ctrl Pts',(5.72137642495094,6.40146868496194,7.91357340076122));
#51400=CARTESIAN_POINT('Ctrl Pts',(5.81312989580529,6.30944394505649,7.94114488602853));
#51401=CARTESIAN_POINT('Ctrl Pts',(5.87715279420531,6.20973494694733,7.98666537269705));
#51402=CARTESIAN_POINT('Ctrl Pts',(5.90753939606212,6.12074388781985,8.03925603483806));
#51403=CARTESIAN_POINT('Ctrl Pts',(5.91179865681948,6.06956203278856,8.07558361900822));
#51404=CARTESIAN_POINT('Ctrl Pts',(5.91117126135558,6.04949611706124,8.09091432397107));
#51405=CARTESIAN_POINT('Ctrl Pts',(5.57597263223173,6.48127925322056,7.59591028107758));
#51406=CARTESIAN_POINT('Ctrl Pts',(5.58273758482897,6.47792626708818,7.59545099347781));
#51407=CARTESIAN_POINT('Ctrl Pts',(5.64510830703547,6.44608460045405,7.5919303212076));
#51408=CARTESIAN_POINT('Ctrl Pts',(5.75644759897633,6.37296939409402,7.5981443156954));
#51409=CARTESIAN_POINT('Ctrl Pts',(5.88585584667335,6.24539458879271,7.63765045596241));
#51410=CARTESIAN_POINT('Ctrl Pts',(5.97748415205553,6.10548886830425,7.70282854503511));
#51411=CARTESIAN_POINT('Ctrl Pts',(6.02250848732848,5.976818340779,7.77966536946315));
#51412=CARTESIAN_POINT('Ctrl Pts',(6.02923395546078,5.89948703576177,7.834648132105));
#51413=CARTESIAN_POINT('Ctrl Pts',(6.02824683811861,5.868477692758,7.85831508294452));
#51414=CARTESIAN_POINT('Ctrl Pts',(5.66860840586943,6.69359454132171,7.37930452174859));
#51415=CARTESIAN_POINT('Ctrl Pts',(5.67842908309909,6.68874171019614,7.37868303011404));
#51416=CARTESIAN_POINT('Ctrl Pts',(5.76890893218883,6.64269404293812,7.37401309649988));
#51417=CARTESIAN_POINT('Ctrl Pts',(5.92944679261123,6.53762650096011,7.38414049452444));
#51418=CARTESIAN_POINT('Ctrl Pts',(6.11595471194353,6.3546200579059,7.44293675038479));
#51419=CARTESIAN_POINT('Ctrl Pts',(6.24937488282923,6.15194807007878,7.53935356989418));
#51420=CARTESIAN_POINT('Ctrl Pts',(6.31648358865281,5.96142879087898,7.65428422951676));
#51421=CARTESIAN_POINT('Ctrl Pts',(6.32691160405283,5.84348172036974,7.73829558507271));
#51422=CARTESIAN_POINT('Ctrl Pts',(6.3253843013646,5.79550278490975,7.77488190927595));
#51423=CARTESIAN_POINT('',(5.99999999999929,6.09544950676928,8.13560044756764));
#51424=CARTESIAN_POINT('Ctrl Pts',(5.99998827407956,6.09544950560664,8.13560044835052));
#51425=CARTESIAN_POINT('Ctrl Pts',(5.99998537178181,6.0985235188595,8.11167900213626));
#51426=CARTESIAN_POINT('Ctrl Pts',(5.99998616180659,6.1020672978436,8.08790876283193));
#51427=CARTESIAN_POINT('Ctrl Pts',(5.99999964263501,6.10614414461004,8.06438762436252));
#51428=CARTESIAN_POINT('Ctrl Pts',(6.00000808539942,6.10869738953676,8.04965682114416));
#51429=CARTESIAN_POINT('Ctrl Pts',(6.00002053204976,6.11145911940312,8.03502411123104));
#51430=CARTESIAN_POINT('Ctrl Pts',(6.00003309722689,6.11443703572943,8.02051631282948));
#51431=CARTESIAN_POINT('Ctrl Pts',(6.00005418885645,6.11943570048125,7.99616384199079));
#51432=CARTESIAN_POINT('Ctrl Pts',(6.00007686014713,6.12504607350498,7.97216315652948));
#51433=CARTESIAN_POINT('Ctrl Pts',(6.00009746231146,6.13126411378436,7.94863439925196));
#51434=CARTESIAN_POINT('Ctrl Pts',(6.00010841241073,6.13456901695795,7.93612880888857));
#51435=CARTESIAN_POINT('Ctrl Pts',(6.00011838637384,6.13804472091411,7.92375664857546));
#51436=CARTESIAN_POINT('Ctrl Pts',(6.00012560696237,6.14168481188013,7.91153595676546));
#51437=CARTESIAN_POINT('Ctrl Pts',(6.00013953874254,6.14870819328121,7.88795671647509));
#51438=CARTESIAN_POINT('Ctrl Pts',(6.0001421475481,6.15634660115405,7.86494246365324));
#51439=CARTESIAN_POINT('Ctrl Pts',(6.00012604298399,6.16451476811207,7.84261416200171));
#51440=CARTESIAN_POINT('Ctrl Pts',(6.00011913996253,6.16801595146733,7.83304341271422));
#51441=CARTESIAN_POINT('Ctrl Pts',(6.00010897012775,6.17161385499292,7.82359849664904));
#51442=CARTESIAN_POINT('Ctrl Pts',(6.00009598241838,6.17529925506742,7.81428784213583));
#51443=CARTESIAN_POINT('Ctrl Pts',(6.00009379118139,6.1759210417689,7.81271698387312));
#51444=CARTESIAN_POINT('Ctrl Pts',(6.00009152155428,6.17654531603784,7.8111499455311));
#51445=CARTESIAN_POINT('Ctrl Pts',(6.00008918129249,6.17717203250874,7.80958676236975));
#51446=CARTESIAN_POINT('Ctrl Pts',(6.00007044381521,6.18218988379821,7.79707102198934));
#51447=CARTESIAN_POINT('Ctrl Pts',(6.00005227277352,6.18742746363513,7.78463200772731));
#51448=CARTESIAN_POINT('Ctrl Pts',(6.00003127527203,6.19279782868115,7.77248562475542));
#51449=CARTESIAN_POINT('Ctrl Pts',(6.00001008664516,6.19821707635837,7.76022868185808));
#51450=CARTESIAN_POINT('Ctrl Pts',(5.99998556854563,6.20377138573136,7.74827022814555));
#51451=CARTESIAN_POINT('Ctrl Pts',(5.99996740877935,6.20932028803311,7.73682129885285));
#51452=CARTESIAN_POINT('Ctrl Pts',(5.99995691476844,6.21252684038545,7.73020528920647));
#51453=CARTESIAN_POINT('Ctrl Pts',(5.99994883619827,6.21573063522951,7.72375917760543));
#51454=CARTESIAN_POINT('Ctrl Pts',(5.99994773775714,6.21889758122576,7.71752118994764));
#51455=CARTESIAN_POINT('Ctrl Pts',(5.99994375377365,6.2303839142034,7.6948963635589));
#51456=CARTESIAN_POINT('Ctrl Pts',(5.99996351071227,6.24267211096661,7.67263884761238));
#51457=CARTESIAN_POINT('Ctrl Pts',(5.99998940177669,6.2557542052183,7.65091230797903));
#51458=CARTESIAN_POINT('Ctrl Pts',(6.00001515384743,6.26876606950817,7.62930240517918));
#51459=CARTESIAN_POINT('Ctrl Pts',(6.00004625470305,6.28256328239365,7.60821873855136));
#51460=CARTESIAN_POINT('Ctrl Pts',(6.00006686787884,6.29708667041071,7.58781913651103));
#51461=CARTESIAN_POINT('Ctrl Pts',(6.0000726178758,6.3011379353728,7.58212871545434));
#51462=CARTESIAN_POINT('Ctrl Pts',(6.00007759523361,6.30524540300111,7.57649145646077));
#51463=CARTESIAN_POINT('Ctrl Pts',(6.00008158486497,6.30940710200007,7.57091058889349));
#51464=CARTESIAN_POINT('Ctrl Pts',(6.00009591088445,6.32435098414694,7.55087073804807));
#51465=CARTESIAN_POINT('Ctrl Pts',(6.00009642673619,6.33999756707795,7.53155982479057));
#51466=CARTESIAN_POINT('Ctrl Pts',(6.00008390520131,6.35622965439619,7.51311008864557));
#51467=CARTESIAN_POINT('Ctrl Pts',(6.0000712262293,6.37266583277199,7.49442837825795));
#51468=CARTESIAN_POINT('Ctrl Pts',(6.000044816293,6.38970156778594,7.47663037459175));
#51469=CARTESIAN_POINT('Ctrl Pts',(6.00002344711442,6.40717531708069,7.45982218522411));
#51470=CARTESIAN_POINT('Ctrl Pts',(6.00001019823316,6.41800903391686,7.44940111524846));
#51471=CARTESIAN_POINT('Ctrl Pts',(5.99999928041887,6.42901037243094,7.43935984833557));
#51472=CARTESIAN_POINT('Ctrl Pts',(5.99999922550778,6.44013547507157,7.42971620739118));
#51473=CARTESIAN_POINT('Ctrl Pts',(5.73278343882478,6.65588366033016,8.10254996066954));
#51474=CARTESIAN_POINT('Ctrl Pts',(5.74652216226264,6.64290705362911,8.09796672996633));
#51475=CARTESIAN_POINT('Ctrl Pts',(5.75957819268944,6.6297391121596,8.09404270281397));
#51476=CARTESIAN_POINT('Ctrl Pts',(5.77191402195044,6.6165246743462,8.09067264558843));
#51477=CARTESIAN_POINT('Ctrl Pts',(5.78455326508681,6.60298521227193,8.08721969793848));
#51478=CARTESIAN_POINT('Ctrl Pts',(5.79643718469295,6.58939758209051,8.08434749272246));
#51479=CARTESIAN_POINT('Ctrl Pts',(5.80757705713372,6.57590082893888,8.08195774837986));
#51480=CARTESIAN_POINT('Ctrl Pts',(5.81921372581329,6.56180217157,8.07946143046495));
#51481=CARTESIAN_POINT('Ctrl Pts',(5.83003943422937,6.54780315409756,8.07749092628001));
#51482=CARTESIAN_POINT('Ctrl Pts',(5.84010967404772,6.53403521658879,8.07596191120139));
#51483=CARTESIAN_POINT('Ctrl Pts',(5.84591284550348,6.52610117495753,8.07508078653904));
#51484=CARTESIAN_POINT('Ctrl Pts',(5.85146583339613,6.5182433251846,8.07434684899726));
#51485=CARTESIAN_POINT('Ctrl Pts',(5.85678336455151,6.51048234910576,8.07374880498796));
#51486=CARTESIAN_POINT('Ctrl Pts',(5.8670115993516,6.49555416471101,8.07259847142729));
#51487=CARTESIAN_POINT('Ctrl Pts',(5.87634426622871,6.4809886970225,8.07192749106764));
#51488=CARTESIAN_POINT('Ctrl Pts',(5.88485691334425,6.46691376275036,8.07161710097136));
#51489=CARTESIAN_POINT('Ctrl Pts',(5.88966062429399,6.458971237357,8.07144194695828));
#51490=CARTESIAN_POINT('Ctrl Pts',(5.89420384053122,6.4511843623423,8.07138221398306));
#51491=CARTESIAN_POINT('Ctrl Pts',(5.89850363154804,6.44357186666483,8.07142126578559));
#51492=CARTESIAN_POINT('Ctrl Pts',(5.90446335283279,6.43302057420861,8.07147539349966));
#51493=CARTESIAN_POINT('Ctrl Pts',(5.90995415386343,6.42280438722931,8.0717172162624));
#51494=CARTESIAN_POINT('Ctrl Pts',(5.9150194297642,6.41296495876872,8.07210178476554));
#51495=CARTESIAN_POINT('Ctrl Pts',(5.91755206771458,6.40804524453842,8.07229406901711));
#51496=CARTESIAN_POINT('Ctrl Pts',(5.91997825702204,6.40321969767778,8.07252206789));
#51497=CARTESIAN_POINT('Ctrl Pts',(5.92230356304916,6.39849258665512,8.0727806332584));
#51498=CARTESIAN_POINT('Ctrl Pts',(5.92346621606272,6.39612903114379,8.07290991594259));
#51499=CARTESIAN_POINT('Ctrl Pts',(5.92460364371983,6.39379008282668,8.0730468424592));
#51500=CARTESIAN_POINT('Ctrl Pts',(5.92571653121906,6.3914762444007,8.0731907941147));
#51501=CARTESIAN_POINT('Ctrl Pts',(5.92650181455179,6.38984353781373,8.0732923702721));
#51502=CARTESIAN_POINT('Ctrl Pts',(5.9269696212441,6.38886378412244,8.07335487663796));
#51503=CARTESIAN_POINT('Ctrl Pts',(5.92776753993371,6.3871818633714,8.07346749913357));
#51504=CARTESIAN_POINT('Ctrl Pts',(5.92810041531301,6.38648020038837,8.07351448293836));
#51505=CARTESIAN_POINT('Ctrl Pts',(5.92849041668746,6.38565619733019,8.0735703947824));
#51506=CARTESIAN_POINT('Ctrl Pts',(5.92898224825978,6.38461054370544,8.07364311834452));
#51507=CARTESIAN_POINT('Ctrl Pts',(5.93824263884224,6.36492258237076,8.0750123850361));
#51508=CARTESIAN_POINT('Ctrl Pts',(5.94647893757245,6.34554238942372,8.07701435392396));
#51509=CARTESIAN_POINT('Ctrl Pts',(5.95372901404908,6.32660267221935,8.07949390178515));
#51510=CARTESIAN_POINT('Ctrl Pts',(5.96117537732152,6.30715018574758,8.08204058031818));
#51511=CARTESIAN_POINT('Ctrl Pts',(5.96758228145031,6.28816272684888,8.08509044760169));
#51512=CARTESIAN_POINT('Ctrl Pts',(5.97303224009227,6.26975867528639,8.08850160394176));
#51513=CARTESIAN_POINT('Ctrl Pts',(5.9787505155944,6.2504485402737,8.09208070114504));
#51514=CARTESIAN_POINT('Ctrl Pts',(5.98341631050524,6.2317809266297,8.09605707728519));
#51515=CARTESIAN_POINT('Ctrl Pts',(5.9871551247652,6.21385976069274,8.10030389064878));
#51516=CARTESIAN_POINT('Ctrl Pts',(5.99100606181786,6.19540115934611,8.10467806112115));
#51517=CARTESIAN_POINT('Ctrl Pts',(5.99387471606403,6.17773434412722,8.1093391054874));
#51518=CARTESIAN_POINT('Ctrl Pts',(5.9959123780958,6.16093782306683,8.11419052900978));
#51519=CARTESIAN_POINT('Ctrl Pts',(5.99805099892841,6.14330909499754,8.11928232306151));
#51520=CARTESIAN_POINT('Ctrl Pts',(5.99927528159734,6.12663881069711,8.12458397046569));
#51521=CARTESIAN_POINT('Ctrl Pts',(5.99975824748392,6.11098214001741,8.13002891614501));
#51522=CARTESIAN_POINT('Ctrl Pts',(5.99992154067033,6.10568854120467,8.13186987956394));
#51523=CARTESIAN_POINT('Ctrl Pts',(6.0000000065821,6.10051054258625,8.13372757636712));
#51524=CARTESIAN_POINT('Ctrl Pts',(5.99999999999929,6.09544950676928,8.13560044756764));
#51525=CARTESIAN_POINT('Ctrl Pts',(5.99968415523845,6.00656139605184,8.08769837817367));
#51526=CARTESIAN_POINT('Ctrl Pts',(5.99968415523845,6.35078816638231,8.34790825714588));
#51527=CARTESIAN_POINT('Ctrl Pts',(5.99968415523845,7.06928852668172,8.96885076597258));
#51528=CARTESIAN_POINT('Ctrl Pts',(5.99968415523845,8.03053011388277,10.075949619057));
#51529=CARTESIAN_POINT('Ctrl Pts',(5.99968415523845,8.85193945551654,11.3901955327746));
#51530=CARTESIAN_POINT('Ctrl Pts',(5.99968415523845,9.45913036146108,12.8152579698838));
#51531=CARTESIAN_POINT('Ctrl Pts',(5.99968415523845,9.83821289603149,14.3183256849662));
#51532=CARTESIAN_POINT('Ctrl Pts',(5.99968415523845,9.96603145443171,15.7255914318733));
#51533=CARTESIAN_POINT('Ctrl Pts',(5.99968415523845,9.92625398667906,16.6207279726114));
#51534=CARTESIAN_POINT('Ctrl Pts',(5.99968415523845,9.8878432222398,16.9970837242003));
#51535=CARTESIAN_POINT('Ctrl Pts',(6.00710925937989,6.11916148493871,7.93873236047488));
#51536=CARTESIAN_POINT('Ctrl Pts',(6.00710925937989,6.46990577187445,8.20386673730895));
#51537=CARTESIAN_POINT('Ctrl Pts',(6.00710925937989,7.20187340659612,8.83644658604556));
#51538=CARTESIAN_POINT('Ctrl Pts',(6.00710925937989,8.18131791270368,9.96451835081638));
#51539=CARTESIAN_POINT('Ctrl Pts',(6.00710925937989,9.0181474918832,11.3034312647952));
#51540=CARTESIAN_POINT('Ctrl Pts',(6.00710925937989,9.63683604404024,12.7554734616408));
#51541=CARTESIAN_POINT('Ctrl Pts',(6.00710925937989,10.0230315315726,14.2867682665207));
#51542=CARTESIAN_POINT('Ctrl Pts',(6.00710925937989,10.1532734887705,15.7206563920744));
#51543=CARTESIAN_POINT('Ctrl Pts',(6.00710925937989,10.1127513948415,16.6325797415481));
#51544=CARTESIAN_POINT('Ctrl Pts',(6.00710925937989,10.0736127087543,17.0160475747281));
#51545=CARTESIAN_POINT('Ctrl Pts',(5.89995655749497,6.21158111094138,7.81646439622245));
#51546=CARTESIAN_POINT('Ctrl Pts',(5.89995655749497,6.56767482924154,8.08564069038753));
#51547=CARTESIAN_POINT('Ctrl Pts',(5.89995655749497,7.31069610057991,8.72777220655928));
#51548=CARTESIAN_POINT('Ctrl Pts',(5.89995655749497,8.30508115401766,9.87305806657078));
#51549=CARTESIAN_POINT('Ctrl Pts',(5.89995655749497,9.15456731811607,11.2322171007898));
#51550=CARTESIAN_POINT('Ctrl Pts',(5.89995655749497,9.78269288025933,12.7064036789539));
#51551=CARTESIAN_POINT('Ctrl Pts',(5.89995655749497,10.1747265199527,14.2608666456689));
#51552=CARTESIAN_POINT('Ctrl Pts',(5.89995655749497,10.3069575484958,15.7166058221585));
#51553=CARTESIAN_POINT('Ctrl Pts',(5.89995655749497,10.2658242821102,16.6423074075148));
#51554=CARTESIAN_POINT('Ctrl Pts',(5.89995655749497,10.226088134276,17.0316126776586));
#51555=CARTESIAN_POINT('Ctrl Pts',(5.72168991350276,6.2459107561173,7.77104746466054));
#51556=CARTESIAN_POINT('Ctrl Pts',(5.72168991350276,6.60399154240885,8.04172514542314));
#51557=CARTESIAN_POINT('Ctrl Pts',(5.72168991350276,7.35111873193133,8.68740466723007));
#51558=CARTESIAN_POINT('Ctrl Pts',(5.72168991350276,8.35105351231554,9.83908477278564));
#51559=CARTESIAN_POINT('Ctrl Pts',(5.72168991350276,9.20524101624623,11.2057643105373));
#51560=CARTESIAN_POINT('Ctrl Pts',(5.72168991350276,9.83687199405033,12.6881765090173));
#51561=CARTESIAN_POINT('Ctrl Pts',(5.72168991350276,10.2310742390599,14.2512453834785));
#51562=CARTESIAN_POINT('Ctrl Pts',(5.72168991350276,10.3640441162288,15.7151012215239));
#51563=CARTESIAN_POINT('Ctrl Pts',(5.72168991350276,10.3226838273516,16.6459207885187));
#51564=CARTESIAN_POINT('Ctrl Pts',(5.72168991350276,10.2827257499292,17.0373943983161));
#51565=CARTESIAN_POINT('Ctrl Pts',(5.99999999999929,6.09544950676928,8.13560044756764));
#51566=CARTESIAN_POINT('Ctrl Pts',(5.9999999999993,6.21599272915026,8.22864748093463));
#51567=CARTESIAN_POINT('Ctrl Pts',(6.00000000006295,6.33400221607625,8.32414772917356));
#51568=CARTESIAN_POINT('Ctrl Pts',(5.99999999822618,6.44958311156655,8.422124980624));
#51569=CARTESIAN_POINT('Ctrl Pts',(5.99999999638109,6.56568781639286,8.52054626219558));
#51570=CARTESIAN_POINT('Ctrl Pts',(5.99999999247689,6.67934219993644,8.62146736838768));
#51571=CARTESIAN_POINT('Ctrl Pts',(5.99999999188347,6.79061972240305,8.72495313863626));
#51572=CARTESIAN_POINT('Ctrl Pts',(5.99999999151144,6.86038184500564,8.78983045466269));
#51573=CARTESIAN_POINT('Ctrl Pts',(5.99999999284036,6.92920911788454,8.8557165489303));
#51574=CARTESIAN_POINT('Ctrl Pts',(5.99999999533528,6.99711214007891,8.92263466848373));
#51575=CARTESIAN_POINT('Ctrl Pts',(5.99999999728228,7.05010275404376,8.97485667754776));
#51576=CARTESIAN_POINT('Ctrl Pts',(5.99999999999971,7.10253038140868,9.02770730633247));
#51577=CARTESIAN_POINT('Ctrl Pts',(5.99999999999971,7.15440146857915,9.08120097285816));
#51578=CARTESIAN_POINT('Ctrl Pts',(5.99999999999971,7.28007178588764,9.21080238306546));
#51579=CARTESIAN_POINT('Ctrl Pts',(5.999999984904,7.40251839100925,9.34411442180928));
#51580=CARTESIAN_POINT('Ctrl Pts',(5.99999998011157,7.5213665288948,9.48080996079188));
#51581=CARTESIAN_POINT('Ctrl Pts',(5.99999997532264,7.64012751541815,9.61740526090964));
#51582=CARTESIAN_POINT('Ctrl Pts',(5.99999998034514,7.75529499347647,9.75737878109644));
#51583=CARTESIAN_POINT('Ctrl Pts',(5.99999998874861,7.86653171168378,9.90036730327227));
#51584=CARTESIAN_POINT('Ctrl Pts',(5.99999999244904,7.915514355194,9.96333172653706));
#51585=CARTESIAN_POINT('Ctrl Pts',(5.99999999643384,7.96373531284376,10.0268803217595));
#51586=CARTESIAN_POINT('Ctrl Pts',(5.99999999855295,8.01116828547801,10.0909800599343));
#51587=CARTESIAN_POINT('Ctrl Pts',(5.99999999944824,8.03120793721771,10.118061146324));
#51588=CARTESIAN_POINT('Ctrl Pts',(5.9999999999997,8.05110695913799,10.1452405932687));
#51589=CARTESIAN_POINT('Ctrl Pts',(5.9999999999997,8.07086366361946,10.1725155424444));
#51590=CARTESIAN_POINT('Ctrl Pts',(5.9999999999997,8.19463793080481,10.3433910470058));
#51591=CARTESIAN_POINT('Ctrl Pts',(5.99999998499452,8.31277452188091,10.5180623042338));
#51592=CARTESIAN_POINT('Ctrl Pts',(5.99999998425411,8.42519108889713,10.6962951891408));
#51593=CARTESIAN_POINT('Ctrl Pts',(5.9999999835127,8.53775753234144,10.8747656983488));
#51594=CARTESIAN_POINT('Ctrl Pts',(5.99999999342451,8.64458901980545,11.0568078073897));
#51595=CARTESIAN_POINT('Ctrl Pts',(5.99999999807136,8.74556121729957,11.2422176425727));
#51596=CARTESIAN_POINT('Ctrl Pts',(5.99999999924405,8.77104273958086,11.2890079963893));
#51597=CARTESIAN_POINT('Ctrl Pts',(5.99999999999971,8.79615088361354,11.3360129638309));
#51598=CARTESIAN_POINT('Ctrl Pts',(5.99999999999971,8.82088319339553,11.3832295268562));
#51599=CARTESIAN_POINT('Ctrl Pts',(5.9999999999997,8.82409824626035,11.3893673986344));
#51600=CARTESIAN_POINT('Ctrl Pts',(5.99999999998697,8.82730698839302,11.395508823316));
#51601=CARTESIAN_POINT('Ctrl Pts',(5.99999999996269,8.83050940751732,11.4016537827019));
#51602=CARTESIAN_POINT('Ctrl Pts',(5.99999999919991,8.93112302668215,11.5947161456975));
#51603=CARTESIAN_POINT('Ctrl Pts',(5.99999999014648,9.02549152491428,11.7912698092488));
#51604=CARTESIAN_POINT('Ctrl Pts',(5.99999998974637,9.11332588235521,11.9907230388185));
#51605=CARTESIAN_POINT('Ctrl Pts',(5.99999998934601,9.20121618416255,12.1903033061998));
#51606=CARTESIAN_POINT('Ctrl Pts',(5.99999999678082,9.28256378678173,12.3927863257178));
#51607=CARTESIAN_POINT('Ctrl Pts',(5.99999999936896,9.3571261646783,12.5975570160648));
#51608=CARTESIAN_POINT('Ctrl Pts',(5.99999999976094,9.36841888658775,12.6285702230806));
#51609=CARTESIAN_POINT('Ctrl Pts',(5.9999999999997,9.37955605981923,12.6596358719235));
#51610=CARTESIAN_POINT('Ctrl Pts',(5.9999999999997,9.39053694094342,12.690751792812));
#51611=CARTESIAN_POINT('Ctrl Pts',(5.9999999999997,9.40603018940343,12.7346541616597));
#51612=CARTESIAN_POINT('Ctrl Pts',(5.99999999951884,9.42121086917364,12.7786568707967));
#51613=CARTESIAN_POINT('Ctrl Pts',(5.99999999869869,9.43607805733177,12.8227576339477));
#51614=CARTESIAN_POINT('Ctrl Pts',(5.99999999492022,9.50457105013169,13.0259294254691));
#51615=CARTESIAN_POINT('Ctrl Pts',(5.99999998426479,9.56641442502825,13.2311813385896));
#51616=CARTESIAN_POINT('Ctrl Pts',(5.99999998403914,9.62153670788177,13.4382622973276));
#51617=CARTESIAN_POINT('Ctrl Pts',(5.99999998381348,9.6766589907353,13.6453432560655));
#51618=CARTESIAN_POINT('Ctrl Pts',(5.99999999999971,9.72506028807675,13.8542538365966));
#51619=CARTESIAN_POINT('Ctrl Pts',(5.99999999999971,9.76661736553527,14.0647507043716));
#51620=CARTESIAN_POINT('Ctrl Pts',(5.99999999999971,9.78347351328543,14.1501312585673));
#51621=CARTESIAN_POINT('Ctrl Pts',(5.99999999594492,9.79921712968305,14.235772411136));
#51622=CARTESIAN_POINT('Ctrl Pts',(5.99999999152506,9.81383325134206,14.3216199403523));
#51623=CARTESIAN_POINT('Ctrl Pts',(5.99999998224973,9.84450604590268,14.5017760507502));
#51624=CARTESIAN_POINT('Ctrl Pts',(5.9999999734632,9.87021006131464,14.682841403213));
#51625=CARTESIAN_POINT('Ctrl Pts',(5.99999997653297,9.89090683235236,14.8643171280013));
#51626=CARTESIAN_POINT('Ctrl Pts',(5.99999997960657,9.91162946133668,15.0460195833067));
#51627=CARTESIAN_POINT('Ctrl Pts',(5.99999999486873,9.92733230893222,15.2281329800598));
#51628=CARTESIAN_POINT('Ctrl Pts',(5.9999999991423,9.93802883787374,15.4101537132592));
#51629=CARTESIAN_POINT('Ctrl Pts',(5.99999999968371,9.93938395859166,15.433213536497));
#51630=CARTESIAN_POINT('Ctrl Pts',(5.9999999999997,9.94065879737618,15.4562718740799));
#51631=CARTESIAN_POINT('Ctrl Pts',(5.9999999999997,9.94185344127986,15.479327704528));
#51632=CARTESIAN_POINT('Ctrl Pts',(5.9999999999997,9.94848717375989,15.6073543163301));
#51633=CARTESIAN_POINT('Ctrl Pts',(5.99999999304439,9.95260845370109,15.7352949668062));
#51634=CARTESIAN_POINT('Ctrl Pts',(5.99999999143195,9.95424492247683,15.8632214076251));
#51635=CARTESIAN_POINT('Ctrl Pts',(5.99999998950812,9.95619741266735,16.0158519524361));
#51636=CARTESIAN_POINT('Ctrl Pts',(5.99999999273625,9.95461404479101,16.1684624668109));
#51637=CARTESIAN_POINT('Ctrl Pts',(5.99999999547189,9.94950734202748,16.3211471683246));
#51638=CARTESIAN_POINT('Ctrl Pts',(5.99999999819524,9.94442356206008,16.4731465038703));
#51639=CARTESIAN_POINT('Ctrl Pts',(5.99999999961476,9.93584800483817,16.6252198213967));
#51640=CARTESIAN_POINT('Ctrl Pts',(5.99999999985072,9.92374152693551,16.7774586800326));
#51641=CARTESIAN_POINT('Ctrl Pts',(5.99999999991369,9.92051092369794,16.8180834887958));
#51642=CARTESIAN_POINT('Ctrl Pts',(5.99999999993325,9.91702860387934,16.8587200565166));
#51643=CARTESIAN_POINT('Ctrl Pts',(5.99999999993294,9.9132931986081,16.8993700414499));
#51644=CARTESIAN_POINT('Origin',(7.4,0.,0.));
#51645=CARTESIAN_POINT('',(7.4,5.99999999991914,-10.3923048454599));
#51646=CARTESIAN_POINT('Origin',(7.4,6.74999999990903,-11.6913429511424));
#51647=CARTESIAN_POINT('Origin',(7.4,6.74999999990903,-11.6913429511424));
#51648=CARTESIAN_POINT('',(6.,5.99999999991914,-10.3923048454599));
#51649=CARTESIAN_POINT('',(7.4,5.99999999991914,-10.3923048454599));
#51650=CARTESIAN_POINT('Origin',(6.,6.74999999990903,-11.6913429511424));
#51651=CARTESIAN_POINT('Origin',(7.4,-6.62945397692566E-15,1.14825511146811E-14));
#51652=CARTESIAN_POINT('',(7.4,6.00000000008095,10.3923048453666));
#51653=CARTESIAN_POINT('Origin',(7.4,6.75000000009103,11.6913429510374));
#51654=CARTESIAN_POINT('Origin',(7.4,6.75000000009103,11.6913429510374));
#51655=CARTESIAN_POINT('',(6.,6.00000000008095,10.3923048453666));
#51656=CARTESIAN_POINT('',(7.4,6.00000000008095,10.3923048453666));
#51657=CARTESIAN_POINT('Origin',(6.,6.75000000009103,11.6913429510374));
#51658=CARTESIAN_POINT('Origin',(6.,0.,0.));
#57020=UNCERTAINTY_MEASURE_WITH_UNIT(LENGTH_MEASURE(0.01),#57080,
'DISTANCE_ACCURACY_VALUE',
'Maximum model space distance between geometric entities at asserted c
onnectivities');
#57040=UNCERTAINTY_MEASURE_WITH_UNIT(LENGTH_MEASURE(0.01),#57080,
'DISTANCE_ACCURACY_VALUE',
'Maximum model space distance between geometric entities at asserted c
onnectivities');
#57059=(
GEOMETRIC_REPRESENTATION_CONTEXT(3)
GLOBAL_UNCERTAINTY_ASSIGNED_CONTEXT((#57020))
GLOBAL_UNIT_ASSIGNED_CONTEXT((#57080,#57082,#57083))
REPRESENTATION_CONTEXT('','3D')
);
#57079=(
GEOMETRIC_REPRESENTATION_CONTEXT(3)
GLOBAL_UNCERTAINTY_ASSIGNED_CONTEXT((#57040))
GLOBAL_UNIT_ASSIGNED_CONTEXT((#57080,#57082,#57083))
REPRESENTATION_CONTEXT('','3D')
);
#57080=(
LENGTH_UNIT()
NAMED_UNIT(*)
SI_UNIT(.MILLI.,.METRE.)
);
#57082=(
NAMED_UNIT(*)
PLANE_ANGLE_UNIT()
SI_UNIT($,.RADIAN.)
);
#57083=(
NAMED_UNIT(*)
SI_UNIT($,.STERADIAN.)
SOLID_ANGLE_UNIT()
);
#57102=SHAPE_DEFINITION_REPRESENTATION(#57148,#57267);
#57148=PRODUCT_DEFINITION_SHAPE('',$,#57306);
#57267=SHAPE_REPRESENTATION('',(#25470),#57059);
#57287=PRODUCT_DEFINITION_CONTEXT('part definition',#57403,'design');
#57306=PRODUCT_DEFINITION('Coupling Spider','Coupling Spider',#57344,#57287);
#57344=PRODUCT_DEFINITION_FORMATION('',$,#57423);
#57403=APPLICATION_CONTEXT(
'Core Data for Automotive Mechanical Design Process');
#57404=PRODUCT_CONTEXT('part definition',#57403,'mechanical');
#57423=PRODUCT('Coupling Spider','Coupling Spider',$,(#57404));
#57444=PRESENTATION_STYLE_ASSIGNMENT((#57446));
#57446=SURFACE_STYLE_USAGE(.BOTH.,#57448);
#57448=SURFACE_SIDE_STYLE('',(#57450));
#57450=SURFACE_STYLE_FILL_AREA(#57452);
#57452=FILL_AREA_STYLE('Opaque(202,209,238)',(#57454));
#57454=FILL_AREA_STYLE_COLOUR('Opaque(202,209,238)',#57456);
#57456=COLOUR_RGB('Opaque(202,209,238)',0.792156862745098,0.819607843137255,
0.933333333333333);
ENDSEC;
END-ISO-10303-21;
